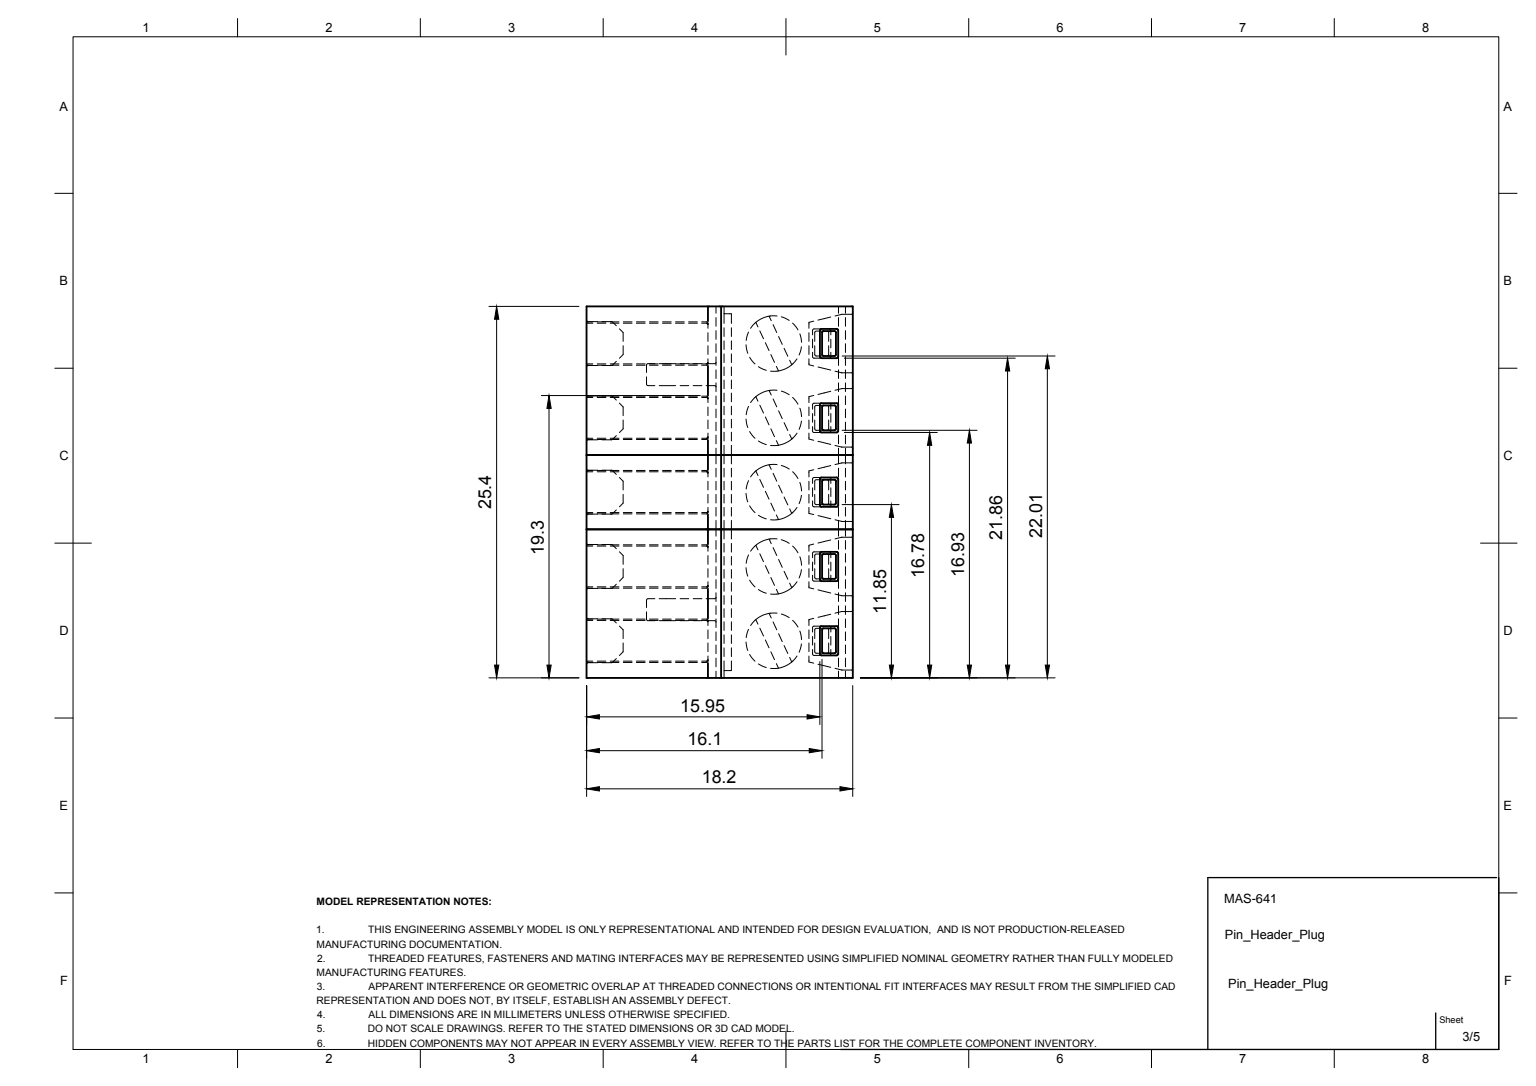
ISO-10303-21;
HEADER;
FILE_DESCRIPTION((''),'2;1');
FILE_NAME('Pin_Header_Plug.step','2026-10-09T09:55:32-07:00',(''),(''),'','','');
FILE_SCHEMA (('AUTOMOTIVE_DESIGN { 1 0 10303 214 3 1 1 }'));
ENDSEC;
DATA;
#10=MECHANICAL_DESIGN_GEOMETRIC_PRESENTATION_REPRESENTATION('',(#79661,#79662,#79663,#79664,#79665,#79666,#79667,#79668,#79669,#79670,#79671,#79672,#79673,#79674,#79675,#79676,#79677,#79678,#79679,#79680,#79681,#79682,#79683,#79684,#79685,#79686,#79687,#79688,#79689,#79690,#79691,#79692,#79693,#79694,#79695,#79696,#79697,#79698,#79699,#79700,#79701,#79702,#79703,#79704,#79705,#79706,#79707,#79708,#79709,#79710,#79711,#79712,#79713,#79714,#79715,#79716,#79717,#79718,#79719,#79720,#79721,#79722,#79723,#79724,#79725,#79726,#79727,#79728,#79729,#79730,#79731,#79732,#79733,#79734,#79735,#79736,#79737,#79738,#79739,#79740,#79741,#79742,#79743,#79744,#79745,#79746,#79747,#79748,#79749,#79750,#79751,#79752,#79753,#79754,#79755,#79756,#79757,#79758,#79759,#79760,#79761,#79762,#79763,#79764,#79765,#79766,#79767,#79768,#79769,#79770,#79771,#79772,#79773,#79774,#79775,#79776,#79777,#79778,#79779,#79780,#79781,#79782,#79783,#79784,#79785,#79786,#79787,#79788,#79789,#79790,#79791,#79792,#79793,#79794,#79795,#79796,#79797,#79798,#79799,#79800,#79801,#79802,#79803,#79804,#79805,#79806,#79807,#79808,#79809,#79810,#79811,#79812,#79813,#79814,#79815,#79816,#79817,#79818,#79819,#79820,#79821,#79822,#79823,#79824,#79825,#79826,#79827,#79828,#79829,#79830,#79831,#79832,#79833,#79834,#79835,#79836,#79837,#79838,#79839,#79840,#79841,#79842,#79843,#79844,#79845,#79846,#79847,#79848,#79849,#79850,#79851,#79852,#79853,#79854,#79855,#79856,#79857,#79858,#79859,#79860,#79861,#79862,#79863,#79864,#79865,#79866,#79867,#79868,#79869,#79870,#79871,#79872,#79873,#79874,#79875,#79876,#79877,#79878,#79879,#79880,#79881,#79882,#79883,#79884,#79885,#79886,#79887,#79888,#79889,#79890,#79891,#79892,#79893,#79894,#79895,#79896,#79897,#79898,#79899,#79900,#79901,#79902,#79903,#79904,#79905,#79906,#79907,#79908,#79909,#79910,#79911,#79912,#79913,#79914,#79915,#79916,#79917,#79918,#79919,#79920,#79921,#79922,#79923,#79924,#79925,#79926,#79927,#79928,#79929,#79930,#79931,#79932,#79933,#79934,#79935,#79936,#79937,#79938,#79939,#79940,#79941,#79942,#79943,#79944,#79945,#79946,#79947,#79948,#79949,#79950,#79951,#79952,#79953,#79954,#79955,#79956,#79957,#79958,#79959,#79960,#79961,#79962,#79963,#79964,#79965,#79966,#79967,#79968,#79969,#79970,#79971,#79972,#79973,#79974,#79975,#79976,#79977,#79978,#79979,#79980,#79981,#79982,#79983,#79984,#79985,#79986,#79987,#79988,#79989,#79990,#79991,#79992,#79993,#79994,#79995,#79996,#79997,#79998,#79999,#80000,#80001,#80002,#80003,#80004,#80005,#80006,#80007,#80008,#80009,#80010,#80011,#80012,#80013,#80014,#80015,#80016,#80017,#80018,#80019,#80020,#80021,#80022,#80023,#80024,#80025,#80026,#80027,#80028,#80029,#80030,#80031,#80032,#80033,#80034,#80035,#80036,#80037,#80038,#80039,#80040,#80041,#80042,#80043,#80044,#80045,#80046,#80047,#80048,#80049,#80050,#80051,#80052,#80053,#80054,#80055,#80056,#80057,#80058,#80059,#80060,#80061,#80062,#80063,#80064,#80065,#80066,#80067,#80068,#80069,#80070,#80071,#80072,#80073,#80074,#80075,#80076,#80077,#80078,#80079,#80080,#80081,#80082,#80083,#80084,#80085,#80086,#80087,#80088,#80089,#80090,#80091,#80092,#80093,#80094,#80095,#80096,#80097,#80098,#80099,#80100,#80101,#80102,#80103,#80104,#80105,#80106,#80107,#80108,#80109,#80110,#80111,#80112,#80113,#80114,#80115,#80116,#80117,#80118,#80119,#80120,#80121,#80122,#80123,#80124,#80125,#80126,#80127,#80128,#80129,#80130,#80131,#80132,#80133,#80134,#80135,#80136,#80137,#80138,#80139,#80140,#80141,#80142,#80143,#80144,#80145,#80146,#80147,#80148,#80149,#80150,#80151,#80152,#80153,#80154,#80155,#80156,#80157,#80158,#80159,#80160,#80161,#80162,#80163,#80164,#80165,#80166,#80167,#80168,#80169,#80170,#80171,#80172,#80173,#80174,#80175,#80176,#80177,#80178,#80179,#80180,#80181,#80182,#80183,#80184,#80185,#80186,#80187,#80188,#80189,#80190,#80191,#80192,#80193,#80194,#80195,#80196,#80197,#80198,#80199,#80200,#80201,#80202,#80203,#80204,#80205,#80206,#80207,#80208,#80209,#80210,#80211,#80212,#80213,#80214,#80215,#80216,#80217,#80218,#80219,#80220,#80221,#80222,#80223,#80224,#80225,#80226,#80227,#80228,#80229,#80230,#80231,#80232,#80233,#80234,#80235,#80236,#80237,#80238,#80239,#80240,#80241,#80242,#80243,#80244,#80245,#80246,#80247,#80248,#80249,#80250,#80251,#80252,#80253,#80254,#80255,#80256,#80257,#80258,#80259,#80260,#80261,#80262,#80263,#80264,#80265,#80266,#80267,#80268,#80269,#80270,#80271,#80272,#80273,#80274,#80275,#80276,#80277,#80278,#80279,#80280,#80281,#80282,#80283,#80284,#80285,#80286,#80287,#80288,#80289,#80290,#80291,#80292,#80293,#80294,#80295,#80296,#80297,#80298,#80299,#80300,#80301,#80302,#80303,#80304,#80305,#80306,#80307,#80308,#80309,#80310,#80311,#80312,#80313,#80314,#80315,#80316,#80317,#80318,#80319,#80320,#80321,#80322,#80323,#80324,#80325,#80326,#80327,#80328,#80329,#80330,#80331,#80332,#80333,#80334,#80335,#80336,#80337,#80338,#80339,#80340,#80341,#80342,#80343,#80344,#80345,#80346,#80347,#80348,#80349,#80350,#80351,#80352,#80353,#80354,#80355,#80356,#80357,#80358,#80359,#80360,#80361,#80362,#80363,#80364,#80365,#80366,#80367,#80368,#80369,#80370,#80371,#80372,#80373,#80374,#80375,#80376,#80377,#80378,#80379,#80380,#80381,#80382,#80383,#80384,#80385,#80386,#80387,#80388,#80389,#80390,#80391,#80392,#80393,#80394,#80395,#80396,#80397,#80398,#80399,#80400,#80401,#80402,#80403,#80404,#80405,#80406,#80407,#80408,#80409,#80410,#80411,#80412,#80413,#80414,#80415,#80416,#80417,#80418,#80419,#80420,#80421,#80422,#80423,#80424,#80425,#80426,#80427,#80428,#80429,#80430,#80431,#80432,#80433,#80434,#80435,#80436,#80437,#80438,#80439,#80440,#80441,#80442,#80443,#80444,#80445,#80446,#80447,#80448,#80449,#80450,#80451,#80452,#80453,#80454,#80455,#80456,#80457,#80458,#80459,#80460,#80461,#80462,#80463,#80464,#80465,#80466,#80467,#80468,#80469,#80470,#80471,#80472,#80473,#80474,#80475,#80476,#80477,#80478,#80479,#80480,#80481,#80482,#80483,#80484,#80485,#80486,#80487,#80488,#80489,#80490,#80491,#80492,#80493,#80494,#80495,#80496,#80497,#80498,#80499,#80500,#80501,#80502,#80503,#80504,#80505,#80506,#80507,#80508,#80509,#80510,#80511,#80512,#80513,#80514,#80515,#80516,#80517,#80518,#80519,#80520,#80521,#80522,#80523,#80524,#80525,#80526,#80527,#80528,#80529,#80530,#80531,#80532,#80533,#80534,#80535,#80536,#80537,#80538,#80539,#80540,#80541,#80542,#80543,#80544,#80545,#80546,#80547,#80548,#80549,#80550,#80551,#80552,#80553,#80554,#80555,#80556,#80557,#80558,#80559,#80560,#80561,#80562,#80563,#80564,#80565,#80566,#80567,#80568,#80569,#80570,#80571,#80572,#80573,#80574,#80575,#80576,#80577,#80578,#80579,#80580,#80581,#80582,#80583,#80584,#80585,#80586,#80587,#80588,#80589,#80590,#80591,#80592,#80593,#80594,#80595,#80596,#80597,#80598,#80599,#80600,#80601,#80602,#80603,#80604,#80605,#80606,#80607,#80608,#80609,#80610,#80611,#80612,#80613,#80614,#80615,#80616,#80617,#80618,#80619,#80620,#80621,#80622,#80623,#80624,#80625,#80626,#80627,#80628,#80629,#80630,#80631,#80632,#80633,#80634,#80635,#80636,#80637,#80638,#80639,#80640,#80641,#80642,#80643,#80644,#80645,#80646,#80647,#80648,#80649,#80650,#80651,#80652,#80653,#80654,#80655,#80656,#80657,#80658,#80659,#80660,#80661,#80662,#80663,#80664,#80665,#80666,#80667,#80668,#80669,#80670,#80671,#80672,#80673,#80674,#80675,#80676,#80677,#80678,#80679,#80680,#80681,#80682,#80683,#80684,#80685,#80686,#80687,#80688,#80689,#80690,#80691,#80692,#80693,#80694,#80695,#80696,#80697,#80698,#80699,#80700,#80701,#80702,#80703,#80704,#80705,#80706,#80707,#80708,#80709,#80710,#80711,#80712,#80713,#80714,#80715,#80716,#80717,#80718,#80719,#80720,#80721,#80722,#80723,#80724,#80725,#80726,#80727,#80728,#80729,#80730,#80731,#80732,#80733,#80734,#80735,#80736,#80737,#80738,#80739,#80740,#80741,#80742,#80743,#80744,#80745,#80746,#80747,#80748,#80749,#80750,#80751,#80752,#80753,#80754,#80755,#80756,#80757,#80758,#80759,#80760,#80761,#80762,#80763,#80764,#80765,#80766,#80767,#80768,#80769,#80770,#80771,#80772,#80773,#80774,#80775,#80776,#80777,#80778,#80779),#170127);
#23=SHAPE_REPRESENTATION_RELATIONSHIP('SRR','None',#170144,#26) ;
#26=ADVANCED_BREP_SHAPE_REPRESENTATION('',(#29,#30,#31),#170124) ;
#29=MANIFOLD_SOLID_BREP('Body1',#91083) ;
#30=MANIFOLD_SOLID_BREP('Body2',#91084) ;
#31=MANIFOLD_SOLID_BREP('Body3',#91085) ;
#34=(
BOUNDED_SURFACE()
B_SPLINE_SURFACE(3,2,((#133940,#133941,#133942),(#133943,#133944,#133945),
(#133946,#133947,#133948),(#133949,#133950,#133951),(#133952,#133953,#133954),
(#133955,#133956,#133957)),.UNSPECIFIED.,.F.,.F.,.F.)
B_SPLINE_SURFACE_WITH_KNOTS((4,2,4),(3,3),(3.14159265358979,3.92699081698724,
4.71238898038469),(0.,1.),.UNSPECIFIED.)
GEOMETRIC_REPRESENTATION_ITEM()
RATIONAL_B_SPLINE_SURFACE(((1.,0.934721701546417,1.),(1.,0.934869636336921,
1.),(1.,0.913780519322362,1.),(1.,0.83464631504231,1.),(1.,0.776518516961033,
1.),(1.,0.707106781186548,1.)))
REPRESENTATION_ITEM('')
SURFACE()
) ;
#35=(
BOUNDED_SURFACE()
B_SPLINE_SURFACE(3,2,((#133968,#133969,#133970),(#133971,#133972,#133973),
(#133974,#133975,#133976),(#133977,#133978,#133979)),.UNSPECIFIED.,.F.,
 .F.,.F.)
B_SPLINE_SURFACE_WITH_KNOTS((4,4),(3,3),(1.5707963267949,2.41495031290807),
(0.,1.),.UNSPECIFIED.)
GEOMETRIC_REPRESENTATION_ITEM()
RATIONAL_B_SPLINE_SURFACE(((1.,0.707106781186547,1.),(1.,0.730803471035897,
1.),(1.,0.752906082887246,1.),(1.,0.76729220397862,1.)))
REPRESENTATION_ITEM('')
SURFACE()
) ;
#36=(
BOUNDED_SURFACE()
B_SPLINE_SURFACE(3,2,((#133996,#133997,#133998),(#133999,#134000,#134001),
(#134002,#134003,#134004),(#134005,#134006,#134007),(#134008,#134009,#134010),
(#134011,#134012,#134013)),.UNSPECIFIED.,.F.,.F.,.F.)
B_SPLINE_SURFACE_WITH_KNOTS((4,2,4),(3,3),(1.56955149927804,2.35619449019234,
3.14283748110665),(-0.00124482751686043,1.),.UNSPECIFIED.)
GEOMETRIC_REPRESENTATION_ITEM()
RATIONAL_B_SPLINE_SURFACE(((1.00073060381457,0.70654415785643,1.),(1.00062673753069,
0.748263304672891,1.),(1.00053422463656,0.785422225437728,1.),(1.00040682904418,
0.836592203069559,1.),(1.00037181710676,0.850655170404881,1.),(1.00037229282027,
0.850464094333141,1.)))
REPRESENTATION_ITEM('')
SURFACE()
) ;
#37=(
BOUNDED_SURFACE()
B_SPLINE_SURFACE(3,2,((#134016,#134017,#134018),(#134019,#134020,#134021),
(#134022,#134023,#134024),(#134025,#134026,#134027),(#134028,#134029,#134030),
(#134031,#134032,#134033)),.UNSPECIFIED.,.F.,.F.,.F.)
B_SPLINE_SURFACE_WITH_KNOTS((4,2,4),(3,3),(4.71238898038469,5.49778714378214,
6.28318530717959),(0.,1.),.UNSPECIFIED.)
GEOMETRIC_REPRESENTATION_ITEM()
RATIONAL_B_SPLINE_SURFACE(((1.,0.707106781186548,1.),(1.,0.776518516961036,
1.),(1.,0.834646315042305,1.),(1.,0.913780519322366,1.),(1.,0.934869636336917,
1.),(1.,0.934721701546417,1.)))
REPRESENTATION_ITEM('')
SURFACE()
) ;
#38=(
BOUNDED_SURFACE()
B_SPLINE_SURFACE(3,2,((#134041,#134042,#134043),(#134044,#134045,#134046),
(#134047,#134048,#134049),(#134050,#134051,#134052)),.UNSPECIFIED.,.F.,
 .F.,.F.)
B_SPLINE_SURFACE_WITH_KNOTS((4,4),(3,3),(0.726642340681724,1.5707963267949),
(0.,1.),.UNSPECIFIED.)
GEOMETRIC_REPRESENTATION_ITEM()
RATIONAL_B_SPLINE_SURFACE(((1.,0.76729220397862,1.),(1.,0.752906082887247,
1.),(1.,0.730803471035896,1.),(1.,0.707106781186548,1.)))
REPRESENTATION_ITEM('')
SURFACE()
) ;
#39=(
BOUNDED_SURFACE()
B_SPLINE_SURFACE(3,2,((#134068,#134069,#134070),(#134071,#134072,#134073),
(#134074,#134075,#134076),(#134077,#134078,#134079),(#134080,#134081,#134082),
(#134083,#134084,#134085)),.UNSPECIFIED.,.F.,.F.,.F.)
B_SPLINE_SURFACE_WITH_KNOTS((4,2,4),(3,3),(-0.00124482751684684,0.785398163397448,
1.57204115431174),(-0.00124482751684684,1.),.UNSPECIFIED.)
GEOMETRIC_REPRESENTATION_ITEM()
RATIONAL_B_SPLINE_SURFACE(((1.00037229282026,0.850464094333143,1.),(1.00037181710676,
0.850655170404876,1.),(1.00040682904417,0.83659220306957,1.),(1.00053422463656,
0.785422225437723,1.),(1.00062673753069,0.748263304672901,1.),(1.00073060381456,
0.706544157856436,1.)))
REPRESENTATION_ITEM('')
SURFACE()
) ;
#40=(
BOUNDED_SURFACE()
B_SPLINE_SURFACE(3,2,((#134097,#134098,#134099),(#134100,#134101,#134102),
(#134103,#134104,#134105),(#134106,#134107,#134108)),.UNSPECIFIED.,.F.,
 .F.,.F.)
B_SPLINE_SURFACE_WITH_KNOTS((4,4),(3,3),(1.10714871779409,1.5707963267949),
(0.,1.),.UNSPECIFIED.)
GEOMETRIC_REPRESENTATION_ITEM()
RATIONAL_B_SPLINE_SURFACE(((1.,0.743704326447946,1.),(1.,0.73267692820235,
1.),(1.,0.720087778783133,1.),(1.,0.707106781186547,1.)))
REPRESENTATION_ITEM('')
SURFACE()
) ;
#41=(
BOUNDED_SURFACE()
B_SPLINE_SURFACE(3,2,((#134116,#134117,#134118),(#134119,#134120,#134121),
(#134122,#134123,#134124),(#134125,#134126,#134127)),.UNSPECIFIED.,.F.,
 .F.,.F.)
B_SPLINE_SURFACE_WITH_KNOTS((4,4),(3,3),(1.5707963267949,2.0344439357957),
(0.,1.),.UNSPECIFIED.)
GEOMETRIC_REPRESENTATION_ITEM()
RATIONAL_B_SPLINE_SURFACE(((1.,0.707106781186547,1.),(1.,0.720087778783132,
1.),(1.,0.73267692820235,1.),(1.,0.743704326447946,1.)))
REPRESENTATION_ITEM('')
SURFACE()
) ;
#42=(
BOUNDED_SURFACE()
B_SPLINE_SURFACE(3,2,((#134402,#134403,#134404),(#134405,#134406,#134407),
(#134408,#134409,#134410),(#134411,#134412,#134413)),.UNSPECIFIED.,.F.,
 .F.,.F.)
B_SPLINE_SURFACE_WITH_KNOTS((4,4),(3,3),(0.000111059871785624,0.00024129664665087),
(0.,1.00030059112233),.UNSPECIFIED.)
GEOMETRIC_REPRESENTATION_ITEM()
RATIONAL_B_SPLINE_SURFACE(((1.,0.839985548969888,1.00009619784685),(1.,
0.797322032917078,1.00012184639519),(1.,0.734686009440384,1.00015950206038),
(1.,0.707018740085181,1.00017613513148)))
REPRESENTATION_ITEM('')
SURFACE()
) ;
#43=(
BOUNDED_SURFACE()
B_SPLINE_SURFACE(3,2,((#134415,#134416,#134417),(#134418,#134419,#134420),
(#134421,#134422,#134423),(#134424,#134425,#134426)),.UNSPECIFIED.,.F.,
 .F.,.F.)
B_SPLINE_SURFACE_WITH_KNOTS((4,4),(3,3),(3.14159265358979,3.68974201455418),
(0.,1.),.UNSPECIFIED.)
GEOMETRIC_REPRESENTATION_ITEM()
RATIONAL_B_SPLINE_SURFACE(((1.,0.860789971413512,1.),(1.,0.86080954675505,
1.),(1.,0.853709425573778,1.),(1.,0.840033633436872,1.)))
REPRESENTATION_ITEM('')
SURFACE()
) ;
#44=(
BOUNDED_SURFACE()
B_SPLINE_SURFACE(3,2,((#134432,#134433,#134434),(#134435,#134436,#134437),
(#134438,#134439,#134440),(#134441,#134442,#134443)),.UNSPECIFIED.,.F.,
 .F.,.F.)
B_SPLINE_SURFACE_WITH_KNOTS((4,4),(3,3),(2.59344329260966,3.14159265358979),
(0.,1.),.UNSPECIFIED.)
GEOMETRIC_REPRESENTATION_ITEM()
RATIONAL_B_SPLINE_SURFACE(((1.,0.840033633435697,1.),(1.,0.853709425573365,
1.),(1.,0.860809546755054,1.),(1.,0.860789971413512,1.)))
REPRESENTATION_ITEM('')
SURFACE()
) ;
#45=(
BOUNDED_SURFACE()
B_SPLINE_SURFACE(3,2,((#134445,#134446,#134447),(#134448,#134449,#134450),
(#134451,#134452,#134453),(#134454,#134455,#134456)),.UNSPECIFIED.,.F.,
 .F.,.F.)
B_SPLINE_SURFACE_WITH_KNOTS((4,4),(3,3),(0.000111059871788868,0.00024129664665087),
(-0.000300086749770041,1.),.UNSPECIFIED.)
GEOMETRIC_REPRESENTATION_ITEM()
RATIONAL_B_SPLINE_SURFACE(((1.00009603638463,0.839985629649273,1.),(1.00012164188345,
0.797322135108583,1.),(1.0001592343459,0.734686143216499,1.),(1.0001758394994,
0.707018887812483,1.)))
REPRESENTATION_ITEM('')
SURFACE()
) ;
#46=(
BOUNDED_SURFACE()
B_SPLINE_SURFACE(3,2,((#134540,#134541,#134542),(#134543,#134544,#134545),
(#134546,#134547,#134548),(#134549,#134550,#134551),(#134552,#134553,#134554),
(#134555,#134556,#134557),(#134558,#134559,#134560),(#134561,#134562,#134563),
(#134564,#134565,#134566),(#134567,#134568,#134569)),.UNSPECIFIED.,.F.,
 .F.,.F.)
B_SPLINE_SURFACE_WITH_KNOTS((4,2,2,2,4),(3,3),(0.00112100122803332,0.00145633576709043,
0.0015908372445872,0.00165808798333558,0.00178849406635728),(-0.000893324189270442,
1.00101552458207),.UNSPECIFIED.)
GEOMETRIC_REPRESENTATION_ITEM()
RATIONAL_B_SPLINE_SURFACE(((1.00061830890916,0.653576280075622,1.00070297498515),
(1.00045188087569,0.746821933830033,1.00051375768191),(1.00032243686652,
0.819346321742885,1.00036658868746),(1.00017052538066,0.904458700444864,
1.00019387570704),(1.00013074576008,0.926746272131238,1.0001486489963),
(1.00007983643892,0.955269549338581,1.0000907685764),(1.00006394848111,
0.964171192776746,1.00007270505389),(1.00002748579919,0.98460036292333,
1.00003124947579),(1.00001632684003,0.990852461324379,1.00001856250163),
(1.00006581963707,0.963122828765907,1.00007483243037)))
REPRESENTATION_ITEM('')
SURFACE()
) ;
#47=(
BOUNDED_SURFACE()
B_SPLINE_SURFACE(3,2,((#134611,#134612,#134613),(#134614,#134615,#134616),
(#134617,#134618,#134619),(#134620,#134621,#134622),(#134623,#134624,#134625),
(#134626,#134627,#134628),(#134629,#134630,#134631),(#134632,#134633,#134634),
(#134635,#134636,#134637),(#134638,#134639,#134640)),.UNSPECIFIED.,.F.,
 .F.,.F.)
B_SPLINE_SURFACE_WITH_KNOTS((4,2,2,2,4),(3,3),(0.00112100122803331,0.00145633576709043,
0.00159083724458721,0.00165808798333559,0.00178849406635727),(-0.00113559264167203,
1.),.UNSPECIFIED.)
GEOMETRIC_REPRESENTATION_ITEM()
RATIONAL_B_SPLINE_SURFACE(((1.0007861837978,0.65384427084655,1.),(1.00057456947123,
0.747017790468101,1.),(1.00040998057203,0.819486074062728,1.),(1.00021682413014,
0.904532610471948,1.),(1.00016624408395,0.926802940661382,1.),(1.00010151255112,
0.955304152477056,1.),(1.00008131090948,0.964198909671164,1.),(1.00003494837236,
0.984612275966157,1.),(1.00002075968326,0.990859537791147,1.),(1.00008369009644,
0.963151356666802,0.999999999999999)))
REPRESENTATION_ITEM('')
SURFACE()
) ;
#48=(
BOUNDED_SURFACE()
B_SPLINE_SURFACE(3,2,((#134677,#134678,#134679),(#134680,#134681,#134682),
(#134683,#134684,#134685),(#134686,#134687,#134688),(#134689,#134690,#134691),
(#134692,#134693,#134694),(#134695,#134696,#134697),(#134698,#134699,#134700),
(#134701,#134702,#134703),(#134704,#134705,#134706),(#134707,#134708,#134709),
(#134710,#134711,#134712),(#134713,#134714,#134715),(#134716,#134717,#134718),
(#134719,#134720,#134721),(#134722,#134723,#134724)),.UNSPECIFIED.,.F.,
 .F.,.F.)
B_SPLINE_SURFACE_WITH_KNOTS((4,2,2,2,2,2,2,4),(3,3),(5.62831031780675E-15,
3.85995771599554E-5,5.7899365737119E-5,6.75492600257008E-5,7.23742071699917E-5,
7.47866807421371E-5,7.59929175282099E-5,7.71991543142826E-5),(0.,1.00107899067816),
 .UNSPECIFIED.)
GEOMETRIC_REPRESENTATION_ITEM()
RATIONAL_B_SPLINE_SURFACE(((1.,0.976255617118809,1.00005123993557),(1.,
0.981339981891257,1.00004026797119),(1.,0.986086237829177,1.00003002563936),
(1.,0.992269463037034,1.00001668235464),(1.,0.994174411180039,1.00001257151206),
(1.,0.996706913506704,1.00000710641926),(1.,0.997492596832092,1.00000541092929),
(1.,0.998537621803389,1.00000315578488),(1.,0.998865045809511,1.00000244920998),
(1.,0.999323526852931,1.00000145981644),(1.,0.999468419970869,1.00000114713979),
(1.,0.99959844684718,1.00000086654422),(1.,0.999614491362717,1.00000083192045),
(1.,0.999732489024762,1.0000005772837),(1.,0.999724369239699,1.00000059480604),
(1.,1.,1.)))
REPRESENTATION_ITEM('')
SURFACE()
) ;
#49=(
BOUNDED_SURFACE()
B_SPLINE_SURFACE(3,2,((#134726,#134727,#134728),(#134729,#134730,#134731),
(#134732,#134733,#134734),(#134735,#134736,#134737),(#134738,#134739,#134740),
(#134741,#134742,#134743),(#134744,#134745,#134746),(#134747,#134748,#134749),
(#134750,#134751,#134752),(#134753,#134754,#134755)),.UNSPECIFIED.,.F.,
 .F.,.F.)
B_SPLINE_SURFACE_WITH_KNOTS((4,2,2,2,4),(3,3),(-0.000110707928511331,0.000553539642556654,
0.000830309463834981,0.000968694374474144,0.00121778721363011),(0.,1.00563383762696),
 .UNSPECIFIED.)
GEOMETRIC_REPRESENTATION_ITEM()
RATIONAL_B_SPLINE_SURFACE(((1.,0.710139408519195,1.00326605501372),(1.,
0.691948125896918,1.00347102847876),(1.,0.728232377173825,1.00306218931854),
(1.,0.818030374423679,1.00205037464707),(1.,0.849110759469254,1.00170017096161),
(1.,0.897979778369935,1.00114953072666),(1.,0.914666724297516,1.00096150763897),
(1.,0.961090538823392,1.00043841917284),(1.,0.990973799041213,1.00010170430118),
(1.,0.9924634551618,1.00008491933977)))
REPRESENTATION_ITEM('')
SURFACE()
) ;
#50=(
BOUNDED_SURFACE()
B_SPLINE_SURFACE(3,2,((#134757,#134758,#134759),(#134760,#134761,#134762),
(#134763,#134764,#134765),(#134766,#134767,#134768),(#134769,#134770,#134771),
(#134772,#134773,#134774),(#134775,#134776,#134777),(#134778,#134779,#134780),
(#134781,#134782,#134783),(#134784,#134785,#134786)),.UNSPECIFIED.,.F.,
 .F.,.F.)
B_SPLINE_SURFACE_WITH_KNOTS((4,2,2,2,4),(3,3),(-0.000137915648493858,0.000139027965246065,
0.000278055930499747,0.00055611186100711,0.00125013859505181),(-0.000741678185408241,
1.00283457365794),.UNSPECIFIED.)
GEOMETRIC_REPRESENTATION_ITEM()
RATIONAL_B_SPLINE_SURFACE(((1.00001340810331,0.990935328833035,1.00005135076282),
(1.00000300543757,0.997968146378466,1.00001151031642),(1.00005311279897,
0.964092605306839,1.00020341301682),(1.00012590576281,0.914880254704014,
1.00048219772916),(1.00015093966337,0.897955856705928,1.00057807332481),
(1.00022375355351,0.84872935869733,1.00085693818127),(1.00026920263019,
0.818003093714666,1.00103100044084),(1.00040494517418,0.726233102310977,
1.0015508713745),(1.00045889592378,0.689759203409617,1.00175749360019),
(1.00042429005305,0.71315481959354,1.00162495898138)))
REPRESENTATION_ITEM('')
SURFACE()
) ;
#51=(
BOUNDED_SURFACE()
B_SPLINE_SURFACE(3,2,((#134788,#134789,#134790),(#134791,#134792,#134793),
(#134794,#134795,#134796),(#134797,#134798,#134799),(#134800,#134801,#134802),
(#134803,#134804,#134805),(#134806,#134807,#134808),(#134809,#134810,#134811),
(#134812,#134813,#134814),(#134815,#134816,#134817),(#134818,#134819,#134820),
(#134821,#134822,#134823),(#134824,#134825,#134826),(#134827,#134828,#134829),
(#134830,#134831,#134832),(#134833,#134834,#134835)),.UNSPECIFIED.,.F.,
 .F.,.F.)
B_SPLINE_SURFACE_WITH_KNOTS((4,2,2,2,2,2,2,4),(3,3),(7.77892019462184E-15,
3.88447601478312E-5,5.82671402178573E-5,6.79783302528704E-5,7.28339252703769E-5,
7.52617227791302E-5,7.64756215335068E-5,7.76895202878834E-5),(-0.00120945525754678,
1.01080070868962),.UNSPECIFIED.)
GEOMETRIC_REPRESENTATION_ITEM()
RATIONAL_B_SPLINE_SURFACE(((1.00005744302265,0.975995723233526,1.00051789333956),
(1.00004519813151,0.981112615457369,1.0004074961621),(1.00003362760161,
0.985947705765597,1.00030317887351),(1.00001854219783,0.992251590743247,
1.00016717227456),(1.00001393966879,0.994174894491123,1.0001256769106),
(1.00000788875349,0.996703449551652,1.00007112322264),(1.00000601414708,
0.997486809637524,1.00005422219392),(1.00000351698944,0.998530321282699,
1.00003170838373),(1.00000273459082,0.998857269833632,1.0000246544542),
(1.00000163903614,0.999315079966001,1.00001477718022),(1.00000129000885,
0.999460931405222,1.00001163042892),(1.0000009745592,0.999592751431242,
1.000008786406),(1.00000093560708,0.99960902873406,1.00000843522246),(1.00000065019919,
0.999728294915416,1.00000586204929),(1.00000066918571,0.99972036083143,
1.00000603322751),(1.,1.,1.)))
REPRESENTATION_ITEM('')
SURFACE()
) ;
#52=(
BOUNDED_SURFACE()
B_SPLINE_SURFACE(3,2,((#135308,#135309,#135310),(#135311,#135312,#135313),
(#135314,#135315,#135316),(#135317,#135318,#135319),(#135320,#135321,#135322),
(#135323,#135324,#135325)),.UNSPECIFIED.,.F.,.F.,.F.)
B_SPLINE_SURFACE_WITH_KNOTS((4,2,4),(3,3),(3.14159265358979,3.92699081698724,
4.71238898038469),(0.,1.),.UNSPECIFIED.)
GEOMETRIC_REPRESENTATION_ITEM()
RATIONAL_B_SPLINE_SURFACE(((1.,0.934721701546417,1.),(1.,0.934869636336909,
1.),(1.,0.913780519322377,1.),(1.,0.834646315042295,1.),(1.,0.776518516961044,
1.),(1.,0.707106781186548,1.)))
REPRESENTATION_ITEM('')
SURFACE()
) ;
#53=(
BOUNDED_SURFACE()
B_SPLINE_SURFACE(3,2,((#135336,#135337,#135338),(#135339,#135340,#135341),
(#135342,#135343,#135344),(#135345,#135346,#135347)),.UNSPECIFIED.,.F.,
 .F.,.F.)
B_SPLINE_SURFACE_WITH_KNOTS((4,4),(3,3),(1.5707963267949,2.41495031290807),
(0.,1.),.UNSPECIFIED.)
GEOMETRIC_REPRESENTATION_ITEM()
RATIONAL_B_SPLINE_SURFACE(((1.,0.707106781186547,1.),(1.,0.730803471035898,
1.),(1.,0.752906082887245,1.),(1.,0.76729220397862,1.)))
REPRESENTATION_ITEM('')
SURFACE()
) ;
#54=(
BOUNDED_SURFACE()
B_SPLINE_SURFACE(3,2,((#135364,#135365,#135366),(#135367,#135368,#135369),
(#135370,#135371,#135372),(#135373,#135374,#135375),(#135376,#135377,#135378),
(#135379,#135380,#135381)),.UNSPECIFIED.,.F.,.F.,.F.)
B_SPLINE_SURFACE_WITH_KNOTS((4,2,4),(3,3),(1.5695514992781,2.35619449019234,
3.14283748110659),(-0.00124482751679711,1.),.UNSPECIFIED.)
GEOMETRIC_REPRESENTATION_ITEM()
RATIONAL_B_SPLINE_SURFACE(((1.00073060381453,0.706544157856458,1.),(1.00062673753066,
0.748263304672962,1.),(1.00053422463654,0.785422225437678,1.),(1.00040682904416,
0.836592203069638,1.),(1.00037181710674,0.850655170404834,1.),(1.00037229282025,
0.850464094333151,1.)))
REPRESENTATION_ITEM('')
SURFACE()
) ;
#55=(
BOUNDED_SURFACE()
B_SPLINE_SURFACE(3,2,((#135384,#135385,#135386),(#135387,#135388,#135389),
(#135390,#135391,#135392),(#135393,#135394,#135395),(#135396,#135397,#135398),
(#135399,#135400,#135401)),.UNSPECIFIED.,.F.,.F.,.F.)
B_SPLINE_SURFACE_WITH_KNOTS((4,2,4),(3,3),(4.71238898038469,5.49778714378214,
6.28318530717959),(0.,1.),.UNSPECIFIED.)
GEOMETRIC_REPRESENTATION_ITEM()
RATIONAL_B_SPLINE_SURFACE(((1.,0.707106781186548,1.),(1.,0.776518516961043,
1.),(1.,0.834646315042294,1.),(1.,0.913780519322378,1.),(1.,0.934869636336909,
1.),(1.,0.934721701546417,1.)))
REPRESENTATION_ITEM('')
SURFACE()
) ;
#56=(
BOUNDED_SURFACE()
B_SPLINE_SURFACE(3,2,((#135409,#135410,#135411),(#135412,#135413,#135414),
(#135415,#135416,#135417),(#135418,#135419,#135420)),.UNSPECIFIED.,.F.,
 .F.,.F.)
B_SPLINE_SURFACE_WITH_KNOTS((4,4),(3,3),(0.726642340681723,1.5707963267949),
(0.,1.),.UNSPECIFIED.)
GEOMETRIC_REPRESENTATION_ITEM()
RATIONAL_B_SPLINE_SURFACE(((1.,0.767292203978618,1.),(1.,0.752906082887251,
1.),(1.,0.730803471035892,1.),(1.,0.70710678118655,1.)))
REPRESENTATION_ITEM('')
SURFACE()
) ;
#57=(
BOUNDED_SURFACE()
B_SPLINE_SURFACE(3,2,((#135436,#135437,#135438),(#135439,#135440,#135441),
(#135442,#135443,#135444),(#135445,#135446,#135447),(#135448,#135449,#135450),
(#135451,#135452,#135453)),.UNSPECIFIED.,.F.,.F.,.F.)
B_SPLINE_SURFACE_WITH_KNOTS((4,2,4),(3,3),(-0.00124482751677724,0.785398163397448,
1.57204115431167),(-0.00124482751677724,1.),.UNSPECIFIED.)
GEOMETRIC_REPRESENTATION_ITEM()
RATIONAL_B_SPLINE_SURFACE(((1.00037229282024,0.850464094333154,1.),(1.00037181710674,
0.850655170404788,1.),(1.00040682904415,0.836592203069706,1.),(1.00053422463653,
0.785422225437613,1.),(1.00062673753065,0.748263304673021,1.),(1.00073060381452,
0.706544157856467,1.)))
REPRESENTATION_ITEM('')
SURFACE()
) ;
#58=(
BOUNDED_SURFACE()
B_SPLINE_SURFACE(3,2,((#135465,#135466,#135467),(#135468,#135469,#135470),
(#135471,#135472,#135473),(#135474,#135475,#135476)),.UNSPECIFIED.,.F.,
 .F.,.F.)
B_SPLINE_SURFACE_WITH_KNOTS((4,4),(3,3),(1.10714871779409,1.5707963267949),
(0.,1.),.UNSPECIFIED.)
GEOMETRIC_REPRESENTATION_ITEM()
RATIONAL_B_SPLINE_SURFACE(((1.,0.743704326447947,1.),(1.,0.732676928202351,
1.),(1.,0.720087778783133,1.),(1.,0.707106781186548,1.)))
REPRESENTATION_ITEM('')
SURFACE()
) ;
#59=(
BOUNDED_SURFACE()
B_SPLINE_SURFACE(3,2,((#135484,#135485,#135486),(#135487,#135488,#135489),
(#135490,#135491,#135492),(#135493,#135494,#135495)),.UNSPECIFIED.,.F.,
 .F.,.F.)
B_SPLINE_SURFACE_WITH_KNOTS((4,4),(3,3),(1.5707963267949,2.0344439357957),
(0.,1.),.UNSPECIFIED.)
GEOMETRIC_REPRESENTATION_ITEM()
RATIONAL_B_SPLINE_SURFACE(((1.,0.707106781186548,1.),(1.,0.720087778783135,
1.),(1.,0.732676928202346,1.),(1.,0.74370432644795,1.)))
REPRESENTATION_ITEM('')
SURFACE()
) ;
#60=(
BOUNDED_SURFACE()
B_SPLINE_SURFACE(3,2,((#135745,#135746,#135747),(#135748,#135749,#135750),
(#135751,#135752,#135753),(#135754,#135755,#135756)),.UNSPECIFIED.,.F.,
 .F.,.F.)
B_SPLINE_SURFACE_WITH_KNOTS((4,4),(3,3),(0.000111059871785624,0.00024129664665087),
(0.,1.00030059112235),.UNSPECIFIED.)
GEOMETRIC_REPRESENTATION_ITEM()
RATIONAL_B_SPLINE_SURFACE(((1.,0.839985548969885,1.00009619784685),(1.,
0.797322032917072,1.0001218463952),(1.,0.734686009440383,1.00015950206039),
(1.,0.707018740085174,1.00017613513149)))
REPRESENTATION_ITEM('')
SURFACE()
) ;
#61=(
BOUNDED_SURFACE()
B_SPLINE_SURFACE(3,2,((#135758,#135759,#135760),(#135761,#135762,#135763),
(#135764,#135765,#135766),(#135767,#135768,#135769)),.UNSPECIFIED.,.F.,
 .F.,.F.)
B_SPLINE_SURFACE_WITH_KNOTS((4,4),(3,3),(3.14159265358979,3.68974201455419),
(0.,1.),.UNSPECIFIED.)
GEOMETRIC_REPRESENTATION_ITEM()
RATIONAL_B_SPLINE_SURFACE(((1.,0.860789971413512,1.),(1.,0.860809546755051,
1.),(1.,0.853709425573777,1.),(1.,0.840033633436872,1.)))
REPRESENTATION_ITEM('')
SURFACE()
) ;
#62=(
BOUNDED_SURFACE()
B_SPLINE_SURFACE(3,2,((#135772,#135773,#135774),(#135775,#135776,#135777),
(#135778,#135779,#135780),(#135781,#135782,#135783)),.UNSPECIFIED.,.F.,
 .F.,.F.)
B_SPLINE_SURFACE_WITH_KNOTS((4,4),(3,3),(2.59344329260966,3.14159265358979),
(0.,1.),.UNSPECIFIED.)
GEOMETRIC_REPRESENTATION_ITEM()
RATIONAL_B_SPLINE_SURFACE(((1.,0.840033633435696,1.),(1.,0.853709425573366,
1.),(1.,0.860809546755054,1.),(1.,0.860789971413512,1.)))
REPRESENTATION_ITEM('')
SURFACE()
) ;
#63=(
BOUNDED_SURFACE()
B_SPLINE_SURFACE(3,2,((#135785,#135786,#135787),(#135788,#135789,#135790),
(#135791,#135792,#135793),(#135794,#135795,#135796)),.UNSPECIFIED.,.F.,
 .F.,.F.)
B_SPLINE_SURFACE_WITH_KNOTS((4,4),(3,3),(0.000111059871788867,0.00024129664665087),
(-0.000300086749674745,1.),.UNSPECIFIED.)
GEOMETRIC_REPRESENTATION_ITEM()
RATIONAL_B_SPLINE_SURFACE(((1.0000960363846,0.839985629649289,1.),(1.00012164188341,
0.797322135108605,1.),(1.00015923434585,0.734686143216524,1.),(1.00017583949934,
0.707018887812511,1.)))
REPRESENTATION_ITEM('')
SURFACE()
) ;
#64=(
BOUNDED_SURFACE()
B_SPLINE_SURFACE(3,2,((#135878,#135879,#135880),(#135881,#135882,#135883),
(#135884,#135885,#135886),(#135887,#135888,#135889),(#135890,#135891,#135892),
(#135893,#135894,#135895),(#135896,#135897,#135898),(#135899,#135900,#135901),
(#135902,#135903,#135904),(#135905,#135906,#135907)),.UNSPECIFIED.,.F.,
 .F.,.F.)
B_SPLINE_SURFACE_WITH_KNOTS((4,2,2,2,4),(3,3),(0.00112100122803333,0.00145633576709043,
0.0015908372445872,0.00165808798333558,0.00178849406635727),(-0.000893324189226138,
1.00101552458159),.UNSPECIFIED.)
GEOMETRIC_REPRESENTATION_ITEM()
RATIONAL_B_SPLINE_SURFACE(((1.00061830890913,0.653576280075824,1.00070297498481),
(1.00045188087567,0.746821933830164,1.00051375768166),(1.0003224368665,
0.819346321742989,1.00036658868727),(1.00017052538065,0.904458700444912,
1.00019387570695),(1.00013074576007,0.926746272131305,1.00014864899623),
(1.00007983643891,0.955269549338591,1.00009076857636),(1.00006394848111,
0.964171192776766,1.00007270505385),(1.00002748579919,0.984600362923336,
1.00003124947577),(1.00001632684003,0.99085246132439,1.00001856250162),
(1.00006581963707,0.963122828765912,1.00007483243033)))
REPRESENTATION_ITEM('')
SURFACE()
) ;
#65=(
BOUNDED_SURFACE()
B_SPLINE_SURFACE(3,2,((#135948,#135949,#135950),(#135951,#135952,#135953),
(#135954,#135955,#135956),(#135957,#135958,#135959),(#135960,#135961,#135962),
(#135963,#135964,#135965),(#135966,#135967,#135968),(#135969,#135970,#135971),
(#135972,#135973,#135974),(#135975,#135976,#135977)),.UNSPECIFIED.,.F.,
 .F.,.F.)
B_SPLINE_SURFACE_WITH_KNOTS((4,2,2,2,4),(3,3),(0.00112100122803332,0.00145633576709043,
0.00159083724458721,0.00165808798333559,0.00178849406635728),(-0.00113559264173565,
1.),.UNSPECIFIED.)
GEOMETRIC_REPRESENTATION_ITEM()
RATIONAL_B_SPLINE_SURFACE(((1.00078618379784,0.653844270846546,1.),(1.00057456947127,
0.747017790468067,1.),(1.00040998057205,0.819486074062731,1.),(1.00021682413015,
0.904532610471937,1.),(1.00016624408396,0.926802940661352,1.),(1.00010151255113,
0.955304152477066,1.),(1.00008131090949,0.964198909671163,1.),(1.00003494837236,
0.984612275966154,1.),(1.00002075968326,0.990859537791153,1.),(1.00008369009645,
0.963151356666784,1.)))
REPRESENTATION_ITEM('')
SURFACE()
) ;
#66=(
BOUNDED_SURFACE()
B_SPLINE_SURFACE(3,2,((#136014,#136015,#136016),(#136017,#136018,#136019),
(#136020,#136021,#136022),(#136023,#136024,#136025),(#136026,#136027,#136028),
(#136029,#136030,#136031),(#136032,#136033,#136034),(#136035,#136036,#136037),
(#136038,#136039,#136040),(#136041,#136042,#136043),(#136044,#136045,#136046),
(#136047,#136048,#136049),(#136050,#136051,#136052),(#136053,#136054,#136055),
(#136056,#136057,#136058),(#136059,#136060,#136061)),.UNSPECIFIED.,.F.,
 .F.,.F.)
B_SPLINE_SURFACE_WITH_KNOTS((4,2,2,2,2,2,2,4),(3,3),(5.62805281979079E-15,
3.85995771599553E-5,5.7899365737119E-5,6.75492600257008E-5,7.23742071699917E-5,
7.47866807421372E-5,7.59929175282099E-5,7.71991543142826E-5),(0.,1.00107899067844),
 .UNSPECIFIED.)
GEOMETRIC_REPRESENTATION_ITEM()
RATIONAL_B_SPLINE_SURFACE(((1.,0.976255617118803,1.00005123993559),(1.,
0.981339981891199,1.0000402679712),(1.,0.986086237829182,1.00003002563937),
(1.,0.992269463037027,1.00001668235464),(1.,0.994174411180035,1.00001257151207),
(1.,0.996706913506705,1.00000710641926),(1.,0.997492596832093,1.00000541092929),
(1.,0.998537621803387,1.00000315578488),(1.,0.998865045809509,1.00000244920998),
(1.,0.999323526852929,1.00000145981644),(1.,0.999468419970868,1.00000114713979),
(1.,0.999598446847179,1.00000086654422),(1.,0.999614491362717,1.00000083192045),
(1.,0.999732489024762,1.0000005772837),(1.,0.999724369239699,1.00000059480604),
(1.,1.,1.)))
REPRESENTATION_ITEM('')
SURFACE()
) ;
#67=(
BOUNDED_SURFACE()
B_SPLINE_SURFACE(3,2,((#136063,#136064,#136065),(#136066,#136067,#136068),
(#136069,#136070,#136071),(#136072,#136073,#136074),(#136075,#136076,#136077),
(#136078,#136079,#136080),(#136081,#136082,#136083),(#136084,#136085,#136086),
(#136087,#136088,#136089),(#136090,#136091,#136092)),.UNSPECIFIED.,.F.,
 .F.,.F.)
B_SPLINE_SURFACE_WITH_KNOTS((4,2,2,2,4),(3,3),(-0.000110707928511331,0.000553539642556654,
0.000830309463834981,0.000968694374474145,0.00121778721363011),(0.,1.00563383762722),
 .UNSPECIFIED.)
GEOMETRIC_REPRESENTATION_ITEM()
RATIONAL_B_SPLINE_SURFACE(((1.,0.710139408519121,1.00326605501387),(1.,
0.691948125896839,1.00347102847892),(1.,0.728232377173756,1.00306218931868),
(1.,0.818030374423633,1.00205037464717),(1.,0.849110759469252,1.00170017096169),
(1.,0.897979778369892,1.00114953072671),(1.,0.914666724297501,1.00096150763901),
(1.,0.961090538823375,1.00043841917286),(1.,0.990973799041227,1.00010170430118),
(1.,0.992463455161771,1.00008491933978)))
REPRESENTATION_ITEM('')
SURFACE()
) ;
#68=(
BOUNDED_SURFACE()
B_SPLINE_SURFACE(3,2,((#136094,#136095,#136096),(#136097,#136098,#136099),
(#136100,#136101,#136102),(#136103,#136104,#136105),(#136106,#136107,#136108),
(#136109,#136110,#136111),(#136112,#136113,#136114),(#136115,#136116,#136117),
(#136118,#136119,#136120),(#136121,#136122,#136123)),.UNSPECIFIED.,.F.,
 .F.,.F.)
B_SPLINE_SURFACE_WITH_KNOTS((4,2,2,2,4),(3,3),(-0.000137915648493859,0.000139027965246065,
0.000278055930499747,0.000556111861007111,0.00125013859505181),(-0.000741678185857755,
1.00283457365566),.UNSPECIFIED.)
GEOMETRIC_REPRESENTATION_ITEM()
RATIONAL_B_SPLINE_SURFACE(((1.00001340810332,0.990935328833157,1.00005135076278),
(1.00000300543756,0.997968146378419,1.00001151031642),(1.00005311279899,
0.96409260530692,1.00020341301665),(1.00012590576288,0.914880254704161,
1.00048219772877),(1.00015093966347,0.897955856706116,1.00057807332434),
(1.00022375355364,0.8487293586976,1.00085693818058),(1.00026920263035,0.818003093714992,
1.00103100044001),(1.00040494517442,0.726233102311489,1.00155087137326),
(1.00045889592406,0.689759203410164,1.00175749359878),(1.0004242900533,
0.713154819594072,1.00162495898007)))
REPRESENTATION_ITEM('')
SURFACE()
) ;
#69=(
BOUNDED_SURFACE()
B_SPLINE_SURFACE(3,2,((#136125,#136126,#136127),(#136128,#136129,#136130),
(#136131,#136132,#136133),(#136134,#136135,#136136),(#136137,#136138,#136139),
(#136140,#136141,#136142),(#136143,#136144,#136145),(#136146,#136147,#136148),
(#136149,#136150,#136151),(#136152,#136153,#136154),(#136155,#136156,#136157),
(#136158,#136159,#136160),(#136161,#136162,#136163),(#136164,#136165,#136166),
(#136167,#136168,#136169),(#136170,#136171,#136172)),.UNSPECIFIED.,.F.,
 .F.,.F.)
B_SPLINE_SURFACE_WITH_KNOTS((4,2,2,2,2,2,2,4),(3,3),(7.77840519858991E-15,
3.8844760147831E-5,5.82671402178573E-5,6.79783302528705E-5,7.28339252703771E-5,
7.52617227791304E-5,7.6475621533507E-5,7.76895202878836E-5),(-0.00120945525754052,
1.01080070868977),.UNSPECIFIED.)
GEOMETRIC_REPRESENTATION_ITEM()
RATIONAL_B_SPLINE_SURFACE(((1.00005744302265,0.975995723233522,1.00051789333957),
(1.00004519813151,0.981112615457372,1.0004074961621),(1.00003362760161,
0.985947705765589,1.00030317887352),(1.00001854219783,0.992251590743248,
1.00016717227456),(1.00001393966879,0.994174894491119,1.0001256769106),
(1.00000788875349,0.996703449551654,1.00007112322264),(1.00000601414708,
0.997486809637525,1.00005422219392),(1.00000351698944,0.9985303212827,1.00003170838373),
(1.00000273459082,0.998857269833632,1.0000246544542),(1.00000163903614,
0.999315079965995,1.00001477718022),(1.00000129000885,0.999460931405222,
1.00001163042892),(1.0000009745592,0.999592751431241,1.000008786406),(1.00000093560708,
0.999609028734061,1.00000843522246),(1.00000065019919,0.999728294915418,
1.00000586204929),(1.00000066918571,0.999720360831427,1.00000603322751),
(1.,1.,1.)))
REPRESENTATION_ITEM('')
SURFACE()
) ;
#70=(
BOUNDED_SURFACE()
B_SPLINE_SURFACE(3,2,((#136214,#136215,#136216),(#136217,#136218,#136219),
(#136220,#136221,#136222),(#136223,#136224,#136225)),.UNSPECIFIED.,.F.,
 .F.,.F.)
B_SPLINE_SURFACE_WITH_KNOTS((4,4),(3,3),(3.14159265358979,4.71238898038469),
(0.,1.),.UNSPECIFIED.)
GEOMETRIC_REPRESENTATION_ITEM()
RATIONAL_B_SPLINE_SURFACE(((1.,0.75750200074082,1.),(1.,0.758151925542941,
1.),(1.,0.735025202593057,1.),(1.,0.707106781186548,1.)))
REPRESENTATION_ITEM('')
SURFACE()
) ;
#71=(
BOUNDED_SURFACE()
B_SPLINE_SURFACE(3,2,((#136227,#136228,#136229),(#136230,#136231,#136232),
(#136233,#136234,#136235),(#136236,#136237,#136238)),.UNSPECIFIED.,.F.,
 .F.,.F.)
B_SPLINE_SURFACE_WITH_KNOTS((4,4),(3,3),(4.71238898038469,6.28318530717959),
(0.,1.),.UNSPECIFIED.)
GEOMETRIC_REPRESENTATION_ITEM()
RATIONAL_B_SPLINE_SURFACE(((1.,0.707106781186548,1.),(1.,0.735025202593054,
1.),(1.,0.758151925542943,1.),(1.,0.75750200074082,1.)))
REPRESENTATION_ITEM('')
SURFACE()
) ;
#72=(
BOUNDED_SURFACE()
B_SPLINE_SURFACE(3,2,((#137643,#137644,#137645),(#137646,#137647,#137648),
(#137649,#137650,#137651),(#137652,#137653,#137654),(#137655,#137656,#137657),
(#137658,#137659,#137660)),.UNSPECIFIED.,.F.,.F.,.F.)
B_SPLINE_SURFACE_WITH_KNOTS((4,2,4),(3,3),(3.14159265358979,3.92699081698724,
4.71238898038469),(0.,1.),.UNSPECIFIED.)
GEOMETRIC_REPRESENTATION_ITEM()
RATIONAL_B_SPLINE_SURFACE(((1.,0.934721701546417,1.),(1.,0.934869636336908,
1.),(1.,0.913780519322379,1.),(1.,0.834646315042289,1.),(1.,0.776518516961048,
1.),(1.,0.707106781186548,1.)))
REPRESENTATION_ITEM('')
SURFACE()
) ;
#73=(
BOUNDED_SURFACE()
B_SPLINE_SURFACE(3,2,((#137671,#137672,#137673),(#137674,#137675,#137676),
(#137677,#137678,#137679),(#137680,#137681,#137682)),.UNSPECIFIED.,.F.,
 .F.,.F.)
B_SPLINE_SURFACE_WITH_KNOTS((4,4),(3,3),(1.5707963267949,2.41495031290807),
(0.,1.),.UNSPECIFIED.)
GEOMETRIC_REPRESENTATION_ITEM()
RATIONAL_B_SPLINE_SURFACE(((1.,0.707106781186547,1.),(1.,0.730803471035896,
1.),(1.,0.752906082887246,1.),(1.,0.767292203978619,1.)))
REPRESENTATION_ITEM('')
SURFACE()
) ;
#74=(
BOUNDED_SURFACE()
B_SPLINE_SURFACE(3,2,((#137699,#137700,#137701),(#137702,#137703,#137704),
(#137705,#137706,#137707),(#137708,#137709,#137710),(#137711,#137712,#137713),
(#137714,#137715,#137716)),.UNSPECIFIED.,.F.,.F.,.F.)
B_SPLINE_SURFACE_WITH_KNOTS((4,2,4),(3,3),(1.56955149927807,2.35619449019234,
3.14283748110662),(-0.00124482751682279,1.),.UNSPECIFIED.)
GEOMETRIC_REPRESENTATION_ITEM()
RATIONAL_B_SPLINE_SURFACE(((1.00073060381455,0.706544157856447,1.),(1.00062673753067,
0.748263304672953,1.),(1.00053422463655,0.78542222543767,1.),(1.00040682904416,
0.836592203069634,1.),(1.00037181710675,0.850655170404833,1.),(1.00037229282025,
0.850464094333147,1.)))
REPRESENTATION_ITEM('')
SURFACE()
) ;
#75=(
BOUNDED_SURFACE()
B_SPLINE_SURFACE(3,2,((#137719,#137720,#137721),(#137722,#137723,#137724),
(#137725,#137726,#137727),(#137728,#137729,#137730),(#137731,#137732,#137733),
(#137734,#137735,#137736)),.UNSPECIFIED.,.F.,.F.,.F.)
B_SPLINE_SURFACE_WITH_KNOTS((4,2,4),(3,3),(4.71238898038469,5.49778714378214,
6.28318530717959),(0.,1.),.UNSPECIFIED.)
GEOMETRIC_REPRESENTATION_ITEM()
RATIONAL_B_SPLINE_SURFACE(((1.,0.707106781186548,1.),(1.,0.776518516961086,
1.),(1.,0.83464631504224,1.),(1.,0.913780519322428,1.),(1.,0.934869636336872,
1.),(1.,0.934721701546417,1.)))
REPRESENTATION_ITEM('')
SURFACE()
) ;
#76=(
BOUNDED_SURFACE()
B_SPLINE_SURFACE(3,2,((#137744,#137745,#137746),(#137747,#137748,#137749),
(#137750,#137751,#137752),(#137753,#137754,#137755)),.UNSPECIFIED.,.F.,
 .F.,.F.)
B_SPLINE_SURFACE_WITH_KNOTS((4,4),(3,3),(0.726642340681723,1.5707963267949),
(0.,1.),.UNSPECIFIED.)
GEOMETRIC_REPRESENTATION_ITEM()
RATIONAL_B_SPLINE_SURFACE(((1.,0.767292203978619,1.),(1.,0.752906082887264,
1.),(1.,0.730803471035884,1.),(1.,0.707106781186547,1.)))
REPRESENTATION_ITEM('')
SURFACE()
) ;
#77=(
BOUNDED_SURFACE()
B_SPLINE_SURFACE(3,2,((#137771,#137772,#137773),(#137774,#137775,#137776),
(#137777,#137778,#137779),(#137780,#137781,#137782),(#137783,#137784,#137785),
(#137786,#137787,#137788)),.UNSPECIFIED.,.F.,.F.,.F.)
B_SPLINE_SURFACE_WITH_KNOTS((4,2,4),(3,3),(-0.00124482751685595,0.785398163397448,
1.57204115431175),(-0.00124482751685595,1.),.UNSPECIFIED.)
GEOMETRIC_REPRESENTATION_ITEM()
RATIONAL_B_SPLINE_SURFACE(((1.00037229282026,0.850464094333142,1.),(1.00037181710676,
0.850655170404827,1.),(1.00040682904418,0.836592203069629,1.),(1.00053422463656,
0.785422225437663,1.),(1.00062673753069,0.748263304672945,1.),(1.00073060381456,
0.706544157856431,1.)))
REPRESENTATION_ITEM('')
SURFACE()
) ;
#78=(
BOUNDED_SURFACE()
B_SPLINE_SURFACE(3,2,((#137800,#137801,#137802),(#137803,#137804,#137805),
(#137806,#137807,#137808),(#137809,#137810,#137811)),.UNSPECIFIED.,.F.,
 .F.,.F.)
B_SPLINE_SURFACE_WITH_KNOTS((4,4),(3,3),(1.10714871779409,1.5707963267949),
(0.,1.),.UNSPECIFIED.)
GEOMETRIC_REPRESENTATION_ITEM()
RATIONAL_B_SPLINE_SURFACE(((1.,0.743704326447947,1.),(1.,0.732676928202348,
1.),(1.,0.720087778783133,1.),(1.,0.707106781186548,1.)))
REPRESENTATION_ITEM('')
SURFACE()
) ;
#79=(
BOUNDED_SURFACE()
B_SPLINE_SURFACE(3,2,((#137819,#137820,#137821),(#137822,#137823,#137824),
(#137825,#137826,#137827),(#137828,#137829,#137830)),.UNSPECIFIED.,.F.,
 .F.,.F.)
B_SPLINE_SURFACE_WITH_KNOTS((4,4),(3,3),(1.5707963267949,2.0344439357957),
(0.,1.),.UNSPECIFIED.)
GEOMETRIC_REPRESENTATION_ITEM()
RATIONAL_B_SPLINE_SURFACE(((1.,0.707106781186548,1.),(1.,0.720087778783145,
1.),(1.,0.732676928202328,1.),(1.,0.743704326447957,1.)))
REPRESENTATION_ITEM('')
SURFACE()
) ;
#80=(
BOUNDED_SURFACE()
B_SPLINE_SURFACE(3,2,((#138105,#138106,#138107),(#138108,#138109,#138110),
(#138111,#138112,#138113),(#138114,#138115,#138116)),.UNSPECIFIED.,.F.,
 .F.,.F.)
B_SPLINE_SURFACE_WITH_KNOTS((4,4),(3,3),(0.000111059871785624,0.000241296646650869),
(0.,1.00030059112236),.UNSPECIFIED.)
GEOMETRIC_REPRESENTATION_ITEM()
RATIONAL_B_SPLINE_SURFACE(((1.,0.839985548969886,1.00009619784686),(1.,
0.79732203291707,1.0001218463952),(1.,0.73468600944038,1.0001595020604),
(1.,0.707018740085173,1.00017613513149)))
REPRESENTATION_ITEM('')
SURFACE()
) ;
#81=(
BOUNDED_SURFACE()
B_SPLINE_SURFACE(3,2,((#138118,#138119,#138120),(#138121,#138122,#138123),
(#138124,#138125,#138126),(#138127,#138128,#138129)),.UNSPECIFIED.,.F.,
 .F.,.F.)
B_SPLINE_SURFACE_WITH_KNOTS((4,4),(3,3),(3.14159265358979,3.68974201455418),
(0.,1.),.UNSPECIFIED.)
GEOMETRIC_REPRESENTATION_ITEM()
RATIONAL_B_SPLINE_SURFACE(((1.,0.860789971413512,1.),(1.,0.860809546755052,
1.),(1.,0.853709425573776,1.),(1.,0.840033633436873,1.)))
REPRESENTATION_ITEM('')
SURFACE()
) ;
#82=(
BOUNDED_SURFACE()
B_SPLINE_SURFACE(3,2,((#138135,#138136,#138137),(#138138,#138139,#138140),
(#138141,#138142,#138143),(#138144,#138145,#138146)),.UNSPECIFIED.,.F.,
 .F.,.F.)
B_SPLINE_SURFACE_WITH_KNOTS((4,4),(3,3),(2.59344329260967,3.14159265358979),
(0.,1.),.UNSPECIFIED.)
GEOMETRIC_REPRESENTATION_ITEM()
RATIONAL_B_SPLINE_SURFACE(((1.,0.840033633435699,1.),(1.,0.853709425573365,
1.),(1.,0.860809546755054,1.),(1.,0.860789971413512,1.)))
REPRESENTATION_ITEM('')
SURFACE()
) ;
#83=(
BOUNDED_SURFACE()
B_SPLINE_SURFACE(3,2,((#138148,#138149,#138150),(#138151,#138152,#138153),
(#138154,#138155,#138156),(#138157,#138158,#138159)),.UNSPECIFIED.,.F.,
 .F.,.F.)
B_SPLINE_SURFACE_WITH_KNOTS((4,4),(3,3),(0.000111059871788868,0.000241296646650869),
(-0.000300086750004719,1.),.UNSPECIFIED.)
GEOMETRIC_REPRESENTATION_ITEM()
RATIONAL_B_SPLINE_SURFACE(((1.00009603638471,0.839985629649231,1.),(1.00012164188355,
0.797322135108548,1.),(1.00015923434603,0.734686143216427,1.),(1.00017583949954,
0.707018887812415,1.)))
REPRESENTATION_ITEM('')
SURFACE()
) ;
#84=(
BOUNDED_SURFACE()
B_SPLINE_SURFACE(3,2,((#138244,#138245,#138246),(#138247,#138248,#138249),
(#138250,#138251,#138252),(#138253,#138254,#138255),(#138256,#138257,#138258),
(#138259,#138260,#138261),(#138262,#138263,#138264),(#138265,#138266,#138267),
(#138268,#138269,#138270),(#138271,#138272,#138273)),.UNSPECIFIED.,.F.,
 .F.,.F.)
B_SPLINE_SURFACE_WITH_KNOTS((4,2,2,2,4),(3,3),(0.00112100122803336,0.00145633576709043,
0.0015908372445872,0.00165808798333558,0.00178849406635727),(-0.000893324189260702,
1.00101552458171),.UNSPECIFIED.)
GEOMETRIC_REPRESENTATION_ITEM()
RATIONAL_B_SPLINE_SURFACE(((1.00061830890916,0.653576280075716,1.0007029749849),
(1.00045188087569,0.746821933830268,1.00051375768173),(1.00032243686651,
0.819346321742879,1.00036658868733),(1.00017052538065,0.904458700444932,
1.00019387570697),(1.00013074576008,0.926746272131252,1.00014864899624),
(1.00007983643892,0.955269549338603,1.00009076857637),(1.00006394848111,
0.964171192776776,1.00007270505386),(1.00002748579919,0.984600362923306,
1.00003124947578),(1.00001632684003,0.990852461324469,1.00001856250162),
(1.00006581963707,0.963122828765763,1.00007483243035)))
REPRESENTATION_ITEM('')
SURFACE()
) ;
#85=(
BOUNDED_SURFACE()
B_SPLINE_SURFACE(3,2,((#138314,#138315,#138316),(#138317,#138318,#138319),
(#138320,#138321,#138322),(#138323,#138324,#138325),(#138326,#138327,#138328),
(#138329,#138330,#138331),(#138332,#138333,#138334),(#138335,#138336,#138337),
(#138338,#138339,#138340),(#138341,#138342,#138343)),.UNSPECIFIED.,.F.,
 .F.,.F.)
B_SPLINE_SURFACE_WITH_KNOTS((4,2,2,2,4),(3,3),(0.00112100122803338,0.00145633576709043,
0.00159083724458721,0.00165808798333559,0.00178849406635728),(-0.00113559264167306,
1.),.UNSPECIFIED.)
GEOMETRIC_REPRESENTATION_ITEM()
RATIONAL_B_SPLINE_SURFACE(((1.0007861837978,0.653844270846518,1.),(1.00057456947124,
0.747017790468252,1.),(1.00040998057203,0.81948607406265,1.),(1.00021682413014,
0.904532610471983,1.),(1.00016624408395,0.926802940661303,1.),(1.00010151255112,
0.955304152477097,1.),(1.00008131090948,0.964198909671178,1.),(1.00003494837236,
0.984612275966134,1.),(1.00002075968324,0.990859537791216,1.),(1.00008369009644,
0.963151356666673,1.)))
REPRESENTATION_ITEM('')
SURFACE()
) ;
#86=(
BOUNDED_SURFACE()
B_SPLINE_SURFACE(3,2,((#138380,#138381,#138382),(#138383,#138384,#138385),
(#138386,#138387,#138388),(#138389,#138390,#138391),(#138392,#138393,#138394),
(#138395,#138396,#138397),(#138398,#138399,#138400),(#138401,#138402,#138403),
(#138404,#138405,#138406),(#138407,#138408,#138409),(#138410,#138411,#138412),
(#138413,#138414,#138415),(#138416,#138417,#138418),(#138419,#138420,#138421),
(#138422,#138423,#138424),(#138425,#138426,#138427)),.UNSPECIFIED.,.F.,
 .F.,.F.)
B_SPLINE_SURFACE_WITH_KNOTS((4,2,2,2,2,2,2,4),(3,3),(5.6285407107684E-15,
3.85995771599558E-5,5.78993657371195E-5,6.75492600257013E-5,7.23742071699922E-5,
7.47866807421377E-5,7.59929175282104E-5,7.71991543142831E-5),(0.,1.00107899067822),
 .UNSPECIFIED.)
GEOMETRIC_REPRESENTATION_ITEM()
RATIONAL_B_SPLINE_SURFACE(((1.,0.976255617118807,1.00005123993558),(1.,
0.981339981891218,1.00004026797119),(1.,0.986086237829171,1.00003002563936),
(1.,0.992269463037035,1.00001668235464),(1.,0.994174411180035,1.00001257151206),
(1.,0.996706913506707,1.00000710641926),(1.,0.997492596832092,1.00000541092929),
(1.,0.998537621803386,1.00000315578488),(1.,0.998865045809506,1.00000244920998),
(1.,0.999323526852926,1.00000145981644),(1.,0.999468419970867,1.00000114713979),
(1.,0.99959844684718,1.00000086654422),(1.,0.999614491362716,1.00000083192045),
(1.,0.999732489024761,1.0000005772837),(1.,0.999724369239699,1.00000059480604),
(1.,1.,1.)))
REPRESENTATION_ITEM('')
SURFACE()
) ;
#87=(
BOUNDED_SURFACE()
B_SPLINE_SURFACE(3,2,((#138429,#138430,#138431),(#138432,#138433,#138434),
(#138435,#138436,#138437),(#138438,#138439,#138440),(#138441,#138442,#138443),
(#138444,#138445,#138446),(#138447,#138448,#138449),(#138450,#138451,#138452),
(#138453,#138454,#138455),(#138456,#138457,#138458)),.UNSPECIFIED.,.F.,
 .F.,.F.)
B_SPLINE_SURFACE_WITH_KNOTS((4,2,2,2,4),(3,3),(-0.00011070792851133,0.000553539642556655,
0.000830309463834981,0.000968694374474145,0.00121778721363011),(0.,1.00563383762715),
 .UNSPECIFIED.)
GEOMETRIC_REPRESENTATION_ITEM()
RATIONAL_B_SPLINE_SURFACE(((1.,0.710139408519237,1.00326605501383),(1.,
0.691948125896667,1.00347102847888),(1.,0.728232377173921,1.00306218931864),
(1.,0.818030374423583,1.00205037464714),(1.,0.8491107594692,1.00170017096167),
(1.,0.897979778369929,1.0011495307267),(1.,0.914666724297522,1.000961507639),
(1.,0.961090538823349,1.00043841917286),(1.,0.990973799041317,1.00010170430118),
(1.,0.992463455161609,1.00008491933978)))
REPRESENTATION_ITEM('')
SURFACE()
) ;
#88=(
BOUNDED_SURFACE()
B_SPLINE_SURFACE(3,2,((#138460,#138461,#138462),(#138463,#138464,#138465),
(#138466,#138467,#138468),(#138469,#138470,#138471),(#138472,#138473,#138474),
(#138475,#138476,#138477),(#138478,#138479,#138480),(#138481,#138482,#138483),
(#138484,#138485,#138486),(#138487,#138488,#138489)),.UNSPECIFIED.,.F.,
 .F.,.F.)
B_SPLINE_SURFACE_WITH_KNOTS((4,2,2,2,4),(3,3),(-0.000137915648493747,0.000139027965246066,
0.000278055930499748,0.000556111861007113,0.00125013859505175),(-0.000741678186154432,
1.00283457365368),.UNSPECIFIED.)
GEOMETRIC_REPRESENTATION_ITEM()
RATIONAL_B_SPLINE_SURFACE(((1.00001340810332,0.990935328832712,1.00005135076275),
(1.00000300543757,0.997968146378609,1.00001151031641),(1.00005311279901,
0.964092605306906,1.0002034130165),(1.00012590576293,0.914880254704336,
1.00048219772843),(1.00015093966353,0.897955856706345,1.00057807332394),
(1.00022375355373,0.848729358697742,1.00085693817998),(1.00026920263046,
0.818003093715361,1.00103100043929),(1.00040494517458,0.726233102311804,
1.00155087137217),(1.00045889592424,0.689759203410913,1.00175749359754),
(1.00042429005347,0.713154819594415,1.00162495897893)))
REPRESENTATION_ITEM('')
SURFACE()
) ;
#89=(
BOUNDED_SURFACE()
B_SPLINE_SURFACE(3,2,((#138491,#138492,#138493),(#138494,#138495,#138496),
(#138497,#138498,#138499),(#138500,#138501,#138502),(#138503,#138504,#138505),
(#138506,#138507,#138508),(#138509,#138510,#138511),(#138512,#138513,#138514),
(#138515,#138516,#138517),(#138518,#138519,#138520),(#138521,#138522,#138523),
(#138524,#138525,#138526),(#138527,#138528,#138529),(#138530,#138531,#138532),
(#138533,#138534,#138535),(#138536,#138537,#138538)),.UNSPECIFIED.,.F.,
 .F.,.F.)
B_SPLINE_SURFACE_WITH_KNOTS((4,2,2,2,2,2,2,4),(3,3),(7.7799501866857E-15,
3.88447601478329E-5,5.82671402178594E-5,6.79783302528727E-5,7.28339252703793E-5,
7.52617227791326E-5,7.64756215335093E-5,7.76895202878859E-5),(-0.00120945525743048,
1.010800708689),.UNSPECIFIED.)
GEOMETRIC_REPRESENTATION_ITEM()
RATIONAL_B_SPLINE_SURFACE(((1.00005744302265,0.975995723233542,1.00051789333953),
(1.00004519813151,0.98111261545739,1.00040749616208),(1.00003362760161,
0.985947705765599,1.00030317887349),(1.00001854219782,0.992251590743256,
1.00016717227455),(1.00001393966879,0.994174894491125,1.0001256769106),
(1.00000788875349,0.996703449551656,1.00007112322263),(1.00000601414708,
0.997486809637528,1.00005422219392),(1.00000351698944,0.998530321282699,
1.00003170838373),(1.00000273459082,0.998857269833612,1.0000246544542),
(1.00000163903614,0.999315079966002,1.00001477718022),(1.00000129000885,
0.999460931405225,1.00001163042892),(1.0000009745592,0.99959275143124,1.000008786406),
(1.00000093560708,0.99960902873406,1.00000843522246),(1.00000065019919,
0.999728294915416,1.00000586204929),(1.00000066918571,0.99972036083143,
1.00000603322751),(1.,1.,1.)))
REPRESENTATION_ITEM('')
SURFACE()
) ;
#90=(
BOUNDED_SURFACE()
B_SPLINE_SURFACE(3,2,((#139011,#139012,#139013),(#139014,#139015,#139016),
(#139017,#139018,#139019),(#139020,#139021,#139022),(#139023,#139024,#139025),
(#139026,#139027,#139028)),.UNSPECIFIED.,.F.,.F.,.F.)
B_SPLINE_SURFACE_WITH_KNOTS((4,2,4),(3,3),(3.14159265358979,3.92699081698724,
4.71238898038469),(0.,1.),.UNSPECIFIED.)
GEOMETRIC_REPRESENTATION_ITEM()
RATIONAL_B_SPLINE_SURFACE(((1.,0.934721701546417,1.),(1.,0.934869636336949,
1.),(1.,0.913780519322321,1.),(1.,0.834646315042351,1.),(1.,0.776518516961002,
1.),(1.,0.707106781186548,1.)))
REPRESENTATION_ITEM('')
SURFACE()
) ;
#91=(
BOUNDED_SURFACE()
B_SPLINE_SURFACE(3,2,((#139039,#139040,#139041),(#139042,#139043,#139044),
(#139045,#139046,#139047),(#139048,#139049,#139050)),.UNSPECIFIED.,.F.,
 .F.,.F.)
B_SPLINE_SURFACE_WITH_KNOTS((4,4),(3,3),(1.5707963267949,2.41495031290807),
(0.,1.),.UNSPECIFIED.)
GEOMETRIC_REPRESENTATION_ITEM()
RATIONAL_B_SPLINE_SURFACE(((1.,0.707106781186553,1.),(1.,0.730803471035898,
1.),(1.,0.752906082887247,1.),(1.,0.76729220397862,1.)))
REPRESENTATION_ITEM('')
SURFACE()
) ;
#92=(
BOUNDED_SURFACE()
B_SPLINE_SURFACE(3,2,((#139067,#139068,#139069),(#139070,#139071,#139072),
(#139073,#139074,#139075),(#139076,#139077,#139078),(#139079,#139080,#139081),
(#139082,#139083,#139084)),.UNSPECIFIED.,.F.,.F.,.F.)
B_SPLINE_SURFACE_WITH_KNOTS((4,2,4),(3,3),(1.56955149927814,2.35619449019234,
3.14283748110655),(-0.00124482751675719,1.),.UNSPECIFIED.)
GEOMETRIC_REPRESENTATION_ITEM()
RATIONAL_B_SPLINE_SURFACE(((1.00073060381451,0.706544157856477,1.),(1.00062673753064,
0.748263304672955,1.),(1.00053422463652,0.785422225437717,1.),(1.00040682904414,
0.83659220306961,1.),(1.00037181710673,0.850655170404864,1.),(1.00037229282023,
0.850464094333156,1.)))
REPRESENTATION_ITEM('')
SURFACE()
) ;
#93=(
BOUNDED_SURFACE()
B_SPLINE_SURFACE(3,2,((#139087,#139088,#139089),(#139090,#139091,#139092),
(#139093,#139094,#139095),(#139096,#139097,#139098),(#139099,#139100,#139101),
(#139102,#139103,#139104)),.UNSPECIFIED.,.F.,.F.,.F.)
B_SPLINE_SURFACE_WITH_KNOTS((4,2,4),(3,3),(4.71238898038469,5.49778714378214,
6.28318530717959),(0.,1.),.UNSPECIFIED.)
GEOMETRIC_REPRESENTATION_ITEM()
RATIONAL_B_SPLINE_SURFACE(((1.,0.707106781186548,1.),(1.,0.776518516960999,
1.),(1.,0.834646315042352,1.),(1.,0.913780519322316,1.),(1.,0.934869636336956,
1.),(1.,0.934721701546417,1.)))
REPRESENTATION_ITEM('')
SURFACE()
) ;
#94=(
BOUNDED_SURFACE()
B_SPLINE_SURFACE(3,2,((#139112,#139113,#139114),(#139115,#139116,#139117),
(#139118,#139119,#139120),(#139121,#139122,#139123)),.UNSPECIFIED.,.F.,
 .F.,.F.)
B_SPLINE_SURFACE_WITH_KNOTS((4,4),(3,3),(0.726642340681723,1.5707963267949),
(0.,1.),.UNSPECIFIED.)
GEOMETRIC_REPRESENTATION_ITEM()
RATIONAL_B_SPLINE_SURFACE(((1.,0.767292203978619,1.),(1.,0.752906082887246,
1.),(1.,0.730803471035896,1.),(1.,0.707106781186547,1.)))
REPRESENTATION_ITEM('')
SURFACE()
) ;
#95=(
BOUNDED_SURFACE()
B_SPLINE_SURFACE(3,2,((#139139,#139140,#139141),(#139142,#139143,#139144),
(#139145,#139146,#139147),(#139148,#139149,#139150),(#139151,#139152,#139153),
(#139154,#139155,#139156)),.UNSPECIFIED.,.F.,.F.,.F.)
B_SPLINE_SURFACE_WITH_KNOTS((4,2,4),(3,3),(-0.00124482751681696,0.785398163397448,
1.57204115431171),(-0.00124482751681696,1.),.UNSPECIFIED.)
GEOMETRIC_REPRESENTATION_ITEM()
RATIONAL_B_SPLINE_SURFACE(((1.00037229282025,0.850464094333147,1.),(1.00037181710675,
0.850655170404832,1.),(1.00040682904416,0.836592203069633,1.),(1.00053422463654,
0.785422225437673,1.),(1.00062673753067,0.748263304672954,1.),(1.00073060381454,
0.706544157856449,1.)))
REPRESENTATION_ITEM('')
SURFACE()
) ;
#96=(
BOUNDED_SURFACE()
B_SPLINE_SURFACE(3,2,((#139168,#139169,#139170),(#139171,#139172,#139173),
(#139174,#139175,#139176),(#139177,#139178,#139179)),.UNSPECIFIED.,.F.,
 .F.,.F.)
B_SPLINE_SURFACE_WITH_KNOTS((4,4),(3,3),(1.10714871779409,1.5707963267949),
(0.,1.),.UNSPECIFIED.)
GEOMETRIC_REPRESENTATION_ITEM()
RATIONAL_B_SPLINE_SURFACE(((1.,0.743704326447947,1.),(1.,0.732676928202349,
1.),(1.,0.720087778783133,1.),(1.,0.707106781186553,1.)))
REPRESENTATION_ITEM('')
SURFACE()
) ;
#97=(
BOUNDED_SURFACE()
B_SPLINE_SURFACE(3,2,((#139187,#139188,#139189),(#139190,#139191,#139192),
(#139193,#139194,#139195),(#139196,#139197,#139198)),.UNSPECIFIED.,.F.,
 .F.,.F.)
B_SPLINE_SURFACE_WITH_KNOTS((4,4),(3,3),(1.5707963267949,2.0344439357957),
(0.,1.),.UNSPECIFIED.)
GEOMETRIC_REPRESENTATION_ITEM()
RATIONAL_B_SPLINE_SURFACE(((1.,0.707106781186548,1.),(1.,0.720087778783133,
1.),(1.,0.73267692820235,1.),(1.,0.743704326447947,1.)))
REPRESENTATION_ITEM('')
SURFACE()
) ;
#98=(
BOUNDED_SURFACE()
B_SPLINE_SURFACE(3,2,((#139448,#139449,#139450),(#139451,#139452,#139453),
(#139454,#139455,#139456),(#139457,#139458,#139459)),.UNSPECIFIED.,.F.,
 .F.,.F.)
B_SPLINE_SURFACE_WITH_KNOTS((4,4),(3,3),(0.000111059871785622,0.000241296646650869),
(0.,1.00030059112227),.UNSPECIFIED.)
GEOMETRIC_REPRESENTATION_ITEM()
RATIONAL_B_SPLINE_SURFACE(((1.,0.839985548969898,1.00009619784683),(1.,
0.797322032917094,1.00012184639517),(1.,0.734686009440392,1.00015950206035),
(1.,0.707018740085205,1.00017613513144)))
REPRESENTATION_ITEM('')
SURFACE()
) ;
#99=(
BOUNDED_SURFACE()
B_SPLINE_SURFACE(3,2,((#139461,#139462,#139463),(#139464,#139465,#139466),
(#139467,#139468,#139469),(#139470,#139471,#139472)),.UNSPECIFIED.,.F.,
 .F.,.F.)
B_SPLINE_SURFACE_WITH_KNOTS((4,4),(3,3),(3.14159265358979,3.68974201455418),
(0.,1.),.UNSPECIFIED.)
GEOMETRIC_REPRESENTATION_ITEM()
RATIONAL_B_SPLINE_SURFACE(((1.,0.860789971413512,1.),(1.,0.860809546755051,
1.),(1.,0.853709425573778,1.),(1.,0.840033633436873,1.)))
REPRESENTATION_ITEM('')
SURFACE()
) ;
#100=(
BOUNDED_SURFACE()
B_SPLINE_SURFACE(3,2,((#139475,#139476,#139477),(#139478,#139479,#139480),
(#139481,#139482,#139483),(#139484,#139485,#139486)),.UNSPECIFIED.,.F.,
 .F.,.F.)
B_SPLINE_SURFACE_WITH_KNOTS((4,4),(3,3),(2.59344329260967,3.14159265358979),
(0.,1.),.UNSPECIFIED.)
GEOMETRIC_REPRESENTATION_ITEM()
RATIONAL_B_SPLINE_SURFACE(((1.,0.840033633435699,1.),(1.,0.853709425573363,
1.),(1.,0.860809546755055,1.),(1.,0.860789971413512,1.)))
REPRESENTATION_ITEM('')
SURFACE()
) ;
#101=(
BOUNDED_SURFACE()
B_SPLINE_SURFACE(3,2,((#139488,#139489,#139490),(#139491,#139492,#139493),
(#139494,#139495,#139496),(#139497,#139498,#139499)),.UNSPECIFIED.,.F.,
 .F.,.F.)
B_SPLINE_SURFACE_WITH_KNOTS((4,4),(3,3),(0.000111059871788868,0.000241296646650869),
(-0.000300086750003606,1.),.UNSPECIFIED.)
GEOMETRIC_REPRESENTATION_ITEM()
RATIONAL_B_SPLINE_SURFACE(((1.0000960363847,0.839985629649235,1.),(1.00012164188355,
0.797322135108538,1.),(1.00015923434603,0.734686143216438,1.),(1.00017583949954,
0.707018887812415,1.)))
REPRESENTATION_ITEM('')
SURFACE()
) ;
#102=(
BOUNDED_SURFACE()
B_SPLINE_SURFACE(3,2,((#139583,#139584,#139585),(#139586,#139587,#139588),
(#139589,#139590,#139591),(#139592,#139593,#139594),(#139595,#139596,#139597),
(#139598,#139599,#139600),(#139601,#139602,#139603),(#139604,#139605,#139606),
(#139607,#139608,#139609),(#139610,#139611,#139612)),.UNSPECIFIED.,.F.,
 .F.,.F.)
B_SPLINE_SURFACE_WITH_KNOTS((4,2,2,2,4),(3,3),(0.00112100122803331,0.00145633576709043,
0.0015908372445872,0.00165808798333558,0.00178849406635728),(-0.000893324189052896,
1.00101552458165),.UNSPECIFIED.)
GEOMETRIC_REPRESENTATION_ITEM()
RATIONAL_B_SPLINE_SURFACE(((1.00061830890902,0.653576280075841,1.00070297498485),
(1.00045188087558,0.746821933830185,1.0005137576817),(1.00032243686644,
0.819346321743005,1.0003665886873),(1.00017052538062,0.904458700444923,
1.00019387570696),(1.00013074576005,0.926746272131313,1.00014864899624),
(1.0000798364389,0.955269549338596,1.00009076857636),(1.0000639484811,0.964171192776782,
1.00007270505386),(1.00002748579918,0.984600362923314,1.00003124947578),
(1.00001632684004,0.990852461324472,1.00001856250162),(1.00006581963706,
0.963122828765752,1.00007483243035)))
REPRESENTATION_ITEM('')
SURFACE()
) ;
#103=(
BOUNDED_SURFACE()
B_SPLINE_SURFACE(3,2,((#139651,#139652,#139653),(#139654,#139655,#139656),
(#139657,#139658,#139659),(#139660,#139661,#139662),(#139663,#139664,#139665),
(#139666,#139667,#139668),(#139669,#139670,#139671),(#139672,#139673,#139674),
(#139675,#139676,#139677),(#139678,#139679,#139680)),.UNSPECIFIED.,.F.,
 .F.,.F.)
B_SPLINE_SURFACE_WITH_KNOTS((4,2,2,2,4),(3,3),(0.00112100122803326,0.00145633576709043,
0.00159083724458721,0.00165808798333559,0.00178849406635729),(-0.00113559264180098,
1.),.UNSPECIFIED.)
GEOMETRIC_REPRESENTATION_ITEM()
RATIONAL_B_SPLINE_SURFACE(((1.00078618379789,0.653844270846382,1.),(1.0005745694713,
0.747017790468173,1.),(1.00040998057207,0.819486074062609,1.),(1.00021682413016,
0.904532610471971,1.),(1.00016624408397,0.926802940661278,1.),(1.00010151255113,
0.955304152477099,1.),(1.00008131090949,0.964198909671174,1.),(1.00003494837237,
0.984612275966134,1.),(1.00002075968325,0.990859537791216,1.),(1.00008369009645,
0.963151356666666,1.)))
REPRESENTATION_ITEM('')
SURFACE()
) ;
#104=(
BOUNDED_SURFACE()
B_SPLINE_SURFACE(3,2,((#139717,#139718,#139719),(#139720,#139721,#139722),
(#139723,#139724,#139725),(#139726,#139727,#139728),(#139729,#139730,#139731),
(#139732,#139733,#139734),(#139735,#139736,#139737),(#139738,#139739,#139740),
(#139741,#139742,#139743),(#139744,#139745,#139746),(#139747,#139748,#139749),
(#139750,#139751,#139752),(#139753,#139754,#139755),(#139756,#139757,#139758),
(#139759,#139760,#139761),(#139762,#139763,#139764)),.UNSPECIFIED.,.F.,
 .F.,.F.)
B_SPLINE_SURFACE_WITH_KNOTS((4,2,2,2,2,2,2,4),(3,3),(5.6278630844106E-15,
3.85995771599556E-5,5.78993657371195E-5,6.75492600257015E-5,7.23742071699924E-5,
7.47866807421379E-5,7.59929175282107E-5,7.71991543142834E-5),(0.,1.00107899067813),
 .UNSPECIFIED.)
GEOMETRIC_REPRESENTATION_ITEM()
RATIONAL_B_SPLINE_SURFACE(((1.,0.976255617118809,1.00005123993557),(1.,
0.981339981891254,1.00004026797119),(1.,0.986086237829182,1.00003002563936),
(1.,0.992269463037031,1.00001668235464),(1.,0.994174411180037,1.00001257151206),
(1.,0.996706913506705,1.00000710641926),(1.,0.997492596832093,1.00000541092929),
(1.,0.99853762180339,1.00000315578488),(1.,0.998865045809501,1.00000244920998),
(1.,0.999323526852926,1.00000145981644),(1.,0.999468419970872,1.00000114713979),
(1.,0.999598446847179,1.00000086654422),(1.,0.999614491362717,1.00000083192045),
(1.,0.999732489024762,1.0000005772837),(1.,0.999724369239697,1.00000059480604),
(1.,1.,1.)))
REPRESENTATION_ITEM('')
SURFACE()
) ;
#105=(
BOUNDED_SURFACE()
B_SPLINE_SURFACE(3,2,((#139766,#139767,#139768),(#139769,#139770,#139771),
(#139772,#139773,#139774),(#139775,#139776,#139777),(#139778,#139779,#139780),
(#139781,#139782,#139783),(#139784,#139785,#139786),(#139787,#139788,#139789),
(#139790,#139791,#139792),(#139793,#139794,#139795)),.UNSPECIFIED.,.F.,
 .F.,.F.)
B_SPLINE_SURFACE_WITH_KNOTS((4,2,2,2,4),(3,3),(-0.000110707928511331,0.000553539642556653,
0.00083030946383498,0.000968694374474144,0.00121778721363011),(0.,1.00563383762645),
 .UNSPECIFIED.)
GEOMETRIC_REPRESENTATION_ITEM()
RATIONAL_B_SPLINE_SURFACE(((1.,0.710139408519343,1.00326605501342),(1.,
0.691948125897072,1.00347102847844),(1.,0.728232377173963,1.00306218931826),
(1.,0.818030374423771,1.00205037464689),(1.,0.849110759469331,1.00170017096146),
(1.,0.897979778369987,1.00114953072656),(1.,0.914666724297546,1.00096150763888),
(1.,0.961090538823436,1.0004384191728),(1.,0.990973799041145,1.00010170430117),
(1.,0.992463455161931,1.00008491933976)))
REPRESENTATION_ITEM('')
SURFACE()
) ;
#106=(
BOUNDED_SURFACE()
B_SPLINE_SURFACE(3,2,((#139797,#139798,#139799),(#139800,#139801,#139802),
(#139803,#139804,#139805),(#139806,#139807,#139808),(#139809,#139810,#139811),
(#139812,#139813,#139814),(#139815,#139816,#139817),(#139818,#139819,#139820),
(#139821,#139822,#139823),(#139824,#139825,#139826)),.UNSPECIFIED.,.F.,
 .F.,.F.)
B_SPLINE_SURFACE_WITH_KNOTS((4,2,2,2,4),(3,3),(-0.000137915648493774,0.000139027965246066,
0.000278055930499748,0.000556111861007112,0.00125013859505186),(-0.000741678186100512,
1.00283457365347),.UNSPECIFIED.)
GEOMETRIC_REPRESENTATION_ITEM()
RATIONAL_B_SPLINE_SURFACE(((1.00001340810332,0.990935328832901,1.00005135076275),
(1.00000300543757,0.997968146378528,1.0000115103164),(1.00005311279901,
0.964092605306946,1.00020341301648),(1.00012590576293,0.914880254704346,
1.00048219772839),(1.00015093966352,0.897955856706357,1.00057807332389),
(1.00022375355372,0.848729358697813,1.00085693817992),(1.00026920263044,
0.818003093715353,1.00103100043921),(1.00040494517455,0.726233102312007,
1.00155087137205),(1.0004588959242,0.689759203410784,1.00175749359741),
(1.00042429005344,0.713154819594625,1.00162495897881)))
REPRESENTATION_ITEM('')
SURFACE()
) ;
#107=(
BOUNDED_SURFACE()
B_SPLINE_SURFACE(3,2,((#139828,#139829,#139830),(#139831,#139832,#139833),
(#139834,#139835,#139836),(#139837,#139838,#139839),(#139840,#139841,#139842),
(#139843,#139844,#139845),(#139846,#139847,#139848),(#139849,#139850,#139851),
(#139852,#139853,#139854),(#139855,#139856,#139857),(#139858,#139859,#139860),
(#139861,#139862,#139863),(#139864,#139865,#139866),(#139867,#139868,#139869),
(#139870,#139871,#139872),(#139873,#139874,#139875)),.UNSPECIFIED.,.F.,
 .F.,.F.)
B_SPLINE_SURFACE_WITH_KNOTS((4,2,2,2,2,2,2,4),(3,3),(7.7799501866857E-15,
3.88447601478329E-5,5.82671402178594E-5,6.79783302528727E-5,7.28339252703793E-5,
7.52617227791326E-5,7.64756215335093E-5,7.76895202878859E-5),(-0.00120945525752119,
1.01080070868862),.UNSPECIFIED.)
GEOMETRIC_REPRESENTATION_ITEM()
RATIONAL_B_SPLINE_SURFACE(((1.00005744302265,0.975995723233548,1.00051789333951),
(1.00004519813151,0.981112615457395,1.00040749616206),(1.00003362760161,
0.985947705765603,1.00030317887348),(1.00001854219783,0.992251590743258,
1.00016717227455),(1.00001393966879,0.994174894491126,1.00012567691059),
(1.00000788875349,0.996703449551657,1.00007112322263),(1.00000601414708,
0.997486809637528,1.00005422219392),(1.00000351698944,0.9985303212827,1.00003170838373),
(1.00000273459082,0.998857269833613,1.0000246544542),(1.00000163903614,
0.999315079966002,1.00001477718021),(1.00000129000885,0.999460931405225,
1.00001163042892),(1.0000009745592,0.99959275143124,1.00000878640599),(1.00000093560708,
0.99960902873406,1.00000843522246),(1.00000065019919,0.999728294915417,
1.00000586204929),(1.00000066918571,0.99972036083143,1.00000603322751),
(1.,1.,1.)))
REPRESENTATION_ITEM('')
SURFACE()
) ;
#108=(
BOUNDED_SURFACE()
B_SPLINE_SURFACE(3,2,((#139917,#139918,#139919),(#139920,#139921,#139922),
(#139923,#139924,#139925),(#139926,#139927,#139928)),.UNSPECIFIED.,.F.,
 .F.,.F.)
B_SPLINE_SURFACE_WITH_KNOTS((4,4),(3,3),(3.14159265358979,4.71238898038469),
(0.,1.),.UNSPECIFIED.)
GEOMETRIC_REPRESENTATION_ITEM()
RATIONAL_B_SPLINE_SURFACE(((1.,0.75750200074082,1.),(1.,0.758151925542946,
1.),(1.,0.735025202593052,1.),(1.,0.707106781186548,1.)))
REPRESENTATION_ITEM('')
SURFACE()
) ;
#109=(
BOUNDED_SURFACE()
B_SPLINE_SURFACE(3,2,((#139930,#139931,#139932),(#139933,#139934,#139935),
(#139936,#139937,#139938),(#139939,#139940,#139941)),.UNSPECIFIED.,.F.,
 .F.,.F.)
B_SPLINE_SURFACE_WITH_KNOTS((4,4),(3,3),(4.71238898038469,6.28318530717959),
(0.,1.),.UNSPECIFIED.)
GEOMETRIC_REPRESENTATION_ITEM()
RATIONAL_B_SPLINE_SURFACE(((1.,0.707106781186548,1.),(1.,0.735025202593053,
1.),(1.,0.758151925542945,1.),(1.,0.75750200074082,1.)))
REPRESENTATION_ITEM('')
SURFACE()
) ;
#110=(
BOUNDED_SURFACE()
B_SPLINE_SURFACE(3,2,((#140939,#140940,#140941),(#140942,#140943,#140944),
(#140945,#140946,#140947),(#140948,#140949,#140950),(#140951,#140952,#140953),
(#140954,#140955,#140956)),.UNSPECIFIED.,.F.,.F.,.F.)
B_SPLINE_SURFACE_WITH_KNOTS((4,2,4),(3,3),(3.14159265358979,3.92699081698724,
4.71238898038469),(0.,1.),.UNSPECIFIED.)
GEOMETRIC_REPRESENTATION_ITEM()
RATIONAL_B_SPLINE_SURFACE(((1.,0.934721701546417,1.),(1.,0.934869636336908,
1.),(1.,0.913780519322377,1.),(1.,0.834646315042295,1.),(1.,0.776518516961044,
1.),(1.,0.707106781186548,1.)))
REPRESENTATION_ITEM('')
SURFACE()
) ;
#111=(
BOUNDED_SURFACE()
B_SPLINE_SURFACE(3,2,((#140967,#140968,#140969),(#140970,#140971,#140972),
(#140973,#140974,#140975),(#140976,#140977,#140978)),.UNSPECIFIED.,.F.,
 .F.,.F.)
B_SPLINE_SURFACE_WITH_KNOTS((4,4),(3,3),(1.5707963267949,2.41495031290807),
(0.,1.),.UNSPECIFIED.)
GEOMETRIC_REPRESENTATION_ITEM()
RATIONAL_B_SPLINE_SURFACE(((1.,0.707106781186547,1.),(1.,0.730803471035897,
1.),(1.,0.752906082887246,1.),(1.,0.76729220397862,1.)))
REPRESENTATION_ITEM('')
SURFACE()
) ;
#112=(
BOUNDED_SURFACE()
B_SPLINE_SURFACE(3,2,((#140995,#140996,#140997),(#140998,#140999,#141000),
(#141001,#141002,#141003),(#141004,#141005,#141006),(#141007,#141008,#141009),
(#141010,#141011,#141012)),.UNSPECIFIED.,.F.,.F.,.F.)
B_SPLINE_SURFACE_WITH_KNOTS((4,2,4),(3,3),(1.56955149927815,2.35619449019234,
3.14283748110654),(-0.00124482751675201,1.),.UNSPECIFIED.)
GEOMETRIC_REPRESENTATION_ITEM()
RATIONAL_B_SPLINE_SURFACE(((1.0007306038145,0.706544157856479,1.),(1.00062673753064,
0.748263304672957,1.),(1.00053422463652,0.785422225437718,1.),(1.00040682904414,
0.83659220306961,1.),(1.00037181710673,0.850655170404865,1.),(1.00037229282023,
0.850464094333157,1.)))
REPRESENTATION_ITEM('')
SURFACE()
) ;
#113=(
BOUNDED_SURFACE()
B_SPLINE_SURFACE(3,2,((#141015,#141016,#141017),(#141018,#141019,#141020),
(#141021,#141022,#141023),(#141024,#141025,#141026),(#141027,#141028,#141029),
(#141030,#141031,#141032)),.UNSPECIFIED.,.F.,.F.,.F.)
B_SPLINE_SURFACE_WITH_KNOTS((4,2,4),(3,3),(4.71238898038469,5.49778714378214,
6.28318530717959),(0.,1.),.UNSPECIFIED.)
GEOMETRIC_REPRESENTATION_ITEM()
RATIONAL_B_SPLINE_SURFACE(((1.,0.707106781186548,1.),(1.,0.776518516961005,
1.),(1.,0.834646315042348,1.),(1.,0.913780519322327,1.),(1.,0.934869636336944,
1.),(1.,0.934721701546417,1.)))
REPRESENTATION_ITEM('')
SURFACE()
) ;
#114=(
BOUNDED_SURFACE()
B_SPLINE_SURFACE(3,2,((#141040,#141041,#141042),(#141043,#141044,#141045),
(#141046,#141047,#141048),(#141049,#141050,#141051)),.UNSPECIFIED.,.F.,
 .F.,.F.)
B_SPLINE_SURFACE_WITH_KNOTS((4,4),(3,3),(0.726642340681723,1.5707963267949),
(0.,1.),.UNSPECIFIED.)
GEOMETRIC_REPRESENTATION_ITEM()
RATIONAL_B_SPLINE_SURFACE(((1.,0.76729220397862,1.),(1.,0.752906082887249,
1.),(1.,0.730803471035892,1.),(1.,0.707106781186547,1.)))
REPRESENTATION_ITEM('')
SURFACE()
) ;
#115=(
BOUNDED_SURFACE()
B_SPLINE_SURFACE(3,2,((#141067,#141068,#141069),(#141070,#141071,#141072),
(#141073,#141074,#141075),(#141076,#141077,#141078),(#141079,#141080,#141081),
(#141082,#141083,#141084)),.UNSPECIFIED.,.F.,.F.,.F.)
B_SPLINE_SURFACE_WITH_KNOTS((4,2,4),(3,3),(-0.001244827516706,0.785398163397448,
1.5720411543116),(-0.001244827516706,1.),.UNSPECIFIED.)
GEOMETRIC_REPRESENTATION_ITEM()
RATIONAL_B_SPLINE_SURFACE(((1.00037229282022,0.850464094333164,1.),(1.00037181710672,
0.850655170404816,1.),(1.00040682904413,0.836592203069687,1.),(1.0005342246365,
0.785422225437665,1.),(1.00062673753062,0.748263304673023,1.),(1.00073060381448,
0.7065441578565,1.)))
REPRESENTATION_ITEM('')
SURFACE()
) ;
#116=(
BOUNDED_SURFACE()
B_SPLINE_SURFACE(3,2,((#141096,#141097,#141098),(#141099,#141100,#141101),
(#141102,#141103,#141104),(#141105,#141106,#141107)),.UNSPECIFIED.,.F.,
 .F.,.F.)
B_SPLINE_SURFACE_WITH_KNOTS((4,4),(3,3),(1.10714871779409,1.5707963267949),
(0.,1.),.UNSPECIFIED.)
GEOMETRIC_REPRESENTATION_ITEM()
RATIONAL_B_SPLINE_SURFACE(((1.,0.743704326447947,1.),(1.,0.732676928202348,
1.),(1.,0.720087778783135,1.),(1.,0.707106781186548,1.)))
REPRESENTATION_ITEM('')
SURFACE()
) ;
#117=(
BOUNDED_SURFACE()
B_SPLINE_SURFACE(3,2,((#141115,#141116,#141117),(#141118,#141119,#141120),
(#141121,#141122,#141123),(#141124,#141125,#141126)),.UNSPECIFIED.,.F.,
 .F.,.F.)
B_SPLINE_SURFACE_WITH_KNOTS((4,4),(3,3),(1.5707963267949,2.0344439357957),
(0.,1.),.UNSPECIFIED.)
GEOMETRIC_REPRESENTATION_ITEM()
RATIONAL_B_SPLINE_SURFACE(((1.,0.707106781186548,1.),(1.,0.720087778783125,
1.),(1.,0.732676928202353,1.),(1.,0.743704326447947,1.)))
REPRESENTATION_ITEM('')
SURFACE()
) ;
#118=(
BOUNDED_SURFACE()
B_SPLINE_SURFACE(3,2,((#141394,#141395,#141396),(#141397,#141398,#141399),
(#141400,#141401,#141402),(#141403,#141404,#141405)),.UNSPECIFIED.,.F.,
 .F.,.F.)
B_SPLINE_SURFACE_WITH_KNOTS((4,4),(3,3),(0.000111059871785624,0.00024129664665087),
(0.,1.00030059112224),.UNSPECIFIED.)
GEOMETRIC_REPRESENTATION_ITEM()
RATIONAL_B_SPLINE_SURFACE(((1.,0.839985548969901,1.00009619784682),(1.,
0.797322032917093,1.00012184639516),(1.,0.734686009440409,1.00015950206034),
(1.,0.707018740085206,1.00017613513143)))
REPRESENTATION_ITEM('')
SURFACE()
) ;
#119=(
BOUNDED_SURFACE()
B_SPLINE_SURFACE(3,2,((#141407,#141408,#141409),(#141410,#141411,#141412),
(#141413,#141414,#141415),(#141416,#141417,#141418)),.UNSPECIFIED.,.F.,
 .F.,.F.)
B_SPLINE_SURFACE_WITH_KNOTS((4,4),(3,3),(3.14159265358979,3.68974201455418),
(0.,1.),.UNSPECIFIED.)
GEOMETRIC_REPRESENTATION_ITEM()
RATIONAL_B_SPLINE_SURFACE(((1.,0.860789971413512,1.),(1.,0.860809546755051,
1.),(1.,0.853709425573777,1.),(1.,0.840033633436873,1.)))
REPRESENTATION_ITEM('')
SURFACE()
) ;
#120=(
BOUNDED_SURFACE()
B_SPLINE_SURFACE(3,2,((#141423,#141424,#141425),(#141426,#141427,#141428),
(#141429,#141430,#141431),(#141432,#141433,#141434)),.UNSPECIFIED.,.F.,
 .F.,.F.)
B_SPLINE_SURFACE_WITH_KNOTS((4,4),(3,3),(2.59344329260965,3.14159265358979),
(0.,1.),.UNSPECIFIED.)
GEOMETRIC_REPRESENTATION_ITEM()
RATIONAL_B_SPLINE_SURFACE(((1.,0.840033633435695,1.),(1.,0.853709425573363,
1.),(1.,0.860809546755055,1.),(1.,0.860789971413512,1.)))
REPRESENTATION_ITEM('')
SURFACE()
) ;
#121=(
BOUNDED_SURFACE()
B_SPLINE_SURFACE(3,2,((#141436,#141437,#141438),(#141439,#141440,#141441),
(#141442,#141443,#141444),(#141445,#141446,#141447)),.UNSPECIFIED.,.F.,
 .F.,.F.)
B_SPLINE_SURFACE_WITH_KNOTS((4,4),(3,3),(0.000111059871788868,0.00024129664665087),
(-0.000300086749610278,1.),.UNSPECIFIED.)
GEOMETRIC_REPRESENTATION_ITEM()
RATIONAL_B_SPLINE_SURFACE(((1.00009603638458,0.839985629649299,1.),(1.00012164188339,
0.797322135108613,1.),(1.00015923434582,0.734686143216544,1.),(1.00017583949931,
0.70701888781253,1.)))
REPRESENTATION_ITEM('')
SURFACE()
) ;
#122=(
BOUNDED_SURFACE()
B_SPLINE_SURFACE(3,2,((#141531,#141532,#141533),(#141534,#141535,#141536),
(#141537,#141538,#141539),(#141540,#141541,#141542),(#141543,#141544,#141545),
(#141546,#141547,#141548),(#141549,#141550,#141551),(#141552,#141553,#141554),
(#141555,#141556,#141557),(#141558,#141559,#141560)),.UNSPECIFIED.,.F.,
 .F.,.F.)
B_SPLINE_SURFACE_WITH_KNOTS((4,2,2,2,4),(3,3),(0.00112100122803331,0.00145633576709043,
0.0015908372445872,0.00165808798333558,0.00178849406635726),(-0.000893324189041646,
1.00101552458189),.UNSPECIFIED.)
GEOMETRIC_REPRESENTATION_ITEM()
RATIONAL_B_SPLINE_SURFACE(((1.00061830890901,0.653576280075763,1.00070297498501),
(1.00045188087558,0.74682193383013,1.00051375768181),(1.00032243686644,
0.819346321742964,1.00036658868739),(1.00017052538061,0.904458700444901,
1.000193875707),(1.00013074576005,0.926746272131261,1.00014864899627),(1.0000798364389,
0.955269549338603,1.00009076857638),(1.0000639484811,0.964171192776774,
1.00007270505388),(1.00002748579918,0.98460036292331,1.00003124947578),
(1.00001632684003,0.990852461324468,1.00001856250162),(1.00006581963706,
0.96312282876575,1.00007483243036)))
REPRESENTATION_ITEM('')
SURFACE()
) ;
#123=(
BOUNDED_SURFACE()
B_SPLINE_SURFACE(3,2,((#141601,#141602,#141603),(#141604,#141605,#141606),
(#141607,#141608,#141609),(#141610,#141611,#141612),(#141613,#141614,#141615),
(#141616,#141617,#141618),(#141619,#141620,#141621),(#141622,#141623,#141624),
(#141625,#141626,#141627),(#141628,#141629,#141630)),.UNSPECIFIED.,.F.,
 .F.,.F.)
B_SPLINE_SURFACE_WITH_KNOTS((4,2,2,2,4),(3,3),(0.00112100122803333,0.00145633576709044,
0.00159083724458721,0.00165808798333559,0.00178849406635728),(-0.00113559264181192,
1.),.UNSPECIFIED.)
GEOMETRIC_REPRESENTATION_ITEM()
RATIONAL_B_SPLINE_SURFACE(((1.0007861837979,0.653844270846462,0.999999999999999),
(1.00057456947131,0.747017790468138,1.),(1.00040998057208,0.819486074062655,
1.),(1.00021682413016,0.904532610471955,1.),(1.00016624408397,0.926802940661334,
1.),(1.00010151255113,0.955304152477068,1.),(1.00008131090949,0.964198909671162,
1.),(1.00003494837237,0.984612275966151,1.),(1.00002075968325,0.990859537791165,
1.),(1.00008369009645,0.963151356666752,1.)))
REPRESENTATION_ITEM('')
SURFACE()
) ;
#124=(
BOUNDED_SURFACE()
B_SPLINE_SURFACE(3,2,((#141667,#141668,#141669),(#141670,#141671,#141672),
(#141673,#141674,#141675),(#141676,#141677,#141678),(#141679,#141680,#141681),
(#141682,#141683,#141684),(#141685,#141686,#141687),(#141688,#141689,#141690),
(#141691,#141692,#141693),(#141694,#141695,#141696),(#141697,#141698,#141699),
(#141700,#141701,#141702),(#141703,#141704,#141705),(#141706,#141707,#141708),
(#141709,#141710,#141711),(#141712,#141713,#141714)),.UNSPECIFIED.,.F.,
 .F.,.F.)
B_SPLINE_SURFACE_WITH_KNOTS((4,2,2,2,2,2,2,4),(3,3),(5.6278630844106E-15,
3.85995771599548E-5,5.78993657371183E-5,6.75492600257001E-5,7.23742071699909E-5,
7.47866807421364E-5,7.59929175282091E-5,7.71991543142818E-5),(0.,1.00107899067834),
 .UNSPECIFIED.)
GEOMETRIC_REPRESENTATION_ITEM()
RATIONAL_B_SPLINE_SURFACE(((1.,0.976255617118804,1.00005123993558),(1.,
0.981339981891258,1.00004026797119),(1.,0.986086237829169,1.00003002563937),
(1.,0.992269463037034,1.00001668235464),(1.,0.994174411180042,1.00001257151207),
(1.,0.996706913506702,1.00000710641926),(1.,0.997492596832094,1.00000541092929),
(1.,0.998537621803387,1.00000315578488),(1.,0.998865045809503,1.00000244920998),
(1.,0.999323526852936,1.00000145981644),(1.,0.999468419970867,1.00000114713979),
(1.,0.99959844684718,1.00000086654422),(1.,0.999614491362718,1.00000083192045),
(1.,0.999732489024762,1.0000005772837),(1.,0.999724369239699,1.00000059480604),
(1.,1.,1.)))
REPRESENTATION_ITEM('')
SURFACE()
) ;
#125=(
BOUNDED_SURFACE()
B_SPLINE_SURFACE(3,2,((#141716,#141717,#141718),(#141719,#141720,#141721),
(#141722,#141723,#141724),(#141725,#141726,#141727),(#141728,#141729,#141730),
(#141731,#141732,#141733),(#141734,#141735,#141736),(#141737,#141738,#141739),
(#141740,#141741,#141742),(#141743,#141744,#141745)),.UNSPECIFIED.,.F.,
 .F.,.F.)
B_SPLINE_SURFACE_WITH_KNOTS((4,2,2,2,4),(3,3),(-0.000110707928511331,0.000553539642556653,
0.00083030946383498,0.000968694374474144,0.00121778721363011),(0.,1.00563383762648),
 .UNSPECIFIED.)
GEOMETRIC_REPRESENTATION_ITEM()
RATIONAL_B_SPLINE_SURFACE(((1.,0.710139408519336,1.00326605501343),(1.,
0.691948125897064,1.00347102847846),(1.,0.728232377173955,1.00306218931827),
(1.,0.818030374423766,1.0020503746469),(1.,0.849110759469326,1.00170017096147),
(1.,0.897979778369984,1.00114953072656),(1.,0.914666724297552,1.00096150763889),
(1.,0.961090538823421,1.00043841917281),(1.,0.990973799041186,1.00010170430117),
(1.,0.992463455161859,1.00008491933977)))
REPRESENTATION_ITEM('')
SURFACE()
) ;
#126=(
BOUNDED_SURFACE()
B_SPLINE_SURFACE(3,2,((#141747,#141748,#141749),(#141750,#141751,#141752),
(#141753,#141754,#141755),(#141756,#141757,#141758),(#141759,#141760,#141761),
(#141762,#141763,#141764),(#141765,#141766,#141767),(#141768,#141769,#141770),
(#141771,#141772,#141773),(#141774,#141775,#141776)),.UNSPECIFIED.,.F.,
 .F.,.F.)
B_SPLINE_SURFACE_WITH_KNOTS((4,2,2,2,4),(3,3),(-0.000137915648493739,0.000139027965246064,
0.000278055930499746,0.00055611186100711,0.00125013859505175),(-0.000741678185789884,
1.00283457365337),.UNSPECIFIED.)
GEOMETRIC_REPRESENTATION_ITEM()
RATIONAL_B_SPLINE_SURFACE(((1.00001340810331,0.990935328832968,1.00005135076275),
(1.00000300543756,0.997968146378497,1.0000115103164),(1.00005311279899,
0.96409260530696,1.00020341301648),(1.00012590576287,0.914880254704378,
1.00048219772838),(1.00015093966345,0.897955856706366,1.00057807332388),
(1.00022375355362,0.848729358697935,1.00085693817989),(1.00026920263033,
0.818003093715416,1.00103100043918),(1.00040494517438,0.726233102312152,
1.001550871372),(1.00045889592401,0.689759203410882,1.00175749359735),(1.00042429005326,
0.713154819594753,1.00162495897875)))
REPRESENTATION_ITEM('')
SURFACE()
) ;
#127=(
BOUNDED_SURFACE()
B_SPLINE_SURFACE(3,2,((#141778,#141779,#141780),(#141781,#141782,#141783),
(#141784,#141785,#141786),(#141787,#141788,#141789),(#141790,#141791,#141792),
(#141793,#141794,#141795),(#141796,#141797,#141798),(#141799,#141800,#141801),
(#141802,#141803,#141804),(#141805,#141806,#141807),(#141808,#141809,#141810),
(#141811,#141812,#141813),(#141814,#141815,#141816),(#141817,#141818,#141819),
(#141820,#141821,#141822),(#141823,#141824,#141825)),.UNSPECIFIED.,.F.,
 .F.,.F.)
B_SPLINE_SURFACE_WITH_KNOTS((4,2,2,2,2,2,2,4),(3,3),(7.77892019462184E-15,
3.88447601478307E-5,5.82671402178566E-5,6.79783302528695E-5,7.2833925270376E-5,
7.52617227791293E-5,7.64756215335059E-5,7.76895202878825E-5),(-0.0012094552576271,
1.01080070868954),.UNSPECIFIED.)
GEOMETRIC_REPRESENTATION_ITEM()
RATIONAL_B_SPLINE_SURFACE(((1.00005744302266,0.975995723233527,1.00051789333955),
(1.00004519813152,0.981112615457371,1.0004074961621),(1.00003362760161,
0.985947705765597,1.00030317887351),(1.00001854219783,0.992251590743248,
1.00016717227456),(1.00001393966879,0.994174894491124,1.0001256769106),
(1.00000788875349,0.996703449551651,1.00007112322264),(1.00000601414708,
0.997486809637525,1.00005422219392),(1.00000351698944,0.998530321282699,
1.00003170838373),(1.00000273459082,0.998857269833631,1.0000246544542),
(1.00000163903614,0.999315079965992,1.00001477718022),(1.00000129000885,
0.999460931405225,1.00001163042892),(1.0000009745592,0.99959275143124,1.000008786406),
(1.00000093560708,0.99960902873406,1.00000843522246),(1.00000065019919,
0.999728294915417,1.00000586204929),(1.00000066918571,0.99972036083143,
1.00000603322751),(1.,1.,1.)))
REPRESENTATION_ITEM('')
SURFACE()
) ;
#267=ELLIPSE('',#91249,0.191322338734783,0.178429548359619) ;
#268=ELLIPSE('',#91250,0.19132233878183,0.178429548383724) ;
#269=ELLIPSE('',#91251,0.191322338731802,0.178429548357439) ;
#270=ELLIPSE('',#91252,0.191322338779123,0.17842954838245) ;
#271=ELLIPSE('',#91300,0.190951225717336,0.171364150514683) ;
#272=ELLIPSE('',#91301,0.184110979856706,0.15942086075581) ;
#273=ELLIPSE('',#91303,0.102944309528002,0.0999999999999975) ;
#274=ELLIPSE('',#91304,0.102944309527982,0.0999999999999795) ;
#275=ELLIPSE('',#91305,0.102944309527979,0.0999999999999756) ;
#276=ELLIPSE('',#91306,0.102944309527978,0.0999999999999751) ;
#277=ELLIPSE('',#91308,0.184110979853722,0.159420860750542) ;
#278=ELLIPSE('',#91309,0.19095122571746,0.171364150514935) ;
#279=ELLIPSE('',#91378,0.102447207929153,0.0855466862257129) ;
#280=ELLIPSE('',#91388,0.102447207928901,0.0855466862253011) ;
#281=ELLIPSE('',#91393,0.141421356237246,0.099999999999956) ;
#282=ELLIPSE('',#91411,0.141421356237246,0.0999999999999589) ;
#283=ELLIPSE('',#91422,0.111310931434027,0.0999999999994426) ;
#284=ELLIPSE('',#91426,0.111310931436794,0.100000000004093) ;
#285=ELLIPSE('',#91433,0.126113554280143,0.0912763326628817) ;
#286=ELLIPSE('',#91447,0.126113554274935,0.0912763326607385) ;
#287=ELLIPSE('',#91665,0.190951225717095,0.171364150514224) ;
#288=ELLIPSE('',#91666,0.18411097985465,0.159420860752213) ;
#289=ELLIPSE('',#91668,0.102944309528002,0.0999999999999973) ;
#290=ELLIPSE('',#91669,0.102944309528015,0.100000000000011) ;
#291=ELLIPSE('',#91670,0.102944309528021,0.100000000000013) ;
#292=ELLIPSE('',#91671,0.102944309527952,0.0999999999999486) ;
#293=ELLIPSE('',#91673,0.184110979853536,0.159420860750266) ;
#294=ELLIPSE('',#91674,0.19095122571723,0.17136415051449) ;
#295=ELLIPSE('',#91743,0.102447207929021,0.085546686225496) ;
#296=ELLIPSE('',#91753,0.102447207929205,0.0855466862258343) ;
#297=ELLIPSE('',#91758,0.14142135623734,0.100000000000021) ;
#298=ELLIPSE('',#91776,0.141421356237089,0.0999999999998527) ;
#299=ELLIPSE('',#91787,0.11131093143594,0.100000000002612) ;
#300=ELLIPSE('',#91791,0.111310931435708,0.10000000000223) ;
#301=ELLIPSE('',#91798,0.126113554274573,0.0912763326605795) ;
#302=ELLIPSE('',#91811,0.126113554276116,0.0912763326612655) ;
#303=ELLIPSE('',#92137,0.191322338736984,0.178429548360737) ;
#304=ELLIPSE('',#92138,0.191322338786359,0.178429548386577) ;
#305=ELLIPSE('',#92139,0.191322338724264,0.17842954835187) ;
#306=ELLIPSE('',#92140,0.191322338783867,0.178429548384638) ;
#307=ELLIPSE('',#92189,0.190951225717061,0.171364150514171) ;
#308=ELLIPSE('',#92190,0.184110979854607,0.159420860752121) ;
#309=ELLIPSE('',#92192,0.102944309527925,0.0999999999999341) ;
#310=ELLIPSE('',#92193,0.102944309528208,0.100000000000198) ;
#311=ELLIPSE('',#92194,0.102944309528197,0.100000000000187) ;
#312=ELLIPSE('',#92195,0.10294430952777,0.0999999999997609) ;
#313=ELLIPSE('',#92197,0.184110979849685,0.159420860743423) ;
#314=ELLIPSE('',#92198,0.190951225717448,0.171364150514883) ;
#315=ELLIPSE('',#92267,0.102447207929559,0.0855466862264446) ;
#316=ELLIPSE('',#92277,0.102447207929716,0.0855466862267171) ;
#317=ELLIPSE('',#92282,0.141421356237578,0.100000000000185) ;
#318=ELLIPSE('',#92300,0.141421356237136,0.0999999999998538) ;
#319=ELLIPSE('',#92311,0.111310931434914,0.100000000000826) ;
#320=ELLIPSE('',#92315,0.111310931434193,0.099999999999555) ;
#321=ELLIPSE('',#92322,0.12611355428909,0.0912763326666119) ;
#322=ELLIPSE('',#92336,0.126113554268033,0.0912763326579103) ;
#323=ELLIPSE('',#92554,0.190951225717901,0.171364150515768) ;
#324=ELLIPSE('',#92555,0.184110979854194,0.159420860751403) ;
#325=ELLIPSE('',#92557,0.102944309528061,0.100000000000057) ;
#326=ELLIPSE('',#92558,0.102944309528071,0.100000000000074) ;
#327=ELLIPSE('',#92559,0.102944309527994,0.0999999999999879) ;
#328=ELLIPSE('',#92560,0.102944309527827,0.0999999999998399) ;
#329=ELLIPSE('',#92562,0.184110979851928,0.159420860747419) ;
#330=ELLIPSE('',#92563,0.190951225717375,0.17136415051477) ;
#331=ELLIPSE('',#92632,0.102447207928804,0.0855466862251576) ;
#332=ELLIPSE('',#92642,0.102447207929456,0.0855466862262483) ;
#333=ELLIPSE('',#92647,0.141421356237259,0.0999999999999835) ;
#334=ELLIPSE('',#92665,0.141421356237111,0.0999999999998622) ;
#335=ELLIPSE('',#92676,0.111310931436081,0.100000000002901) ;
#336=ELLIPSE('',#92680,0.111310931433336,0.0999999999981691) ;
#337=ELLIPSE('',#92686,0.126113554288552,0.0912763326663696) ;
#338=ELLIPSE('',#92700,0.126113554294105,0.0912763326688326) ;
#339=ELLIPSE('',#92960,0.191322338738038,0.178429548361451) ;
#340=ELLIPSE('',#92961,0.191322338777325,0.178429548380458) ;
#341=ELLIPSE('',#93028,0.190951225717903,0.171364150515775) ;
#342=ELLIPSE('',#93029,0.184110979854543,0.159420860752014) ;
#343=ELLIPSE('',#93031,0.10294430952807,0.100000000000064) ;
#344=ELLIPSE('',#93032,0.102944309528103,0.1000000000001) ;
#345=ELLIPSE('',#93033,0.102944309528091,0.100000000000089) ;
#346=ELLIPSE('',#93034,0.102944309527858,0.0999999999998653) ;
#347=ELLIPSE('',#93036,0.184110979854767,0.159420860752386) ;
#348=ELLIPSE('',#93037,0.190951225717425,0.171364150514857) ;
#349=ELLIPSE('',#93106,0.102447207929024,0.0855466862255089) ;
#350=ELLIPSE('',#93116,0.102447207928841,0.0855466862251956) ;
#351=ELLIPSE('',#93121,0.141421356237363,0.100000000000039) ;
#352=ELLIPSE('',#93139,0.141421356237142,0.0999999999998897) ;
#353=ELLIPSE('',#93150,0.111310931435548,0.10000000000196) ;
#354=ELLIPSE('',#93154,0.111310931436154,0.100000000003053) ;
#355=ELLIPSE('',#93161,0.126113554273832,0.0912763326602602) ;
#356=ELLIPSE('',#93175,0.126113554282611,0.0912763326639418) ;
#647=FACE_BOUND('',#22787,.T.) ;
#648=FACE_BOUND('',#22800,.T.) ;
#649=FACE_BOUND('',#22801,.T.) ;
#650=FACE_BOUND('',#22807,.T.) ;
#651=FACE_BOUND('',#22808,.T.) ;
#652=FACE_BOUND('',#22809,.T.) ;
#653=FACE_BOUND('',#22810,.T.) ;
#654=FACE_BOUND('',#22815,.T.) ;
#655=FACE_BOUND('',#22816,.T.) ;
#656=FACE_BOUND('',#22818,.T.) ;
#657=FACE_BOUND('',#22819,.T.) ;
#658=FACE_BOUND('',#22839,.T.) ;
#659=FACE_BOUND('',#22858,.T.) ;
#660=FACE_BOUND('',#23042,.T.) ;
#661=FACE_BOUND('',#23061,.T.) ;
#662=FACE_BOUND('',#23250,.T.) ;
#663=FACE_BOUND('',#23263,.T.) ;
#664=FACE_BOUND('',#23264,.T.) ;
#665=FACE_BOUND('',#23270,.T.) ;
#666=FACE_BOUND('',#23271,.T.) ;
#667=FACE_BOUND('',#23272,.T.) ;
#668=FACE_BOUND('',#23273,.T.) ;
#669=FACE_BOUND('',#23278,.T.) ;
#670=FACE_BOUND('',#23279,.T.) ;
#671=FACE_BOUND('',#23281,.T.) ;
#672=FACE_BOUND('',#23282,.T.) ;
#673=FACE_BOUND('',#23302,.T.) ;
#674=FACE_BOUND('',#23321,.T.) ;
#675=FACE_BOUND('',#23505,.T.) ;
#676=FACE_BOUND('',#23524,.T.) ;
#677=FACE_BOUND('',#23706,.T.) ;
#678=FACE_BOUND('',#23716,.T.) ;
#679=FACE_BOUND('',#23717,.T.) ;
#680=FACE_BOUND('',#23722,.T.) ;
#681=FACE_BOUND('',#23724,.T.) ;
#682=FACE_BOUND('',#23745,.T.) ;
#683=FACE_BOUND('',#23764,.T.) ;
#794=PLANE('',#91213) ;
#795=PLANE('',#91216) ;
#796=PLANE('',#91217) ;
#797=PLANE('',#91218) ;
#798=PLANE('',#91232) ;
#799=PLANE('',#91235) ;
#800=PLANE('',#91236) ;
#801=PLANE('',#91237) ;
#802=PLANE('',#91238) ;
#803=PLANE('',#91247) ;
#804=PLANE('',#91248) ;
#805=PLANE('',#91253) ;
#806=PLANE('',#91254) ;
#807=PLANE('',#91255) ;
#808=PLANE('',#91264) ;
#809=PLANE('',#91265) ;
#810=PLANE('',#91266) ;
#811=PLANE('',#91267) ;
#812=PLANE('',#91268) ;
#813=PLANE('',#91277) ;
#814=PLANE('',#91278) ;
#815=PLANE('',#91279) ;
#816=PLANE('',#91281) ;
#817=PLANE('',#91282) ;
#818=PLANE('',#91297) ;
#819=PLANE('',#91298) ;
#820=PLANE('',#91299) ;
#821=PLANE('',#91302) ;
#822=PLANE('',#91307) ;
#823=PLANE('',#91310) ;
#824=PLANE('',#91311) ;
#825=PLANE('',#91312) ;
#826=PLANE('',#91313) ;
#827=PLANE('',#91314) ;
#828=PLANE('',#91315) ;
#829=PLANE('',#91316) ;
#830=PLANE('',#91317) ;
#831=PLANE('',#91318) ;
#832=PLANE('',#91325) ;
#833=PLANE('',#91328) ;
#834=PLANE('',#91331) ;
#835=PLANE('',#91334) ;
#836=PLANE('',#91335) ;
#837=PLANE('',#91336) ;
#838=PLANE('',#91337) ;
#839=PLANE('',#91338) ;
#840=PLANE('',#91339) ;
#841=PLANE('',#91340) ;
#842=PLANE('',#91341) ;
#843=PLANE('',#91342) ;
#844=PLANE('',#91343) ;
#845=PLANE('',#91344) ;
#846=PLANE('',#91351) ;
#847=PLANE('',#91354) ;
#848=PLANE('',#91357) ;
#849=PLANE('',#91360) ;
#850=PLANE('',#91361) ;
#851=PLANE('',#91362) ;
#852=PLANE('',#91363) ;
#853=PLANE('',#91364) ;
#854=PLANE('',#91365) ;
#855=PLANE('',#91367) ;
#856=PLANE('',#91629) ;
#857=PLANE('',#91630) ;
#858=PLANE('',#91634) ;
#859=PLANE('',#91638) ;
#860=PLANE('',#91642) ;
#861=PLANE('',#91646) ;
#862=PLANE('',#91647) ;
#863=PLANE('',#91649) ;
#864=PLANE('',#91651) ;
#865=PLANE('',#91653) ;
#866=PLANE('',#91654) ;
#867=PLANE('',#91655) ;
#868=PLANE('',#91656) ;
#869=PLANE('',#91662) ;
#870=PLANE('',#91663) ;
#871=PLANE('',#91664) ;
#872=PLANE('',#91667) ;
#873=PLANE('',#91672) ;
#874=PLANE('',#91675) ;
#875=PLANE('',#91676) ;
#876=PLANE('',#91677) ;
#877=PLANE('',#91678) ;
#878=PLANE('',#91679) ;
#879=PLANE('',#91680) ;
#880=PLANE('',#91681) ;
#881=PLANE('',#91682) ;
#882=PLANE('',#91683) ;
#883=PLANE('',#91690) ;
#884=PLANE('',#91693) ;
#885=PLANE('',#91696) ;
#886=PLANE('',#91699) ;
#887=PLANE('',#91700) ;
#888=PLANE('',#91701) ;
#889=PLANE('',#91702) ;
#890=PLANE('',#91703) ;
#891=PLANE('',#91704) ;
#892=PLANE('',#91705) ;
#893=PLANE('',#91706) ;
#894=PLANE('',#91707) ;
#895=PLANE('',#91708) ;
#896=PLANE('',#91709) ;
#897=PLANE('',#91716) ;
#898=PLANE('',#91719) ;
#899=PLANE('',#91722) ;
#900=PLANE('',#91725) ;
#901=PLANE('',#91726) ;
#902=PLANE('',#91727) ;
#903=PLANE('',#91728) ;
#904=PLANE('',#91729) ;
#905=PLANE('',#91730) ;
#906=PLANE('',#91732) ;
#907=PLANE('',#92102) ;
#908=PLANE('',#92105) ;
#909=PLANE('',#92106) ;
#910=PLANE('',#92107) ;
#911=PLANE('',#92121) ;
#912=PLANE('',#92123) ;
#913=PLANE('',#92124) ;
#914=PLANE('',#92125) ;
#915=PLANE('',#92126) ;
#916=PLANE('',#92135) ;
#917=PLANE('',#92136) ;
#918=PLANE('',#92141) ;
#919=PLANE('',#92142) ;
#920=PLANE('',#92143) ;
#921=PLANE('',#92152) ;
#922=PLANE('',#92153) ;
#923=PLANE('',#92154) ;
#924=PLANE('',#92155) ;
#925=PLANE('',#92156) ;
#926=PLANE('',#92165) ;
#927=PLANE('',#92166) ;
#928=PLANE('',#92167) ;
#929=PLANE('',#92170) ;
#930=PLANE('',#92171) ;
#931=PLANE('',#92186) ;
#932=PLANE('',#92187) ;
#933=PLANE('',#92188) ;
#934=PLANE('',#92191) ;
#935=PLANE('',#92196) ;
#936=PLANE('',#92199) ;
#937=PLANE('',#92200) ;
#938=PLANE('',#92201) ;
#939=PLANE('',#92202) ;
#940=PLANE('',#92203) ;
#941=PLANE('',#92204) ;
#942=PLANE('',#92205) ;
#943=PLANE('',#92206) ;
#944=PLANE('',#92207) ;
#945=PLANE('',#92214) ;
#946=PLANE('',#92217) ;
#947=PLANE('',#92220) ;
#948=PLANE('',#92223) ;
#949=PLANE('',#92224) ;
#950=PLANE('',#92225) ;
#951=PLANE('',#92226) ;
#952=PLANE('',#92227) ;
#953=PLANE('',#92228) ;
#954=PLANE('',#92229) ;
#955=PLANE('',#92230) ;
#956=PLANE('',#92231) ;
#957=PLANE('',#92232) ;
#958=PLANE('',#92233) ;
#959=PLANE('',#92240) ;
#960=PLANE('',#92243) ;
#961=PLANE('',#92246) ;
#962=PLANE('',#92249) ;
#963=PLANE('',#92250) ;
#964=PLANE('',#92251) ;
#965=PLANE('',#92252) ;
#966=PLANE('',#92253) ;
#967=PLANE('',#92254) ;
#968=PLANE('',#92256) ;
#969=PLANE('',#92518) ;
#970=PLANE('',#92519) ;
#971=PLANE('',#92523) ;
#972=PLANE('',#92527) ;
#973=PLANE('',#92531) ;
#974=PLANE('',#92535) ;
#975=PLANE('',#92536) ;
#976=PLANE('',#92538) ;
#977=PLANE('',#92540) ;
#978=PLANE('',#92541) ;
#979=PLANE('',#92542) ;
#980=PLANE('',#92543) ;
#981=PLANE('',#92545) ;
#982=PLANE('',#92551) ;
#983=PLANE('',#92552) ;
#984=PLANE('',#92553) ;
#985=PLANE('',#92556) ;
#986=PLANE('',#92561) ;
#987=PLANE('',#92564) ;
#988=PLANE('',#92565) ;
#989=PLANE('',#92566) ;
#990=PLANE('',#92567) ;
#991=PLANE('',#92568) ;
#992=PLANE('',#92569) ;
#993=PLANE('',#92570) ;
#994=PLANE('',#92571) ;
#995=PLANE('',#92572) ;
#996=PLANE('',#92579) ;
#997=PLANE('',#92582) ;
#998=PLANE('',#92585) ;
#999=PLANE('',#92588) ;
#1000=PLANE('',#92589) ;
#1001=PLANE('',#92590) ;
#1002=PLANE('',#92591) ;
#1003=PLANE('',#92592) ;
#1004=PLANE('',#92593) ;
#1005=PLANE('',#92594) ;
#1006=PLANE('',#92595) ;
#1007=PLANE('',#92596) ;
#1008=PLANE('',#92597) ;
#1009=PLANE('',#92598) ;
#1010=PLANE('',#92605) ;
#1011=PLANE('',#92608) ;
#1012=PLANE('',#92611) ;
#1013=PLANE('',#92614) ;
#1014=PLANE('',#92615) ;
#1015=PLANE('',#92616) ;
#1016=PLANE('',#92617) ;
#1017=PLANE('',#92618) ;
#1018=PLANE('',#92619) ;
#1019=PLANE('',#92621) ;
#1020=PLANE('',#92948) ;
#1021=PLANE('',#92950) ;
#1022=PLANE('',#92951) ;
#1023=PLANE('',#92952) ;
#1024=PLANE('',#92953) ;
#1025=PLANE('',#92958) ;
#1026=PLANE('',#92959) ;
#1027=PLANE('',#92962) ;
#1028=PLANE('',#92963) ;
#1029=PLANE('',#92964) ;
#1030=PLANE('',#92965) ;
#1031=PLANE('',#92966) ;
#1032=PLANE('',#92967) ;
#1033=PLANE('',#92968) ;
#1034=PLANE('',#92973) ;
#1035=PLANE('',#92974) ;
#1036=PLANE('',#92975) ;
#1037=PLANE('',#92976) ;
#1038=PLANE('',#92977) ;
#1039=PLANE('',#92982) ;
#1040=PLANE('',#92983) ;
#1041=PLANE('',#92984) ;
#1042=PLANE('',#92986) ;
#1043=PLANE('',#92987) ;
#1044=PLANE('',#93006) ;
#1045=PLANE('',#93025) ;
#1046=PLANE('',#93026) ;
#1047=PLANE('',#93027) ;
#1048=PLANE('',#93030) ;
#1049=PLANE('',#93035) ;
#1050=PLANE('',#93038) ;
#1051=PLANE('',#93039) ;
#1052=PLANE('',#93040) ;
#1053=PLANE('',#93041) ;
#1054=PLANE('',#93042) ;
#1055=PLANE('',#93043) ;
#1056=PLANE('',#93044) ;
#1057=PLANE('',#93045) ;
#1058=PLANE('',#93046) ;
#1059=PLANE('',#93053) ;
#1060=PLANE('',#93056) ;
#1061=PLANE('',#93059) ;
#1062=PLANE('',#93062) ;
#1063=PLANE('',#93063) ;
#1064=PLANE('',#93064) ;
#1065=PLANE('',#93065) ;
#1066=PLANE('',#93066) ;
#1067=PLANE('',#93067) ;
#1068=PLANE('',#93068) ;
#1069=PLANE('',#93069) ;
#1070=PLANE('',#93070) ;
#1071=PLANE('',#93071) ;
#1072=PLANE('',#93072) ;
#1073=PLANE('',#93079) ;
#1074=PLANE('',#93082) ;
#1075=PLANE('',#93085) ;
#1076=PLANE('',#93088) ;
#1077=PLANE('',#93089) ;
#1078=PLANE('',#93090) ;
#1079=PLANE('',#93091) ;
#1080=PLANE('',#93092) ;
#1081=PLANE('',#93093) ;
#1082=PLANE('',#93095) ;
#1999=B_SPLINE_CURVE_WITH_KNOTS('',3,(#132623,#132624,#132625,#132626,#132627,
#132628,#132629,#132630,#132631,#132632),.UNSPECIFIED.,.F.,.F.,(4,2,2,2,
4),(0.0155454932989835,0.0194994353522834,0.0234533774055832,0.0272081302045205,
0.0309628830034577),.UNSPECIFIED.) ;
#2000=B_SPLINE_CURVE_WITH_KNOTS('',3,(#132636,#132637,#132638,#132639,#132640,
#132641,#132642,#132643,#132644,#132645),.UNSPECIFIED.,.F.,.F.,(4,2,2,2,
4),(-0.0304888223793686,-0.0267236306519753,-0.0229584389245819,-0.0190821381960852,
-0.0152058374675885),.UNSPECIFIED.) ;
#2001=B_SPLINE_CURVE_WITH_KNOTS('',3,(#132649,#132650,#132651,#132652,#132653,
#132654,#132655,#132656,#132657,#132658),.UNSPECIFIED.,.F.,.F.,(4,2,2,2,
4),(-0.0457718072911488,-0.041895506562652,-0.0380192058341553,-0.034254014106762,
-0.0304888223793686),.UNSPECIFIED.) ;
#2002=B_SPLINE_CURVE_WITH_KNOTS('',3,(#132662,#132663,#132664,#132665,#132666,
#132667,#132668,#132669,#132670,#132671,#132672,#132673,#132674,#132675,
#132676,#132677,#132678,#132679,#132680,#132681,#132682,#132683,#132684,
#132685,#132686,#132687,#132688,#132689,#132690,#132691,#132692),
 .UNSPECIFIED.,.F.,.F.,(4,3,3,3,3,3,3,3,3,3,4),(0.,1.73748728562045E-5,
3.26506729531324E-5,5.02804002574634E-5,6.52741227887637E-5,8.3439070256478E-5,
9.83241608049985E-5,0.00011756895656783,0.00013250051079383,0.000151525967767889,
0.000159849152172774),.UNSPECIFIED.) ;
#2003=B_SPLINE_CURVE_WITH_KNOTS('',3,(#132696,#132697,#132698,#132699,#132700,
#132701,#132702,#132703,#132704,#132705),.UNSPECIFIED.,.F.,.F.,(4,2,2,2,
4),(0.0155454932989835,0.0194994353522834,0.0234533774055832,0.0272081302045204,
0.0309628830034577),.UNSPECIFIED.) ;
#2004=B_SPLINE_CURVE_WITH_KNOTS('',3,(#132709,#132710,#132711,#132712,#132713,
#132714,#132715,#132716,#132717,#132718),.UNSPECIFIED.,.F.,.F.,(4,2,2,2,
4),(-0.0304888223793686,-0.0267236306519752,-0.0229584389245819,-0.0190821381960852,
-0.0152058374675885),.UNSPECIFIED.) ;
#2005=B_SPLINE_CURVE_WITH_KNOTS('',3,(#132722,#132723,#132724,#132725,#132726,
#132727,#132728,#132729,#132730,#132731),.UNSPECIFIED.,.F.,.F.,(4,2,2,2,
4),(-0.0457718072911488,-0.0418955065626521,-0.0380192058341553,-0.034254014106762,
-0.0304888223793686),.UNSPECIFIED.) ;
#2006=B_SPLINE_CURVE_WITH_KNOTS('',3,(#132735,#132736,#132737,#132738,#132739,
#132740,#132741,#132742,#132743,#132744,#132745,#132746,#132747,#132748,
#132749,#132750,#132751,#132752,#132753,#132754,#132755,#132756,#132757,
#132758,#132759,#132760,#132761,#132762,#132763,#132764,#132765),
 .UNSPECIFIED.,.F.,.F.,(4,3,3,3,3,3,3,3,3,3,4),(0.,1.73748728562068E-5,
3.26506729531323E-5,5.02804002574648E-5,6.52741227887635E-5,8.34390702564692E-5,
9.83241608049985E-5,0.000117568956567848,0.00013250051079383,0.000151525967767866,
0.000159849152172774),.UNSPECIFIED.) ;
#2007=B_SPLINE_CURVE_WITH_KNOTS('',3,(#132848,#132849,#132850,#132851,#132852,
#132853,#132854,#132855,#132856,#132857),.UNSPECIFIED.,.F.,.F.,(4,2,2,2,
4),(0.0155454932989836,0.0194994353522834,0.0234533774055832,0.0272081302045205,
0.0309628830034577),.UNSPECIFIED.) ;
#2008=B_SPLINE_CURVE_WITH_KNOTS('',3,(#132861,#132862,#132863,#132864,#132865,
#132866,#132867,#132868,#132869,#132870),.UNSPECIFIED.,.F.,.F.,(4,2,2,2,
4),(-0.0304888223793686,-0.0267236306519753,-0.0229584389245819,-0.0190821381960852,
-0.0152058374675885),.UNSPECIFIED.) ;
#2009=B_SPLINE_CURVE_WITH_KNOTS('',3,(#132874,#132875,#132876,#132877,#132878,
#132879,#132880,#132881,#132882,#132883),.UNSPECIFIED.,.F.,.F.,(4,2,2,2,
4),(-0.0457718072911489,-0.0418955065626522,-0.0380192058341554,-0.0342540141067621,
-0.0304888223793687),.UNSPECIFIED.) ;
#2010=B_SPLINE_CURVE_WITH_KNOTS('',3,(#132887,#132888,#132889,#132890,#132891,
#132892,#132893,#132894,#132895,#132896,#132897,#132898,#132899,#132900,
#132901,#132902,#132903,#132904,#132905,#132906,#132907,#132908,#132909,
#132910,#132911,#132912,#132913,#132914,#132915,#132916,#132917),
 .UNSPECIFIED.,.F.,.F.,(4,3,3,3,3,3,3,3,3,3,4),(0.,1.73748728562045E-5,
3.26506729531323E-5,5.02804002574719E-5,6.52741227887636E-5,8.34390702564519E-5,
9.83241608049985E-5,0.000117568956567851,0.00013250051079383,0.00015152596776785,
0.000159849152172774),.UNSPECIFIED.) ;
#2011=B_SPLINE_CURVE_WITH_KNOTS('',3,(#132921,#132922,#132923,#132924,#132925,
#132926,#132927,#132928,#132929,#132930),.UNSPECIFIED.,.F.,.F.,(4,2,2,2,
4),(0.0155454932989836,0.0194994353522834,0.0234533774055832,0.0272081302045205,
0.0309628830034577),.UNSPECIFIED.) ;
#2012=B_SPLINE_CURVE_WITH_KNOTS('',3,(#132934,#132935,#132936,#132937,#132938,
#132939,#132940,#132941,#132942,#132943),.UNSPECIFIED.,.F.,.F.,(4,2,2,2,
4),(-0.0304888223793687,-0.0267236306519753,-0.022958438924582,-0.0190821381960853,
-0.0152058374675885),.UNSPECIFIED.) ;
#2013=B_SPLINE_CURVE_WITH_KNOTS('',3,(#132947,#132948,#132949,#132950,#132951,
#132952,#132953,#132954,#132955,#132956),.UNSPECIFIED.,.F.,.F.,(4,2,2,2,
4),(-0.0457718072911488,-0.0418955065626521,-0.0380192058341554,-0.034254014106762,
-0.0304888223793687),.UNSPECIFIED.) ;
#2014=B_SPLINE_CURVE_WITH_KNOTS('',3,(#132960,#132961,#132962,#132963,#132964,
#132965,#132966,#132967,#132968,#132969,#132970,#132971,#132972,#132973,
#132974,#132975,#132976,#132977,#132978,#132979,#132980,#132981,#132982,
#132983,#132984,#132985,#132986,#132987,#132988,#132989,#132990),
 .UNSPECIFIED.,.F.,.F.,(4,3,3,3,3,3,3,3,3,3,4),(0.,1.73748728562037E-5,
3.26506729531323E-5,5.02804002574677E-5,6.52741227887636E-5,8.34390702564633E-5,
9.83241608049985E-5,0.000117568956567858,0.00013250051079383,0.000151525967767868,
0.000159849152172774),.UNSPECIFIED.) ;
#2015=B_SPLINE_CURVE_WITH_KNOTS('',3,(#133008,#133009,#133010,#133011),
 .UNSPECIFIED.,.F.,.F.,(4,4),(0.,1.5707963267949),.UNSPECIFIED.) ;
#2016=B_SPLINE_CURVE_WITH_KNOTS('',3,(#133015,#133016,#133017,#133018),
 .UNSPECIFIED.,.F.,.F.,(4,4),(1.5707963267949,3.14159265358979),
 .UNSPECIFIED.) ;
#2017=B_SPLINE_CURVE_WITH_KNOTS('',3,(#133260,#133261,#133262,#133263,#133264,
#133265),.UNSPECIFIED.,.F.,.F.,(4,2,4),(3.14159265358979,3.92699081698724,
4.71238898038469),.UNSPECIFIED.) ;
#2018=B_SPLINE_CURVE_WITH_KNOTS('',3,(#133269,#133270,#133271,#133272,#133273,
#133274),.UNSPECIFIED.,.F.,.F.,(4,2,4),(3.14159265358979,3.92699081698724,
4.71238898038469),.UNSPECIFIED.) ;
#2019=B_SPLINE_CURVE_WITH_KNOTS('',3,(#133278,#133279,#133280,#133281,#133282,
#133283),.UNSPECIFIED.,.F.,.F.,(4,2,4),(4.71238898038469,5.49778714378214,
6.28318530717959),.UNSPECIFIED.) ;
#2020=B_SPLINE_CURVE_WITH_KNOTS('',3,(#133286,#133287,#133288,#133289,#133290,
#133291),.UNSPECIFIED.,.F.,.F.,(4,2,4),(4.71238898038469,5.49778714378214,
6.28318530717959),.UNSPECIFIED.) ;
#2021=B_SPLINE_CURVE_WITH_KNOTS('',3,(#133296,#133297,#133298,#133299,#133300,
#133301),.UNSPECIFIED.,.F.,.F.,(4,2,4),(3.14159265358979,3.92699081698724,
4.71238898038469),.UNSPECIFIED.) ;
#2022=B_SPLINE_CURVE_WITH_KNOTS('',3,(#133305,#133306,#133307,#133308,#133309,
#133310),.UNSPECIFIED.,.F.,.F.,(4,2,4),(3.14159265358979,3.92699081698724,
4.71238898038469),.UNSPECIFIED.) ;
#2023=B_SPLINE_CURVE_WITH_KNOTS('',3,(#133314,#133315,#133316,#133317,#133318,
#133319),.UNSPECIFIED.,.F.,.F.,(4,2,4),(4.71238898038469,5.49778714378214,
6.28318530717959),.UNSPECIFIED.) ;
#2024=B_SPLINE_CURVE_WITH_KNOTS('',3,(#133322,#133323,#133324,#133325,#133326,
#133327),.UNSPECIFIED.,.F.,.F.,(4,2,4),(4.71238898038469,5.49778714378214,
6.28318530717959),.UNSPECIFIED.) ;
#2025=B_SPLINE_CURVE_WITH_KNOTS('',3,(#133381,#133382,#133383,#133384,#133385,
#133386,#133387,#133388,#133389,#133390,#133391,#133392,#133393,#133394,
#133395,#133396,#133397,#133398,#133399,#133400,#133401,#133402,#133403,
#133404,#133405,#133406,#133407,#133408),.UNSPECIFIED.,.F.,.F.,(4,3,3,3,
3,3,3,3,3,4),(2.16840434497101E-19,0.00010866297864345,0.0002173259572869,
0.000239795331094194,0.000268321712743107,0.000359692996641291,0.000370380550777844,
0.000402443213187502,0.000469559030214579,0.000479590662188387),
 .UNSPECIFIED.) ;
#2026=B_SPLINE_CURVE_WITH_KNOTS('',3,(#133410,#133411,#133412,#133413,#133414,
#133415,#133416,#133417,#133418,#133419),.UNSPECIFIED.,.F.,.F.,(4,2,2,2,
4),(4.46821448257462E-15,0.000139027965256961,0.000278055930509455,0.000556111861014442,
0.00111222372202442),.UNSPECIFIED.) ;
#2027=B_SPLINE_CURVE_WITH_KNOTS('',3,(#133421,#133422,#133423,#133424,#133425,
#133426,#133427,#133428,#133429,#133430,#133431,#133432,#133433,#133434,
#133435,#133436,#133437,#133438,#133439,#133440,#133441,#133442,#133443,
#133444,#133445),.UNSPECIFIED.,.F.,.F.,(4,3,3,3,3,3,3,3,4),(0.,0.000553539642553921,
0.000830309463830882,0.000968694374469362,0.000985992488299172,0.00104653588670351,
0.00108059154830595,0.00109383541670689,0.00110707928510784),
 .UNSPECIFIED.) ;
#2028=B_SPLINE_CURVE_WITH_KNOTS('',3,(#133447,#133448,#133449,#133450,#133451,
#133452,#133453,#133454,#133455,#133456,#133457,#133458,#133459,#133460,
#133461,#133462),.UNSPECIFIED.,.F.,.F.,(4,2,2,2,2,2,2,4),(2.46381126959653E-5,
3.49307346223092E-5,0.000103812737360936,0.000147753773859884,0.000241616793832017,
0.000270869435023803,0.000448933238085274,0.000517100757351641),
 .UNSPECIFIED.) ;
#2029=B_SPLINE_CURVE_WITH_KNOTS('',3,(#133474,#133475,#133476,#133477,#133478,
#133479,#133480,#133481,#133482,#133483,#133484,#133485,#133486,#133487,
#133488,#133489,#133490,#133491,#133492,#133493,#133494,#133495,#133496,
#133497,#133498,#133499,#133500,#133501),.UNSPECIFIED.,.F.,.F.,(4,3,3,3,
3,3,3,3,3,4),(0.,0.000108662978644149,0.000217325957288299,0.000239795331094193,
0.000268321712743106,0.00035969299664129,0.000370380550777843,0.000402443213187502,
0.000469559030214579,0.000479590662188388),.UNSPECIFIED.) ;
#2030=B_SPLINE_CURVE_WITH_KNOTS('',3,(#133503,#133504,#133505,#133506,#133507,
#133508,#133509,#133510,#133511,#133512),.UNSPECIFIED.,.F.,.F.,(4,2,2,2,
4),(4.4671593419464E-15,0.000139027965256961,0.000278055930509454,0.000556111861014442,
0.00111222372202441),.UNSPECIFIED.) ;
#2031=B_SPLINE_CURVE_WITH_KNOTS('',3,(#133514,#133515,#133516,#133517,#133518,
#133519,#133520,#133521,#133522,#133523,#133524,#133525,#133526,#133527,
#133528,#133529,#133530,#133531,#133532,#133533,#133534,#133535,#133536,
#133537,#133538),.UNSPECIFIED.,.F.,.F.,(4,3,3,3,3,3,3,3,4),(0.,0.000553539642553921,
0.000830309463830883,0.000968694374469362,0.000985992488299172,0.00104653588670351,
0.00108059154830595,0.00109383541670689,0.00110707928510784),
 .UNSPECIFIED.) ;
#2032=B_SPLINE_CURVE_WITH_KNOTS('',3,(#133540,#133541,#133542,#133543,#133544,
#133545,#133546,#133547,#133548,#133549,#133550,#133551,#133552,#133553,
#133554,#133555),.UNSPECIFIED.,.F.,.F.,(4,2,2,2,2,2,2,4),(2.46381126959657E-5,
3.49307346223102E-5,0.000103812737360935,0.000147753773859885,0.000241616793832018,
0.000270869435023804,0.000448933238082175,0.00051710075735164),
 .UNSPECIFIED.) ;
#2033=B_SPLINE_CURVE_WITH_KNOTS('',3,(#133959,#133960,#133961,#133962,#133963,
#133964),.UNSPECIFIED.,.F.,.F.,(4,2,4),(1.5707963267949,2.35619449019234,
3.14159265358979),.UNSPECIFIED.) ;
#2034=B_SPLINE_CURVE_WITH_KNOTS('',3,(#134035,#134036,#134037,#134038,#134039,
#134040),.UNSPECIFIED.,.F.,.F.,(4,2,4),(0.,0.785398163397445,1.57079632679489),
 .UNSPECIFIED.) ;
#2035=B_SPLINE_CURVE_WITH_KNOTS('',3,(#134134,#134135,#134136,#134137,#134138,
#134139,#134140,#134141,#134142,#134143,#134144,#134145,#134146,#134147,
#134148,#134149,#134150,#134151,#134152),.UNSPECIFIED.,.F.,.F.,(4,3,3,3,
3,3,4),(5.8575878041605E-5,6.39772274846954E-5,8.50081925564311E-5,0.000101719137060913,
0.000115369906146044,0.000121992710600423,0.000127737589255657),
 .UNSPECIFIED.) ;
#2036=B_SPLINE_CURVE_WITH_KNOTS('',3,(#134159,#134160,#134161,#134162,#134163,
#134164,#134165,#134166,#134167,#134168,#134169,#134170,#134171,#134172),
 .UNSPECIFIED.,.F.,.F.,(4,2,2,2,2,2,4),(0.000106030898883045,0.000114450588602972,
0.0001358619160635,0.000155180925252374,0.000169070632935497,0.000187290067688934,
0.000202757041675869),.UNSPECIFIED.) ;
#2037=B_SPLINE_CURVE_WITH_KNOTS('',3,(#134173,#134174,#134175,#134176,#134177,
#134178,#134179,#134180,#134181,#134182,#134183,#134184,#134185,#134186),
 .UNSPECIFIED.,.F.,.F.,(4,2,2,2,2,2,4),(0.,1.81852425157699E-5,3.36231897823057E-5,
5.26817905680866E-5,7.3668643005217E-5,8.81407292049458E-5,9.65446177718808E-5),
 .UNSPECIFIED.) ;
#2038=B_SPLINE_CURVE_WITH_KNOTS('',3,(#134196,#134197,#134198,#134199,#134200,
#134201,#134202,#134203,#134204,#134205,#134206,#134207,#134208,#134209,
#134210,#134211,#134212,#134213,#134214),.UNSPECIFIED.,.F.,.F.,(4,3,3,3,
3,3,4),(0.,1.26126247467577E-5,2.08447799633808E-5,2.61321988210988E-5,
4.72564717706651E-5,6.39499555081058E-5,6.93621596435636E-5),
 .UNSPECIFIED.) ;
#2039=B_SPLINE_CURVE_WITH_KNOTS('',3,(#134324,#134325,#134326,#134327,#134328,
#134329,#134330,#134331,#134332,#134333,#134334,#134335),.UNSPECIFIED.,
 .F.,.F.,(4,2,2,2,2,4),(2.16840434497101E-19,0.000230913708713648,0.000346370563070472,
0.000404098990248884,0.00043296320383809,0.000461827417427296),
 .UNSPECIFIED.) ;
#2040=B_SPLINE_CURVE_WITH_KNOTS('',3,(#134362,#134363,#134364,#134365,#134366,
#134367,#134368,#134369,#134370,#134371,#134372,#134373),.UNSPECIFIED.,
 .F.,.F.,(4,2,2,2,2,4),(0.,2.92942635586613E-5,5.85885271173226E-5,0.000117177054234646,
0.000234354108469295,0.000468708216938589),.UNSPECIFIED.) ;
#2041=B_SPLINE_CURVE_WITH_KNOTS('',3,(#134463,#134464,#134465,#134466,#134467,
#134468,#134469,#134470,#134471,#134472,#134473,#134474),.UNSPECIFIED.,
 .F.,.F.,(4,2,2,2,2,4),(7.70621319460113E-10,0.000528455713264078,0.000792683184585458,
0.000924796920246148,0.000990853788076493,0.00105691065590684),
 .UNSPECIFIED.) ;
#2042=B_SPLINE_CURVE_WITH_KNOTS('',3,(#134475,#134476,#134477,#134478,#134479,
#134480,#134481,#134482,#134483,#134484,#134485,#134486,#134487,#134488,
#134489,#134490,#134491,#134492,#134493,#134494,#134495,#134496,#134497,
#134498,#134499,#134500,#134501,#134502),.UNSPECIFIED.,.F.,.F.,(4,2,2,2,
2,2,2,2,2,2,2,2,2,4),(0.,1.88814447164022E-5,2.66390109708352E-5,2.82246506940909E-5,
2.82548001019668E-5,4.36852952398544E-5,4.37205777570019E-5,4.63087975636132E-5,
5.19857273366478E-5,5.63013930903595E-5,5.77982263345347E-5,5.8493669267456E-5,
5.96281966878496E-5,6.07824730943691E-5),.UNSPECIFIED.) ;
#2043=B_SPLINE_CURVE_WITH_KNOTS('',3,(#134504,#134505,#134506,#134507,#134508,
#134509,#134510,#134511,#134512,#134513,#134514,#134515,#134516,#134517,
#134518,#134519,#134520,#134521,#134522,#134523,#134524,#134525),
 .UNSPECIFIED.,.F.,.F.,(4,2,2,2,2,2,2,2,2,2,4),(-2.98424671548918E-6,-1.83179854035004E-6,
-6.78494605943823E-7,0.,1.61207185756534E-6,5.98431127542647E-6,1.25056665528015E-5,
1.40350946485193E-5,2.93914218611999E-5,4.85423642734616E-5,5.82245408950306E-5),
 .UNSPECIFIED.) ;
#2044=B_SPLINE_CURVE_WITH_KNOTS('',3,(#134526,#134527,#134528,#134529,#134530,
#134531,#134532,#134533,#134534,#134535,#134536,#134537),.UNSPECIFIED.,
 .F.,.F.,(4,2,2,2,2,4),(0.,6.61189708719518E-5,0.000132237941743904,0.000264475883487807,
0.000528951766975614,0.00105790353395123),.UNSPECIFIED.) ;
#2045=B_SPLINE_CURVE_WITH_KNOTS('',3,(#134570,#134571,#134572,#134573,#134574,
#134575,#134576,#134577,#134578,#134579,#134580,#134581,#134582,#134583,
#134584,#134585,#134586,#134587,#134588,#134589,#134590,#134591,#134592,
#134593,#134594,#134595,#134596,#134597,#134598,#134599,#134600,#134601,
#134602,#134603,#134604,#134605,#134606,#134607),.UNSPECIFIED.,.F.,.F.,
(4,2,2,2,2,2,2,2,2,2,2,2,2,2,2,2,2,2,4),(4.08242498362039E-13,1.91825894880777E-5,
2.29499826201368E-5,2.74799101222728E-5,3.52358269328764E-5,4.12198651829317E-5,
4.25319315563255E-5,4.54442131893302E-5,4.69409045132628E-5,4.80898427132611E-5,
4.9446473946099E-5,4.96432742482141E-5,5.04298720437356E-5,5.14115331535164E-5,
5.17333590635578E-5,5.22889985287821E-5,5.29242843672018E-5,5.37719008581487E-5,
5.49598202435906E-5),.UNSPECIFIED.) ;
#2046=B_SPLINE_CURVE_WITH_KNOTS('',3,(#134641,#134642,#134643,#134644,#134645,
#134646,#134647,#134648,#134649,#134650,#134651,#134652,#134653,#134654,
#134655,#134656,#134657,#134658,#134659,#134660,#134661,#134662,#134663,
#134664,#134665,#134666,#134667,#134668,#134669,#134670,#134671,#134672,
#134673,#134674,#134675,#134676),.UNSPECIFIED.,.F.,.F.,(4,2,2,2,2,2,2,2,
2,2,2,2,2,2,2,2,2,4),(-2.90335387328764E-6,-1.36780202085548E-6,-6.41515161605833E-7,
-6.4061093095502E-8,3.81173304657634E-7,1.44450314270962E-6,2.24472183150878E-6,
2.5078329807616E-6,3.96662365739235E-6,5.28616271355818E-6,8.35978425194598E-6,
9.71024741494835E-6,1.08366011880723E-5,1.65505252295058E-5,2.45765562494323E-5,
2.90642498315122E-5,4.41638722239744E-5,5.20477084101052E-5),
 .UNSPECIFIED.) ;
#2047=B_SPLINE_CURVE_WITH_KNOTS('',3,(#135327,#135328,#135329,#135330,#135331,
#135332),.UNSPECIFIED.,.F.,.F.,(4,2,4),(1.5707963267949,2.35619449019234,
3.14159265358979),.UNSPECIFIED.) ;
#2048=B_SPLINE_CURVE_WITH_KNOTS('',3,(#135403,#135404,#135405,#135406,#135407,
#135408),.UNSPECIFIED.,.F.,.F.,(4,2,4),(0.,0.785398163397448,1.57079632679489),
 .UNSPECIFIED.) ;
#2049=B_SPLINE_CURVE_WITH_KNOTS('',3,(#135502,#135503,#135504,#135505,#135506,
#135507,#135508,#135509,#135510,#135511,#135512,#135513,#135514,#135515,
#135516,#135517,#135518,#135519,#135520),.UNSPECIFIED.,.F.,.F.,(4,3,3,3,
3,3,4),(5.85758780416049E-5,6.39772274846956E-5,8.50081925566845E-5,0.000101719137060913,
0.000115369906146169,0.000121992710600423,0.000127737589255657),
 .UNSPECIFIED.) ;
#2050=B_SPLINE_CURVE_WITH_KNOTS('',3,(#135527,#135528,#135529,#135530,#135531,
#135532,#135533,#135534,#135535,#135536,#135537,#135538,#135539,#135540),
 .UNSPECIFIED.,.F.,.F.,(4,2,2,2,2,2,4),(0.000106030898883045,0.000114450588602972,
0.000135861916063515,0.000155180925252387,0.000169070632935497,0.000187290067688863,
0.000202757041675869),.UNSPECIFIED.) ;
#2051=B_SPLINE_CURVE_WITH_KNOTS('',3,(#135541,#135542,#135543,#135544,#135545,
#135546,#135547,#135548,#135549,#135550,#135551,#135552,#135553,#135554),
 .UNSPECIFIED.,.F.,.F.,(4,2,2,2,2,2,4),(0.,1.81852425155684E-5,3.36231897823057E-5,
5.26817905680615E-5,7.36686430051892E-5,8.81407292049454E-5,9.65446177718809E-5),
 .UNSPECIFIED.) ;
#2052=B_SPLINE_CURVE_WITH_KNOTS('',3,(#135563,#135564,#135565,#135566,#135567,
#135568,#135569,#135570,#135571,#135572,#135573,#135574,#135575,#135576,
#135577,#135578,#135579,#135580,#135581),.UNSPECIFIED.,.F.,.F.,(4,3,3,3,
3,3,4),(0.,1.26126247467848E-5,2.08447799633808E-5,2.61321988210988E-5,
4.72564717709744E-5,6.39499555081057E-5,6.93621596435632E-5),
 .UNSPECIFIED.) ;
#2053=B_SPLINE_CURVE_WITH_KNOTS('',3,(#135691,#135692,#135693,#135694,#135695,
#135696,#135697,#135698,#135699,#135700,#135701,#135702),.UNSPECIFIED.,
 .F.,.F.,(4,2,2,2,2,4),(4.33680868994202E-19,0.000230913708713649,0.000346370563070474,
0.000404098990248885,0.000432963203838091,0.000461827417427296),
 .UNSPECIFIED.) ;
#2054=B_SPLINE_CURVE_WITH_KNOTS('',3,(#135723,#135724,#135725,#135726,#135727,
#135728,#135729,#135730,#135731,#135732,#135733,#135734),.UNSPECIFIED.,
 .F.,.F.,(4,2,2,2,2,4),(0.,2.92942635586604E-5,5.85885271173207E-5,0.000117177054234645,
0.000234354108469293,0.000468708216938593),.UNSPECIFIED.) ;
#2055=B_SPLINE_CURVE_WITH_KNOTS('',3,(#135803,#135804,#135805,#135806,#135807,
#135808,#135809,#135810,#135811,#135812,#135813,#135814),.UNSPECIFIED.,
 .F.,.F.,(4,2,2,2,2,4),(7.70621318557099E-10,0.000528455713264077,0.000792683184585457,
0.000924796920246147,0.000990853788076492,0.00105691065590684),
 .UNSPECIFIED.) ;
#2056=B_SPLINE_CURVE_WITH_KNOTS('',3,(#135815,#135816,#135817,#135818,#135819,
#135820,#135821,#135822,#135823,#135824,#135825,#135826,#135827,#135828,
#135829,#135830,#135831,#135832,#135833,#135834,#135835,#135836,#135837,
#135838,#135839,#135840,#135841,#135842),.UNSPECIFIED.,.F.,.F.,(4,2,2,2,
2,2,2,2,2,2,2,2,2,4),(0.,1.88814447164821E-5,2.66390109708352E-5,2.82246506940927E-5,
2.82548001019694E-5,4.36852952398541E-5,4.37205777570016E-5,4.63087975636134E-5,
5.19857273366473E-5,5.63013930903587E-5,5.77982263345345E-5,5.84936692674544E-5,
5.96281966878474E-5,6.07824730943697E-5),.UNSPECIFIED.) ;
#2057=B_SPLINE_CURVE_WITH_KNOTS('',3,(#135844,#135845,#135846,#135847,#135848,
#135849,#135850,#135851,#135852,#135853,#135854,#135855,#135856,#135857,
#135858,#135859,#135860,#135861,#135862,#135863,#135864,#135865),
 .UNSPECIFIED.,.F.,.F.,(4,2,2,2,2,2,2,2,2,2,4),(-2.98424671548898E-6,-1.83179854035005E-6,
-6.78494605944079E-7,0.,1.61207185756418E-6,5.9843112754236E-6,1.25056665528019E-5,
1.40350946485009E-5,2.93914218611391E-5,4.85423642729475E-5,5.82245408950306E-5),
 .UNSPECIFIED.) ;
#2058=B_SPLINE_CURVE_WITH_KNOTS('',3,(#135866,#135867,#135868,#135869,#135870,
#135871,#135872,#135873,#135874,#135875,#135876,#135877),.UNSPECIFIED.,
 .F.,.F.,(4,2,2,2,2,4),(0.,6.61189708719504E-5,0.000132237941743901,0.000264475883487804,
0.000528951766975613,0.00105790353395123),.UNSPECIFIED.) ;
#2059=B_SPLINE_CURVE_WITH_KNOTS('',3,(#135908,#135909,#135910,#135911,#135912,
#135913,#135914,#135915,#135916,#135917,#135918,#135919,#135920,#135921,
#135922,#135923,#135924,#135925,#135926,#135927,#135928,#135929,#135930,
#135931,#135932,#135933,#135934,#135935,#135936,#135937,#135938,#135939,
#135940,#135941,#135942,#135943,#135944,#135945),.UNSPECIFIED.,.F.,.F.,
(4,2,2,2,2,2,2,2,2,2,2,2,2,2,2,2,2,2,4),(4.08242998125434E-13,1.91825894890263E-5,
2.29499826201337E-5,2.74799101222727E-5,3.52358269328724E-5,4.12198651829315E-5,
4.25319315563219E-5,4.54442131893529E-5,4.694090451326E-5,4.8089842713261E-5,
4.94464739460923E-5,4.9643274248211E-5,5.04298720437361E-5,5.14115331535221E-5,
5.17333590635549E-5,5.22889985287794E-5,5.29242843671993E-5,5.3771900858147E-5,
5.49598202435904E-5),.UNSPECIFIED.) ;
#2060=B_SPLINE_CURVE_WITH_KNOTS('',3,(#135978,#135979,#135980,#135981,#135982,
#135983,#135984,#135985,#135986,#135987,#135988,#135989,#135990,#135991,
#135992,#135993,#135994,#135995,#135996,#135997,#135998,#135999,#136000,
#136001,#136002,#136003,#136004,#136005,#136006,#136007,#136008,#136009,
#136010,#136011,#136012,#136013),.UNSPECIFIED.,.F.,.F.,(4,2,2,2,2,2,2,2,
2,2,2,2,2,2,2,2,2,4),(-2.90335387328765E-6,-1.36780202088648E-6,-6.41515161635526E-7,
-6.40610931249841E-8,3.81173304645144E-7,1.44450314269772E-6,2.24472183150306E-6,
2.5078329807503E-6,3.96662365739234E-6,5.28616271355017E-6,8.35978425189786E-6,
9.71024741494142E-6,1.08366011880723E-5,1.65505252294989E-5,2.45765562494323E-5,
2.9064249831501E-5,4.41638722239248E-5,5.20477084101053E-5),
 .UNSPECIFIED.) ;
#2061=B_SPLINE_CURVE_WITH_KNOTS('',3,(#136198,#136199,#136200,#136201),
 .UNSPECIFIED.,.F.,.F.,(4,4),(3.14159265358979,4.71238898038469),
 .UNSPECIFIED.) ;
#2062=B_SPLINE_CURVE_WITH_KNOTS('',3,(#136206,#136207,#136208,#136209),
 .UNSPECIFIED.,.F.,.F.,(4,4),(4.71238898038469,6.28318530717959),
 .UNSPECIFIED.) ;
#2063=B_SPLINE_CURVE_WITH_KNOTS('',3,(#136326,#136327,#136328,#136329,#136330,
#136331,#136332,#136333,#136334,#136335),.UNSPECIFIED.,.F.,.F.,(4,2,2,2,
4),(0.0155454932989846,0.0194994353522841,0.0234533774055837,0.0272081302045207,
0.0309628830034577),.UNSPECIFIED.) ;
#2064=B_SPLINE_CURVE_WITH_KNOTS('',3,(#136339,#136340,#136341,#136342,#136343,
#136344,#136345,#136346,#136347,#136348),.UNSPECIFIED.,.F.,.F.,(4,2,2,2,
4),(-0.0304888223793687,-0.0267236306519748,-0.0229584389245809,-0.0190821381960837,
-0.0152058374675865),.UNSPECIFIED.) ;
#2065=B_SPLINE_CURVE_WITH_KNOTS('',3,(#136352,#136353,#136354,#136355,#136356,
#136357,#136358,#136359,#136360,#136361),.UNSPECIFIED.,.F.,.F.,(4,2,2,2,
4),(-0.0457718072911502,-0.0418955065626531,-0.038019205834156,-0.0342540141067624,
-0.0304888223793687),.UNSPECIFIED.) ;
#2066=B_SPLINE_CURVE_WITH_KNOTS('',3,(#136365,#136366,#136367,#136368,#136369,
#136370,#136371,#136372,#136373,#136374,#136375,#136376,#136377,#136378,
#136379,#136380,#136381,#136382,#136383,#136384,#136385,#136386,#136387,
#136388,#136389,#136390,#136391,#136392,#136393,#136394,#136395),
 .UNSPECIFIED.,.F.,.F.,(4,3,3,3,3,3,3,3,3,3,4),(0.,1.73748728561907E-5,
3.26506729531324E-5,5.02804002574635E-5,6.52741227887648E-5,8.34390702564386E-5,
9.83241608050006E-5,0.000117568956567835,0.000132500510793831,0.000151525967767874,
0.000159849152172776),.UNSPECIFIED.) ;
#2067=B_SPLINE_CURVE_WITH_KNOTS('',3,(#136399,#136400,#136401,#136402,#136403,
#136404,#136405,#136406,#136407,#136408),.UNSPECIFIED.,.F.,.F.,(4,2,2,2,
4),(0.015545493298985,0.0194994353522845,0.023453377405584,0.0272081302045209,
0.0309628830034578),.UNSPECIFIED.) ;
#2068=B_SPLINE_CURVE_WITH_KNOTS('',3,(#136412,#136413,#136414,#136415,#136416,
#136417,#136418,#136419,#136420,#136421),.UNSPECIFIED.,.F.,.F.,(4,2,2,2,
4),(-0.0304888223793687,-0.0267236306519748,-0.0229584389245809,-0.0190821381960837,
-0.0152058374675865),.UNSPECIFIED.) ;
#2069=B_SPLINE_CURVE_WITH_KNOTS('',3,(#136425,#136426,#136427,#136428,#136429,
#136430,#136431,#136432,#136433,#136434),.UNSPECIFIED.,.F.,.F.,(4,2,2,2,
4),(-0.0457718072911503,-0.0418955065626532,-0.0380192058341561,-0.0342540141067624,
-0.0304888223793688),.UNSPECIFIED.) ;
#2070=B_SPLINE_CURVE_WITH_KNOTS('',3,(#136438,#136439,#136440,#136441,#136442,
#136443,#136444,#136445,#136446,#136447,#136448,#136449,#136450,#136451,
#136452,#136453,#136454,#136455,#136456,#136457,#136458,#136459,#136460,
#136461,#136462,#136463,#136464,#136465,#136466,#136467,#136468),
 .UNSPECIFIED.,.F.,.F.,(4,3,3,3,3,3,3,3,3,3,4),(0.,1.73748728562053E-5,
3.26506729531322E-5,5.02804002574541E-5,6.52741227887639E-5,8.34390702564725E-5,
9.8324160804999E-5,0.000117568956567813,0.00013250051079383,0.000151525967767858,
0.000159849152172774),.UNSPECIFIED.) ;
#2071=B_SPLINE_CURVE_WITH_KNOTS('',3,(#136551,#136552,#136553,#136554,#136555,
#136556,#136557,#136558,#136559,#136560),.UNSPECIFIED.,.F.,.F.,(4,2,2,2,
4),(0.0155454932989845,0.019499435352284,0.0234533774055836,0.0272081302045206,
0.0309628830034576),.UNSPECIFIED.) ;
#2072=B_SPLINE_CURVE_WITH_KNOTS('',3,(#136564,#136565,#136566,#136567,#136568,
#136569,#136570,#136571,#136572,#136573),.UNSPECIFIED.,.F.,.F.,(4,2,2,2,
4),(-0.0304888223793686,-0.0267236306519753,-0.0229584389245819,-0.0190821381960852,
-0.0152058374675885),.UNSPECIFIED.) ;
#2073=B_SPLINE_CURVE_WITH_KNOTS('',3,(#136577,#136578,#136579,#136580,#136581,
#136582,#136583,#136584,#136585,#136586),.UNSPECIFIED.,.F.,.F.,(4,2,2,2,
4),(-0.04577180729115,-0.041895506562653,-0.0380192058341561,-0.0342540141067623,
-0.0304888223793686),.UNSPECIFIED.) ;
#2074=B_SPLINE_CURVE_WITH_KNOTS('',3,(#136590,#136591,#136592,#136593,#136594,
#136595,#136596,#136597,#136598,#136599,#136600,#136601,#136602,#136603,
#136604,#136605,#136606,#136607,#136608,#136609,#136610,#136611,#136612,
#136613,#136614,#136615,#136616,#136617,#136618,#136619,#136620),
 .UNSPECIFIED.,.F.,.F.,(4,3,3,3,3,3,3,3,3,3,4),(0.,1.73748728562061E-5,
3.26506729531324E-5,5.02804002574579E-5,6.52741227887648E-5,8.34390702564438E-5,
9.83241608050006E-5,0.000117568956567808,0.000132500510793831,0.000151525967767823,
0.000159849152172776),.UNSPECIFIED.) ;
#2075=B_SPLINE_CURVE_WITH_KNOTS('',3,(#136624,#136625,#136626,#136627,#136628,
#136629,#136630,#136631,#136632,#136633),.UNSPECIFIED.,.F.,.F.,(4,2,2,2,
4),(0.0155454932989848,0.0194994353522843,0.0234533774055838,0.0272081302045207,
0.0309628830034576),.UNSPECIFIED.) ;
#2076=B_SPLINE_CURVE_WITH_KNOTS('',3,(#136637,#136638,#136639,#136640,#136641,
#136642,#136643,#136644,#136645,#136646),.UNSPECIFIED.,.F.,.F.,(4,2,2,2,
4),(-0.0304888223793686,-0.0267236306519748,-0.0229584389245809,-0.0190821381960837,
-0.0152058374675865),.UNSPECIFIED.) ;
#2077=B_SPLINE_CURVE_WITH_KNOTS('',3,(#136650,#136651,#136652,#136653,#136654,
#136655,#136656,#136657,#136658,#136659),.UNSPECIFIED.,.F.,.F.,(4,2,2,2,
4),(-0.04577180729115,-0.041895506562653,-0.038019205834156,-0.0342540141067624,
-0.0304888223793687),.UNSPECIFIED.) ;
#2078=B_SPLINE_CURVE_WITH_KNOTS('',3,(#136663,#136664,#136665,#136666,#136667,
#136668,#136669,#136670,#136671,#136672,#136673,#136674,#136675,#136676,
#136677,#136678,#136679,#136680,#136681,#136682,#136683,#136684,#136685,
#136686,#136687,#136688,#136689,#136690,#136691,#136692,#136693),
 .UNSPECIFIED.,.F.,.F.,(4,3,3,3,3,3,3,3,3,3,4),(0.,1.73748728562032E-5,
3.26506729531328E-5,5.02804002574436E-5,6.52741227887643E-5,8.34390702564541E-5,
9.83241608049997E-5,0.000117568956567832,0.00013250051079383,0.000151525967767753,
0.000159849152172774),.UNSPECIFIED.) ;
#2079=B_SPLINE_CURVE_WITH_KNOTS('',3,(#136711,#136712,#136713,#136714),
 .UNSPECIFIED.,.F.,.F.,(4,4),(0.,1.5707963267949),.UNSPECIFIED.) ;
#2080=B_SPLINE_CURVE_WITH_KNOTS('',3,(#136718,#136719,#136720,#136721),
 .UNSPECIFIED.,.F.,.F.,(4,4),(1.5707963267949,3.14159265358979),
 .UNSPECIFIED.) ;
#2081=B_SPLINE_CURVE_WITH_KNOTS('',3,(#136963,#136964,#136965,#136966,#136967,
#136968),.UNSPECIFIED.,.F.,.F.,(4,2,4),(3.14159265358979,3.92699081698724,
4.71238898038469),.UNSPECIFIED.) ;
#2082=B_SPLINE_CURVE_WITH_KNOTS('',3,(#136972,#136973,#136974,#136975,#136976,
#136977),.UNSPECIFIED.,.F.,.F.,(4,2,4),(3.14159265358979,3.92699081698724,
4.71238898038469),.UNSPECIFIED.) ;
#2083=B_SPLINE_CURVE_WITH_KNOTS('',3,(#136981,#136982,#136983,#136984,#136985,
#136986),.UNSPECIFIED.,.F.,.F.,(4,2,4),(4.71238898038469,5.49778714378214,
6.28318530717959),.UNSPECIFIED.) ;
#2084=B_SPLINE_CURVE_WITH_KNOTS('',3,(#136989,#136990,#136991,#136992,#136993,
#136994),.UNSPECIFIED.,.F.,.F.,(4,2,4),(4.71238898038469,5.49778714378214,
6.28318530717959),.UNSPECIFIED.) ;
#2085=B_SPLINE_CURVE_WITH_KNOTS('',3,(#136999,#137000,#137001,#137002,#137003,
#137004),.UNSPECIFIED.,.F.,.F.,(4,2,4),(3.14159265358979,3.92699081698724,
4.71238898038469),.UNSPECIFIED.) ;
#2086=B_SPLINE_CURVE_WITH_KNOTS('',3,(#137008,#137009,#137010,#137011,#137012,
#137013),.UNSPECIFIED.,.F.,.F.,(4,2,4),(3.14159265358979,3.92699081698724,
4.71238898038469),.UNSPECIFIED.) ;
#2087=B_SPLINE_CURVE_WITH_KNOTS('',3,(#137017,#137018,#137019,#137020,#137021,
#137022),.UNSPECIFIED.,.F.,.F.,(4,2,4),(4.71238898038469,5.49778714378214,
6.28318530717959),.UNSPECIFIED.) ;
#2088=B_SPLINE_CURVE_WITH_KNOTS('',3,(#137025,#137026,#137027,#137028,#137029,
#137030),.UNSPECIFIED.,.F.,.F.,(4,2,4),(4.71238898038469,5.49778714378214,
6.28318530717959),.UNSPECIFIED.) ;
#2089=B_SPLINE_CURVE_WITH_KNOTS('',3,(#137084,#137085,#137086,#137087,#137088,
#137089,#137090,#137091,#137092,#137093,#137094,#137095,#137096,#137097,
#137098,#137099,#137100,#137101,#137102,#137103,#137104,#137105,#137106,
#137107,#137108,#137109,#137110,#137111),.UNSPECIFIED.,.F.,.F.,(4,3,3,3,
3,3,3,3,3,4),(0.,0.000108662978650454,0.000217325957300909,0.000239795331094189,
0.00026832171274309,0.000359692996641288,0.000370380550777836,0.000402443213187482,
0.000469559030214573,0.000479590662188388),.UNSPECIFIED.) ;
#2090=B_SPLINE_CURVE_WITH_KNOTS('',3,(#137113,#137114,#137115,#137116,#137117,
#137118,#137119,#137120,#137121,#137122),.UNSPECIFIED.,.F.,.F.,(4,2,2,2,
4),(4.46893664505693E-15,0.00013902796525696,0.000278055930509451,0.000556111861014443,
0.00111222372202442),.UNSPECIFIED.) ;
#2091=B_SPLINE_CURVE_WITH_KNOTS('',3,(#137124,#137125,#137126,#137127,#137128,
#137129,#137130,#137131,#137132,#137133,#137134,#137135,#137136,#137137,
#137138,#137139,#137140,#137141,#137142,#137143,#137144,#137145,#137146,
#137147,#137148),.UNSPECIFIED.,.F.,.F.,(4,3,3,3,3,3,3,3,4),(0.,0.000553539642553915,
0.000830309463830878,0.000968694374469359,0.000985992488299169,0.0010465358867035,
0.00108059154830594,0.00109383541670689,0.00110707928510784),
 .UNSPECIFIED.) ;
#2092=B_SPLINE_CURVE_WITH_KNOTS('',3,(#137150,#137151,#137152,#137153,#137154,
#137155,#137156,#137157,#137158,#137159,#137160,#137161,#137162,#137163,
#137164,#137165),.UNSPECIFIED.,.F.,.F.,(4,2,2,2,2,2,2,4),(2.46381126959637E-5,
3.49307346222979E-5,0.000103812737360902,0.00014775377385988,0.000241616793832009,
0.000270869435023796,0.000448933238137038,0.000517100757351638),
 .UNSPECIFIED.) ;
#2093=B_SPLINE_CURVE_WITH_KNOTS('',3,(#137169,#137170,#137171,#137172,#137173,
#137174,#137175,#137176,#137177,#137178,#137179,#137180,#137181,#137182,
#137183,#137184,#137185,#137186,#137187,#137188,#137189,#137190,#137191,
#137192,#137193,#137194,#137195,#137196),.UNSPECIFIED.,.F.,.F.,(4,3,3,3,
3,3,3,3,3,4),(0.,0.000108662978648,0.000217325957296001,0.000239795331094189,
0.000268321712743099,0.000359692996641288,0.000370380550777836,0.00040244321318748,
0.000469559030214573,0.000479590662188388),.UNSPECIFIED.) ;
#2094=B_SPLINE_CURVE_WITH_KNOTS('',3,(#137198,#137199,#137200,#137201,#137202,
#137203,#137204,#137205,#137206,#137207),.UNSPECIFIED.,.F.,.F.,(4,2,2,2,
4),(4.46893664505693E-15,0.00013902796525696,0.00027805593050945,0.000556111861014442,
0.00111222372202442),.UNSPECIFIED.) ;
#2095=B_SPLINE_CURVE_WITH_KNOTS('',3,(#137209,#137210,#137211,#137212,#137213,
#137214,#137215,#137216,#137217,#137218,#137219,#137220,#137221,#137222,
#137223,#137224,#137225,#137226,#137227,#137228,#137229,#137230,#137231,
#137232,#137233),.UNSPECIFIED.,.F.,.F.,(4,3,3,3,3,3,3,3,4),(0.,0.000553539642553922,
0.00083030946383088,0.000968694374469362,0.000985992488299172,0.00104653588670351,
0.00108059154830595,0.00109383541670689,0.00110707928510784),
 .UNSPECIFIED.) ;
#2096=B_SPLINE_CURVE_WITH_KNOTS('',3,(#137235,#137236,#137237,#137238,#137239,
#137240,#137241,#137242,#137243,#137244,#137245,#137246,#137247,#137248,
#137249,#137250),.UNSPECIFIED.,.F.,.F.,(4,2,2,2,2,2,2,4),(2.46381126959657E-5,
3.49307346222963E-5,0.000103812737360898,0.000147753773859885,0.000241616793832011,
0.000270869435023803,0.000448933238140248,0.00051710075735164),
 .UNSPECIFIED.) ;
#2097=B_SPLINE_CURVE_WITH_KNOTS('',3,(#137662,#137663,#137664,#137665,#137666,
#137667),.UNSPECIFIED.,.F.,.F.,(4,2,4),(1.5707963267949,2.35619449019234,
3.14159265358979),.UNSPECIFIED.) ;
#2098=B_SPLINE_CURVE_WITH_KNOTS('',3,(#137738,#137739,#137740,#137741,#137742,
#137743),.UNSPECIFIED.,.F.,.F.,(4,2,4),(0.,0.785398163397447,1.57079632679489),
 .UNSPECIFIED.) ;
#2099=B_SPLINE_CURVE_WITH_KNOTS('',3,(#137837,#137838,#137839,#137840,#137841,
#137842,#137843,#137844,#137845,#137846,#137847,#137848,#137849,#137850,
#137851,#137852,#137853,#137854,#137855),.UNSPECIFIED.,.F.,.F.,(4,3,3,3,
3,3,4),(5.85758780416038E-5,6.39772274846938E-5,8.50081925559283E-5,0.000101719137060913,
0.000115369906146282,0.000121992710600423,0.000127737589255657),
 .UNSPECIFIED.) ;
#2100=B_SPLINE_CURVE_WITH_KNOTS('',3,(#137862,#137863,#137864,#137865,#137866,
#137867,#137868,#137869,#137870,#137871,#137872,#137873,#137874,#137875),
 .UNSPECIFIED.,.F.,.F.,(4,2,2,2,2,2,4),(0.000106030898883045,0.000114450588602971,
0.000135861916063415,0.000155180925252132,0.000169070632935497,0.000187290067688046,
0.000202757041675868),.UNSPECIFIED.) ;
#2101=B_SPLINE_CURVE_WITH_KNOTS('',3,(#137876,#137877,#137878,#137879,#137880,
#137881,#137882,#137883,#137884,#137885,#137886,#137887,#137888,#137889),
 .UNSPECIFIED.,.F.,.F.,(4,2,2,2,2,2,4),(0.,1.81852425150456E-5,3.36231897823044E-5,
5.26817905679537E-5,7.36686430049931E-5,8.81407292049456E-5,9.65446177718811E-5),
 .UNSPECIFIED.) ;
#2102=B_SPLINE_CURVE_WITH_KNOTS('',3,(#137899,#137900,#137901,#137902,#137903,
#137904,#137905,#137906,#137907,#137908,#137909,#137910,#137911,#137912,
#137913,#137914,#137915,#137916,#137917),.UNSPECIFIED.,.F.,.F.,(4,3,3,3,
3,3,4),(0.,1.26126247466114E-5,2.08447799633796E-5,2.61321988210975E-5,
4.72564717703709E-5,6.3949955508106E-5,6.93621596435493E-5),
 .UNSPECIFIED.) ;
#2103=B_SPLINE_CURVE_WITH_KNOTS('',3,(#138027,#138028,#138029,#138030,#138031,
#138032,#138033,#138034,#138035,#138036,#138037,#138038),.UNSPECIFIED.,
 .F.,.F.,(4,2,2,2,2,4),(0.,0.000230913708713649,0.000346370563070478,0.000404098990248888,
0.000432963203838092,0.000461827417427297),.UNSPECIFIED.) ;
#2104=B_SPLINE_CURVE_WITH_KNOTS('',3,(#138065,#138066,#138067,#138068,#138069,
#138070,#138071,#138072,#138073,#138074,#138075,#138076),.UNSPECIFIED.,
 .F.,.F.,(4,2,2,2,2,4),(0.,2.92942635586651E-5,5.85885271173302E-5,0.00011717705423465,
0.000234354108469299,0.000468708216938598),.UNSPECIFIED.) ;
#2105=B_SPLINE_CURVE_WITH_KNOTS('',3,(#138166,#138167,#138168,#138169,#138170,
#138171,#138172,#138173,#138174,#138175,#138176,#138177),.UNSPECIFIED.,
 .F.,.F.,(4,2,2,2,2,4),(7.70621319424336E-10,0.000528455713264088,0.000792683184585472,
0.00092479692024616,0.000990853788076498,0.00105691065590684),
 .UNSPECIFIED.) ;
#2106=B_SPLINE_CURVE_WITH_KNOTS('',3,(#138178,#138179,#138180,#138181,#138182,
#138183,#138184,#138185,#138186,#138187,#138188,#138189,#138190,#138191,
#138192,#138193,#138194,#138195,#138196,#138197,#138198,#138199,#138200,
#138201,#138202,#138203,#138204,#138205),.UNSPECIFIED.,.F.,.F.,(4,2,2,2,
2,2,2,2,2,2,2,2,2,4),(0.,1.88814447163025E-5,2.66390109708352E-5,2.82246506940943E-5,
2.82548001019656E-5,4.36852952398557E-5,4.3720577757044E-5,4.63087975636134E-5,
5.19857273366473E-5,5.63013930903634E-5,5.77982263345347E-5,5.84936692674664E-5,
5.96281966878638E-5,6.07824730943714E-5),.UNSPECIFIED.) ;
#2107=B_SPLINE_CURVE_WITH_KNOTS('',3,(#138207,#138208,#138209,#138210,#138211,
#138212,#138213,#138214,#138215,#138216,#138217,#138218,#138219,#138220,
#138221,#138222,#138223,#138224,#138225,#138226,#138227,#138228),
 .UNSPECIFIED.,.F.,.F.,(4,2,2,2,2,2,2,2,2,2,4),(-2.98424671549139E-6,-1.83179854035283E-6,
-6.78494605945076E-7,0.,1.61207185756484E-6,5.98431127542434E-6,1.25056665527988E-5,
1.40350946484969E-5,2.93914218611264E-5,4.85423642724965E-5,5.82245408950303E-5),
 .UNSPECIFIED.) ;
#2108=B_SPLINE_CURVE_WITH_KNOTS('',3,(#138229,#138230,#138231,#138232,#138233,
#138234,#138235,#138236,#138237,#138238,#138239,#138240),.UNSPECIFIED.,
 .F.,.F.,(4,2,2,2,2,4),(0.,6.61189708719449E-5,0.00013223794174389,0.00026447588348779,
0.000528951766975601,0.00105790353395122),.UNSPECIFIED.) ;
#2109=B_SPLINE_CURVE_WITH_KNOTS('',3,(#138274,#138275,#138276,#138277,#138278,
#138279,#138280,#138281,#138282,#138283,#138284,#138285,#138286,#138287,
#138288,#138289,#138290,#138291,#138292,#138293,#138294,#138295,#138296,
#138297,#138298,#138299,#138300,#138301,#138302,#138303,#138304,#138305,
#138306,#138307,#138308,#138309,#138310,#138311),.UNSPECIFIED.,.F.,.F.,
(4,2,2,2,2,2,2,2,2,2,2,2,2,2,2,2,2,2,4),(4.08239077498685E-13,1.91825894886969E-5,
2.29499826201334E-5,2.74799101222721E-5,3.52358269328737E-5,4.1219865182931E-5,
4.25319315563233E-5,4.54442131892892E-5,4.69409045132602E-5,4.80898427132604E-5,
4.94464739460608E-5,4.9643274248212E-5,5.04298720437271E-5,5.14115331534997E-5,
5.17333590635563E-5,5.22889985287807E-5,5.29242843672003E-5,5.37719008581471E-5,
5.49598202435899E-5),.UNSPECIFIED.) ;
#2110=B_SPLINE_CURVE_WITH_KNOTS('',3,(#138344,#138345,#138346,#138347,#138348,
#138349,#138350,#138351,#138352,#138353,#138354,#138355,#138356,#138357,
#138358,#138359,#138360,#138361,#138362,#138363,#138364,#138365,#138366,
#138367,#138368,#138369,#138370,#138371,#138372,#138373,#138374,#138375,
#138376,#138377,#138378,#138379),.UNSPECIFIED.,.F.,.F.,(4,2,2,2,2,2,2,2,
2,2,2,2,2,2,2,2,2,4),(-2.90335387328777E-6,-1.36780202097199E-6,-6.41515161704647E-7,
-6.40610931867504E-8,3.8117330464249E-7,1.44450314269995E-6,2.24472183151459E-6,
2.50783298075742E-6,3.9666236573922E-6,5.28616271357864E-6,8.35978425016734E-6,
9.71024741498647E-6,1.08366011880722E-5,1.65505252295115E-5,2.45765562494321E-5,
2.90642498314919E-5,4.41638722245607E-5,5.20477084101079E-5),
 .UNSPECIFIED.) ;
#2111=B_SPLINE_CURVE_WITH_KNOTS('',3,(#139030,#139031,#139032,#139033,#139034,
#139035),.UNSPECIFIED.,.F.,.F.,(4,2,4),(1.5707963267949,2.35619449019234,
3.14159265358979),.UNSPECIFIED.) ;
#2112=B_SPLINE_CURVE_WITH_KNOTS('',3,(#139106,#139107,#139108,#139109,#139110,
#139111),.UNSPECIFIED.,.F.,.F.,(4,2,4),(0.,0.785398163397446,1.57079632679489),
 .UNSPECIFIED.) ;
#2113=B_SPLINE_CURVE_WITH_KNOTS('',3,(#139204,#139205,#139206,#139207,#139208,
#139209,#139210,#139211,#139212,#139213,#139214,#139215,#139216,#139217,
#139218,#139219,#139220,#139221,#139222),.UNSPECIFIED.,.F.,.F.,(4,3,3,3,
3,3,4),(5.85758780416038E-5,6.39772274846938E-5,8.5008192556256E-5,0.000101719137060913,
0.000115369906146167,0.000121992710600423,0.000127737589255657),
 .UNSPECIFIED.) ;
#2114=B_SPLINE_CURVE_WITH_KNOTS('',3,(#139229,#139230,#139231,#139232,#139233,
#139234,#139235,#139236,#139237,#139238,#139239,#139240,#139241,#139242),
 .UNSPECIFIED.,.F.,.F.,(4,2,2,2,2,2,4),(0.000106030898883045,0.000114450588602972,
0.00013586191606343,0.000155180925252192,0.000169070632935497,0.00018729006768833,
0.000202757041675869),.UNSPECIFIED.) ;
#2115=B_SPLINE_CURVE_WITH_KNOTS('',3,(#139243,#139244,#139245,#139246,#139247,
#139248,#139249,#139250,#139251,#139252,#139253,#139254,#139255,#139256),
 .UNSPECIFIED.,.F.,.F.,(4,2,2,2,2,2,4),(0.,1.81852425150232E-5,3.36231897823044E-5,
5.26817905679335E-5,7.36686430049626E-5,8.81407292049456E-5,9.65446177718811E-5),
 .UNSPECIFIED.) ;
#2116=B_SPLINE_CURVE_WITH_KNOTS('',3,(#139266,#139267,#139268,#139269,#139270,
#139271,#139272,#139273,#139274,#139275,#139276,#139277,#139278,#139279,
#139280,#139281,#139282,#139283,#139284),.UNSPECIFIED.,.F.,.F.,(4,3,3,3,
3,3,4),(0.,1.26126247466293E-5,2.08447799633812E-5,2.61321988210992E-5,
4.72564717703644E-5,6.39499555081068E-5,6.93621596435509E-5),
 .UNSPECIFIED.) ;
#2117=B_SPLINE_CURVE_WITH_KNOTS('',3,(#139394,#139395,#139396,#139397,#139398,
#139399,#139400,#139401,#139402,#139403,#139404,#139405),.UNSPECIFIED.,
 .F.,.F.,(4,2,2,2,2,4),(0.,0.000230913708713646,0.000346370563070469,0.00040409899024888,
0.000432963203838088,0.000461827417427296),.UNSPECIFIED.) ;
#2118=B_SPLINE_CURVE_WITH_KNOTS('',3,(#139426,#139427,#139428,#139429,#139430,
#139431,#139432,#139433,#139434,#139435,#139436,#139437),.UNSPECIFIED.,
 .F.,.F.,(4,2,2,2,2,4),(0.,2.92942635586651E-5,5.85885271173302E-5,0.00011717705423465,
0.000234354108469299,0.000468708216938598),.UNSPECIFIED.) ;
#2119=B_SPLINE_CURVE_WITH_KNOTS('',3,(#139506,#139507,#139508,#139509,#139510,
#139511,#139512,#139513,#139514,#139515,#139516,#139517),.UNSPECIFIED.,
 .F.,.F.,(4,2,2,2,2,4),(7.70621319424336E-10,0.000528455713264091,0.000792683184585474,
0.00092479692024616,0.000990853788076498,0.00105691065590684),
 .UNSPECIFIED.) ;
#2120=B_SPLINE_CURVE_WITH_KNOTS('',3,(#139518,#139519,#139520,#139521,#139522,
#139523,#139524,#139525,#139526,#139527,#139528,#139529,#139530,#139531,
#139532,#139533,#139534,#139535,#139536,#139537,#139538,#139539,#139540,
#139541,#139542,#139543,#139544,#139545),.UNSPECIFIED.,.F.,.F.,(4,2,2,2,
2,2,2,2,2,2,2,2,2,4),(0.,1.88814447163332E-5,2.66390109708352E-5,2.82246506940923E-5,
2.82548001019634E-5,4.36852952398549E-5,4.37205777570411E-5,4.63087975636134E-5,
5.1985727336649E-5,5.6301393090365E-5,5.77982263345347E-5,5.84936692674662E-5,
5.96281966878616E-5,6.07824730943714E-5),.UNSPECIFIED.) ;
#2121=B_SPLINE_CURVE_WITH_KNOTS('',3,(#139547,#139548,#139549,#139550,#139551,
#139552,#139553,#139554,#139555,#139556,#139557,#139558,#139559,#139560,
#139561,#139562,#139563,#139564,#139565,#139566,#139567,#139568),
 .UNSPECIFIED.,.F.,.F.,(4,2,2,2,2,2,2,2,2,2,4),(-2.98424671548978E-6,-1.83179854034966E-6,
-6.78494605943072E-7,0.,1.6120718575636E-6,5.9843112754229E-6,1.25056665528019E-5,
1.40350946485183E-5,2.93914218612042E-5,4.85423642734593E-5,5.82245408950314E-5),
 .UNSPECIFIED.) ;
#2122=B_SPLINE_CURVE_WITH_KNOTS('',3,(#139569,#139570,#139571,#139572,#139573,
#139574,#139575,#139576,#139577,#139578,#139579,#139580),.UNSPECIFIED.,
 .F.,.F.,(4,2,2,2,2,4),(0.,6.61189708719511E-5,0.000132237941743902,0.000264475883487804,
0.000528951766975613,0.00105790353395123),.UNSPECIFIED.) ;
#2123=B_SPLINE_CURVE_WITH_KNOTS('',3,(#139613,#139614,#139615,#139616,#139617,
#139618,#139619,#139620,#139621,#139622,#139623,#139624,#139625,#139626,
#139627,#139628,#139629,#139630,#139631,#139632,#139633,#139634,#139635,
#139636,#139637,#139638,#139639,#139640,#139641,#139642,#139643,#139644,
#139645,#139646,#139647,#139648,#139649,#139650),.UNSPECIFIED.,.F.,.F.,
(4,2,2,2,2,2,2,2,2,2,2,2,2,2,2,2,2,2,4),(4.08242776004549E-13,1.91825894880122E-5,
2.29499826201316E-5,2.7479910122273E-5,3.52358269328682E-5,4.1219865182932E-5,
4.25319315563182E-5,4.54442131889642E-5,4.6940904513264E-5,4.80898427132615E-5,
4.94464739459852E-5,4.96432742482264E-5,5.04298720437672E-5,5.14115331535745E-5,
5.17333590635751E-5,5.22889985288004E-5,5.2924284367221E-5,5.37719008581647E-5,
5.4959820243591E-5),.UNSPECIFIED.) ;
#2124=B_SPLINE_CURVE_WITH_KNOTS('',3,(#139681,#139682,#139683,#139684,#139685,
#139686,#139687,#139688,#139689,#139690,#139691,#139692,#139693,#139694,
#139695,#139696,#139697,#139698,#139699,#139700,#139701,#139702,#139703,
#139704,#139705,#139706,#139707,#139708,#139709,#139710,#139711,#139712,
#139713,#139714,#139715,#139716),.UNSPECIFIED.,.F.,.F.,(4,2,2,2,2,2,2,2,
2,2,2,2,2,2,2,2,2,4),(-2.90335387328777E-6,-1.36780202111177E-6,-6.41515161821873E-7,
-6.40610932957299E-8,3.81173304625258E-7,1.44450314268527E-6,2.24472183149534E-6,
2.50783298074528E-6,3.9666236573922E-6,5.28616271357869E-6,8.35978424998975E-6,
9.71024741500059E-6,1.08366011880722E-5,1.65505252295281E-5,2.45765562494321E-5,
2.90642498314901E-5,4.41638722228978E-5,5.20477084101061E-5),
 .UNSPECIFIED.) ;
#2125=B_SPLINE_CURVE_WITH_KNOTS('',3,(#139901,#139902,#139903,#139904),
 .UNSPECIFIED.,.F.,.F.,(4,4),(3.14159265358979,4.71238898038469),
 .UNSPECIFIED.) ;
#2126=B_SPLINE_CURVE_WITH_KNOTS('',3,(#139909,#139910,#139911,#139912),
 .UNSPECIFIED.,.F.,.F.,(4,4),(4.71238898038469,6.28318530717959),
 .UNSPECIFIED.) ;
#2127=B_SPLINE_CURVE_WITH_KNOTS('',3,(#140038,#140039,#140040,#140041,#140042,
#140043,#140044,#140045,#140046,#140047),.UNSPECIFIED.,.F.,.F.,(4,2,2,2,
4),(0.0155454932989836,0.0194994353522834,0.0234533774055832,0.0272081302045205,
0.0309628830034577),.UNSPECIFIED.) ;
#2128=B_SPLINE_CURVE_WITH_KNOTS('',3,(#140051,#140052,#140053,#140054,#140055,
#140056,#140057,#140058,#140059,#140060),.UNSPECIFIED.,.F.,.F.,(4,2,2,2,
4),(-0.0304888223793687,-0.0267236306519753,-0.0229584389245819,-0.0190821381960852,
-0.0152058374675885),.UNSPECIFIED.) ;
#2129=B_SPLINE_CURVE_WITH_KNOTS('',3,(#140064,#140065,#140066,#140067,#140068,
#140069,#140070,#140071,#140072,#140073),.UNSPECIFIED.,.F.,.F.,(4,2,2,2,
4),(-0.0457718072911489,-0.0418955065626522,-0.0380192058341555,-0.0342540141067621,
-0.0304888223793687),.UNSPECIFIED.) ;
#2130=B_SPLINE_CURVE_WITH_KNOTS('',3,(#140077,#140078,#140079,#140080,#140081,
#140082,#140083,#140084,#140085,#140086,#140087,#140088,#140089,#140090,
#140091,#140092,#140093,#140094,#140095,#140096,#140097,#140098,#140099,
#140100,#140101,#140102,#140103,#140104,#140105,#140106,#140107),
 .UNSPECIFIED.,.F.,.F.,(4,3,3,3,3,3,3,3,3,3,4),(0.,1.73748728562024E-5,
3.26506729531322E-5,5.028040025746E-5,6.5274122788763E-5,8.34390702564348E-5,
9.83241608049979E-5,0.000117568956567809,0.000132500510793829,0.000151525967767831,
0.000159849152172774),.UNSPECIFIED.) ;
#2131=B_SPLINE_CURVE_WITH_KNOTS('',3,(#140111,#140112,#140113,#140114,#140115,
#140116,#140117,#140118,#140119,#140120),.UNSPECIFIED.,.F.,.F.,(4,2,2,2,
4),(0.0155454932989836,0.0194994353522835,0.0234533774055833,0.0272081302045205,
0.0309628830034578),.UNSPECIFIED.) ;
#2132=B_SPLINE_CURVE_WITH_KNOTS('',3,(#140124,#140125,#140126,#140127,#140128,
#140129,#140130,#140131,#140132,#140133),.UNSPECIFIED.,.F.,.F.,(4,2,2,2,
4),(-0.0304888223793687,-0.0267236306519753,-0.022958438924582,-0.0190821381960853,
-0.0152058374675886),.UNSPECIFIED.) ;
#2133=B_SPLINE_CURVE_WITH_KNOTS('',3,(#140137,#140138,#140139,#140140,#140141,
#140142,#140143,#140144,#140145,#140146),.UNSPECIFIED.,.F.,.F.,(4,2,2,2,
4),(-0.0457718072911489,-0.0418955065626522,-0.0380192058341554,-0.0342540141067621,
-0.0304888223793687),.UNSPECIFIED.) ;
#2134=B_SPLINE_CURVE_WITH_KNOTS('',3,(#140150,#140151,#140152,#140153,#140154,
#140155,#140156,#140157,#140158,#140159,#140160,#140161,#140162,#140163,
#140164,#140165,#140166,#140167,#140168,#140169,#140170,#140171,#140172,
#140173,#140174,#140175,#140176,#140177,#140178,#140179,#140180),
 .UNSPECIFIED.,.F.,.F.,(4,3,3,3,3,3,3,3,3,3,4),(0.,1.73748728562086E-5,
3.2650672953132E-5,5.02804002574591E-5,6.52741227887635E-5,8.34390702564457E-5,
9.83241608049975E-5,0.000117568956567842,0.000132500510793829,0.000151525967767912,
0.000159849152172773),.UNSPECIFIED.) ;
#2135=B_SPLINE_CURVE_WITH_KNOTS('',3,(#140373,#140374,#140375,#140376,#140377,
#140378),.UNSPECIFIED.,.F.,.F.,(4,2,4),(3.14159265358979,3.92699081698724,
4.71238898038469),.UNSPECIFIED.) ;
#2136=B_SPLINE_CURVE_WITH_KNOTS('',3,(#140382,#140383,#140384,#140385,#140386,
#140387),.UNSPECIFIED.,.F.,.F.,(4,2,4),(3.14159265358979,3.92699081698724,
4.71238898038469),.UNSPECIFIED.) ;
#2137=B_SPLINE_CURVE_WITH_KNOTS('',3,(#140391,#140392,#140393,#140394,#140395,
#140396),.UNSPECIFIED.,.F.,.F.,(4,2,4),(4.71238898038469,5.49778714378214,
6.28318530717959),.UNSPECIFIED.) ;
#2138=B_SPLINE_CURVE_WITH_KNOTS('',3,(#140399,#140400,#140401,#140402,#140403,
#140404),.UNSPECIFIED.,.F.,.F.,(4,2,4),(4.71238898038469,5.49778714378214,
6.28318530717959),.UNSPECIFIED.) ;
#2139=B_SPLINE_CURVE_WITH_KNOTS('',3,(#140442,#140443,#140444,#140445,#140446,
#140447,#140448,#140449,#140450,#140451,#140452,#140453,#140454,#140455,
#140456,#140457,#140458,#140459,#140460,#140461,#140462,#140463,#140464,
#140465,#140466,#140467,#140468,#140469),.UNSPECIFIED.,.F.,.F.,(4,3,3,3,
3,3,3,3,3,4),(0.,0.000108662978633385,0.00021732595726677,0.000239795331094194,
0.000268321712743107,0.000359692996641291,0.000370380550777844,0.000402443213187504,
0.000469559030214583,0.000479590662188388),.UNSPECIFIED.) ;
#2140=B_SPLINE_CURVE_WITH_KNOTS('',3,(#140471,#140472,#140473,#140474,#140475,
#140476,#140477,#140478,#140479,#140480),.UNSPECIFIED.,.F.,.F.,(4,2,2,2,
4),(4.46838099282933E-15,0.000139027965256961,0.000278055930509455,0.000556111861014441,
0.00111222372202441),.UNSPECIFIED.) ;
#2141=B_SPLINE_CURVE_WITH_KNOTS('',3,(#140482,#140483,#140484,#140485,#140486,
#140487,#140488,#140489,#140490,#140491,#140492,#140493,#140494,#140495,
#140496,#140497,#140498,#140499,#140500,#140501,#140502,#140503,#140504,
#140505,#140506),.UNSPECIFIED.,.F.,.F.,(4,3,3,3,3,3,3,3,4),(0.,0.000553539642553922,
0.000830309463830885,0.000968694374469364,0.000985992488299174,0.00104653588670351,
0.00108059154830595,0.0010938354167069,0.00110707928510784),
 .UNSPECIFIED.) ;
#2142=B_SPLINE_CURVE_WITH_KNOTS('',3,(#140508,#140509,#140510,#140511,#140512,
#140513,#140514,#140515,#140516,#140517,#140518,#140519,#140520,#140521,
#140522,#140523),.UNSPECIFIED.,.F.,.F.,(4,2,2,2,2,2,2,4),(2.46381126959657E-5,
3.49307346223165E-5,0.000103812737360941,0.000147753773859885,0.000241616793832021,
0.000270869435023803,0.00044893323810819,0.00051710075735164),
 .UNSPECIFIED.) ;
#2143=B_SPLINE_CURVE_WITH_KNOTS('',3,(#140958,#140959,#140960,#140961,#140962,
#140963),.UNSPECIFIED.,.F.,.F.,(4,2,4),(1.5707963267949,2.35619449019235,
3.14159265358979),.UNSPECIFIED.) ;
#2144=B_SPLINE_CURVE_WITH_KNOTS('',3,(#141034,#141035,#141036,#141037,#141038,
#141039),.UNSPECIFIED.,.F.,.F.,(4,2,4),(0.,0.785398163397447,1.57079632679489),
 .UNSPECIFIED.) ;
#2145=B_SPLINE_CURVE_WITH_KNOTS('',3,(#141133,#141134,#141135,#141136,#141137,
#141138,#141139,#141140,#141141,#141142,#141143,#141144,#141145,#141146,
#141147,#141148,#141149,#141150,#141151),.UNSPECIFIED.,.F.,.F.,(4,3,3,3,
3,3,4),(5.85758780416056E-5,6.39772274846961E-5,8.50081925558201E-5,0.000101719137060913,
0.000115369906146294,0.000121992710600423,0.000127737589255657),
 .UNSPECIFIED.) ;
#2146=B_SPLINE_CURVE_WITH_KNOTS('',3,(#141158,#141159,#141160,#141161,#141162,
#141163,#141164,#141165,#141166,#141167,#141168,#141169,#141170,#141171),
 .UNSPECIFIED.,.F.,.F.,(4,2,2,2,2,2,4),(0.000106030898883045,0.000114450588602972,
0.000135861916063444,0.00015518092525221,0.000169070632935497,0.00018729006768838,
0.000202757041675869),.UNSPECIFIED.) ;
#2147=B_SPLINE_CURVE_WITH_KNOTS('',3,(#141172,#141173,#141174,#141175,#141176,
#141177,#141178,#141179,#141180,#141181,#141182,#141183,#141184,#141185),
 .UNSPECIFIED.,.F.,.F.,(4,2,2,2,2,2,4),(0.,1.81852425165316E-5,3.36231897823057E-5,
5.26817905682147E-5,7.36686430054364E-5,8.81407292049455E-5,9.65446177718808E-5),
 .UNSPECIFIED.) ;
#2148=B_SPLINE_CURVE_WITH_KNOTS('',3,(#141195,#141196,#141197,#141198,#141199,
#141200,#141201,#141202,#141203,#141204,#141205,#141206,#141207,#141208,
#141209,#141210,#141211,#141212,#141213),.UNSPECIFIED.,.F.,.F.,(4,3,3,3,
3,3,4),(0.,1.2612624746691E-5,2.08447799633812E-5,2.61321988210992E-5,4.72564717707153E-5,
6.39499555081056E-5,6.93621596435645E-5),.UNSPECIFIED.) ;
#2149=B_SPLINE_CURVE_WITH_KNOTS('',3,(#141323,#141324,#141325,#141326,#141327,
#141328,#141329,#141330,#141331,#141332,#141333,#141334),.UNSPECIFIED.,
 .F.,.F.,(4,2,2,2,2,4),(0.,0.000230913708713651,0.000346370563070476,0.000404098990248888,
0.000432963203838092,0.000461827417427296),.UNSPECIFIED.) ;
#2150=B_SPLINE_CURVE_WITH_KNOTS('',3,(#141359,#141360,#141361,#141362,#141363,
#141364,#141365,#141366,#141367,#141368,#141369,#141370),.UNSPECIFIED.,
 .F.,.F.,(4,2,2,2,2,4),(0.,2.92942635586625E-5,5.85885271173251E-5,0.000117177054234649,
0.000234354108469297,0.000468708216938592),.UNSPECIFIED.) ;
#2151=B_SPLINE_CURVE_WITH_KNOTS('',3,(#141454,#141455,#141456,#141457,#141458,
#141459,#141460,#141461,#141462,#141463,#141464,#141465),.UNSPECIFIED.,
 .F.,.F.,(4,2,2,2,2,4),(7.70621319424336E-10,0.000528455713264076,0.000792683184585456,
0.000924796920246147,0.000990853788076492,0.00105691065590684),
 .UNSPECIFIED.) ;
#2152=B_SPLINE_CURVE_WITH_KNOTS('',3,(#141466,#141467,#141468,#141469,#141470,
#141471,#141472,#141473,#141474,#141475,#141476,#141477,#141478,#141479,
#141480,#141481,#141482,#141483,#141484,#141485,#141486,#141487,#141488,
#141489,#141490,#141491,#141492,#141493),.UNSPECIFIED.,.F.,.F.,(4,2,2,2,
2,2,2,2,2,2,2,2,2,4),(0.,1.88814447164933E-5,2.66390109708352E-5,2.82246506940905E-5,
2.8254800101963E-5,4.36852952398535E-5,4.37205777570259E-5,4.63087975636133E-5,
5.19857273366466E-5,5.63013930903582E-5,5.77982263345344E-5,5.84936692674549E-5,
5.96281966878481E-5,6.07824730943679E-5),.UNSPECIFIED.) ;
#2153=B_SPLINE_CURVE_WITH_KNOTS('',3,(#141495,#141496,#141497,#141498,#141499,
#141500,#141501,#141502,#141503,#141504,#141505,#141506,#141507,#141508,
#141509,#141510,#141511,#141512,#141513,#141514,#141515,#141516),
 .UNSPECIFIED.,.F.,.F.,(4,2,2,2,2,2,2,2,2,2,4),(-2.98424671548817E-6,-1.8317985403492E-6,
-6.78494605942832E-7,0.,1.61207185756534E-6,5.98431127542578E-6,1.25056665528019E-5,
1.40350946485201E-5,2.93914218612042E-5,4.85423642732289E-5,5.82245408950313E-5),
 .UNSPECIFIED.) ;
#2154=B_SPLINE_CURVE_WITH_KNOTS('',3,(#141517,#141518,#141519,#141520,#141521,
#141522,#141523,#141524,#141525,#141526,#141527,#141528),.UNSPECIFIED.,
 .F.,.F.,(4,2,2,2,2,4),(0.,6.6118970871953E-5,0.000132237941743906,0.000264475883487812,
0.000528951766975618,0.00105790353395123),.UNSPECIFIED.) ;
#2155=B_SPLINE_CURVE_WITH_KNOTS('',3,(#141561,#141562,#141563,#141564,#141565,
#141566,#141567,#141568,#141569,#141570,#141571,#141572,#141573,#141574,
#141575,#141576,#141577,#141578,#141579,#141580,#141581,#141582,#141583,
#141584,#141585,#141586,#141587,#141588,#141589,#141590,#141591,#141592,
#141593,#141594,#141595,#141596,#141597,#141598),.UNSPECIFIED.,.F.,.F.,
(4,2,2,2,2,2,2,2,2,2,2,2,2,2,2,2,2,2,4),(4.08242331775179E-13,1.91825894882532E-5,
2.29499826201334E-5,2.7479910122273E-5,3.52358269328724E-5,4.1219865182932E-5,
4.25319315563226E-5,4.54442131889474E-5,4.69409045132582E-5,4.80898427132615E-5,
4.9446473946197E-5,4.96432742482032E-5,5.04298720437313E-5,5.1411533153523E-5,
5.17333590635443E-5,5.2288998528769E-5,5.29242843671897E-5,5.37719008581445E-5,
5.4959820243591E-5),.UNSPECIFIED.) ;
#2156=B_SPLINE_CURVE_WITH_KNOTS('',3,(#141631,#141632,#141633,#141634,#141635,
#141636,#141637,#141638,#141639,#141640,#141641,#141642,#141643,#141644,
#141645,#141646,#141647,#141648,#141649,#141650,#141651,#141652,#141653,
#141654,#141655,#141656,#141657,#141658,#141659,#141660,#141661,#141662,
#141663,#141664,#141665,#141666),.UNSPECIFIED.,.F.,.F.,(4,2,2,2,2,2,2,2,
2,2,2,2,2,2,2,2,2,4),(-2.90335387328765E-6,-1.36780202118156E-6,-6.41515161884124E-7,
-6.40610933545424E-8,3.81173304600826E-7,1.44450314266245E-6,2.2447218314835E-6,
2.50783298072407E-6,3.96662365739231E-6,5.28616271356407E-6,8.35978425208288E-6,
9.71024741497824E-6,1.08366011880723E-5,1.65505252295101E-5,2.45765562494322E-5,
2.90642498314973E-5,4.41638722243032E-5,5.20477084101071E-5),
 .UNSPECIFIED.) ;
#2415=CONICAL_SURFACE('',#91158,1.5,0.78539816339745) ;
#2416=CONICAL_SURFACE('',#91204,1.5,0.78539816339745) ;
#2417=CONICAL_SURFACE('',#92047,1.5,0.78539816339745) ;
#2418=CONICAL_SURFACE('',#92093,1.5,0.78539816339745) ;
#2419=CONICAL_SURFACE('',#92939,1.5,0.78539816339745) ;
#2430=LINE('',#132601,#7984) ;
#2431=LINE('',#132604,#7985) ;
#2432=LINE('',#132615,#7986) ;
#2433=LINE('',#132617,#7987) ;
#2434=LINE('',#132634,#7988) ;
#2435=LINE('',#132660,#7989) ;
#2436=LINE('',#132707,#7990) ;
#2437=LINE('',#132733,#7991) ;
#2438=LINE('',#132767,#7992) ;
#2439=LINE('',#132782,#7993) ;
#2440=LINE('',#132785,#7994) ;
#2441=LINE('',#132826,#7995) ;
#2442=LINE('',#132829,#7996) ;
#2443=LINE('',#132840,#7997) ;
#2444=LINE('',#132842,#7998) ;
#2445=LINE('',#132859,#7999) ;
#2446=LINE('',#132885,#8000) ;
#2447=LINE('',#132932,#8001) ;
#2448=LINE('',#132958,#8002) ;
#2449=LINE('',#132992,#8003) ;
#2450=LINE('',#132996,#8004) ;
#2451=LINE('',#132998,#8005) ;
#2452=LINE('',#133000,#8006) ;
#2453=LINE('',#133001,#8007) ;
#2454=LINE('',#133006,#8008) ;
#2455=LINE('',#133013,#8009) ;
#2456=LINE('',#133020,#8010) ;
#2457=LINE('',#133023,#8011) ;
#2458=LINE('',#133027,#8012) ;
#2459=LINE('',#133029,#8013) ;
#2460=LINE('',#133031,#8014) ;
#2461=LINE('',#133032,#8015) ;
#2462=LINE('',#133036,#8016) ;
#2463=LINE('',#133038,#8017) ;
#2464=LINE('',#133040,#8018) ;
#2465=LINE('',#133041,#8019) ;
#2466=LINE('',#133045,#8020) ;
#2467=LINE('',#133047,#8021) ;
#2468=LINE('',#133049,#8022) ;
#2469=LINE('',#133050,#8023) ;
#2470=LINE('',#133054,#8024) ;
#2471=LINE('',#133067,#8025) ;
#2472=LINE('',#133071,#8026) ;
#2473=LINE('',#133078,#8027) ;
#2474=LINE('',#133081,#8028) ;
#2475=LINE('',#133085,#8029) ;
#2476=LINE('',#133087,#8030) ;
#2477=LINE('',#133089,#8031) ;
#2478=LINE('',#133090,#8032) ;
#2479=LINE('',#133092,#8033) ;
#2480=LINE('',#133094,#8034) ;
#2481=LINE('',#133096,#8035) ;
#2482=LINE('',#133097,#8036) ;
#2483=LINE('',#133099,#8037) ;
#2484=LINE('',#133101,#8038) ;
#2485=LINE('',#133103,#8039) ;
#2486=LINE('',#133105,#8040) ;
#2487=LINE('',#133107,#8041) ;
#2488=LINE('',#133115,#8042) ;
#2489=LINE('',#133123,#8043) ;
#2490=LINE('',#133125,#8044) ;
#2491=LINE('',#133126,#8045) ;
#2492=LINE('',#133128,#8046) ;
#2493=LINE('',#133131,#8047) ;
#2494=LINE('',#133132,#8048) ;
#2495=LINE('',#133133,#8049) ;
#2496=LINE('',#133135,#8050) ;
#2497=LINE('',#133138,#8051) ;
#2498=LINE('',#133141,#8052) ;
#2499=LINE('',#133143,#8053) ;
#2500=LINE('',#133145,#8054) ;
#2501=LINE('',#133146,#8055) ;
#2502=LINE('',#133150,#8056) ;
#2503=LINE('',#133152,#8057) ;
#2504=LINE('',#133156,#8058) ;
#2505=LINE('',#133160,#8059) ;
#2506=LINE('',#133164,#8060) ;
#2507=LINE('',#133168,#8061) ;
#2508=LINE('',#133170,#8062) ;
#2509=LINE('',#133171,#8063) ;
#2510=LINE('',#133175,#8064) ;
#2511=LINE('',#133176,#8065) ;
#2512=LINE('',#133177,#8066) ;
#2513=LINE('',#133180,#8067) ;
#2514=LINE('',#133182,#8068) ;
#2515=LINE('',#133183,#8069) ;
#2516=LINE('',#133184,#8070) ;
#2517=LINE('',#133188,#8071) ;
#2518=LINE('',#133190,#8072) ;
#2519=LINE('',#133192,#8073) ;
#2520=LINE('',#133193,#8074) ;
#2521=LINE('',#133198,#8075) ;
#2522=LINE('',#133202,#8076) ;
#2523=LINE('',#133206,#8077) ;
#2524=LINE('',#133209,#8078) ;
#2525=LINE('',#133214,#8079) ;
#2526=LINE('',#133218,#8080) ;
#2527=LINE('',#133222,#8081) ;
#2528=LINE('',#133225,#8082) ;
#2529=LINE('',#133229,#8083) ;
#2530=LINE('',#133231,#8084) ;
#2531=LINE('',#133233,#8085) ;
#2532=LINE('',#133234,#8086) ;
#2533=LINE('',#133238,#8087) ;
#2534=LINE('',#133239,#8088) ;
#2535=LINE('',#133240,#8089) ;
#2536=LINE('',#133243,#8090) ;
#2537=LINE('',#133245,#8091) ;
#2538=LINE('',#133246,#8092) ;
#2539=LINE('',#133250,#8093) ;
#2540=LINE('',#133252,#8094) ;
#2541=LINE('',#133254,#8095) ;
#2542=LINE('',#133255,#8096) ;
#2543=LINE('',#133258,#8097) ;
#2544=LINE('',#133267,#8098) ;
#2545=LINE('',#133276,#8099) ;
#2546=LINE('',#133285,#8100) ;
#2547=LINE('',#133294,#8101) ;
#2548=LINE('',#133303,#8102) ;
#2549=LINE('',#133312,#8103) ;
#2550=LINE('',#133321,#8104) ;
#2551=LINE('',#133331,#8105) ;
#2552=LINE('',#133333,#8106) ;
#2553=LINE('',#133335,#8107) ;
#2554=LINE('',#133336,#8108) ;
#2555=LINE('',#133341,#8109) ;
#2556=LINE('',#133345,#8110) ;
#2557=LINE('',#133349,#8111) ;
#2558=LINE('',#133352,#8112) ;
#2559=LINE('',#133357,#8113) ;
#2560=LINE('',#133361,#8114) ;
#2561=LINE('',#133365,#8115) ;
#2562=LINE('',#133368,#8116) ;
#2563=LINE('',#133372,#8117) ;
#2564=LINE('',#133374,#8118) ;
#2565=LINE('',#133376,#8119) ;
#2566=LINE('',#133377,#8120) ;
#2567=LINE('',#133464,#8121) ;
#2568=LINE('',#133466,#8122) ;
#2569=LINE('',#133468,#8123) ;
#2570=LINE('',#133470,#8124) ;
#2571=LINE('',#133472,#8125) ;
#2572=LINE('',#133556,#8126) ;
#2573=LINE('',#133560,#8127) ;
#2574=LINE('',#133562,#8128) ;
#2575=LINE('',#133565,#8129) ;
#2576=LINE('',#133569,#8130) ;
#2577=LINE('',#133571,#8131) ;
#2578=LINE('',#133573,#8132) ;
#2579=LINE('',#133574,#8133) ;
#2580=LINE('',#133593,#8134) ;
#2581=LINE('',#133595,#8135) ;
#2582=LINE('',#133597,#8136) ;
#2583=LINE('',#133598,#8137) ;
#2584=LINE('',#133602,#8138) ;
#2585=LINE('',#133604,#8139) ;
#2586=LINE('',#133606,#8140) ;
#2587=LINE('',#133607,#8141) ;
#2588=LINE('',#133613,#8142) ;
#2589=LINE('',#133615,#8143) ;
#2590=LINE('',#133617,#8144) ;
#2591=LINE('',#133621,#8145) ;
#2592=LINE('',#133623,#8146) ;
#2593=LINE('',#133624,#8147) ;
#2594=LINE('',#133628,#8148) ;
#2595=LINE('',#133632,#8149) ;
#2596=LINE('',#133637,#8150) ;
#2597=LINE('',#133643,#8151) ;
#2598=LINE('',#133645,#8152) ;
#2599=LINE('',#133649,#8153) ;
#2600=LINE('',#133651,#8154) ;
#2601=LINE('',#133652,#8155) ;
#2602=LINE('',#133655,#8156) ;
#2603=LINE('',#133657,#8157) ;
#2604=LINE('',#133658,#8158) ;
#2605=LINE('',#133661,#8159) ;
#2606=LINE('',#133663,#8160) ;
#2607=LINE('',#133664,#8161) ;
#2608=LINE('',#133668,#8162) ;
#2609=LINE('',#133670,#8163) ;
#2610=LINE('',#133672,#8164) ;
#2611=LINE('',#133674,#8165) ;
#2612=LINE('',#133676,#8166) ;
#2613=LINE('',#133677,#8167) ;
#2614=LINE('',#133681,#8168) ;
#2615=LINE('',#133683,#8169) ;
#2616=LINE('',#133685,#8170) ;
#2617=LINE('',#133687,#8171) ;
#2618=LINE('',#133689,#8172) ;
#2619=LINE('',#133690,#8173) ;
#2620=LINE('',#133694,#8174) ;
#2621=LINE('',#133696,#8175) ;
#2622=LINE('',#133698,#8176) ;
#2623=LINE('',#133699,#8177) ;
#2624=LINE('',#133703,#8178) ;
#2625=LINE('',#133705,#8179) ;
#2626=LINE('',#133707,#8180) ;
#2627=LINE('',#133708,#8181) ;
#2628=LINE('',#133712,#8182) ;
#2629=LINE('',#133714,#8183) ;
#2630=LINE('',#133716,#8184) ;
#2631=LINE('',#133717,#8185) ;
#2632=LINE('',#133721,#8186) ;
#2633=LINE('',#133723,#8187) ;
#2634=LINE('',#133725,#8188) ;
#2635=LINE('',#133726,#8189) ;
#2636=LINE('',#133730,#8190) ;
#2637=LINE('',#133732,#8191) ;
#2638=LINE('',#133734,#8192) ;
#2639=LINE('',#133735,#8193) ;
#2640=LINE('',#133738,#8194) ;
#2641=LINE('',#133742,#8195) ;
#2642=LINE('',#133746,#8196) ;
#2643=LINE('',#133750,#8197) ;
#2644=LINE('',#133756,#8198) ;
#2645=LINE('',#133757,#8199) ;
#2646=LINE('',#133760,#8200) ;
#2647=LINE('',#133761,#8201) ;
#2648=LINE('',#133765,#8202) ;
#2649=LINE('',#133768,#8203) ;
#2650=LINE('',#133769,#8204) ;
#2651=LINE('',#133773,#8205) ;
#2652=LINE('',#133776,#8206) ;
#2653=LINE('',#133777,#8207) ;
#2654=LINE('',#133781,#8208) ;
#2655=LINE('',#133783,#8209) ;
#2656=LINE('',#133786,#8210) ;
#2657=LINE('',#133788,#8211) ;
#2658=LINE('',#133789,#8212) ;
#2659=LINE('',#133791,#8213) ;
#2660=LINE('',#133792,#8214) ;
#2661=LINE('',#133794,#8215) ;
#2662=LINE('',#133795,#8216) ;
#2663=LINE('',#133799,#8217) ;
#2664=LINE('',#133801,#8218) ;
#2665=LINE('',#133803,#8219) ;
#2666=LINE('',#133804,#8220) ;
#2667=LINE('',#133808,#8221) ;
#2668=LINE('',#133810,#8222) ;
#2669=LINE('',#133812,#8223) ;
#2670=LINE('',#133813,#8224) ;
#2671=LINE('',#133817,#8225) ;
#2672=LINE('',#133819,#8226) ;
#2673=LINE('',#133821,#8227) ;
#2674=LINE('',#133822,#8228) ;
#2675=LINE('',#133826,#8229) ;
#2676=LINE('',#133828,#8230) ;
#2677=LINE('',#133830,#8231) ;
#2678=LINE('',#133831,#8232) ;
#2679=LINE('',#133835,#8233) ;
#2680=LINE('',#133837,#8234) ;
#2681=LINE('',#133839,#8235) ;
#2682=LINE('',#133840,#8236) ;
#2683=LINE('',#133843,#8237) ;
#2684=LINE('',#133847,#8238) ;
#2685=LINE('',#133851,#8239) ;
#2686=LINE('',#133855,#8240) ;
#2687=LINE('',#133859,#8241) ;
#2688=LINE('',#133862,#8242) ;
#2689=LINE('',#133865,#8243) ;
#2690=LINE('',#133866,#8244) ;
#2691=LINE('',#133870,#8245) ;
#2692=LINE('',#133873,#8246) ;
#2693=LINE('',#133874,#8247) ;
#2694=LINE('',#133878,#8248) ;
#2695=LINE('',#133881,#8249) ;
#2696=LINE('',#133882,#8250) ;
#2697=LINE('',#133886,#8251) ;
#2698=LINE('',#133888,#8252) ;
#2699=LINE('',#133892,#8253) ;
#2700=LINE('',#133894,#8254) ;
#2701=LINE('',#133896,#8255) ;
#2702=LINE('',#133897,#8256) ;
#2703=LINE('',#133899,#8257) ;
#2704=LINE('',#133901,#8258) ;
#2705=LINE('',#133903,#8259) ;
#2706=LINE('',#133904,#8260) ;
#2707=LINE('',#133907,#8261) ;
#2708=LINE('',#133909,#8262) ;
#2709=LINE('',#133910,#8263) ;
#2710=LINE('',#133913,#8264) ;
#2711=LINE('',#133914,#8265) ;
#2712=LINE('',#133915,#8266) ;
#2713=LINE('',#133918,#8267) ;
#2714=LINE('',#133922,#8268) ;
#2715=LINE('',#133924,#8269) ;
#2716=LINE('',#133925,#8270) ;
#2717=LINE('',#133936,#8271) ;
#2718=LINE('',#133939,#8272) ;
#2719=LINE('',#134840,#8273) ;
#2720=LINE('',#134842,#8274) ;
#2721=LINE('',#134844,#8275) ;
#2722=LINE('',#134845,#8276) ;
#2723=LINE('',#134850,#8277) ;
#2724=LINE('',#134854,#8278) ;
#2725=LINE('',#134856,#8279) ;
#2726=LINE('',#134857,#8280) ;
#2727=LINE('',#134862,#8281) ;
#2728=LINE('',#134866,#8282) ;
#2729=LINE('',#134868,#8283) ;
#2730=LINE('',#134869,#8284) ;
#2731=LINE('',#134874,#8285) ;
#2732=LINE('',#134878,#8286) ;
#2733=LINE('',#134880,#8287) ;
#2734=LINE('',#134881,#8288) ;
#2735=LINE('',#134886,#8289) ;
#2736=LINE('',#134890,#8290) ;
#2737=LINE('',#134892,#8291) ;
#2738=LINE('',#134893,#8292) ;
#2739=LINE('',#134899,#8293) ;
#2740=LINE('',#134901,#8294) ;
#2741=LINE('',#134903,#8295) ;
#2742=LINE('',#134905,#8296) ;
#2743=LINE('',#134907,#8297) ;
#2744=LINE('',#134908,#8298) ;
#2745=LINE('',#134912,#8299) ;
#2746=LINE('',#134914,#8300) ;
#2747=LINE('',#134916,#8301) ;
#2748=LINE('',#134918,#8302) ;
#2749=LINE('',#134922,#8303) ;
#2750=LINE('',#134923,#8304) ;
#2751=LINE('',#134929,#8305) ;
#2752=LINE('',#134931,#8306) ;
#2753=LINE('',#134932,#8307) ;
#2754=LINE('',#134936,#8308) ;
#2755=LINE('',#134938,#8309) ;
#2756=LINE('',#134939,#8310) ;
#2757=LINE('',#134940,#8311) ;
#2758=LINE('',#134942,#8312) ;
#2759=LINE('',#134946,#8313) ;
#2760=LINE('',#134948,#8314) ;
#2761=LINE('',#134950,#8315) ;
#2762=LINE('',#134951,#8316) ;
#2763=LINE('',#134961,#8317) ;
#2764=LINE('',#134963,#8318) ;
#2765=LINE('',#134965,#8319) ;
#2766=LINE('',#134966,#8320) ;
#2767=LINE('',#134970,#8321) ;
#2768=LINE('',#134972,#8322) ;
#2769=LINE('',#134974,#8323) ;
#2770=LINE('',#134975,#8324) ;
#2771=LINE('',#134981,#8325) ;
#2772=LINE('',#134983,#8326) ;
#2773=LINE('',#134985,#8327) ;
#2774=LINE('',#134989,#8328) ;
#2775=LINE('',#134991,#8329) ;
#2776=LINE('',#134992,#8330) ;
#2777=LINE('',#134996,#8331) ;
#2778=LINE('',#135000,#8332) ;
#2779=LINE('',#135005,#8333) ;
#2780=LINE('',#135011,#8334) ;
#2781=LINE('',#135013,#8335) ;
#2782=LINE('',#135017,#8336) ;
#2783=LINE('',#135019,#8337) ;
#2784=LINE('',#135020,#8338) ;
#2785=LINE('',#135023,#8339) ;
#2786=LINE('',#135025,#8340) ;
#2787=LINE('',#135026,#8341) ;
#2788=LINE('',#135029,#8342) ;
#2789=LINE('',#135031,#8343) ;
#2790=LINE('',#135032,#8344) ;
#2791=LINE('',#135036,#8345) ;
#2792=LINE('',#135038,#8346) ;
#2793=LINE('',#135040,#8347) ;
#2794=LINE('',#135042,#8348) ;
#2795=LINE('',#135044,#8349) ;
#2796=LINE('',#135045,#8350) ;
#2797=LINE('',#135049,#8351) ;
#2798=LINE('',#135051,#8352) ;
#2799=LINE('',#135053,#8353) ;
#2800=LINE('',#135055,#8354) ;
#2801=LINE('',#135057,#8355) ;
#2802=LINE('',#135058,#8356) ;
#2803=LINE('',#135062,#8357) ;
#2804=LINE('',#135064,#8358) ;
#2805=LINE('',#135066,#8359) ;
#2806=LINE('',#135067,#8360) ;
#2807=LINE('',#135071,#8361) ;
#2808=LINE('',#135073,#8362) ;
#2809=LINE('',#135075,#8363) ;
#2810=LINE('',#135076,#8364) ;
#2811=LINE('',#135080,#8365) ;
#2812=LINE('',#135082,#8366) ;
#2813=LINE('',#135084,#8367) ;
#2814=LINE('',#135085,#8368) ;
#2815=LINE('',#135089,#8369) ;
#2816=LINE('',#135091,#8370) ;
#2817=LINE('',#135093,#8371) ;
#2818=LINE('',#135094,#8372) ;
#2819=LINE('',#135098,#8373) ;
#2820=LINE('',#135100,#8374) ;
#2821=LINE('',#135102,#8375) ;
#2822=LINE('',#135103,#8376) ;
#2823=LINE('',#135106,#8377) ;
#2824=LINE('',#135110,#8378) ;
#2825=LINE('',#135114,#8379) ;
#2826=LINE('',#135118,#8380) ;
#2827=LINE('',#135124,#8381) ;
#2828=LINE('',#135125,#8382) ;
#2829=LINE('',#135128,#8383) ;
#2830=LINE('',#135129,#8384) ;
#2831=LINE('',#135133,#8385) ;
#2832=LINE('',#135136,#8386) ;
#2833=LINE('',#135137,#8387) ;
#2834=LINE('',#135141,#8388) ;
#2835=LINE('',#135144,#8389) ;
#2836=LINE('',#135145,#8390) ;
#2837=LINE('',#135149,#8391) ;
#2838=LINE('',#135151,#8392) ;
#2839=LINE('',#135154,#8393) ;
#2840=LINE('',#135156,#8394) ;
#2841=LINE('',#135157,#8395) ;
#2842=LINE('',#135159,#8396) ;
#2843=LINE('',#135160,#8397) ;
#2844=LINE('',#135162,#8398) ;
#2845=LINE('',#135163,#8399) ;
#2846=LINE('',#135167,#8400) ;
#2847=LINE('',#135169,#8401) ;
#2848=LINE('',#135171,#8402) ;
#2849=LINE('',#135172,#8403) ;
#2850=LINE('',#135176,#8404) ;
#2851=LINE('',#135178,#8405) ;
#2852=LINE('',#135180,#8406) ;
#2853=LINE('',#135181,#8407) ;
#2854=LINE('',#135185,#8408) ;
#2855=LINE('',#135187,#8409) ;
#2856=LINE('',#135189,#8410) ;
#2857=LINE('',#135190,#8411) ;
#2858=LINE('',#135194,#8412) ;
#2859=LINE('',#135196,#8413) ;
#2860=LINE('',#135198,#8414) ;
#2861=LINE('',#135199,#8415) ;
#2862=LINE('',#135203,#8416) ;
#2863=LINE('',#135205,#8417) ;
#2864=LINE('',#135207,#8418) ;
#2865=LINE('',#135208,#8419) ;
#2866=LINE('',#135211,#8420) ;
#2867=LINE('',#135215,#8421) ;
#2868=LINE('',#135219,#8422) ;
#2869=LINE('',#135223,#8423) ;
#2870=LINE('',#135227,#8424) ;
#2871=LINE('',#135230,#8425) ;
#2872=LINE('',#135233,#8426) ;
#2873=LINE('',#135234,#8427) ;
#2874=LINE('',#135238,#8428) ;
#2875=LINE('',#135241,#8429) ;
#2876=LINE('',#135242,#8430) ;
#2877=LINE('',#135246,#8431) ;
#2878=LINE('',#135249,#8432) ;
#2879=LINE('',#135250,#8433) ;
#2880=LINE('',#135254,#8434) ;
#2881=LINE('',#135256,#8435) ;
#2882=LINE('',#135260,#8436) ;
#2883=LINE('',#135262,#8437) ;
#2884=LINE('',#135264,#8438) ;
#2885=LINE('',#135265,#8439) ;
#2886=LINE('',#135267,#8440) ;
#2887=LINE('',#135269,#8441) ;
#2888=LINE('',#135271,#8442) ;
#2889=LINE('',#135272,#8443) ;
#2890=LINE('',#135275,#8444) ;
#2891=LINE('',#135277,#8445) ;
#2892=LINE('',#135278,#8446) ;
#2893=LINE('',#135281,#8447) ;
#2894=LINE('',#135282,#8448) ;
#2895=LINE('',#135283,#8449) ;
#2896=LINE('',#135286,#8450) ;
#2897=LINE('',#135290,#8451) ;
#2898=LINE('',#135292,#8452) ;
#2899=LINE('',#135293,#8453) ;
#2900=LINE('',#135304,#8454) ;
#2901=LINE('',#135307,#8455) ;
#2902=LINE('',#136304,#8456) ;
#2903=LINE('',#136307,#8457) ;
#2904=LINE('',#136318,#8458) ;
#2905=LINE('',#136320,#8459) ;
#2906=LINE('',#136337,#8460) ;
#2907=LINE('',#136363,#8461) ;
#2908=LINE('',#136410,#8462) ;
#2909=LINE('',#136436,#8463) ;
#2910=LINE('',#136470,#8464) ;
#2911=LINE('',#136485,#8465) ;
#2912=LINE('',#136488,#8466) ;
#2913=LINE('',#136529,#8467) ;
#2914=LINE('',#136532,#8468) ;
#2915=LINE('',#136543,#8469) ;
#2916=LINE('',#136545,#8470) ;
#2917=LINE('',#136562,#8471) ;
#2918=LINE('',#136588,#8472) ;
#2919=LINE('',#136635,#8473) ;
#2920=LINE('',#136661,#8474) ;
#2921=LINE('',#136695,#8475) ;
#2922=LINE('',#136699,#8476) ;
#2923=LINE('',#136701,#8477) ;
#2924=LINE('',#136703,#8478) ;
#2925=LINE('',#136704,#8479) ;
#2926=LINE('',#136709,#8480) ;
#2927=LINE('',#136716,#8481) ;
#2928=LINE('',#136723,#8482) ;
#2929=LINE('',#136726,#8483) ;
#2930=LINE('',#136730,#8484) ;
#2931=LINE('',#136732,#8485) ;
#2932=LINE('',#136734,#8486) ;
#2933=LINE('',#136735,#8487) ;
#2934=LINE('',#136739,#8488) ;
#2935=LINE('',#136741,#8489) ;
#2936=LINE('',#136743,#8490) ;
#2937=LINE('',#136744,#8491) ;
#2938=LINE('',#136748,#8492) ;
#2939=LINE('',#136750,#8493) ;
#2940=LINE('',#136752,#8494) ;
#2941=LINE('',#136753,#8495) ;
#2942=LINE('',#136758,#8496) ;
#2943=LINE('',#136771,#8497) ;
#2944=LINE('',#136775,#8498) ;
#2945=LINE('',#136781,#8499) ;
#2946=LINE('',#136783,#8500) ;
#2947=LINE('',#136784,#8501) ;
#2948=LINE('',#136788,#8502) ;
#2949=LINE('',#136790,#8503) ;
#2950=LINE('',#136792,#8504) ;
#2951=LINE('',#136793,#8505) ;
#2952=LINE('',#136797,#8506) ;
#2953=LINE('',#136799,#8507) ;
#2954=LINE('',#136800,#8508) ;
#2955=LINE('',#136801,#8509) ;
#2956=LINE('',#136803,#8510) ;
#2957=LINE('',#136805,#8511) ;
#2958=LINE('',#136806,#8512) ;
#2959=LINE('',#136808,#8513) ;
#2960=LINE('',#136811,#8514) ;
#2961=LINE('',#136812,#8515) ;
#2962=LINE('',#136814,#8516) ;
#2963=LINE('',#136816,#8517) ;
#2964=LINE('',#136818,#8518) ;
#2965=LINE('',#136826,#8519) ;
#2966=LINE('',#136834,#8520) ;
#2967=LINE('',#136836,#8521) ;
#2968=LINE('',#136837,#8522) ;
#2969=LINE('',#136839,#8523) ;
#2970=LINE('',#136842,#8524) ;
#2971=LINE('',#136845,#8525) ;
#2972=LINE('',#136847,#8526) ;
#2973=LINE('',#136848,#8527) ;
#2974=LINE('',#136849,#8528) ;
#2975=LINE('',#136853,#8529) ;
#2976=LINE('',#136855,#8530) ;
#2977=LINE('',#136857,#8531) ;
#2978=LINE('',#136861,#8532) ;
#2979=LINE('',#136865,#8533) ;
#2980=LINE('',#136869,#8534) ;
#2981=LINE('',#136873,#8535) ;
#2982=LINE('',#136874,#8536) ;
#2983=LINE('',#136877,#8537) ;
#2984=LINE('',#136879,#8538) ;
#2985=LINE('',#136880,#8539) ;
#2986=LINE('',#136883,#8540) ;
#2987=LINE('',#136885,#8541) ;
#2988=LINE('',#136886,#8542) ;
#2989=LINE('',#136887,#8543) ;
#2990=LINE('',#136891,#8544) ;
#2991=LINE('',#136893,#8545) ;
#2992=LINE('',#136895,#8546) ;
#2993=LINE('',#136896,#8547) ;
#2994=LINE('',#136901,#8548) ;
#2995=LINE('',#136905,#8549) ;
#2996=LINE('',#136909,#8550) ;
#2997=LINE('',#136912,#8551) ;
#2998=LINE('',#136917,#8552) ;
#2999=LINE('',#136921,#8553) ;
#3000=LINE('',#136925,#8554) ;
#3001=LINE('',#136928,#8555) ;
#3002=LINE('',#136932,#8556) ;
#3003=LINE('',#136934,#8557) ;
#3004=LINE('',#136936,#8558) ;
#3005=LINE('',#136937,#8559) ;
#3006=LINE('',#136940,#8560) ;
#3007=LINE('',#136942,#8561) ;
#3008=LINE('',#136943,#8562) ;
#3009=LINE('',#136946,#8563) ;
#3010=LINE('',#136948,#8564) ;
#3011=LINE('',#136949,#8565) ;
#3012=LINE('',#136953,#8566) ;
#3013=LINE('',#136955,#8567) ;
#3014=LINE('',#136957,#8568) ;
#3015=LINE('',#136958,#8569) ;
#3016=LINE('',#136961,#8570) ;
#3017=LINE('',#136970,#8571) ;
#3018=LINE('',#136979,#8572) ;
#3019=LINE('',#136988,#8573) ;
#3020=LINE('',#136997,#8574) ;
#3021=LINE('',#137006,#8575) ;
#3022=LINE('',#137015,#8576) ;
#3023=LINE('',#137024,#8577) ;
#3024=LINE('',#137034,#8578) ;
#3025=LINE('',#137036,#8579) ;
#3026=LINE('',#137038,#8580) ;
#3027=LINE('',#137039,#8581) ;
#3028=LINE('',#137044,#8582) ;
#3029=LINE('',#137048,#8583) ;
#3030=LINE('',#137052,#8584) ;
#3031=LINE('',#137055,#8585) ;
#3032=LINE('',#137060,#8586) ;
#3033=LINE('',#137064,#8587) ;
#3034=LINE('',#137068,#8588) ;
#3035=LINE('',#137071,#8589) ;
#3036=LINE('',#137075,#8590) ;
#3037=LINE('',#137077,#8591) ;
#3038=LINE('',#137079,#8592) ;
#3039=LINE('',#137080,#8593) ;
#3040=LINE('',#137167,#8594) ;
#3041=LINE('',#137252,#8595) ;
#3042=LINE('',#137254,#8596) ;
#3043=LINE('',#137256,#8597) ;
#3044=LINE('',#137258,#8598) ;
#3045=LINE('',#137259,#8599) ;
#3046=LINE('',#137263,#8600) ;
#3047=LINE('',#137267,#8601) ;
#3048=LINE('',#137272,#8602) ;
#3049=LINE('',#137274,#8603) ;
#3050=LINE('',#137276,#8604) ;
#3051=LINE('',#137277,#8605) ;
#3052=LINE('',#137296,#8606) ;
#3053=LINE('',#137298,#8607) ;
#3054=LINE('',#137300,#8608) ;
#3055=LINE('',#137301,#8609) ;
#3056=LINE('',#137305,#8610) ;
#3057=LINE('',#137307,#8611) ;
#3058=LINE('',#137309,#8612) ;
#3059=LINE('',#137310,#8613) ;
#3060=LINE('',#137316,#8614) ;
#3061=LINE('',#137318,#8615) ;
#3062=LINE('',#137320,#8616) ;
#3063=LINE('',#137324,#8617) ;
#3064=LINE('',#137326,#8618) ;
#3065=LINE('',#137327,#8619) ;
#3066=LINE('',#137331,#8620) ;
#3067=LINE('',#137335,#8621) ;
#3068=LINE('',#137340,#8622) ;
#3069=LINE('',#137346,#8623) ;
#3070=LINE('',#137348,#8624) ;
#3071=LINE('',#137352,#8625) ;
#3072=LINE('',#137354,#8626) ;
#3073=LINE('',#137355,#8627) ;
#3074=LINE('',#137358,#8628) ;
#3075=LINE('',#137360,#8629) ;
#3076=LINE('',#137361,#8630) ;
#3077=LINE('',#137364,#8631) ;
#3078=LINE('',#137366,#8632) ;
#3079=LINE('',#137367,#8633) ;
#3080=LINE('',#137371,#8634) ;
#3081=LINE('',#137373,#8635) ;
#3082=LINE('',#137375,#8636) ;
#3083=LINE('',#137377,#8637) ;
#3084=LINE('',#137379,#8638) ;
#3085=LINE('',#137380,#8639) ;
#3086=LINE('',#137384,#8640) ;
#3087=LINE('',#137386,#8641) ;
#3088=LINE('',#137388,#8642) ;
#3089=LINE('',#137390,#8643) ;
#3090=LINE('',#137392,#8644) ;
#3091=LINE('',#137393,#8645) ;
#3092=LINE('',#137397,#8646) ;
#3093=LINE('',#137399,#8647) ;
#3094=LINE('',#137401,#8648) ;
#3095=LINE('',#137402,#8649) ;
#3096=LINE('',#137406,#8650) ;
#3097=LINE('',#137408,#8651) ;
#3098=LINE('',#137410,#8652) ;
#3099=LINE('',#137411,#8653) ;
#3100=LINE('',#137415,#8654) ;
#3101=LINE('',#137417,#8655) ;
#3102=LINE('',#137419,#8656) ;
#3103=LINE('',#137420,#8657) ;
#3104=LINE('',#137424,#8658) ;
#3105=LINE('',#137426,#8659) ;
#3106=LINE('',#137428,#8660) ;
#3107=LINE('',#137429,#8661) ;
#3108=LINE('',#137433,#8662) ;
#3109=LINE('',#137435,#8663) ;
#3110=LINE('',#137437,#8664) ;
#3111=LINE('',#137438,#8665) ;
#3112=LINE('',#137441,#8666) ;
#3113=LINE('',#137445,#8667) ;
#3114=LINE('',#137449,#8668) ;
#3115=LINE('',#137453,#8669) ;
#3116=LINE('',#137459,#8670) ;
#3117=LINE('',#137460,#8671) ;
#3118=LINE('',#137463,#8672) ;
#3119=LINE('',#137464,#8673) ;
#3120=LINE('',#137468,#8674) ;
#3121=LINE('',#137471,#8675) ;
#3122=LINE('',#137472,#8676) ;
#3123=LINE('',#137476,#8677) ;
#3124=LINE('',#137479,#8678) ;
#3125=LINE('',#137480,#8679) ;
#3126=LINE('',#137484,#8680) ;
#3127=LINE('',#137486,#8681) ;
#3128=LINE('',#137489,#8682) ;
#3129=LINE('',#137491,#8683) ;
#3130=LINE('',#137492,#8684) ;
#3131=LINE('',#137494,#8685) ;
#3132=LINE('',#137495,#8686) ;
#3133=LINE('',#137497,#8687) ;
#3134=LINE('',#137498,#8688) ;
#3135=LINE('',#137502,#8689) ;
#3136=LINE('',#137504,#8690) ;
#3137=LINE('',#137506,#8691) ;
#3138=LINE('',#137507,#8692) ;
#3139=LINE('',#137511,#8693) ;
#3140=LINE('',#137513,#8694) ;
#3141=LINE('',#137515,#8695) ;
#3142=LINE('',#137516,#8696) ;
#3143=LINE('',#137520,#8697) ;
#3144=LINE('',#137522,#8698) ;
#3145=LINE('',#137524,#8699) ;
#3146=LINE('',#137525,#8700) ;
#3147=LINE('',#137529,#8701) ;
#3148=LINE('',#137531,#8702) ;
#3149=LINE('',#137533,#8703) ;
#3150=LINE('',#137534,#8704) ;
#3151=LINE('',#137538,#8705) ;
#3152=LINE('',#137540,#8706) ;
#3153=LINE('',#137542,#8707) ;
#3154=LINE('',#137543,#8708) ;
#3155=LINE('',#137546,#8709) ;
#3156=LINE('',#137550,#8710) ;
#3157=LINE('',#137554,#8711) ;
#3158=LINE('',#137558,#8712) ;
#3159=LINE('',#137562,#8713) ;
#3160=LINE('',#137565,#8714) ;
#3161=LINE('',#137568,#8715) ;
#3162=LINE('',#137569,#8716) ;
#3163=LINE('',#137573,#8717) ;
#3164=LINE('',#137576,#8718) ;
#3165=LINE('',#137577,#8719) ;
#3166=LINE('',#137581,#8720) ;
#3167=LINE('',#137584,#8721) ;
#3168=LINE('',#137585,#8722) ;
#3169=LINE('',#137589,#8723) ;
#3170=LINE('',#137591,#8724) ;
#3171=LINE('',#137595,#8725) ;
#3172=LINE('',#137597,#8726) ;
#3173=LINE('',#137599,#8727) ;
#3174=LINE('',#137600,#8728) ;
#3175=LINE('',#137602,#8729) ;
#3176=LINE('',#137604,#8730) ;
#3177=LINE('',#137606,#8731) ;
#3178=LINE('',#137607,#8732) ;
#3179=LINE('',#137610,#8733) ;
#3180=LINE('',#137612,#8734) ;
#3181=LINE('',#137613,#8735) ;
#3182=LINE('',#137616,#8736) ;
#3183=LINE('',#137617,#8737) ;
#3184=LINE('',#137618,#8738) ;
#3185=LINE('',#137621,#8739) ;
#3186=LINE('',#137625,#8740) ;
#3187=LINE('',#137627,#8741) ;
#3188=LINE('',#137628,#8742) ;
#3189=LINE('',#137639,#8743) ;
#3190=LINE('',#137642,#8744) ;
#3191=LINE('',#138543,#8745) ;
#3192=LINE('',#138545,#8746) ;
#3193=LINE('',#138547,#8747) ;
#3194=LINE('',#138548,#8748) ;
#3195=LINE('',#138553,#8749) ;
#3196=LINE('',#138557,#8750) ;
#3197=LINE('',#138559,#8751) ;
#3198=LINE('',#138560,#8752) ;
#3199=LINE('',#138565,#8753) ;
#3200=LINE('',#138569,#8754) ;
#3201=LINE('',#138571,#8755) ;
#3202=LINE('',#138572,#8756) ;
#3203=LINE('',#138577,#8757) ;
#3204=LINE('',#138581,#8758) ;
#3205=LINE('',#138583,#8759) ;
#3206=LINE('',#138584,#8760) ;
#3207=LINE('',#138589,#8761) ;
#3208=LINE('',#138593,#8762) ;
#3209=LINE('',#138595,#8763) ;
#3210=LINE('',#138596,#8764) ;
#3211=LINE('',#138602,#8765) ;
#3212=LINE('',#138604,#8766) ;
#3213=LINE('',#138606,#8767) ;
#3214=LINE('',#138608,#8768) ;
#3215=LINE('',#138610,#8769) ;
#3216=LINE('',#138611,#8770) ;
#3217=LINE('',#138615,#8771) ;
#3218=LINE('',#138617,#8772) ;
#3219=LINE('',#138619,#8773) ;
#3220=LINE('',#138621,#8774) ;
#3221=LINE('',#138625,#8775) ;
#3222=LINE('',#138626,#8776) ;
#3223=LINE('',#138630,#8777) ;
#3224=LINE('',#138632,#8778) ;
#3225=LINE('',#138634,#8779) ;
#3226=LINE('',#138635,#8780) ;
#3227=LINE('',#138637,#8781) ;
#3228=LINE('',#138640,#8782) ;
#3229=LINE('',#138642,#8783) ;
#3230=LINE('',#138644,#8784) ;
#3231=LINE('',#138645,#8785) ;
#3232=LINE('',#138649,#8786) ;
#3233=LINE('',#138651,#8787) ;
#3234=LINE('',#138654,#8788) ;
#3235=LINE('',#138664,#8789) ;
#3236=LINE('',#138666,#8790) ;
#3237=LINE('',#138668,#8791) ;
#3238=LINE('',#138669,#8792) ;
#3239=LINE('',#138673,#8793) ;
#3240=LINE('',#138675,#8794) ;
#3241=LINE('',#138677,#8795) ;
#3242=LINE('',#138678,#8796) ;
#3243=LINE('',#138684,#8797) ;
#3244=LINE('',#138686,#8798) ;
#3245=LINE('',#138688,#8799) ;
#3246=LINE('',#138692,#8800) ;
#3247=LINE('',#138694,#8801) ;
#3248=LINE('',#138695,#8802) ;
#3249=LINE('',#138699,#8803) ;
#3250=LINE('',#138703,#8804) ;
#3251=LINE('',#138708,#8805) ;
#3252=LINE('',#138714,#8806) ;
#3253=LINE('',#138716,#8807) ;
#3254=LINE('',#138720,#8808) ;
#3255=LINE('',#138722,#8809) ;
#3256=LINE('',#138723,#8810) ;
#3257=LINE('',#138726,#8811) ;
#3258=LINE('',#138728,#8812) ;
#3259=LINE('',#138729,#8813) ;
#3260=LINE('',#138732,#8814) ;
#3261=LINE('',#138734,#8815) ;
#3262=LINE('',#138735,#8816) ;
#3263=LINE('',#138739,#8817) ;
#3264=LINE('',#138741,#8818) ;
#3265=LINE('',#138743,#8819) ;
#3266=LINE('',#138745,#8820) ;
#3267=LINE('',#138747,#8821) ;
#3268=LINE('',#138748,#8822) ;
#3269=LINE('',#138752,#8823) ;
#3270=LINE('',#138754,#8824) ;
#3271=LINE('',#138756,#8825) ;
#3272=LINE('',#138758,#8826) ;
#3273=LINE('',#138760,#8827) ;
#3274=LINE('',#138761,#8828) ;
#3275=LINE('',#138765,#8829) ;
#3276=LINE('',#138767,#8830) ;
#3277=LINE('',#138769,#8831) ;
#3278=LINE('',#138770,#8832) ;
#3279=LINE('',#138774,#8833) ;
#3280=LINE('',#138776,#8834) ;
#3281=LINE('',#138778,#8835) ;
#3282=LINE('',#138779,#8836) ;
#3283=LINE('',#138783,#8837) ;
#3284=LINE('',#138785,#8838) ;
#3285=LINE('',#138787,#8839) ;
#3286=LINE('',#138788,#8840) ;
#3287=LINE('',#138792,#8841) ;
#3288=LINE('',#138794,#8842) ;
#3289=LINE('',#138796,#8843) ;
#3290=LINE('',#138797,#8844) ;
#3291=LINE('',#138801,#8845) ;
#3292=LINE('',#138803,#8846) ;
#3293=LINE('',#138805,#8847) ;
#3294=LINE('',#138806,#8848) ;
#3295=LINE('',#138809,#8849) ;
#3296=LINE('',#138813,#8850) ;
#3297=LINE('',#138817,#8851) ;
#3298=LINE('',#138821,#8852) ;
#3299=LINE('',#138827,#8853) ;
#3300=LINE('',#138828,#8854) ;
#3301=LINE('',#138831,#8855) ;
#3302=LINE('',#138832,#8856) ;
#3303=LINE('',#138836,#8857) ;
#3304=LINE('',#138839,#8858) ;
#3305=LINE('',#138840,#8859) ;
#3306=LINE('',#138844,#8860) ;
#3307=LINE('',#138847,#8861) ;
#3308=LINE('',#138848,#8862) ;
#3309=LINE('',#138852,#8863) ;
#3310=LINE('',#138854,#8864) ;
#3311=LINE('',#138857,#8865) ;
#3312=LINE('',#138859,#8866) ;
#3313=LINE('',#138860,#8867) ;
#3314=LINE('',#138862,#8868) ;
#3315=LINE('',#138863,#8869) ;
#3316=LINE('',#138865,#8870) ;
#3317=LINE('',#138866,#8871) ;
#3318=LINE('',#138870,#8872) ;
#3319=LINE('',#138872,#8873) ;
#3320=LINE('',#138874,#8874) ;
#3321=LINE('',#138875,#8875) ;
#3322=LINE('',#138879,#8876) ;
#3323=LINE('',#138881,#8877) ;
#3324=LINE('',#138883,#8878) ;
#3325=LINE('',#138884,#8879) ;
#3326=LINE('',#138888,#8880) ;
#3327=LINE('',#138890,#8881) ;
#3328=LINE('',#138892,#8882) ;
#3329=LINE('',#138893,#8883) ;
#3330=LINE('',#138897,#8884) ;
#3331=LINE('',#138899,#8885) ;
#3332=LINE('',#138901,#8886) ;
#3333=LINE('',#138902,#8887) ;
#3334=LINE('',#138906,#8888) ;
#3335=LINE('',#138908,#8889) ;
#3336=LINE('',#138910,#8890) ;
#3337=LINE('',#138911,#8891) ;
#3338=LINE('',#138914,#8892) ;
#3339=LINE('',#138918,#8893) ;
#3340=LINE('',#138922,#8894) ;
#3341=LINE('',#138926,#8895) ;
#3342=LINE('',#138930,#8896) ;
#3343=LINE('',#138933,#8897) ;
#3344=LINE('',#138936,#8898) ;
#3345=LINE('',#138937,#8899) ;
#3346=LINE('',#138941,#8900) ;
#3347=LINE('',#138944,#8901) ;
#3348=LINE('',#138945,#8902) ;
#3349=LINE('',#138949,#8903) ;
#3350=LINE('',#138952,#8904) ;
#3351=LINE('',#138953,#8905) ;
#3352=LINE('',#138957,#8906) ;
#3353=LINE('',#138959,#8907) ;
#3354=LINE('',#138963,#8908) ;
#3355=LINE('',#138965,#8909) ;
#3356=LINE('',#138967,#8910) ;
#3357=LINE('',#138968,#8911) ;
#3358=LINE('',#138970,#8912) ;
#3359=LINE('',#138972,#8913) ;
#3360=LINE('',#138974,#8914) ;
#3361=LINE('',#138975,#8915) ;
#3362=LINE('',#138978,#8916) ;
#3363=LINE('',#138980,#8917) ;
#3364=LINE('',#138981,#8918) ;
#3365=LINE('',#138984,#8919) ;
#3366=LINE('',#138985,#8920) ;
#3367=LINE('',#138986,#8921) ;
#3368=LINE('',#138989,#8922) ;
#3369=LINE('',#138993,#8923) ;
#3370=LINE('',#138995,#8924) ;
#3371=LINE('',#138996,#8925) ;
#3372=LINE('',#139007,#8926) ;
#3373=LINE('',#139010,#8927) ;
#3374=LINE('',#139972,#8928) ;
#3375=LINE('',#139975,#8929) ;
#3376=LINE('',#140016,#8930) ;
#3377=LINE('',#140019,#8931) ;
#3378=LINE('',#140030,#8932) ;
#3379=LINE('',#140032,#8933) ;
#3380=LINE('',#140049,#8934) ;
#3381=LINE('',#140075,#8935) ;
#3382=LINE('',#140122,#8936) ;
#3383=LINE('',#140148,#8937) ;
#3384=LINE('',#140182,#8938) ;
#3385=LINE('',#140188,#8939) ;
#3386=LINE('',#140190,#8940) ;
#3387=LINE('',#140191,#8941) ;
#3388=LINE('',#140195,#8942) ;
#3389=LINE('',#140197,#8943) ;
#3390=LINE('',#140199,#8944) ;
#3391=LINE('',#140200,#8945) ;
#3392=LINE('',#140204,#8946) ;
#3393=LINE('',#140206,#8947) ;
#3394=LINE('',#140207,#8948) ;
#3395=LINE('',#140208,#8949) ;
#3396=LINE('',#140210,#8950) ;
#3397=LINE('',#140212,#8951) ;
#3398=LINE('',#140214,#8952) ;
#3399=LINE('',#140216,#8953) ;
#3400=LINE('',#140218,#8954) ;
#3401=LINE('',#140226,#8955) ;
#3402=LINE('',#140228,#8956) ;
#3403=LINE('',#140229,#8957) ;
#3404=LINE('',#140231,#8958) ;
#3405=LINE('',#140234,#8959) ;
#3406=LINE('',#140237,#8960) ;
#3407=LINE('',#140239,#8961) ;
#3408=LINE('',#140241,#8962) ;
#3409=LINE('',#140242,#8963) ;
#3410=LINE('',#140246,#8964) ;
#3411=LINE('',#140248,#8965) ;
#3412=LINE('',#140252,#8966) ;
#3413=LINE('',#140256,#8967) ;
#3414=LINE('',#140258,#8968) ;
#3415=LINE('',#140259,#8969) ;
#3416=LINE('',#140263,#8970) ;
#3417=LINE('',#140265,#8971) ;
#3418=LINE('',#140267,#8972) ;
#3419=LINE('',#140268,#8973) ;
#3420=LINE('',#140272,#8974) ;
#3421=LINE('',#140274,#8975) ;
#3422=LINE('',#140276,#8976) ;
#3423=LINE('',#140277,#8977) ;
#3424=LINE('',#140281,#8978) ;
#3425=LINE('',#140283,#8979) ;
#3426=LINE('',#140285,#8980) ;
#3427=LINE('',#140286,#8981) ;
#3428=LINE('',#140290,#8982) ;
#3429=LINE('',#140292,#8983) ;
#3430=LINE('',#140294,#8984) ;
#3431=LINE('',#140295,#8985) ;
#3432=LINE('',#140299,#8986) ;
#3433=LINE('',#140301,#8987) ;
#3434=LINE('',#140303,#8988) ;
#3435=LINE('',#140304,#8989) ;
#3436=LINE('',#140308,#8990) ;
#3437=LINE('',#140310,#8991) ;
#3438=LINE('',#140312,#8992) ;
#3439=LINE('',#140313,#8993) ;
#3440=LINE('',#140317,#8994) ;
#3441=LINE('',#140319,#8995) ;
#3442=LINE('',#140321,#8996) ;
#3443=LINE('',#140322,#8997) ;
#3444=LINE('',#140327,#8998) ;
#3445=LINE('',#140331,#8999) ;
#3446=LINE('',#140335,#9000) ;
#3447=LINE('',#140338,#9001) ;
#3448=LINE('',#140342,#9002) ;
#3449=LINE('',#140344,#9003) ;
#3450=LINE('',#140346,#9004) ;
#3451=LINE('',#140347,#9005) ;
#3452=LINE('',#140350,#9006) ;
#3453=LINE('',#140352,#9007) ;
#3454=LINE('',#140353,#9008) ;
#3455=LINE('',#140356,#9009) ;
#3456=LINE('',#140358,#9010) ;
#3457=LINE('',#140359,#9011) ;
#3458=LINE('',#140363,#9012) ;
#3459=LINE('',#140365,#9013) ;
#3460=LINE('',#140367,#9014) ;
#3461=LINE('',#140368,#9015) ;
#3462=LINE('',#140371,#9016) ;
#3463=LINE('',#140380,#9017) ;
#3464=LINE('',#140389,#9018) ;
#3465=LINE('',#140398,#9019) ;
#3466=LINE('',#140408,#9020) ;
#3467=LINE('',#140410,#9021) ;
#3468=LINE('',#140412,#9022) ;
#3469=LINE('',#140413,#9023) ;
#3470=LINE('',#140418,#9024) ;
#3471=LINE('',#140422,#9025) ;
#3472=LINE('',#140426,#9026) ;
#3473=LINE('',#140429,#9027) ;
#3474=LINE('',#140433,#9028) ;
#3475=LINE('',#140435,#9029) ;
#3476=LINE('',#140437,#9030) ;
#3477=LINE('',#140438,#9031) ;
#3478=LINE('',#140525,#9032) ;
#3479=LINE('',#140527,#9033) ;
#3480=LINE('',#140529,#9034) ;
#3481=LINE('',#140531,#9035) ;
#3482=LINE('',#140532,#9036) ;
#3483=LINE('',#140536,#9037) ;
#3484=LINE('',#140538,#9038) ;
#3485=LINE('',#140541,#9039) ;
#3486=LINE('',#140545,#9040) ;
#3487=LINE('',#140547,#9041) ;
#3488=LINE('',#140549,#9042) ;
#3489=LINE('',#140550,#9043) ;
#3490=LINE('',#140592,#9044) ;
#3491=LINE('',#140594,#9045) ;
#3492=LINE('',#140596,#9046) ;
#3493=LINE('',#140597,#9047) ;
#3494=LINE('',#140601,#9048) ;
#3495=LINE('',#140603,#9049) ;
#3496=LINE('',#140605,#9050) ;
#3497=LINE('',#140606,#9051) ;
#3498=LINE('',#140612,#9052) ;
#3499=LINE('',#140614,#9053) ;
#3500=LINE('',#140616,#9054) ;
#3501=LINE('',#140620,#9055) ;
#3502=LINE('',#140622,#9056) ;
#3503=LINE('',#140623,#9057) ;
#3504=LINE('',#140627,#9058) ;
#3505=LINE('',#140631,#9059) ;
#3506=LINE('',#140636,#9060) ;
#3507=LINE('',#140642,#9061) ;
#3508=LINE('',#140644,#9062) ;
#3509=LINE('',#140648,#9063) ;
#3510=LINE('',#140650,#9064) ;
#3511=LINE('',#140651,#9065) ;
#3512=LINE('',#140654,#9066) ;
#3513=LINE('',#140656,#9067) ;
#3514=LINE('',#140657,#9068) ;
#3515=LINE('',#140660,#9069) ;
#3516=LINE('',#140662,#9070) ;
#3517=LINE('',#140663,#9071) ;
#3518=LINE('',#140667,#9072) ;
#3519=LINE('',#140669,#9073) ;
#3520=LINE('',#140671,#9074) ;
#3521=LINE('',#140673,#9075) ;
#3522=LINE('',#140675,#9076) ;
#3523=LINE('',#140676,#9077) ;
#3524=LINE('',#140680,#9078) ;
#3525=LINE('',#140682,#9079) ;
#3526=LINE('',#140684,#9080) ;
#3527=LINE('',#140686,#9081) ;
#3528=LINE('',#140688,#9082) ;
#3529=LINE('',#140689,#9083) ;
#3530=LINE('',#140693,#9084) ;
#3531=LINE('',#140695,#9085) ;
#3532=LINE('',#140697,#9086) ;
#3533=LINE('',#140698,#9087) ;
#3534=LINE('',#140702,#9088) ;
#3535=LINE('',#140704,#9089) ;
#3536=LINE('',#140706,#9090) ;
#3537=LINE('',#140707,#9091) ;
#3538=LINE('',#140711,#9092) ;
#3539=LINE('',#140713,#9093) ;
#3540=LINE('',#140715,#9094) ;
#3541=LINE('',#140716,#9095) ;
#3542=LINE('',#140720,#9096) ;
#3543=LINE('',#140722,#9097) ;
#3544=LINE('',#140724,#9098) ;
#3545=LINE('',#140725,#9099) ;
#3546=LINE('',#140729,#9100) ;
#3547=LINE('',#140731,#9101) ;
#3548=LINE('',#140733,#9102) ;
#3549=LINE('',#140734,#9103) ;
#3550=LINE('',#140737,#9104) ;
#3551=LINE('',#140741,#9105) ;
#3552=LINE('',#140745,#9106) ;
#3553=LINE('',#140749,#9107) ;
#3554=LINE('',#140755,#9108) ;
#3555=LINE('',#140756,#9109) ;
#3556=LINE('',#140759,#9110) ;
#3557=LINE('',#140760,#9111) ;
#3558=LINE('',#140764,#9112) ;
#3559=LINE('',#140767,#9113) ;
#3560=LINE('',#140768,#9114) ;
#3561=LINE('',#140772,#9115) ;
#3562=LINE('',#140775,#9116) ;
#3563=LINE('',#140776,#9117) ;
#3564=LINE('',#140780,#9118) ;
#3565=LINE('',#140782,#9119) ;
#3566=LINE('',#140785,#9120) ;
#3567=LINE('',#140787,#9121) ;
#3568=LINE('',#140788,#9122) ;
#3569=LINE('',#140790,#9123) ;
#3570=LINE('',#140791,#9124) ;
#3571=LINE('',#140793,#9125) ;
#3572=LINE('',#140794,#9126) ;
#3573=LINE('',#140798,#9127) ;
#3574=LINE('',#140800,#9128) ;
#3575=LINE('',#140802,#9129) ;
#3576=LINE('',#140803,#9130) ;
#3577=LINE('',#140807,#9131) ;
#3578=LINE('',#140809,#9132) ;
#3579=LINE('',#140811,#9133) ;
#3580=LINE('',#140812,#9134) ;
#3581=LINE('',#140816,#9135) ;
#3582=LINE('',#140818,#9136) ;
#3583=LINE('',#140820,#9137) ;
#3584=LINE('',#140821,#9138) ;
#3585=LINE('',#140825,#9139) ;
#3586=LINE('',#140827,#9140) ;
#3587=LINE('',#140829,#9141) ;
#3588=LINE('',#140830,#9142) ;
#3589=LINE('',#140834,#9143) ;
#3590=LINE('',#140836,#9144) ;
#3591=LINE('',#140838,#9145) ;
#3592=LINE('',#140839,#9146) ;
#3593=LINE('',#140842,#9147) ;
#3594=LINE('',#140846,#9148) ;
#3595=LINE('',#140850,#9149) ;
#3596=LINE('',#140854,#9150) ;
#3597=LINE('',#140858,#9151) ;
#3598=LINE('',#140861,#9152) ;
#3599=LINE('',#140864,#9153) ;
#3600=LINE('',#140865,#9154) ;
#3601=LINE('',#140869,#9155) ;
#3602=LINE('',#140872,#9156) ;
#3603=LINE('',#140873,#9157) ;
#3604=LINE('',#140877,#9158) ;
#3605=LINE('',#140880,#9159) ;
#3606=LINE('',#140881,#9160) ;
#3607=LINE('',#140885,#9161) ;
#3608=LINE('',#140887,#9162) ;
#3609=LINE('',#140891,#9163) ;
#3610=LINE('',#140893,#9164) ;
#3611=LINE('',#140895,#9165) ;
#3612=LINE('',#140896,#9166) ;
#3613=LINE('',#140898,#9167) ;
#3614=LINE('',#140900,#9168) ;
#3615=LINE('',#140902,#9169) ;
#3616=LINE('',#140903,#9170) ;
#3617=LINE('',#140906,#9171) ;
#3618=LINE('',#140908,#9172) ;
#3619=LINE('',#140909,#9173) ;
#3620=LINE('',#140912,#9174) ;
#3621=LINE('',#140913,#9175) ;
#3622=LINE('',#140914,#9176) ;
#3623=LINE('',#140917,#9177) ;
#3624=LINE('',#140921,#9178) ;
#3625=LINE('',#140923,#9179) ;
#3626=LINE('',#140924,#9180) ;
#3627=LINE('',#140935,#9181) ;
#3628=LINE('',#140938,#9182) ;
#7984=VECTOR('',#103142,1000.) ;
#7985=VECTOR('',#103145,1000.) ;
#7986=VECTOR('',#103158,1.5) ;
#7987=VECTOR('',#103161,1.5) ;
#7988=VECTOR('',#103166,1000.) ;
#7989=VECTOR('',#103169,1000.) ;
#7990=VECTOR('',#103172,1000.) ;
#7991=VECTOR('',#103175,1000.) ;
#7992=VECTOR('',#103178,1.9) ;
#7993=VECTOR('',#103193,1000.) ;
#7994=VECTOR('',#103196,1000.) ;
#7995=VECTOR('',#103245,1000.) ;
#7996=VECTOR('',#103248,1000.) ;
#7997=VECTOR('',#103261,1.5) ;
#7998=VECTOR('',#103264,1.5) ;
#7999=VECTOR('',#103269,1000.) ;
#8000=VECTOR('',#103272,1000.) ;
#8001=VECTOR('',#103275,1000.) ;
#8002=VECTOR('',#103278,1000.) ;
#8003=VECTOR('',#103281,1.9) ;
#8004=VECTOR('',#103284,1000.) ;
#8005=VECTOR('',#103285,1000.) ;
#8006=VECTOR('',#103286,1000.) ;
#8007=VECTOR('',#103287,1000.) ;
#8008=VECTOR('',#103290,1000.) ;
#8009=VECTOR('',#103291,1000.) ;
#8010=VECTOR('',#103292,1000.) ;
#8011=VECTOR('',#103295,1000.) ;
#8012=VECTOR('',#103298,1000.) ;
#8013=VECTOR('',#103299,1000.) ;
#8014=VECTOR('',#103300,1000.) ;
#8015=VECTOR('',#103301,1000.) ;
#8016=VECTOR('',#103304,1000.) ;
#8017=VECTOR('',#103305,1000.) ;
#8018=VECTOR('',#103306,1000.) ;
#8019=VECTOR('',#103307,1000.) ;
#8020=VECTOR('',#103310,1000.) ;
#8021=VECTOR('',#103311,1000.) ;
#8022=VECTOR('',#103312,1000.) ;
#8023=VECTOR('',#103313,1000.) ;
#8024=VECTOR('',#103316,1000.) ;
#8025=VECTOR('',#103337,1000.) ;
#8026=VECTOR('',#103340,1000.) ;
#8027=VECTOR('',#103347,1000.) ;
#8028=VECTOR('',#103350,1000.) ;
#8029=VECTOR('',#103353,1000.) ;
#8030=VECTOR('',#103354,1000.) ;
#8031=VECTOR('',#103355,1000.) ;
#8032=VECTOR('',#103356,1000.) ;
#8033=VECTOR('',#103359,1000.) ;
#8034=VECTOR('',#103360,1000.) ;
#8035=VECTOR('',#103361,1000.) ;
#8036=VECTOR('',#103362,1000.) ;
#8037=VECTOR('',#103365,1000.) ;
#8038=VECTOR('',#103368,1000.) ;
#8039=VECTOR('',#103369,1000.) ;
#8040=VECTOR('',#103370,1000.) ;
#8041=VECTOR('',#103371,1000.) ;
#8042=VECTOR('',#103378,1000.) ;
#8043=VECTOR('',#103385,1000.) ;
#8044=VECTOR('',#103386,1000.) ;
#8045=VECTOR('',#103387,1000.) ;
#8046=VECTOR('',#103388,1000.) ;
#8047=VECTOR('',#103391,1000.) ;
#8048=VECTOR('',#103392,1000.) ;
#8049=VECTOR('',#103393,1000.) ;
#8050=VECTOR('',#103394,1000.) ;
#8051=VECTOR('',#103397,1000.) ;
#8052=VECTOR('',#103400,1000.) ;
#8053=VECTOR('',#103401,1000.) ;
#8054=VECTOR('',#103402,1000.) ;
#8055=VECTOR('',#103403,1000.) ;
#8056=VECTOR('',#103406,1000.) ;
#8057=VECTOR('',#103407,1000.) ;
#8058=VECTOR('',#103410,1000.) ;
#8059=VECTOR('',#103413,1000.) ;
#8060=VECTOR('',#103416,1000.) ;
#8061=VECTOR('',#103419,1000.) ;
#8062=VECTOR('',#103420,1000.) ;
#8063=VECTOR('',#103421,1000.) ;
#8064=VECTOR('',#103424,1000.) ;
#8065=VECTOR('',#103425,1000.) ;
#8066=VECTOR('',#103426,1000.) ;
#8067=VECTOR('',#103429,1000.) ;
#8068=VECTOR('',#103430,1000.) ;
#8069=VECTOR('',#103431,1000.) ;
#8070=VECTOR('',#103432,1000.) ;
#8071=VECTOR('',#103435,1000.) ;
#8072=VECTOR('',#103436,1000.) ;
#8073=VECTOR('',#103437,1000.) ;
#8074=VECTOR('',#103438,1000.) ;
#8075=VECTOR('',#103441,1000.) ;
#8076=VECTOR('',#103444,1000.) ;
#8077=VECTOR('',#103447,1000.) ;
#8078=VECTOR('',#103450,1000.) ;
#8079=VECTOR('',#103453,1000.) ;
#8080=VECTOR('',#103456,1000.) ;
#8081=VECTOR('',#103459,1000.) ;
#8082=VECTOR('',#103462,1000.) ;
#8083=VECTOR('',#103465,1000.) ;
#8084=VECTOR('',#103466,1000.) ;
#8085=VECTOR('',#103467,1000.) ;
#8086=VECTOR('',#103468,1000.) ;
#8087=VECTOR('',#103471,1000.) ;
#8088=VECTOR('',#103472,1000.) ;
#8089=VECTOR('',#103473,1000.) ;
#8090=VECTOR('',#103476,1000.) ;
#8091=VECTOR('',#103477,1000.) ;
#8092=VECTOR('',#103478,1000.) ;
#8093=VECTOR('',#103481,1000.) ;
#8094=VECTOR('',#103482,1000.) ;
#8095=VECTOR('',#103483,1000.) ;
#8096=VECTOR('',#103484,1000.) ;
#8097=VECTOR('',#103485,1000.) ;
#8098=VECTOR('',#103486,1000.) ;
#8099=VECTOR('',#103487,1000.) ;
#8100=VECTOR('',#103488,1000.) ;
#8101=VECTOR('',#103489,1000.) ;
#8102=VECTOR('',#103490,1000.) ;
#8103=VECTOR('',#103491,1000.) ;
#8104=VECTOR('',#103492,1000.) ;
#8105=VECTOR('',#103495,1000.) ;
#8106=VECTOR('',#103496,1000.) ;
#8107=VECTOR('',#103497,1000.) ;
#8108=VECTOR('',#103498,1000.) ;
#8109=VECTOR('',#103501,1000.) ;
#8110=VECTOR('',#103504,1000.) ;
#8111=VECTOR('',#103507,1000.) ;
#8112=VECTOR('',#103510,1000.) ;
#8113=VECTOR('',#103513,1000.) ;
#8114=VECTOR('',#103516,1000.) ;
#8115=VECTOR('',#103519,1000.) ;
#8116=VECTOR('',#103522,1000.) ;
#8117=VECTOR('',#103525,1000.) ;
#8118=VECTOR('',#103526,1000.) ;
#8119=VECTOR('',#103527,1000.) ;
#8120=VECTOR('',#103528,1000.) ;
#8121=VECTOR('',#103531,1000.) ;
#8122=VECTOR('',#103532,1000.) ;
#8123=VECTOR('',#103533,1000.) ;
#8124=VECTOR('',#103534,1000.) ;
#8125=VECTOR('',#103535,1000.) ;
#8126=VECTOR('',#103536,1000.) ;
#8127=VECTOR('',#103539,1000.) ;
#8128=VECTOR('',#103540,1000.) ;
#8129=VECTOR('',#103543,1000.) ;
#8130=VECTOR('',#103546,1000.) ;
#8131=VECTOR('',#103547,1000.) ;
#8132=VECTOR('',#103548,1000.) ;
#8133=VECTOR('',#103549,1000.) ;
#8134=VECTOR('',#103582,1000.) ;
#8135=VECTOR('',#103583,1000.) ;
#8136=VECTOR('',#103584,1000.) ;
#8137=VECTOR('',#103585,1000.) ;
#8138=VECTOR('',#103588,1000.) ;
#8139=VECTOR('',#103589,1000.) ;
#8140=VECTOR('',#103590,1000.) ;
#8141=VECTOR('',#103591,1000.) ;
#8142=VECTOR('',#103596,1000.) ;
#8143=VECTOR('',#103597,1000.) ;
#8144=VECTOR('',#103598,1000.) ;
#8145=VECTOR('',#103601,1000.) ;
#8146=VECTOR('',#103602,1000.) ;
#8147=VECTOR('',#103603,1000.) ;
#8148=VECTOR('',#103606,1000.) ;
#8149=VECTOR('',#103609,1000.) ;
#8150=VECTOR('',#103614,1000.) ;
#8151=VECTOR('',#103621,1000.) ;
#8152=VECTOR('',#103622,1000.) ;
#8153=VECTOR('',#103625,1000.) ;
#8154=VECTOR('',#103626,1000.) ;
#8155=VECTOR('',#103627,1000.) ;
#8156=VECTOR('',#103630,1000.) ;
#8157=VECTOR('',#103631,1000.) ;
#8158=VECTOR('',#103632,1000.) ;
#8159=VECTOR('',#103635,1000.) ;
#8160=VECTOR('',#103636,1000.) ;
#8161=VECTOR('',#103637,1000.) ;
#8162=VECTOR('',#103640,1000.) ;
#8163=VECTOR('',#103641,1000.) ;
#8164=VECTOR('',#103642,1000.) ;
#8165=VECTOR('',#103643,1000.) ;
#8166=VECTOR('',#103644,1000.) ;
#8167=VECTOR('',#103645,1000.) ;
#8168=VECTOR('',#103648,1000.) ;
#8169=VECTOR('',#103649,1000.) ;
#8170=VECTOR('',#103650,1000.) ;
#8171=VECTOR('',#103651,1000.) ;
#8172=VECTOR('',#103652,1000.) ;
#8173=VECTOR('',#103653,1000.) ;
#8174=VECTOR('',#103656,1000.) ;
#8175=VECTOR('',#103657,1000.) ;
#8176=VECTOR('',#103658,1000.) ;
#8177=VECTOR('',#103659,1000.) ;
#8178=VECTOR('',#103662,1000.) ;
#8179=VECTOR('',#103663,1000.) ;
#8180=VECTOR('',#103664,1000.) ;
#8181=VECTOR('',#103665,1000.) ;
#8182=VECTOR('',#103668,1000.) ;
#8183=VECTOR('',#103669,1000.) ;
#8184=VECTOR('',#103670,1000.) ;
#8185=VECTOR('',#103671,1000.) ;
#8186=VECTOR('',#103674,1000.) ;
#8187=VECTOR('',#103675,1000.) ;
#8188=VECTOR('',#103676,1000.) ;
#8189=VECTOR('',#103677,1000.) ;
#8190=VECTOR('',#103680,1000.) ;
#8191=VECTOR('',#103681,1000.) ;
#8192=VECTOR('',#103682,1000.) ;
#8193=VECTOR('',#103683,1000.) ;
#8194=VECTOR('',#103684,1000.) ;
#8195=VECTOR('',#103687,1000.) ;
#8196=VECTOR('',#103690,1000.) ;
#8197=VECTOR('',#103693,1000.) ;
#8198=VECTOR('',#103700,1000.) ;
#8199=VECTOR('',#103701,1000.) ;
#8200=VECTOR('',#103704,1000.) ;
#8201=VECTOR('',#103705,1000.) ;
#8202=VECTOR('',#103710,1000.) ;
#8203=VECTOR('',#103713,1000.) ;
#8204=VECTOR('',#103714,1000.) ;
#8205=VECTOR('',#103719,1000.) ;
#8206=VECTOR('',#103722,1000.) ;
#8207=VECTOR('',#103723,1000.) ;
#8208=VECTOR('',#103728,1000.) ;
#8209=VECTOR('',#103731,1000.) ;
#8210=VECTOR('',#103736,1000.) ;
#8211=VECTOR('',#103739,1000.) ;
#8212=VECTOR('',#103740,1000.) ;
#8213=VECTOR('',#103743,1000.) ;
#8214=VECTOR('',#103744,1000.) ;
#8215=VECTOR('',#103747,1000.) ;
#8216=VECTOR('',#103748,1000.) ;
#8217=VECTOR('',#103751,1000.) ;
#8218=VECTOR('',#103752,1000.) ;
#8219=VECTOR('',#103753,1000.) ;
#8220=VECTOR('',#103754,1000.) ;
#8221=VECTOR('',#103757,1000.) ;
#8222=VECTOR('',#103758,1000.) ;
#8223=VECTOR('',#103759,1000.) ;
#8224=VECTOR('',#103760,1000.) ;
#8225=VECTOR('',#103763,1000.) ;
#8226=VECTOR('',#103764,1000.) ;
#8227=VECTOR('',#103765,1000.) ;
#8228=VECTOR('',#103766,1000.) ;
#8229=VECTOR('',#103769,1000.) ;
#8230=VECTOR('',#103770,1000.) ;
#8231=VECTOR('',#103771,1000.) ;
#8232=VECTOR('',#103772,1000.) ;
#8233=VECTOR('',#103775,1000.) ;
#8234=VECTOR('',#103776,1000.) ;
#8235=VECTOR('',#103777,1000.) ;
#8236=VECTOR('',#103778,1000.) ;
#8237=VECTOR('',#103779,1000.) ;
#8238=VECTOR('',#103782,1000.) ;
#8239=VECTOR('',#103785,1000.) ;
#8240=VECTOR('',#103788,1000.) ;
#8241=VECTOR('',#103793,1000.) ;
#8242=VECTOR('',#103796,1000.) ;
#8243=VECTOR('',#103799,1000.) ;
#8244=VECTOR('',#103800,1000.) ;
#8245=VECTOR('',#103805,1000.) ;
#8246=VECTOR('',#103808,1000.) ;
#8247=VECTOR('',#103809,1000.) ;
#8248=VECTOR('',#103814,1000.) ;
#8249=VECTOR('',#103817,1000.) ;
#8250=VECTOR('',#103818,1000.) ;
#8251=VECTOR('',#103823,1000.) ;
#8252=VECTOR('',#103826,1000.) ;
#8253=VECTOR('',#103829,1000.) ;
#8254=VECTOR('',#103830,1000.) ;
#8255=VECTOR('',#103831,1000.) ;
#8256=VECTOR('',#103832,1000.) ;
#8257=VECTOR('',#103835,1000.) ;
#8258=VECTOR('',#103836,1000.) ;
#8259=VECTOR('',#103837,1000.) ;
#8260=VECTOR('',#103838,1000.) ;
#8261=VECTOR('',#103841,1000.) ;
#8262=VECTOR('',#103842,1000.) ;
#8263=VECTOR('',#103843,1000.) ;
#8264=VECTOR('',#103846,1000.) ;
#8265=VECTOR('',#103847,1000.) ;
#8266=VECTOR('',#103848,1000.) ;
#8267=VECTOR('',#103851,1000.) ;
#8268=VECTOR('',#103854,1000.) ;
#8269=VECTOR('',#103855,1000.) ;
#8270=VECTOR('',#103856,1000.) ;
#8271=VECTOR('',#103867,1000.) ;
#8272=VECTOR('',#103870,1000.) ;
#8273=VECTOR('',#104387,1000.) ;
#8274=VECTOR('',#104388,1000.) ;
#8275=VECTOR('',#104389,1000.) ;
#8276=VECTOR('',#104390,1000.) ;
#8277=VECTOR('',#104395,1000.) ;
#8278=VECTOR('',#104400,1000.) ;
#8279=VECTOR('',#104401,1000.) ;
#8280=VECTOR('',#104402,1000.) ;
#8281=VECTOR('',#104407,1000.) ;
#8282=VECTOR('',#104412,1000.) ;
#8283=VECTOR('',#104413,1000.) ;
#8284=VECTOR('',#104414,1000.) ;
#8285=VECTOR('',#104419,1000.) ;
#8286=VECTOR('',#104424,1000.) ;
#8287=VECTOR('',#104425,1000.) ;
#8288=VECTOR('',#104426,1000.) ;
#8289=VECTOR('',#104431,1000.) ;
#8290=VECTOR('',#104436,1000.) ;
#8291=VECTOR('',#104437,1000.) ;
#8292=VECTOR('',#104438,1000.) ;
#8293=VECTOR('',#104443,1000.) ;
#8294=VECTOR('',#104444,1000.) ;
#8295=VECTOR('',#104445,1000.) ;
#8296=VECTOR('',#104446,1000.) ;
#8297=VECTOR('',#104447,1000.) ;
#8298=VECTOR('',#104448,1000.) ;
#8299=VECTOR('',#104451,1000.) ;
#8300=VECTOR('',#104452,1000.) ;
#8301=VECTOR('',#104453,1000.) ;
#8302=VECTOR('',#104454,1000.) ;
#8303=VECTOR('',#104457,1000.) ;
#8304=VECTOR('',#104458,1000.) ;
#8305=VECTOR('',#104463,1000.) ;
#8306=VECTOR('',#104464,1000.) ;
#8307=VECTOR('',#104465,1000.) ;
#8308=VECTOR('',#104468,1000.) ;
#8309=VECTOR('',#104469,1000.) ;
#8310=VECTOR('',#104470,1000.) ;
#8311=VECTOR('',#104471,1000.) ;
#8312=VECTOR('',#104474,1000.) ;
#8313=VECTOR('',#104477,1000.) ;
#8314=VECTOR('',#104478,1000.) ;
#8315=VECTOR('',#104479,1000.) ;
#8316=VECTOR('',#104480,1000.) ;
#8317=VECTOR('',#104495,1000.) ;
#8318=VECTOR('',#104496,1000.) ;
#8319=VECTOR('',#104497,1000.) ;
#8320=VECTOR('',#104498,1000.) ;
#8321=VECTOR('',#104501,1000.) ;
#8322=VECTOR('',#104502,1000.) ;
#8323=VECTOR('',#104503,1000.) ;
#8324=VECTOR('',#104504,1000.) ;
#8325=VECTOR('',#104509,1000.) ;
#8326=VECTOR('',#104510,1000.) ;
#8327=VECTOR('',#104511,1000.) ;
#8328=VECTOR('',#104514,1000.) ;
#8329=VECTOR('',#104515,1000.) ;
#8330=VECTOR('',#104516,1000.) ;
#8331=VECTOR('',#104519,1000.) ;
#8332=VECTOR('',#104522,1000.) ;
#8333=VECTOR('',#104527,1000.) ;
#8334=VECTOR('',#104534,1000.) ;
#8335=VECTOR('',#104535,1000.) ;
#8336=VECTOR('',#104538,1000.) ;
#8337=VECTOR('',#104539,1000.) ;
#8338=VECTOR('',#104540,1000.) ;
#8339=VECTOR('',#104543,1000.) ;
#8340=VECTOR('',#104544,1000.) ;
#8341=VECTOR('',#104545,1000.) ;
#8342=VECTOR('',#104548,1000.) ;
#8343=VECTOR('',#104549,1000.) ;
#8344=VECTOR('',#104550,1000.) ;
#8345=VECTOR('',#104553,1000.) ;
#8346=VECTOR('',#104554,1000.) ;
#8347=VECTOR('',#104555,1000.) ;
#8348=VECTOR('',#104556,1000.) ;
#8349=VECTOR('',#104557,1000.) ;
#8350=VECTOR('',#104558,1000.) ;
#8351=VECTOR('',#104561,1000.) ;
#8352=VECTOR('',#104562,1000.) ;
#8353=VECTOR('',#104563,1000.) ;
#8354=VECTOR('',#104564,1000.) ;
#8355=VECTOR('',#104565,1000.) ;
#8356=VECTOR('',#104566,1000.) ;
#8357=VECTOR('',#104569,1000.) ;
#8358=VECTOR('',#104570,1000.) ;
#8359=VECTOR('',#104571,1000.) ;
#8360=VECTOR('',#104572,1000.) ;
#8361=VECTOR('',#104575,1000.) ;
#8362=VECTOR('',#104576,1000.) ;
#8363=VECTOR('',#104577,1000.) ;
#8364=VECTOR('',#104578,1000.) ;
#8365=VECTOR('',#104581,1000.) ;
#8366=VECTOR('',#104582,1000.) ;
#8367=VECTOR('',#104583,1000.) ;
#8368=VECTOR('',#104584,1000.) ;
#8369=VECTOR('',#104587,1000.) ;
#8370=VECTOR('',#104588,1000.) ;
#8371=VECTOR('',#104589,1000.) ;
#8372=VECTOR('',#104590,1000.) ;
#8373=VECTOR('',#104593,1000.) ;
#8374=VECTOR('',#104594,1000.) ;
#8375=VECTOR('',#104595,1000.) ;
#8376=VECTOR('',#104596,1000.) ;
#8377=VECTOR('',#104597,1000.) ;
#8378=VECTOR('',#104600,1000.) ;
#8379=VECTOR('',#104603,1000.) ;
#8380=VECTOR('',#104606,1000.) ;
#8381=VECTOR('',#104613,1000.) ;
#8382=VECTOR('',#104614,1000.) ;
#8383=VECTOR('',#104617,1000.) ;
#8384=VECTOR('',#104618,1000.) ;
#8385=VECTOR('',#104623,1000.) ;
#8386=VECTOR('',#104626,1000.) ;
#8387=VECTOR('',#104627,1000.) ;
#8388=VECTOR('',#104632,1000.) ;
#8389=VECTOR('',#104635,1000.) ;
#8390=VECTOR('',#104636,1000.) ;
#8391=VECTOR('',#104641,1000.) ;
#8392=VECTOR('',#104644,1000.) ;
#8393=VECTOR('',#104649,1000.) ;
#8394=VECTOR('',#104652,1000.) ;
#8395=VECTOR('',#104653,1000.) ;
#8396=VECTOR('',#104656,1000.) ;
#8397=VECTOR('',#104657,1000.) ;
#8398=VECTOR('',#104660,1000.) ;
#8399=VECTOR('',#104661,1000.) ;
#8400=VECTOR('',#104664,1000.) ;
#8401=VECTOR('',#104665,1000.) ;
#8402=VECTOR('',#104666,1000.) ;
#8403=VECTOR('',#104667,1000.) ;
#8404=VECTOR('',#104670,1000.) ;
#8405=VECTOR('',#104671,1000.) ;
#8406=VECTOR('',#104672,1000.) ;
#8407=VECTOR('',#104673,1000.) ;
#8408=VECTOR('',#104676,1000.) ;
#8409=VECTOR('',#104677,1000.) ;
#8410=VECTOR('',#104678,1000.) ;
#8411=VECTOR('',#104679,1000.) ;
#8412=VECTOR('',#104682,1000.) ;
#8413=VECTOR('',#104683,1000.) ;
#8414=VECTOR('',#104684,1000.) ;
#8415=VECTOR('',#104685,1000.) ;
#8416=VECTOR('',#104688,1000.) ;
#8417=VECTOR('',#104689,1000.) ;
#8418=VECTOR('',#104690,1000.) ;
#8419=VECTOR('',#104691,1000.) ;
#8420=VECTOR('',#104692,1000.) ;
#8421=VECTOR('',#104695,1000.) ;
#8422=VECTOR('',#104698,1000.) ;
#8423=VECTOR('',#104701,1000.) ;
#8424=VECTOR('',#104706,1000.) ;
#8425=VECTOR('',#104709,1000.) ;
#8426=VECTOR('',#104712,1000.) ;
#8427=VECTOR('',#104713,1000.) ;
#8428=VECTOR('',#104718,1000.) ;
#8429=VECTOR('',#104721,1000.) ;
#8430=VECTOR('',#104722,1000.) ;
#8431=VECTOR('',#104727,1000.) ;
#8432=VECTOR('',#104730,1000.) ;
#8433=VECTOR('',#104731,1000.) ;
#8434=VECTOR('',#104736,1000.) ;
#8435=VECTOR('',#104739,1000.) ;
#8436=VECTOR('',#104742,1000.) ;
#8437=VECTOR('',#104743,1000.) ;
#8438=VECTOR('',#104744,1000.) ;
#8439=VECTOR('',#104745,1000.) ;
#8440=VECTOR('',#104748,1000.) ;
#8441=VECTOR('',#104749,1000.) ;
#8442=VECTOR('',#104750,1000.) ;
#8443=VECTOR('',#104751,1000.) ;
#8444=VECTOR('',#104754,1000.) ;
#8445=VECTOR('',#104755,1000.) ;
#8446=VECTOR('',#104756,1000.) ;
#8447=VECTOR('',#104759,1000.) ;
#8448=VECTOR('',#104760,1000.) ;
#8449=VECTOR('',#104761,1000.) ;
#8450=VECTOR('',#104764,1000.) ;
#8451=VECTOR('',#104767,1000.) ;
#8452=VECTOR('',#104768,1000.) ;
#8453=VECTOR('',#104769,1000.) ;
#8454=VECTOR('',#104780,1000.) ;
#8455=VECTOR('',#104783,1000.) ;
#8456=VECTOR('',#105392,1000.) ;
#8457=VECTOR('',#105395,1000.) ;
#8458=VECTOR('',#105408,1.5) ;
#8459=VECTOR('',#105411,1.5) ;
#8460=VECTOR('',#105416,1000.) ;
#8461=VECTOR('',#105419,1000.) ;
#8462=VECTOR('',#105422,1000.) ;
#8463=VECTOR('',#105425,1000.) ;
#8464=VECTOR('',#105428,1.9) ;
#8465=VECTOR('',#105443,1000.) ;
#8466=VECTOR('',#105446,1000.) ;
#8467=VECTOR('',#105495,1000.) ;
#8468=VECTOR('',#105498,1000.) ;
#8469=VECTOR('',#105511,1.5) ;
#8470=VECTOR('',#105514,1.5) ;
#8471=VECTOR('',#105519,1000.) ;
#8472=VECTOR('',#105522,1000.) ;
#8473=VECTOR('',#105525,1000.) ;
#8474=VECTOR('',#105528,1000.) ;
#8475=VECTOR('',#105531,1.9) ;
#8476=VECTOR('',#105534,1000.) ;
#8477=VECTOR('',#105535,1000.) ;
#8478=VECTOR('',#105536,1000.) ;
#8479=VECTOR('',#105537,1000.) ;
#8480=VECTOR('',#105540,1000.) ;
#8481=VECTOR('',#105541,1000.) ;
#8482=VECTOR('',#105542,1000.) ;
#8483=VECTOR('',#105545,1000.) ;
#8484=VECTOR('',#105548,1000.) ;
#8485=VECTOR('',#105549,1000.) ;
#8486=VECTOR('',#105550,1000.) ;
#8487=VECTOR('',#105551,1000.) ;
#8488=VECTOR('',#105554,1000.) ;
#8489=VECTOR('',#105555,1000.) ;
#8490=VECTOR('',#105556,1000.) ;
#8491=VECTOR('',#105557,1000.) ;
#8492=VECTOR('',#105560,1000.) ;
#8493=VECTOR('',#105561,1000.) ;
#8494=VECTOR('',#105562,1000.) ;
#8495=VECTOR('',#105563,1000.) ;
#8496=VECTOR('',#105568,1000.) ;
#8497=VECTOR('',#105587,1000.) ;
#8498=VECTOR('',#105592,1000.) ;
#8499=VECTOR('',#105597,1000.) ;
#8500=VECTOR('',#105598,1000.) ;
#8501=VECTOR('',#105599,1000.) ;
#8502=VECTOR('',#105602,1000.) ;
#8503=VECTOR('',#105603,1000.) ;
#8504=VECTOR('',#105604,1000.) ;
#8505=VECTOR('',#105605,1000.) ;
#8506=VECTOR('',#105608,1000.) ;
#8507=VECTOR('',#105609,1000.) ;
#8508=VECTOR('',#105610,1000.) ;
#8509=VECTOR('',#105611,1000.) ;
#8510=VECTOR('',#105614,1000.) ;
#8511=VECTOR('',#105617,1000.) ;
#8512=VECTOR('',#105618,1000.) ;
#8513=VECTOR('',#105619,1000.) ;
#8514=VECTOR('',#105622,1000.) ;
#8515=VECTOR('',#105623,1000.) ;
#8516=VECTOR('',#105624,1000.) ;
#8517=VECTOR('',#105625,1000.) ;
#8518=VECTOR('',#105626,1000.) ;
#8519=VECTOR('',#105633,1000.) ;
#8520=VECTOR('',#105640,1000.) ;
#8521=VECTOR('',#105641,1000.) ;
#8522=VECTOR('',#105642,1000.) ;
#8523=VECTOR('',#105643,1000.) ;
#8524=VECTOR('',#105646,1000.) ;
#8525=VECTOR('',#105649,1000.) ;
#8526=VECTOR('',#105650,1000.) ;
#8527=VECTOR('',#105651,1000.) ;
#8528=VECTOR('',#105652,1000.) ;
#8529=VECTOR('',#105655,1000.) ;
#8530=VECTOR('',#105656,1000.) ;
#8531=VECTOR('',#105657,1000.) ;
#8532=VECTOR('',#105660,1000.) ;
#8533=VECTOR('',#105663,1000.) ;
#8534=VECTOR('',#105666,1000.) ;
#8535=VECTOR('',#105669,1000.) ;
#8536=VECTOR('',#105670,1000.) ;
#8537=VECTOR('',#105673,1000.) ;
#8538=VECTOR('',#105674,1000.) ;
#8539=VECTOR('',#105675,1000.) ;
#8540=VECTOR('',#105678,1000.) ;
#8541=VECTOR('',#105679,1000.) ;
#8542=VECTOR('',#105680,1000.) ;
#8543=VECTOR('',#105681,1000.) ;
#8544=VECTOR('',#105684,1000.) ;
#8545=VECTOR('',#105685,1000.) ;
#8546=VECTOR('',#105686,1000.) ;
#8547=VECTOR('',#105687,1000.) ;
#8548=VECTOR('',#105690,1000.) ;
#8549=VECTOR('',#105693,1000.) ;
#8550=VECTOR('',#105696,1000.) ;
#8551=VECTOR('',#105699,1000.) ;
#8552=VECTOR('',#105702,1000.) ;
#8553=VECTOR('',#105705,1000.) ;
#8554=VECTOR('',#105708,1000.) ;
#8555=VECTOR('',#105711,1000.) ;
#8556=VECTOR('',#105714,1000.) ;
#8557=VECTOR('',#105715,1000.) ;
#8558=VECTOR('',#105716,1000.) ;
#8559=VECTOR('',#105717,1000.) ;
#8560=VECTOR('',#105720,1000.) ;
#8561=VECTOR('',#105721,1000.) ;
#8562=VECTOR('',#105722,1000.) ;
#8563=VECTOR('',#105725,1000.) ;
#8564=VECTOR('',#105726,1000.) ;
#8565=VECTOR('',#105727,1000.) ;
#8566=VECTOR('',#105730,1000.) ;
#8567=VECTOR('',#105731,1000.) ;
#8568=VECTOR('',#105732,1000.) ;
#8569=VECTOR('',#105733,1000.) ;
#8570=VECTOR('',#105734,1000.) ;
#8571=VECTOR('',#105735,1000.) ;
#8572=VECTOR('',#105736,1000.) ;
#8573=VECTOR('',#105737,1000.) ;
#8574=VECTOR('',#105738,1000.) ;
#8575=VECTOR('',#105739,1000.) ;
#8576=VECTOR('',#105740,1000.) ;
#8577=VECTOR('',#105741,1000.) ;
#8578=VECTOR('',#105744,1000.) ;
#8579=VECTOR('',#105745,1000.) ;
#8580=VECTOR('',#105746,1000.) ;
#8581=VECTOR('',#105747,1000.) ;
#8582=VECTOR('',#105750,1000.) ;
#8583=VECTOR('',#105753,1000.) ;
#8584=VECTOR('',#105756,1000.) ;
#8585=VECTOR('',#105759,1000.) ;
#8586=VECTOR('',#105762,1000.) ;
#8587=VECTOR('',#105765,1000.) ;
#8588=VECTOR('',#105768,1000.) ;
#8589=VECTOR('',#105771,1000.) ;
#8590=VECTOR('',#105774,1000.) ;
#8591=VECTOR('',#105775,1000.) ;
#8592=VECTOR('',#105776,1000.) ;
#8593=VECTOR('',#105777,1000.) ;
#8594=VECTOR('',#105780,1000.) ;
#8595=VECTOR('',#105781,1000.) ;
#8596=VECTOR('',#105782,1000.) ;
#8597=VECTOR('',#105783,1000.) ;
#8598=VECTOR('',#105784,1000.) ;
#8599=VECTOR('',#105785,1000.) ;
#8600=VECTOR('',#105788,1000.) ;
#8601=VECTOR('',#105791,1000.) ;
#8602=VECTOR('',#105796,1000.) ;
#8603=VECTOR('',#105797,1000.) ;
#8604=VECTOR('',#105798,1000.) ;
#8605=VECTOR('',#105799,1000.) ;
#8606=VECTOR('',#105832,1000.) ;
#8607=VECTOR('',#105833,1000.) ;
#8608=VECTOR('',#105834,1000.) ;
#8609=VECTOR('',#105835,1000.) ;
#8610=VECTOR('',#105838,1000.) ;
#8611=VECTOR('',#105839,1000.) ;
#8612=VECTOR('',#105840,1000.) ;
#8613=VECTOR('',#105841,1000.) ;
#8614=VECTOR('',#105846,1000.) ;
#8615=VECTOR('',#105847,1000.) ;
#8616=VECTOR('',#105848,1000.) ;
#8617=VECTOR('',#105851,1000.) ;
#8618=VECTOR('',#105852,1000.) ;
#8619=VECTOR('',#105853,1000.) ;
#8620=VECTOR('',#105856,1000.) ;
#8621=VECTOR('',#105859,1000.) ;
#8622=VECTOR('',#105864,1000.) ;
#8623=VECTOR('',#105871,1000.) ;
#8624=VECTOR('',#105872,1000.) ;
#8625=VECTOR('',#105875,1000.) ;
#8626=VECTOR('',#105876,1000.) ;
#8627=VECTOR('',#105877,1000.) ;
#8628=VECTOR('',#105880,1000.) ;
#8629=VECTOR('',#105881,1000.) ;
#8630=VECTOR('',#105882,1000.) ;
#8631=VECTOR('',#105885,1000.) ;
#8632=VECTOR('',#105886,1000.) ;
#8633=VECTOR('',#105887,1000.) ;
#8634=VECTOR('',#105890,1000.) ;
#8635=VECTOR('',#105891,1000.) ;
#8636=VECTOR('',#105892,1000.) ;
#8637=VECTOR('',#105893,1000.) ;
#8638=VECTOR('',#105894,1000.) ;
#8639=VECTOR('',#105895,1000.) ;
#8640=VECTOR('',#105898,1000.) ;
#8641=VECTOR('',#105899,1000.) ;
#8642=VECTOR('',#105900,1000.) ;
#8643=VECTOR('',#105901,1000.) ;
#8644=VECTOR('',#105902,1000.) ;
#8645=VECTOR('',#105903,1000.) ;
#8646=VECTOR('',#105906,1000.) ;
#8647=VECTOR('',#105907,1000.) ;
#8648=VECTOR('',#105908,1000.) ;
#8649=VECTOR('',#105909,1000.) ;
#8650=VECTOR('',#105912,1000.) ;
#8651=VECTOR('',#105913,1000.) ;
#8652=VECTOR('',#105914,1000.) ;
#8653=VECTOR('',#105915,1000.) ;
#8654=VECTOR('',#105918,1000.) ;
#8655=VECTOR('',#105919,1000.) ;
#8656=VECTOR('',#105920,1000.) ;
#8657=VECTOR('',#105921,1000.) ;
#8658=VECTOR('',#105924,1000.) ;
#8659=VECTOR('',#105925,1000.) ;
#8660=VECTOR('',#105926,1000.) ;
#8661=VECTOR('',#105927,1000.) ;
#8662=VECTOR('',#105930,1000.) ;
#8663=VECTOR('',#105931,1000.) ;
#8664=VECTOR('',#105932,1000.) ;
#8665=VECTOR('',#105933,1000.) ;
#8666=VECTOR('',#105934,1000.) ;
#8667=VECTOR('',#105937,1000.) ;
#8668=VECTOR('',#105940,1000.) ;
#8669=VECTOR('',#105943,1000.) ;
#8670=VECTOR('',#105950,1000.) ;
#8671=VECTOR('',#105951,1000.) ;
#8672=VECTOR('',#105954,1000.) ;
#8673=VECTOR('',#105955,1000.) ;
#8674=VECTOR('',#105960,1000.) ;
#8675=VECTOR('',#105963,1000.) ;
#8676=VECTOR('',#105964,1000.) ;
#8677=VECTOR('',#105969,1000.) ;
#8678=VECTOR('',#105972,1000.) ;
#8679=VECTOR('',#105973,1000.) ;
#8680=VECTOR('',#105978,1000.) ;
#8681=VECTOR('',#105981,1000.) ;
#8682=VECTOR('',#105986,1000.) ;
#8683=VECTOR('',#105989,1000.) ;
#8684=VECTOR('',#105990,1000.) ;
#8685=VECTOR('',#105993,1000.) ;
#8686=VECTOR('',#105994,1000.) ;
#8687=VECTOR('',#105997,1000.) ;
#8688=VECTOR('',#105998,1000.) ;
#8689=VECTOR('',#106001,1000.) ;
#8690=VECTOR('',#106002,1000.) ;
#8691=VECTOR('',#106003,1000.) ;
#8692=VECTOR('',#106004,1000.) ;
#8693=VECTOR('',#106007,1000.) ;
#8694=VECTOR('',#106008,1000.) ;
#8695=VECTOR('',#106009,1000.) ;
#8696=VECTOR('',#106010,1000.) ;
#8697=VECTOR('',#106013,1000.) ;
#8698=VECTOR('',#106014,1000.) ;
#8699=VECTOR('',#106015,1000.) ;
#8700=VECTOR('',#106016,1000.) ;
#8701=VECTOR('',#106019,1000.) ;
#8702=VECTOR('',#106020,1000.) ;
#8703=VECTOR('',#106021,1000.) ;
#8704=VECTOR('',#106022,1000.) ;
#8705=VECTOR('',#106025,1000.) ;
#8706=VECTOR('',#106026,1000.) ;
#8707=VECTOR('',#106027,1000.) ;
#8708=VECTOR('',#106028,1000.) ;
#8709=VECTOR('',#106029,1000.) ;
#8710=VECTOR('',#106032,1000.) ;
#8711=VECTOR('',#106035,1000.) ;
#8712=VECTOR('',#106038,1000.) ;
#8713=VECTOR('',#106043,1000.) ;
#8714=VECTOR('',#106046,1000.) ;
#8715=VECTOR('',#106049,1000.) ;
#8716=VECTOR('',#106050,1000.) ;
#8717=VECTOR('',#106055,1000.) ;
#8718=VECTOR('',#106058,1000.) ;
#8719=VECTOR('',#106059,1000.) ;
#8720=VECTOR('',#106064,1000.) ;
#8721=VECTOR('',#106067,1000.) ;
#8722=VECTOR('',#106068,1000.) ;
#8723=VECTOR('',#106073,1000.) ;
#8724=VECTOR('',#106076,1000.) ;
#8725=VECTOR('',#106079,1000.) ;
#8726=VECTOR('',#106080,1000.) ;
#8727=VECTOR('',#106081,1000.) ;
#8728=VECTOR('',#106082,1000.) ;
#8729=VECTOR('',#106085,1000.) ;
#8730=VECTOR('',#106086,1000.) ;
#8731=VECTOR('',#106087,1000.) ;
#8732=VECTOR('',#106088,1000.) ;
#8733=VECTOR('',#106091,1000.) ;
#8734=VECTOR('',#106092,1000.) ;
#8735=VECTOR('',#106093,1000.) ;
#8736=VECTOR('',#106096,1000.) ;
#8737=VECTOR('',#106097,1000.) ;
#8738=VECTOR('',#106098,1000.) ;
#8739=VECTOR('',#106101,1000.) ;
#8740=VECTOR('',#106104,1000.) ;
#8741=VECTOR('',#106105,1000.) ;
#8742=VECTOR('',#106106,1000.) ;
#8743=VECTOR('',#106117,1000.) ;
#8744=VECTOR('',#106120,1000.) ;
#8745=VECTOR('',#106637,1000.) ;
#8746=VECTOR('',#106638,1000.) ;
#8747=VECTOR('',#106639,1000.) ;
#8748=VECTOR('',#106640,1000.) ;
#8749=VECTOR('',#106645,1000.) ;
#8750=VECTOR('',#106650,1000.) ;
#8751=VECTOR('',#106651,1000.) ;
#8752=VECTOR('',#106652,1000.) ;
#8753=VECTOR('',#106657,1000.) ;
#8754=VECTOR('',#106662,1000.) ;
#8755=VECTOR('',#106663,1000.) ;
#8756=VECTOR('',#106664,1000.) ;
#8757=VECTOR('',#106669,1000.) ;
#8758=VECTOR('',#106674,1000.) ;
#8759=VECTOR('',#106675,1000.) ;
#8760=VECTOR('',#106676,1000.) ;
#8761=VECTOR('',#106681,1000.) ;
#8762=VECTOR('',#106686,1000.) ;
#8763=VECTOR('',#106687,1000.) ;
#8764=VECTOR('',#106688,1000.) ;
#8765=VECTOR('',#106693,1000.) ;
#8766=VECTOR('',#106694,1000.) ;
#8767=VECTOR('',#106695,1000.) ;
#8768=VECTOR('',#106696,1000.) ;
#8769=VECTOR('',#106697,1000.) ;
#8770=VECTOR('',#106698,1000.) ;
#8771=VECTOR('',#106701,1000.) ;
#8772=VECTOR('',#106702,1000.) ;
#8773=VECTOR('',#106703,1000.) ;
#8774=VECTOR('',#106704,1000.) ;
#8775=VECTOR('',#106707,1000.) ;
#8776=VECTOR('',#106708,1000.) ;
#8777=VECTOR('',#106711,1000.) ;
#8778=VECTOR('',#106712,1000.) ;
#8779=VECTOR('',#106713,1000.) ;
#8780=VECTOR('',#106714,1000.) ;
#8781=VECTOR('',#106717,1000.) ;
#8782=VECTOR('',#106720,1000.) ;
#8783=VECTOR('',#106721,1000.) ;
#8784=VECTOR('',#106722,1000.) ;
#8785=VECTOR('',#106723,1000.) ;
#8786=VECTOR('',#106726,1000.) ;
#8787=VECTOR('',#106727,1000.) ;
#8788=VECTOR('',#106730,1000.) ;
#8789=VECTOR('',#106745,1000.) ;
#8790=VECTOR('',#106746,1000.) ;
#8791=VECTOR('',#106747,1000.) ;
#8792=VECTOR('',#106748,1000.) ;
#8793=VECTOR('',#106751,1000.) ;
#8794=VECTOR('',#106752,1000.) ;
#8795=VECTOR('',#106753,1000.) ;
#8796=VECTOR('',#106754,1000.) ;
#8797=VECTOR('',#106759,1000.) ;
#8798=VECTOR('',#106760,1000.) ;
#8799=VECTOR('',#106761,1000.) ;
#8800=VECTOR('',#106764,1000.) ;
#8801=VECTOR('',#106765,1000.) ;
#8802=VECTOR('',#106766,1000.) ;
#8803=VECTOR('',#106769,1000.) ;
#8804=VECTOR('',#106772,1000.) ;
#8805=VECTOR('',#106777,1000.) ;
#8806=VECTOR('',#106784,1000.) ;
#8807=VECTOR('',#106785,1000.) ;
#8808=VECTOR('',#106788,1000.) ;
#8809=VECTOR('',#106789,1000.) ;
#8810=VECTOR('',#106790,1000.) ;
#8811=VECTOR('',#106793,1000.) ;
#8812=VECTOR('',#106794,1000.) ;
#8813=VECTOR('',#106795,1000.) ;
#8814=VECTOR('',#106798,1000.) ;
#8815=VECTOR('',#106799,1000.) ;
#8816=VECTOR('',#106800,1000.) ;
#8817=VECTOR('',#106803,1000.) ;
#8818=VECTOR('',#106804,1000.) ;
#8819=VECTOR('',#106805,1000.) ;
#8820=VECTOR('',#106806,1000.) ;
#8821=VECTOR('',#106807,1000.) ;
#8822=VECTOR('',#106808,1000.) ;
#8823=VECTOR('',#106811,1000.) ;
#8824=VECTOR('',#106812,1000.) ;
#8825=VECTOR('',#106813,1000.) ;
#8826=VECTOR('',#106814,1000.) ;
#8827=VECTOR('',#106815,1000.) ;
#8828=VECTOR('',#106816,1000.) ;
#8829=VECTOR('',#106819,1000.) ;
#8830=VECTOR('',#106820,1000.) ;
#8831=VECTOR('',#106821,1000.) ;
#8832=VECTOR('',#106822,1000.) ;
#8833=VECTOR('',#106825,1000.) ;
#8834=VECTOR('',#106826,1000.) ;
#8835=VECTOR('',#106827,1000.) ;
#8836=VECTOR('',#106828,1000.) ;
#8837=VECTOR('',#106831,1000.) ;
#8838=VECTOR('',#106832,1000.) ;
#8839=VECTOR('',#106833,1000.) ;
#8840=VECTOR('',#106834,1000.) ;
#8841=VECTOR('',#106837,1000.) ;
#8842=VECTOR('',#106838,1000.) ;
#8843=VECTOR('',#106839,1000.) ;
#8844=VECTOR('',#106840,1000.) ;
#8845=VECTOR('',#106843,1000.) ;
#8846=VECTOR('',#106844,1000.) ;
#8847=VECTOR('',#106845,1000.) ;
#8848=VECTOR('',#106846,1000.) ;
#8849=VECTOR('',#106847,1000.) ;
#8850=VECTOR('',#106850,1000.) ;
#8851=VECTOR('',#106853,1000.) ;
#8852=VECTOR('',#106856,1000.) ;
#8853=VECTOR('',#106863,1000.) ;
#8854=VECTOR('',#106864,1000.) ;
#8855=VECTOR('',#106867,1000.) ;
#8856=VECTOR('',#106868,1000.) ;
#8857=VECTOR('',#106873,1000.) ;
#8858=VECTOR('',#106876,1000.) ;
#8859=VECTOR('',#106877,1000.) ;
#8860=VECTOR('',#106882,1000.) ;
#8861=VECTOR('',#106885,1000.) ;
#8862=VECTOR('',#106886,1000.) ;
#8863=VECTOR('',#106891,1000.) ;
#8864=VECTOR('',#106894,1000.) ;
#8865=VECTOR('',#106899,1000.) ;
#8866=VECTOR('',#106902,1000.) ;
#8867=VECTOR('',#106903,1000.) ;
#8868=VECTOR('',#106906,1000.) ;
#8869=VECTOR('',#106907,1000.) ;
#8870=VECTOR('',#106910,1000.) ;
#8871=VECTOR('',#106911,1000.) ;
#8872=VECTOR('',#106914,1000.) ;
#8873=VECTOR('',#106915,1000.) ;
#8874=VECTOR('',#106916,1000.) ;
#8875=VECTOR('',#106917,1000.) ;
#8876=VECTOR('',#106920,1000.) ;
#8877=VECTOR('',#106921,1000.) ;
#8878=VECTOR('',#106922,1000.) ;
#8879=VECTOR('',#106923,1000.) ;
#8880=VECTOR('',#106926,1000.) ;
#8881=VECTOR('',#106927,1000.) ;
#8882=VECTOR('',#106928,1000.) ;
#8883=VECTOR('',#106929,1000.) ;
#8884=VECTOR('',#106932,1000.) ;
#8885=VECTOR('',#106933,1000.) ;
#8886=VECTOR('',#106934,1000.) ;
#8887=VECTOR('',#106935,1000.) ;
#8888=VECTOR('',#106938,1000.) ;
#8889=VECTOR('',#106939,1000.) ;
#8890=VECTOR('',#106940,1000.) ;
#8891=VECTOR('',#106941,1000.) ;
#8892=VECTOR('',#106942,1000.) ;
#8893=VECTOR('',#106945,1000.) ;
#8894=VECTOR('',#106948,1000.) ;
#8895=VECTOR('',#106951,1000.) ;
#8896=VECTOR('',#106956,1000.) ;
#8897=VECTOR('',#106959,1000.) ;
#8898=VECTOR('',#106962,1000.) ;
#8899=VECTOR('',#106963,1000.) ;
#8900=VECTOR('',#106968,1000.) ;
#8901=VECTOR('',#106971,1000.) ;
#8902=VECTOR('',#106972,1000.) ;
#8903=VECTOR('',#106977,1000.) ;
#8904=VECTOR('',#106980,1000.) ;
#8905=VECTOR('',#106981,1000.) ;
#8906=VECTOR('',#106986,1000.) ;
#8907=VECTOR('',#106989,1000.) ;
#8908=VECTOR('',#106992,1000.) ;
#8909=VECTOR('',#106993,1000.) ;
#8910=VECTOR('',#106994,1000.) ;
#8911=VECTOR('',#106995,1000.) ;
#8912=VECTOR('',#106998,1000.) ;
#8913=VECTOR('',#106999,1000.) ;
#8914=VECTOR('',#107000,1000.) ;
#8915=VECTOR('',#107001,1000.) ;
#8916=VECTOR('',#107004,1000.) ;
#8917=VECTOR('',#107005,1000.) ;
#8918=VECTOR('',#107006,1000.) ;
#8919=VECTOR('',#107009,1000.) ;
#8920=VECTOR('',#107010,1000.) ;
#8921=VECTOR('',#107011,1000.) ;
#8922=VECTOR('',#107014,1000.) ;
#8923=VECTOR('',#107017,1000.) ;
#8924=VECTOR('',#107018,1000.) ;
#8925=VECTOR('',#107019,1000.) ;
#8926=VECTOR('',#107030,1000.) ;
#8927=VECTOR('',#107033,1000.) ;
#8928=VECTOR('',#107598,1000.) ;
#8929=VECTOR('',#107601,1000.) ;
#8930=VECTOR('',#107650,1000.) ;
#8931=VECTOR('',#107653,1000.) ;
#8932=VECTOR('',#107666,1.5) ;
#8933=VECTOR('',#107669,1.5) ;
#8934=VECTOR('',#107674,1000.) ;
#8935=VECTOR('',#107677,1000.) ;
#8936=VECTOR('',#107680,1000.) ;
#8937=VECTOR('',#107683,1000.) ;
#8938=VECTOR('',#107686,1.9) ;
#8939=VECTOR('',#107691,1000.) ;
#8940=VECTOR('',#107692,1000.) ;
#8941=VECTOR('',#107693,1000.) ;
#8942=VECTOR('',#107696,1000.) ;
#8943=VECTOR('',#107697,1000.) ;
#8944=VECTOR('',#107698,1000.) ;
#8945=VECTOR('',#107699,1000.) ;
#8946=VECTOR('',#107702,1000.) ;
#8947=VECTOR('',#107703,1000.) ;
#8948=VECTOR('',#107704,1000.) ;
#8949=VECTOR('',#107705,1000.) ;
#8950=VECTOR('',#107708,1000.) ;
#8951=VECTOR('',#107711,1000.) ;
#8952=VECTOR('',#107712,1000.) ;
#8953=VECTOR('',#107713,1000.) ;
#8954=VECTOR('',#107714,1000.) ;
#8955=VECTOR('',#107721,1000.) ;
#8956=VECTOR('',#107722,1000.) ;
#8957=VECTOR('',#107723,1000.) ;
#8958=VECTOR('',#107724,1000.) ;
#8959=VECTOR('',#107727,1000.) ;
#8960=VECTOR('',#107730,1000.) ;
#8961=VECTOR('',#107731,1000.) ;
#8962=VECTOR('',#107732,1000.) ;
#8963=VECTOR('',#107733,1000.) ;
#8964=VECTOR('',#107736,1000.) ;
#8965=VECTOR('',#107737,1000.) ;
#8966=VECTOR('',#107740,1000.) ;
#8967=VECTOR('',#107743,1000.) ;
#8968=VECTOR('',#107744,1000.) ;
#8969=VECTOR('',#107745,1000.) ;
#8970=VECTOR('',#107748,1000.) ;
#8971=VECTOR('',#107749,1000.) ;
#8972=VECTOR('',#107750,1000.) ;
#8973=VECTOR('',#107751,1000.) ;
#8974=VECTOR('',#107754,1000.) ;
#8975=VECTOR('',#107755,1000.) ;
#8976=VECTOR('',#107756,1000.) ;
#8977=VECTOR('',#107757,1000.) ;
#8978=VECTOR('',#107760,1000.) ;
#8979=VECTOR('',#107761,1000.) ;
#8980=VECTOR('',#107762,1000.) ;
#8981=VECTOR('',#107763,1000.) ;
#8982=VECTOR('',#107766,1000.) ;
#8983=VECTOR('',#107767,1000.) ;
#8984=VECTOR('',#107768,1000.) ;
#8985=VECTOR('',#107769,1000.) ;
#8986=VECTOR('',#107772,1000.) ;
#8987=VECTOR('',#107773,1000.) ;
#8988=VECTOR('',#107774,1000.) ;
#8989=VECTOR('',#107775,1000.) ;
#8990=VECTOR('',#107778,1000.) ;
#8991=VECTOR('',#107779,1000.) ;
#8992=VECTOR('',#107780,1000.) ;
#8993=VECTOR('',#107781,1000.) ;
#8994=VECTOR('',#107784,1000.) ;
#8995=VECTOR('',#107785,1000.) ;
#8996=VECTOR('',#107786,1000.) ;
#8997=VECTOR('',#107787,1000.) ;
#8998=VECTOR('',#107790,1000.) ;
#8999=VECTOR('',#107793,1000.) ;
#9000=VECTOR('',#107796,1000.) ;
#9001=VECTOR('',#107799,1000.) ;
#9002=VECTOR('',#107802,1000.) ;
#9003=VECTOR('',#107803,1000.) ;
#9004=VECTOR('',#107804,1000.) ;
#9005=VECTOR('',#107805,1000.) ;
#9006=VECTOR('',#107808,1000.) ;
#9007=VECTOR('',#107809,1000.) ;
#9008=VECTOR('',#107810,1000.) ;
#9009=VECTOR('',#107813,1000.) ;
#9010=VECTOR('',#107814,1000.) ;
#9011=VECTOR('',#107815,1000.) ;
#9012=VECTOR('',#107818,1000.) ;
#9013=VECTOR('',#107819,1000.) ;
#9014=VECTOR('',#107820,1000.) ;
#9015=VECTOR('',#107821,1000.) ;
#9016=VECTOR('',#107822,1000.) ;
#9017=VECTOR('',#107823,1000.) ;
#9018=VECTOR('',#107824,1000.) ;
#9019=VECTOR('',#107825,1000.) ;
#9020=VECTOR('',#107828,1000.) ;
#9021=VECTOR('',#107829,1000.) ;
#9022=VECTOR('',#107830,1000.) ;
#9023=VECTOR('',#107831,1000.) ;
#9024=VECTOR('',#107834,1000.) ;
#9025=VECTOR('',#107837,1000.) ;
#9026=VECTOR('',#107840,1000.) ;
#9027=VECTOR('',#107843,1000.) ;
#9028=VECTOR('',#107846,1000.) ;
#9029=VECTOR('',#107847,1000.) ;
#9030=VECTOR('',#107848,1000.) ;
#9031=VECTOR('',#107849,1000.) ;
#9032=VECTOR('',#107852,1000.) ;
#9033=VECTOR('',#107853,1000.) ;
#9034=VECTOR('',#107854,1000.) ;
#9035=VECTOR('',#107855,1000.) ;
#9036=VECTOR('',#107856,1000.) ;
#9037=VECTOR('',#107859,1000.) ;
#9038=VECTOR('',#107860,1000.) ;
#9039=VECTOR('',#107863,1000.) ;
#9040=VECTOR('',#107866,1000.) ;
#9041=VECTOR('',#107867,1000.) ;
#9042=VECTOR('',#107868,1000.) ;
#9043=VECTOR('',#107869,1000.) ;
#9044=VECTOR('',#107948,1000.) ;
#9045=VECTOR('',#107949,1000.) ;
#9046=VECTOR('',#107950,1000.) ;
#9047=VECTOR('',#107951,1000.) ;
#9048=VECTOR('',#107954,1000.) ;
#9049=VECTOR('',#107955,1000.) ;
#9050=VECTOR('',#107956,1000.) ;
#9051=VECTOR('',#107957,1000.) ;
#9052=VECTOR('',#107962,1000.) ;
#9053=VECTOR('',#107963,1000.) ;
#9054=VECTOR('',#107964,1000.) ;
#9055=VECTOR('',#107967,1000.) ;
#9056=VECTOR('',#107968,1000.) ;
#9057=VECTOR('',#107969,1000.) ;
#9058=VECTOR('',#107972,1000.) ;
#9059=VECTOR('',#107975,1000.) ;
#9060=VECTOR('',#107980,1000.) ;
#9061=VECTOR('',#107987,1000.) ;
#9062=VECTOR('',#107988,1000.) ;
#9063=VECTOR('',#107991,1000.) ;
#9064=VECTOR('',#107992,1000.) ;
#9065=VECTOR('',#107993,1000.) ;
#9066=VECTOR('',#107996,1000.) ;
#9067=VECTOR('',#107997,1000.) ;
#9068=VECTOR('',#107998,1000.) ;
#9069=VECTOR('',#108001,1000.) ;
#9070=VECTOR('',#108002,1000.) ;
#9071=VECTOR('',#108003,1000.) ;
#9072=VECTOR('',#108006,1000.) ;
#9073=VECTOR('',#108007,1000.) ;
#9074=VECTOR('',#108008,1000.) ;
#9075=VECTOR('',#108009,1000.) ;
#9076=VECTOR('',#108010,1000.) ;
#9077=VECTOR('',#108011,1000.) ;
#9078=VECTOR('',#108014,1000.) ;
#9079=VECTOR('',#108015,1000.) ;
#9080=VECTOR('',#108016,1000.) ;
#9081=VECTOR('',#108017,1000.) ;
#9082=VECTOR('',#108018,1000.) ;
#9083=VECTOR('',#108019,1000.) ;
#9084=VECTOR('',#108022,1000.) ;
#9085=VECTOR('',#108023,1000.) ;
#9086=VECTOR('',#108024,1000.) ;
#9087=VECTOR('',#108025,1000.) ;
#9088=VECTOR('',#108028,1000.) ;
#9089=VECTOR('',#108029,1000.) ;
#9090=VECTOR('',#108030,1000.) ;
#9091=VECTOR('',#108031,1000.) ;
#9092=VECTOR('',#108034,1000.) ;
#9093=VECTOR('',#108035,1000.) ;
#9094=VECTOR('',#108036,1000.) ;
#9095=VECTOR('',#108037,1000.) ;
#9096=VECTOR('',#108040,1000.) ;
#9097=VECTOR('',#108041,1000.) ;
#9098=VECTOR('',#108042,1000.) ;
#9099=VECTOR('',#108043,1000.) ;
#9100=VECTOR('',#108046,1000.) ;
#9101=VECTOR('',#108047,1000.) ;
#9102=VECTOR('',#108048,1000.) ;
#9103=VECTOR('',#108049,1000.) ;
#9104=VECTOR('',#108050,1000.) ;
#9105=VECTOR('',#108053,1000.) ;
#9106=VECTOR('',#108056,1000.) ;
#9107=VECTOR('',#108059,1000.) ;
#9108=VECTOR('',#108066,1000.) ;
#9109=VECTOR('',#108067,1000.) ;
#9110=VECTOR('',#108070,1000.) ;
#9111=VECTOR('',#108071,1000.) ;
#9112=VECTOR('',#108076,1000.) ;
#9113=VECTOR('',#108079,1000.) ;
#9114=VECTOR('',#108080,1000.) ;
#9115=VECTOR('',#108085,1000.) ;
#9116=VECTOR('',#108088,1000.) ;
#9117=VECTOR('',#108089,1000.) ;
#9118=VECTOR('',#108094,1000.) ;
#9119=VECTOR('',#108097,1000.) ;
#9120=VECTOR('',#108102,1000.) ;
#9121=VECTOR('',#108105,1000.) ;
#9122=VECTOR('',#108106,1000.) ;
#9123=VECTOR('',#108109,1000.) ;
#9124=VECTOR('',#108110,1000.) ;
#9125=VECTOR('',#108113,1000.) ;
#9126=VECTOR('',#108114,1000.) ;
#9127=VECTOR('',#108117,1000.) ;
#9128=VECTOR('',#108118,1000.) ;
#9129=VECTOR('',#108119,1000.) ;
#9130=VECTOR('',#108120,1000.) ;
#9131=VECTOR('',#108123,1000.) ;
#9132=VECTOR('',#108124,1000.) ;
#9133=VECTOR('',#108125,1000.) ;
#9134=VECTOR('',#108126,1000.) ;
#9135=VECTOR('',#108129,1000.) ;
#9136=VECTOR('',#108130,1000.) ;
#9137=VECTOR('',#108131,1000.) ;
#9138=VECTOR('',#108132,1000.) ;
#9139=VECTOR('',#108135,1000.) ;
#9140=VECTOR('',#108136,1000.) ;
#9141=VECTOR('',#108137,1000.) ;
#9142=VECTOR('',#108138,1000.) ;
#9143=VECTOR('',#108141,1000.) ;
#9144=VECTOR('',#108142,1000.) ;
#9145=VECTOR('',#108143,1000.) ;
#9146=VECTOR('',#108144,1000.) ;
#9147=VECTOR('',#108145,1000.) ;
#9148=VECTOR('',#108148,1000.) ;
#9149=VECTOR('',#108151,1000.) ;
#9150=VECTOR('',#108154,1000.) ;
#9151=VECTOR('',#108159,1000.) ;
#9152=VECTOR('',#108162,1000.) ;
#9153=VECTOR('',#108165,1000.) ;
#9154=VECTOR('',#108166,1000.) ;
#9155=VECTOR('',#108171,1000.) ;
#9156=VECTOR('',#108174,1000.) ;
#9157=VECTOR('',#108175,1000.) ;
#9158=VECTOR('',#108180,1000.) ;
#9159=VECTOR('',#108183,1000.) ;
#9160=VECTOR('',#108184,1000.) ;
#9161=VECTOR('',#108189,1000.) ;
#9162=VECTOR('',#108192,1000.) ;
#9163=VECTOR('',#108195,1000.) ;
#9164=VECTOR('',#108196,1000.) ;
#9165=VECTOR('',#108197,1000.) ;
#9166=VECTOR('',#108198,1000.) ;
#9167=VECTOR('',#108201,1000.) ;
#9168=VECTOR('',#108202,1000.) ;
#9169=VECTOR('',#108203,1000.) ;
#9170=VECTOR('',#108204,1000.) ;
#9171=VECTOR('',#108207,1000.) ;
#9172=VECTOR('',#108208,1000.) ;
#9173=VECTOR('',#108209,1000.) ;
#9174=VECTOR('',#108212,1000.) ;
#9175=VECTOR('',#108213,1000.) ;
#9176=VECTOR('',#108214,1000.) ;
#9177=VECTOR('',#108217,1000.) ;
#9178=VECTOR('',#108220,1000.) ;
#9179=VECTOR('',#108221,1000.) ;
#9180=VECTOR('',#108222,1000.) ;
#9181=VECTOR('',#108233,1000.) ;
#9182=VECTOR('',#108236,1000.) ;
#13538=CYLINDRICAL_SURFACE('',#91152,0.0999999999999998) ;
#13539=CYLINDRICAL_SURFACE('',#91160,1.5) ;
#13540=CYLINDRICAL_SURFACE('',#91161,1.9) ;
#13541=CYLINDRICAL_SURFACE('',#91172,0.1) ;
#13542=CYLINDRICAL_SURFACE('',#91198,0.1) ;
#13543=CYLINDRICAL_SURFACE('',#91206,1.5) ;
#13544=CYLINDRICAL_SURFACE('',#91207,1.9) ;
#13545=CYLINDRICAL_SURFACE('',#91219,0.0999999999999998) ;
#13546=CYLINDRICAL_SURFACE('',#91222,0.0999999999999998) ;
#13547=CYLINDRICAL_SURFACE('',#91225,0.0999999999999998) ;
#13548=CYLINDRICAL_SURFACE('',#91228,0.0999999999999998) ;
#13549=CYLINDRICAL_SURFACE('',#91323,0.1) ;
#13550=CYLINDRICAL_SURFACE('',#91326,0.1) ;
#13551=CYLINDRICAL_SURFACE('',#91329,0.1) ;
#13552=CYLINDRICAL_SURFACE('',#91332,0.1) ;
#13553=CYLINDRICAL_SURFACE('',#91349,0.1) ;
#13554=CYLINDRICAL_SURFACE('',#91352,0.1) ;
#13555=CYLINDRICAL_SURFACE('',#91355,0.1) ;
#13556=CYLINDRICAL_SURFACE('',#91358,0.1) ;
#13557=CYLINDRICAL_SURFACE('',#91368,3.) ;
#13558=CYLINDRICAL_SURFACE('',#91375,0.1) ;
#13559=CYLINDRICAL_SURFACE('',#91379,0.0999999999999997) ;
#13560=CYLINDRICAL_SURFACE('',#91381,0.0999999999999997) ;
#13561=CYLINDRICAL_SURFACE('',#91383,0.0999999999999998) ;
#13562=CYLINDRICAL_SURFACE('',#91385,0.1) ;
#13563=CYLINDRICAL_SURFACE('',#91387,0.0999999999999998) ;
#13564=CYLINDRICAL_SURFACE('',#91389,0.0999999999999999) ;
#13565=CYLINDRICAL_SURFACE('',#91397,0.1) ;
#13566=CYLINDRICAL_SURFACE('',#91399,0.0999999999999999) ;
#13567=CYLINDRICAL_SURFACE('',#91401,0.1) ;
#13568=CYLINDRICAL_SURFACE('',#91403,0.0999999999999998) ;
#13569=CYLINDRICAL_SURFACE('',#91405,0.0999999999999997) ;
#13570=CYLINDRICAL_SURFACE('',#91407,0.1) ;
#13571=CYLINDRICAL_SURFACE('',#91414,0.1) ;
#13572=CYLINDRICAL_SURFACE('',#91416,0.0999999999999999) ;
#13573=CYLINDRICAL_SURFACE('',#91418,0.0999999999999999) ;
#13574=CYLINDRICAL_SURFACE('',#91420,0.1) ;
#13575=CYLINDRICAL_SURFACE('',#91425,0.0999999999999998) ;
#13576=CYLINDRICAL_SURFACE('',#91427,0.1) ;
#13577=CYLINDRICAL_SURFACE('',#91430,0.1) ;
#13578=CYLINDRICAL_SURFACE('',#91431,0.0999999999999994) ;
#13579=CYLINDRICAL_SURFACE('',#91432,0.0999999999999998) ;
#13580=CYLINDRICAL_SURFACE('',#91434,0.1) ;
#13581=CYLINDRICAL_SURFACE('',#91437,0.1) ;
#13582=CYLINDRICAL_SURFACE('',#91439,0.1) ;
#13583=CYLINDRICAL_SURFACE('',#91440,0.1) ;
#13584=CYLINDRICAL_SURFACE('',#91445,0.0999999999999994) ;
#13585=CYLINDRICAL_SURFACE('',#91446,0.0999999999999998) ;
#13586=CYLINDRICAL_SURFACE('',#91449,0.0999999999999994) ;
#13587=CYLINDRICAL_SURFACE('',#91450,0.1) ;
#13588=CYLINDRICAL_SURFACE('',#91454,0.1) ;
#13589=CYLINDRICAL_SURFACE('',#91456,0.0999999999999998) ;
#13590=CYLINDRICAL_SURFACE('',#91462,0.0999999999999998) ;
#13591=CYLINDRICAL_SURFACE('',#91464,0.1) ;
#13592=CYLINDRICAL_SURFACE('',#91467,0.0999999999999998) ;
#13593=CYLINDRICAL_SURFACE('',#91476,0.1) ;
#13594=CYLINDRICAL_SURFACE('',#91478,0.1) ;
#13595=CYLINDRICAL_SURFACE('',#91480,0.0999999999999998) ;
#13596=CYLINDRICAL_SURFACE('',#91483,0.1) ;
#13597=CYLINDRICAL_SURFACE('',#91485,0.1) ;
#13598=CYLINDRICAL_SURFACE('',#91487,0.1) ;
#13599=CYLINDRICAL_SURFACE('',#91498,0.1) ;
#13600=CYLINDRICAL_SURFACE('',#91500,0.1) ;
#13601=CYLINDRICAL_SURFACE('',#91502,0.1) ;
#13602=CYLINDRICAL_SURFACE('',#91504,0.1) ;
#13603=CYLINDRICAL_SURFACE('',#91510,0.1) ;
#13604=CYLINDRICAL_SURFACE('',#91511,0.0999999999999998) ;
#13605=CYLINDRICAL_SURFACE('',#91520,0.1) ;
#13606=CYLINDRICAL_SURFACE('',#91522,0.1) ;
#13607=CYLINDRICAL_SURFACE('',#91524,0.0999999999999998) ;
#13608=CYLINDRICAL_SURFACE('',#91527,0.1) ;
#13609=CYLINDRICAL_SURFACE('',#91529,0.1) ;
#13610=CYLINDRICAL_SURFACE('',#91531,0.0999999999999998) ;
#13611=CYLINDRICAL_SURFACE('',#91542,0.1) ;
#13612=CYLINDRICAL_SURFACE('',#91544,0.1) ;
#13613=CYLINDRICAL_SURFACE('',#91546,0.1) ;
#13614=CYLINDRICAL_SURFACE('',#91548,0.1) ;
#13615=CYLINDRICAL_SURFACE('',#91554,0.0999999999999998) ;
#13616=CYLINDRICAL_SURFACE('',#91557,0.1) ;
#13617=CYLINDRICAL_SURFACE('',#91561,0.1) ;
#13618=CYLINDRICAL_SURFACE('',#91563,0.0999999999999994) ;
#13619=CYLINDRICAL_SURFACE('',#91569,0.0999999999999994) ;
#13620=CYLINDRICAL_SURFACE('',#91574,0.0999999999999998) ;
#13621=CYLINDRICAL_SURFACE('',#91576,0.1) ;
#13622=CYLINDRICAL_SURFACE('',#91582,0.0999999999999998) ;
#13623=CYLINDRICAL_SURFACE('',#91584,0.0999999999999998) ;
#13624=CYLINDRICAL_SURFACE('',#91586,0.1) ;
#13625=CYLINDRICAL_SURFACE('',#91588,0.1) ;
#13626=CYLINDRICAL_SURFACE('',#91590,0.1) ;
#13627=CYLINDRICAL_SURFACE('',#91592,0.1) ;
#13628=CYLINDRICAL_SURFACE('',#91594,0.1) ;
#13629=CYLINDRICAL_SURFACE('',#91595,0.1) ;
#13630=CYLINDRICAL_SURFACE('',#91596,0.1) ;
#13631=CYLINDRICAL_SURFACE('',#91597,0.0999999999999999) ;
#13632=CYLINDRICAL_SURFACE('',#91598,0.0999999999999998) ;
#13633=CYLINDRICAL_SURFACE('',#91600,0.0999999999999998) ;
#13634=CYLINDRICAL_SURFACE('',#91602,0.1) ;
#13635=CYLINDRICAL_SURFACE('',#91606,0.1) ;
#13636=CYLINDRICAL_SURFACE('',#91612,0.1) ;
#13637=CYLINDRICAL_SURFACE('',#91613,0.1) ;
#13638=CYLINDRICAL_SURFACE('',#91617,0.1) ;
#13639=CYLINDRICAL_SURFACE('',#91621,0.1) ;
#13640=CYLINDRICAL_SURFACE('',#91623,0.1) ;
#13641=CYLINDRICAL_SURFACE('',#91631,0.100000000000001) ;
#13642=CYLINDRICAL_SURFACE('',#91635,0.0999999999999994) ;
#13643=CYLINDRICAL_SURFACE('',#91639,0.100000000000001) ;
#13644=CYLINDRICAL_SURFACE('',#91643,0.0999999999999994) ;
#13645=CYLINDRICAL_SURFACE('',#91688,0.1) ;
#13646=CYLINDRICAL_SURFACE('',#91691,0.1) ;
#13647=CYLINDRICAL_SURFACE('',#91694,0.1) ;
#13648=CYLINDRICAL_SURFACE('',#91697,0.1) ;
#13649=CYLINDRICAL_SURFACE('',#91714,0.1) ;
#13650=CYLINDRICAL_SURFACE('',#91717,0.1) ;
#13651=CYLINDRICAL_SURFACE('',#91720,0.1) ;
#13652=CYLINDRICAL_SURFACE('',#91723,0.1) ;
#13653=CYLINDRICAL_SURFACE('',#91733,3.) ;
#13654=CYLINDRICAL_SURFACE('',#91740,0.1) ;
#13655=CYLINDRICAL_SURFACE('',#91744,0.0999999999999997) ;
#13656=CYLINDRICAL_SURFACE('',#91746,0.0999999999999997) ;
#13657=CYLINDRICAL_SURFACE('',#91748,0.0999999999999998) ;
#13658=CYLINDRICAL_SURFACE('',#91750,0.1) ;
#13659=CYLINDRICAL_SURFACE('',#91752,0.0999999999999998) ;
#13660=CYLINDRICAL_SURFACE('',#91754,0.0999999999999999) ;
#13661=CYLINDRICAL_SURFACE('',#91762,0.0999999999999998) ;
#13662=CYLINDRICAL_SURFACE('',#91764,0.0999999999999999) ;
#13663=CYLINDRICAL_SURFACE('',#91766,0.1) ;
#13664=CYLINDRICAL_SURFACE('',#91768,0.1) ;
#13665=CYLINDRICAL_SURFACE('',#91770,0.0999999999999997) ;
#13666=CYLINDRICAL_SURFACE('',#91772,0.1) ;
#13667=CYLINDRICAL_SURFACE('',#91779,0.0999999999999999) ;
#13668=CYLINDRICAL_SURFACE('',#91781,0.0999999999999999) ;
#13669=CYLINDRICAL_SURFACE('',#91783,0.0999999999999999) ;
#13670=CYLINDRICAL_SURFACE('',#91785,0.1) ;
#13671=CYLINDRICAL_SURFACE('',#91790,0.0999999999999998) ;
#13672=CYLINDRICAL_SURFACE('',#91792,0.1) ;
#13673=CYLINDRICAL_SURFACE('',#91795,0.0999999999999999) ;
#13674=CYLINDRICAL_SURFACE('',#91796,0.0999999999999994) ;
#13675=CYLINDRICAL_SURFACE('',#91797,0.0999999999999998) ;
#13676=CYLINDRICAL_SURFACE('',#91799,0.1) ;
#13677=CYLINDRICAL_SURFACE('',#91802,0.1) ;
#13678=CYLINDRICAL_SURFACE('',#91804,0.1) ;
#13679=CYLINDRICAL_SURFACE('',#91805,0.1) ;
#13680=CYLINDRICAL_SURFACE('',#91810,0.0999999999999998) ;
#13681=CYLINDRICAL_SURFACE('',#91813,0.0999999999999994) ;
#13682=CYLINDRICAL_SURFACE('',#91814,0.0999999999999999) ;
#13683=CYLINDRICAL_SURFACE('',#91818,0.1) ;
#13684=CYLINDRICAL_SURFACE('',#91820,0.0999999999999998) ;
#13685=CYLINDRICAL_SURFACE('',#91826,0.0999999999999998) ;
#13686=CYLINDRICAL_SURFACE('',#91828,0.1) ;
#13687=CYLINDRICAL_SURFACE('',#91831,0.0999999999999998) ;
#13688=CYLINDRICAL_SURFACE('',#91840,0.0999999999999998) ;
#13689=CYLINDRICAL_SURFACE('',#91842,0.1) ;
#13690=CYLINDRICAL_SURFACE('',#91844,0.0999999999999998) ;
#13691=CYLINDRICAL_SURFACE('',#91847,0.1) ;
#13692=CYLINDRICAL_SURFACE('',#91849,0.1) ;
#13693=CYLINDRICAL_SURFACE('',#91851,0.1) ;
#13694=CYLINDRICAL_SURFACE('',#91862,0.1) ;
#13695=CYLINDRICAL_SURFACE('',#91864,0.1) ;
#13696=CYLINDRICAL_SURFACE('',#91866,0.1) ;
#13697=CYLINDRICAL_SURFACE('',#91868,0.1) ;
#13698=CYLINDRICAL_SURFACE('',#91874,0.1) ;
#13699=CYLINDRICAL_SURFACE('',#91875,0.0999999999999998) ;
#13700=CYLINDRICAL_SURFACE('',#91884,0.1) ;
#13701=CYLINDRICAL_SURFACE('',#91886,0.1) ;
#13702=CYLINDRICAL_SURFACE('',#91888,0.0999999999999998) ;
#13703=CYLINDRICAL_SURFACE('',#91891,0.1) ;
#13704=CYLINDRICAL_SURFACE('',#91893,0.1) ;
#13705=CYLINDRICAL_SURFACE('',#91895,0.0999999999999998) ;
#13706=CYLINDRICAL_SURFACE('',#91906,0.1) ;
#13707=CYLINDRICAL_SURFACE('',#91908,0.1) ;
#13708=CYLINDRICAL_SURFACE('',#91910,0.1) ;
#13709=CYLINDRICAL_SURFACE('',#91912,0.1) ;
#13710=CYLINDRICAL_SURFACE('',#91918,0.0999999999999998) ;
#13711=CYLINDRICAL_SURFACE('',#91923,0.0999999999999998) ;
#13712=CYLINDRICAL_SURFACE('',#91929,0.0999999999999994) ;
#13713=CYLINDRICAL_SURFACE('',#91933,0.1) ;
#13714=CYLINDRICAL_SURFACE('',#91935,0.1) ;
#13715=CYLINDRICAL_SURFACE('',#91940,0.0999999999999998) ;
#13716=CYLINDRICAL_SURFACE('',#91941,0.0999999999999998) ;
#13717=CYLINDRICAL_SURFACE('',#91942,0.1) ;
#13718=CYLINDRICAL_SURFACE('',#91943,0.1) ;
#13719=CYLINDRICAL_SURFACE('',#91946,0.0999999999999999) ;
#13720=CYLINDRICAL_SURFACE('',#91951,0.1) ;
#13721=CYLINDRICAL_SURFACE('',#91954,0.1) ;
#13722=CYLINDRICAL_SURFACE('',#91958,0.1) ;
#13723=CYLINDRICAL_SURFACE('',#91969,0.0999999999999998) ;
#13724=CYLINDRICAL_SURFACE('',#91971,0.1) ;
#13725=CYLINDRICAL_SURFACE('',#91973,0.1) ;
#13726=CYLINDRICAL_SURFACE('',#91975,0.1) ;
#13727=CYLINDRICAL_SURFACE('',#91985,0.1) ;
#13728=CYLINDRICAL_SURFACE('',#91987,0.1) ;
#13729=CYLINDRICAL_SURFACE('',#91988,0.1) ;
#13730=CYLINDRICAL_SURFACE('',#91991,0.1) ;
#13731=CYLINDRICAL_SURFACE('',#91992,0.1) ;
#13732=CYLINDRICAL_SURFACE('',#92000,0.1) ;
#13733=CYLINDRICAL_SURFACE('',#92002,0.0999999999999998) ;
#13734=CYLINDRICAL_SURFACE('',#92004,0.1) ;
#13735=CYLINDRICAL_SURFACE('',#92006,0.1) ;
#13736=CYLINDRICAL_SURFACE('',#92012,0.1) ;
#13737=CYLINDRICAL_SURFACE('',#92041,0.0999999999999994) ;
#13738=CYLINDRICAL_SURFACE('',#92049,1.5) ;
#13739=CYLINDRICAL_SURFACE('',#92050,1.9) ;
#13740=CYLINDRICAL_SURFACE('',#92061,0.1) ;
#13741=CYLINDRICAL_SURFACE('',#92087,0.0999999999999994) ;
#13742=CYLINDRICAL_SURFACE('',#92095,1.5) ;
#13743=CYLINDRICAL_SURFACE('',#92096,1.9) ;
#13744=CYLINDRICAL_SURFACE('',#92108,0.0999999999999998) ;
#13745=CYLINDRICAL_SURFACE('',#92111,0.0999999999999998) ;
#13746=CYLINDRICAL_SURFACE('',#92114,0.0999999999999998) ;
#13747=CYLINDRICAL_SURFACE('',#92117,0.0999999999999998) ;
#13748=CYLINDRICAL_SURFACE('',#92212,0.0999999999999994) ;
#13749=CYLINDRICAL_SURFACE('',#92215,0.0999999999999994) ;
#13750=CYLINDRICAL_SURFACE('',#92218,0.0999999999999994) ;
#13751=CYLINDRICAL_SURFACE('',#92221,0.0999999999999994) ;
#13752=CYLINDRICAL_SURFACE('',#92238,0.0999999999999994) ;
#13753=CYLINDRICAL_SURFACE('',#92241,0.0999999999999994) ;
#13754=CYLINDRICAL_SURFACE('',#92244,0.0999999999999994) ;
#13755=CYLINDRICAL_SURFACE('',#92247,0.0999999999999994) ;
#13756=CYLINDRICAL_SURFACE('',#92257,3.) ;
#13757=CYLINDRICAL_SURFACE('',#92264,0.100000000000002) ;
#13758=CYLINDRICAL_SURFACE('',#92268,0.0999999999999997) ;
#13759=CYLINDRICAL_SURFACE('',#92270,0.0999999999999997) ;
#13760=CYLINDRICAL_SURFACE('',#92272,0.0999999999999994) ;
#13761=CYLINDRICAL_SURFACE('',#92274,0.1) ;
#13762=CYLINDRICAL_SURFACE('',#92276,0.0999999999999998) ;
#13763=CYLINDRICAL_SURFACE('',#92278,0.100000000000002) ;
#13764=CYLINDRICAL_SURFACE('',#92286,0.0999999999999994) ;
#13765=CYLINDRICAL_SURFACE('',#92288,0.0999999999999999) ;
#13766=CYLINDRICAL_SURFACE('',#92290,0.1) ;
#13767=CYLINDRICAL_SURFACE('',#92292,0.0999999999999994) ;
#13768=CYLINDRICAL_SURFACE('',#92294,0.0999999999999997) ;
#13769=CYLINDRICAL_SURFACE('',#92296,0.1) ;
#13770=CYLINDRICAL_SURFACE('',#92303,0.100000000000002) ;
#13771=CYLINDRICAL_SURFACE('',#92305,0.0999999999999999) ;
#13772=CYLINDRICAL_SURFACE('',#92307,0.0999999999999999) ;
#13773=CYLINDRICAL_SURFACE('',#92309,0.0999999999999994) ;
#13774=CYLINDRICAL_SURFACE('',#92314,0.0999999999999998) ;
#13775=CYLINDRICAL_SURFACE('',#92316,0.1) ;
#13776=CYLINDRICAL_SURFACE('',#92319,0.100000000000002) ;
#13777=CYLINDRICAL_SURFACE('',#92320,0.0999999999999994) ;
#13778=CYLINDRICAL_SURFACE('',#92321,0.0999999999999998) ;
#13779=CYLINDRICAL_SURFACE('',#92323,0.0999999999999994) ;
#13780=CYLINDRICAL_SURFACE('',#92326,0.0999999999999994) ;
#13781=CYLINDRICAL_SURFACE('',#92328,0.1) ;
#13782=CYLINDRICAL_SURFACE('',#92329,0.1) ;
#13783=CYLINDRICAL_SURFACE('',#92334,0.0999999999999994) ;
#13784=CYLINDRICAL_SURFACE('',#92335,0.0999999999999998) ;
#13785=CYLINDRICAL_SURFACE('',#92338,0.0999999999999994) ;
#13786=CYLINDRICAL_SURFACE('',#92339,0.0999999999999994) ;
#13787=CYLINDRICAL_SURFACE('',#92343,0.0999999999999994) ;
#13788=CYLINDRICAL_SURFACE('',#92345,0.0999999999999998) ;
#13789=CYLINDRICAL_SURFACE('',#92351,0.0999999999999998) ;
#13790=CYLINDRICAL_SURFACE('',#92353,0.0999999999999994) ;
#13791=CYLINDRICAL_SURFACE('',#92356,0.0999999999999998) ;
#13792=CYLINDRICAL_SURFACE('',#92365,0.0999999999999994) ;
#13793=CYLINDRICAL_SURFACE('',#92367,0.0999999999999994) ;
#13794=CYLINDRICAL_SURFACE('',#92369,0.0999999999999998) ;
#13795=CYLINDRICAL_SURFACE('',#92372,0.0999999999999994) ;
#13796=CYLINDRICAL_SURFACE('',#92374,0.0999999999999994) ;
#13797=CYLINDRICAL_SURFACE('',#92376,0.1) ;
#13798=CYLINDRICAL_SURFACE('',#92387,0.0999999999999994) ;
#13799=CYLINDRICAL_SURFACE('',#92389,0.0999999999999994) ;
#13800=CYLINDRICAL_SURFACE('',#92391,0.0999999999999994) ;
#13801=CYLINDRICAL_SURFACE('',#92393,0.0999999999999994) ;
#13802=CYLINDRICAL_SURFACE('',#92399,0.1) ;
#13803=CYLINDRICAL_SURFACE('',#92400,0.0999999999999998) ;
#13804=CYLINDRICAL_SURFACE('',#92409,0.0999999999999994) ;
#13805=CYLINDRICAL_SURFACE('',#92411,0.0999999999999994) ;
#13806=CYLINDRICAL_SURFACE('',#92413,0.0999999999999998) ;
#13807=CYLINDRICAL_SURFACE('',#92416,0.0999999999999994) ;
#13808=CYLINDRICAL_SURFACE('',#92418,0.0999999999999994) ;
#13809=CYLINDRICAL_SURFACE('',#92420,0.0999999999999998) ;
#13810=CYLINDRICAL_SURFACE('',#92431,0.0999999999999994) ;
#13811=CYLINDRICAL_SURFACE('',#92433,0.0999999999999994) ;
#13812=CYLINDRICAL_SURFACE('',#92435,0.0999999999999994) ;
#13813=CYLINDRICAL_SURFACE('',#92437,0.0999999999999994) ;
#13814=CYLINDRICAL_SURFACE('',#92443,0.0999999999999998) ;
#13815=CYLINDRICAL_SURFACE('',#92446,0.1) ;
#13816=CYLINDRICAL_SURFACE('',#92451,0.0999999999999994) ;
#13817=CYLINDRICAL_SURFACE('',#92453,0.0999999999999994) ;
#13818=CYLINDRICAL_SURFACE('',#92460,0.0999999999999994) ;
#13819=CYLINDRICAL_SURFACE('',#92464,0.0999999999999994) ;
#13820=CYLINDRICAL_SURFACE('',#92466,0.1) ;
#13821=CYLINDRICAL_SURFACE('',#92471,0.0999999999999998) ;
#13822=CYLINDRICAL_SURFACE('',#92473,0.0999999999999998) ;
#13823=CYLINDRICAL_SURFACE('',#92475,0.1) ;
#13824=CYLINDRICAL_SURFACE('',#92477,0.1) ;
#13825=CYLINDRICAL_SURFACE('',#92479,0.1) ;
#13826=CYLINDRICAL_SURFACE('',#92481,0.1) ;
#13827=CYLINDRICAL_SURFACE('',#92483,0.0999999999999995) ;
#13828=CYLINDRICAL_SURFACE('',#92484,0.0999999999999995) ;
#13829=CYLINDRICAL_SURFACE('',#92485,0.0999999999999995) ;
#13830=CYLINDRICAL_SURFACE('',#92486,0.0999999999999995) ;
#13831=CYLINDRICAL_SURFACE('',#92487,0.0999999999999998) ;
#13832=CYLINDRICAL_SURFACE('',#92489,0.0999999999999998) ;
#13833=CYLINDRICAL_SURFACE('',#92491,0.1) ;
#13834=CYLINDRICAL_SURFACE('',#92495,0.0999999999999994) ;
#13835=CYLINDRICAL_SURFACE('',#92501,0.1) ;
#13836=CYLINDRICAL_SURFACE('',#92503,0.1) ;
#13837=CYLINDRICAL_SURFACE('',#92506,0.0999999999999994) ;
#13838=CYLINDRICAL_SURFACE('',#92510,0.1) ;
#13839=CYLINDRICAL_SURFACE('',#92513,0.1) ;
#13840=CYLINDRICAL_SURFACE('',#92520,0.100000000000001) ;
#13841=CYLINDRICAL_SURFACE('',#92524,0.0999999999999994) ;
#13842=CYLINDRICAL_SURFACE('',#92528,0.100000000000001) ;
#13843=CYLINDRICAL_SURFACE('',#92532,0.0999999999999994) ;
#13844=CYLINDRICAL_SURFACE('',#92577,0.0999999999999994) ;
#13845=CYLINDRICAL_SURFACE('',#92580,0.0999999999999994) ;
#13846=CYLINDRICAL_SURFACE('',#92583,0.0999999999999994) ;
#13847=CYLINDRICAL_SURFACE('',#92586,0.0999999999999994) ;
#13848=CYLINDRICAL_SURFACE('',#92603,0.0999999999999994) ;
#13849=CYLINDRICAL_SURFACE('',#92606,0.0999999999999994) ;
#13850=CYLINDRICAL_SURFACE('',#92609,0.0999999999999994) ;
#13851=CYLINDRICAL_SURFACE('',#92612,0.0999999999999994) ;
#13852=CYLINDRICAL_SURFACE('',#92622,3.) ;
#13853=CYLINDRICAL_SURFACE('',#92629,0.1) ;
#13854=CYLINDRICAL_SURFACE('',#92633,0.0999999999999997) ;
#13855=CYLINDRICAL_SURFACE('',#92635,0.0999999999999997) ;
#13856=CYLINDRICAL_SURFACE('',#92637,0.0999999999999994) ;
#13857=CYLINDRICAL_SURFACE('',#92639,0.1) ;
#13858=CYLINDRICAL_SURFACE('',#92641,0.0999999999999998) ;
#13859=CYLINDRICAL_SURFACE('',#92643,0.100000000000002) ;
#13860=CYLINDRICAL_SURFACE('',#92651,0.0999999999999994) ;
#13861=CYLINDRICAL_SURFACE('',#92653,0.0999999999999999) ;
#13862=CYLINDRICAL_SURFACE('',#92655,0.1) ;
#13863=CYLINDRICAL_SURFACE('',#92657,0.0999999999999994) ;
#13864=CYLINDRICAL_SURFACE('',#92659,0.0999999999999997) ;
#13865=CYLINDRICAL_SURFACE('',#92661,0.1) ;
#13866=CYLINDRICAL_SURFACE('',#92668,0.0999999999999999) ;
#13867=CYLINDRICAL_SURFACE('',#92670,0.0999999999999999) ;
#13868=CYLINDRICAL_SURFACE('',#92672,0.0999999999999999) ;
#13869=CYLINDRICAL_SURFACE('',#92674,0.0999999999999994) ;
#13870=CYLINDRICAL_SURFACE('',#92679,0.0999999999999998) ;
#13871=CYLINDRICAL_SURFACE('',#92681,0.1) ;
#13872=CYLINDRICAL_SURFACE('',#92684,0.100000000000002) ;
#13873=CYLINDRICAL_SURFACE('',#92685,0.0999999999999998) ;
#13874=CYLINDRICAL_SURFACE('',#92687,0.0999999999999994) ;
#13875=CYLINDRICAL_SURFACE('',#92690,0.0999999999999994) ;
#13876=CYLINDRICAL_SURFACE('',#92692,0.1) ;
#13877=CYLINDRICAL_SURFACE('',#92693,0.1) ;
#13878=CYLINDRICAL_SURFACE('',#92698,0.0999999999999994) ;
#13879=CYLINDRICAL_SURFACE('',#92699,0.0999999999999998) ;
#13880=CYLINDRICAL_SURFACE('',#92702,0.0999999999999994) ;
#13881=CYLINDRICAL_SURFACE('',#92703,0.0999999999999994) ;
#13882=CYLINDRICAL_SURFACE('',#92707,0.0999999999999994) ;
#13883=CYLINDRICAL_SURFACE('',#92709,0.0999999999999998) ;
#13884=CYLINDRICAL_SURFACE('',#92715,0.0999999999999998) ;
#13885=CYLINDRICAL_SURFACE('',#92717,0.0999999999999994) ;
#13886=CYLINDRICAL_SURFACE('',#92720,0.0999999999999998) ;
#13887=CYLINDRICAL_SURFACE('',#92729,0.0999999999999994) ;
#13888=CYLINDRICAL_SURFACE('',#92731,0.0999999999999994) ;
#13889=CYLINDRICAL_SURFACE('',#92733,0.0999999999999998) ;
#13890=CYLINDRICAL_SURFACE('',#92736,0.0999999999999994) ;
#13891=CYLINDRICAL_SURFACE('',#92738,0.0999999999999994) ;
#13892=CYLINDRICAL_SURFACE('',#92740,0.1) ;
#13893=CYLINDRICAL_SURFACE('',#92751,0.0999999999999994) ;
#13894=CYLINDRICAL_SURFACE('',#92753,0.0999999999999994) ;
#13895=CYLINDRICAL_SURFACE('',#92755,0.0999999999999994) ;
#13896=CYLINDRICAL_SURFACE('',#92757,0.0999999999999994) ;
#13897=CYLINDRICAL_SURFACE('',#92763,0.1) ;
#13898=CYLINDRICAL_SURFACE('',#92764,0.0999999999999998) ;
#13899=CYLINDRICAL_SURFACE('',#92773,0.0999999999999994) ;
#13900=CYLINDRICAL_SURFACE('',#92775,0.0999999999999994) ;
#13901=CYLINDRICAL_SURFACE('',#92777,0.0999999999999998) ;
#13902=CYLINDRICAL_SURFACE('',#92780,0.0999999999999994) ;
#13903=CYLINDRICAL_SURFACE('',#92782,0.0999999999999994) ;
#13904=CYLINDRICAL_SURFACE('',#92784,0.0999999999999998) ;
#13905=CYLINDRICAL_SURFACE('',#92795,0.0999999999999994) ;
#13906=CYLINDRICAL_SURFACE('',#92797,0.0999999999999994) ;
#13907=CYLINDRICAL_SURFACE('',#92799,0.0999999999999994) ;
#13908=CYLINDRICAL_SURFACE('',#92801,0.0999999999999994) ;
#13909=CYLINDRICAL_SURFACE('',#92807,0.0999999999999998) ;
#13910=CYLINDRICAL_SURFACE('',#92810,0.1) ;
#13911=CYLINDRICAL_SURFACE('',#92814,0.0999999999999994) ;
#13912=CYLINDRICAL_SURFACE('',#92816,0.0999999999999994) ;
#13913=CYLINDRICAL_SURFACE('',#92824,0.0999999999999994) ;
#13914=CYLINDRICAL_SURFACE('',#92829,0.1) ;
#13915=CYLINDRICAL_SURFACE('',#92830,0.1) ;
#13916=CYLINDRICAL_SURFACE('',#92831,0.1) ;
#13917=CYLINDRICAL_SURFACE('',#92832,0.1) ;
#13918=CYLINDRICAL_SURFACE('',#92835,0.0999999999999994) ;
#13919=CYLINDRICAL_SURFACE('',#92841,0.1) ;
#13920=CYLINDRICAL_SURFACE('',#92843,0.0999999999999994) ;
#13921=CYLINDRICAL_SURFACE('',#92847,0.1) ;
#13922=CYLINDRICAL_SURFACE('',#92858,0.0999999999999994) ;
#13923=CYLINDRICAL_SURFACE('',#92860,0.1) ;
#13924=CYLINDRICAL_SURFACE('',#92862,0.1) ;
#13925=CYLINDRICAL_SURFACE('',#92864,0.0999999999999994) ;
#13926=CYLINDRICAL_SURFACE('',#92874,0.1) ;
#13927=CYLINDRICAL_SURFACE('',#92876,0.1) ;
#13928=CYLINDRICAL_SURFACE('',#92877,0.1) ;
#13929=CYLINDRICAL_SURFACE('',#92880,0.1) ;
#13930=CYLINDRICAL_SURFACE('',#92881,0.1) ;
#13931=CYLINDRICAL_SURFACE('',#92889,0.1) ;
#13932=CYLINDRICAL_SURFACE('',#92891,0.0999999999999994) ;
#13933=CYLINDRICAL_SURFACE('',#92893,0.0999999999999994) ;
#13934=CYLINDRICAL_SURFACE('',#92895,0.1) ;
#13935=CYLINDRICAL_SURFACE('',#92901,0.1) ;
#13936=CYLINDRICAL_SURFACE('',#92907,0.1) ;
#13937=CYLINDRICAL_SURFACE('',#92933,0.0999999999999994) ;
#13938=CYLINDRICAL_SURFACE('',#92941,1.5) ;
#13939=CYLINDRICAL_SURFACE('',#92942,1.9) ;
#13940=CYLINDRICAL_SURFACE('',#93051,0.0999999999999994) ;
#13941=CYLINDRICAL_SURFACE('',#93054,0.0999999999999994) ;
#13942=CYLINDRICAL_SURFACE('',#93057,0.0999999999999994) ;
#13943=CYLINDRICAL_SURFACE('',#93060,0.0999999999999994) ;
#13944=CYLINDRICAL_SURFACE('',#93077,0.0999999999999994) ;
#13945=CYLINDRICAL_SURFACE('',#93080,0.0999999999999994) ;
#13946=CYLINDRICAL_SURFACE('',#93083,0.0999999999999994) ;
#13947=CYLINDRICAL_SURFACE('',#93086,0.0999999999999994) ;
#13948=CYLINDRICAL_SURFACE('',#93096,3.) ;
#13949=CYLINDRICAL_SURFACE('',#93103,0.1) ;
#13950=CYLINDRICAL_SURFACE('',#93107,0.0999999999999997) ;
#13951=CYLINDRICAL_SURFACE('',#93109,0.0999999999999997) ;
#13952=CYLINDRICAL_SURFACE('',#93111,0.0999999999999994) ;
#13953=CYLINDRICAL_SURFACE('',#93113,0.1) ;
#13954=CYLINDRICAL_SURFACE('',#93115,0.0999999999999998) ;
#13955=CYLINDRICAL_SURFACE('',#93117,0.0999999999999999) ;
#13956=CYLINDRICAL_SURFACE('',#93125,0.0999999999999994) ;
#13957=CYLINDRICAL_SURFACE('',#93127,0.0999999999999999) ;
#13958=CYLINDRICAL_SURFACE('',#93129,0.1) ;
#13959=CYLINDRICAL_SURFACE('',#93131,0.0999999999999994) ;
#13960=CYLINDRICAL_SURFACE('',#93133,0.0999999999999997) ;
#13961=CYLINDRICAL_SURFACE('',#93135,0.1) ;
#13962=CYLINDRICAL_SURFACE('',#93142,0.0999999999999999) ;
#13963=CYLINDRICAL_SURFACE('',#93144,0.0999999999999999) ;
#13964=CYLINDRICAL_SURFACE('',#93146,0.0999999999999999) ;
#13965=CYLINDRICAL_SURFACE('',#93148,0.0999999999999994) ;
#13966=CYLINDRICAL_SURFACE('',#93153,0.0999999999999998) ;
#13967=CYLINDRICAL_SURFACE('',#93155,0.1) ;
#13968=CYLINDRICAL_SURFACE('',#93158,0.0999999999999999) ;
#13969=CYLINDRICAL_SURFACE('',#93159,0.0999999999999994) ;
#13970=CYLINDRICAL_SURFACE('',#93160,0.0999999999999998) ;
#13971=CYLINDRICAL_SURFACE('',#93162,0.0999999999999994) ;
#13972=CYLINDRICAL_SURFACE('',#93165,0.0999999999999994) ;
#13973=CYLINDRICAL_SURFACE('',#93167,0.1) ;
#13974=CYLINDRICAL_SURFACE('',#93168,0.1) ;
#13975=CYLINDRICAL_SURFACE('',#93173,0.0999999999999994) ;
#13976=CYLINDRICAL_SURFACE('',#93174,0.0999999999999998) ;
#13977=CYLINDRICAL_SURFACE('',#93177,0.0999999999999994) ;
#13978=CYLINDRICAL_SURFACE('',#93178,0.0999999999999994) ;
#13979=CYLINDRICAL_SURFACE('',#93182,0.0999999999999994) ;
#13980=CYLINDRICAL_SURFACE('',#93184,0.0999999999999998) ;
#13981=CYLINDRICAL_SURFACE('',#93190,0.0999999999999998) ;
#13982=CYLINDRICAL_SURFACE('',#93192,0.0999999999999994) ;
#13983=CYLINDRICAL_SURFACE('',#93195,0.0999999999999998) ;
#13984=CYLINDRICAL_SURFACE('',#93204,0.0999999999999994) ;
#13985=CYLINDRICAL_SURFACE('',#93206,0.0999999999999994) ;
#13986=CYLINDRICAL_SURFACE('',#93208,0.0999999999999998) ;
#13987=CYLINDRICAL_SURFACE('',#93211,0.0999999999999994) ;
#13988=CYLINDRICAL_SURFACE('',#93213,0.0999999999999994) ;
#13989=CYLINDRICAL_SURFACE('',#93215,0.1) ;
#13990=CYLINDRICAL_SURFACE('',#93226,0.0999999999999994) ;
#13991=CYLINDRICAL_SURFACE('',#93228,0.0999999999999994) ;
#13992=CYLINDRICAL_SURFACE('',#93230,0.0999999999999994) ;
#13993=CYLINDRICAL_SURFACE('',#93232,0.0999999999999994) ;
#13994=CYLINDRICAL_SURFACE('',#93238,0.1) ;
#13995=CYLINDRICAL_SURFACE('',#93239,0.0999999999999998) ;
#13996=CYLINDRICAL_SURFACE('',#93248,0.0999999999999994) ;
#13997=CYLINDRICAL_SURFACE('',#93250,0.0999999999999994) ;
#13998=CYLINDRICAL_SURFACE('',#93252,0.0999999999999998) ;
#13999=CYLINDRICAL_SURFACE('',#93255,0.0999999999999994) ;
#14000=CYLINDRICAL_SURFACE('',#93257,0.0999999999999994) ;
#14001=CYLINDRICAL_SURFACE('',#93259,0.0999999999999998) ;
#14002=CYLINDRICAL_SURFACE('',#93270,0.0999999999999994) ;
#14003=CYLINDRICAL_SURFACE('',#93272,0.0999999999999994) ;
#14004=CYLINDRICAL_SURFACE('',#93274,0.0999999999999994) ;
#14005=CYLINDRICAL_SURFACE('',#93276,0.0999999999999994) ;
#14006=CYLINDRICAL_SURFACE('',#93282,0.0999999999999998) ;
#14007=CYLINDRICAL_SURFACE('',#93285,0.1) ;
#14008=CYLINDRICAL_SURFACE('',#93289,0.0999999999999994) ;
#14009=CYLINDRICAL_SURFACE('',#93291,0.0999999999999994) ;
#14010=CYLINDRICAL_SURFACE('',#93297,0.0999999999999994) ;
#14011=CYLINDRICAL_SURFACE('',#93301,0.0999999999999994) ;
#14012=CYLINDRICAL_SURFACE('',#93303,0.1) ;
#14013=CYLINDRICAL_SURFACE('',#93308,0.0999999999999998) ;
#14014=CYLINDRICAL_SURFACE('',#93309,0.0999999999999998) ;
#14015=CYLINDRICAL_SURFACE('',#93310,0.1) ;
#14016=CYLINDRICAL_SURFACE('',#93311,0.1) ;
#14017=CYLINDRICAL_SURFACE('',#93312,0.1) ;
#14018=CYLINDRICAL_SURFACE('',#93313,0.1) ;
#14019=CYLINDRICAL_SURFACE('',#93314,0.1) ;
#14020=CYLINDRICAL_SURFACE('',#93315,0.1) ;
#14021=CYLINDRICAL_SURFACE('',#93316,0.1) ;
#14022=CYLINDRICAL_SURFACE('',#93317,0.1) ;
#14023=CYLINDRICAL_SURFACE('',#93318,0.0999999999999998) ;
#14024=CYLINDRICAL_SURFACE('',#93319,0.0999999999999998) ;
#14025=CYLINDRICAL_SURFACE('',#93320,0.0999999999999998) ;
#14026=CYLINDRICAL_SURFACE('',#93321,0.0999999999999998) ;
#14027=CYLINDRICAL_SURFACE('',#93322,0.0999999999999998) ;
#14028=CYLINDRICAL_SURFACE('',#93323,0.0999999999999998) ;
#14029=CYLINDRICAL_SURFACE('',#93324,0.1) ;
#14030=CYLINDRICAL_SURFACE('',#93327,0.0999999999999994) ;
#14031=CYLINDRICAL_SURFACE('',#93333,0.1) ;
#14032=CYLINDRICAL_SURFACE('',#93334,0.1) ;
#14033=CYLINDRICAL_SURFACE('',#93337,0.0999999999999994) ;
#14034=CYLINDRICAL_SURFACE('',#93341,0.1) ;
#14035=CYLINDRICAL_SURFACE('',#93343,0.1) ;
#16155=SPHERICAL_SURFACE('',#91148,0.1) ;
#16156=SPHERICAL_SURFACE('',#91154,0.1) ;
#16157=SPHERICAL_SURFACE('',#91194,0.1) ;
#16158=SPHERICAL_SURFACE('',#91200,0.1) ;
#16159=SPHERICAL_SURFACE('',#91391,0.1) ;
#16160=SPHERICAL_SURFACE('',#91409,0.1) ;
#16161=SPHERICAL_SURFACE('',#91412,0.1) ;
#16162=SPHERICAL_SURFACE('',#91423,0.1) ;
#16163=SPHERICAL_SURFACE('',#91451,0.1) ;
#16164=SPHERICAL_SURFACE('',#91458,0.1) ;
#16165=SPHERICAL_SURFACE('',#91460,0.1) ;
#16166=SPHERICAL_SURFACE('',#91466,0.1) ;
#16167=SPHERICAL_SURFACE('',#91492,0.1) ;
#16168=SPHERICAL_SURFACE('',#91494,0.1) ;
#16169=SPHERICAL_SURFACE('',#91506,0.1) ;
#16170=SPHERICAL_SURFACE('',#91508,0.1) ;
#16171=SPHERICAL_SURFACE('',#91536,0.1) ;
#16172=SPHERICAL_SURFACE('',#91538,0.1) ;
#16173=SPHERICAL_SURFACE('',#91550,0.1) ;
#16174=SPHERICAL_SURFACE('',#91552,0.1) ;
#16175=SPHERICAL_SURFACE('',#91559,0.1) ;
#16176=SPHERICAL_SURFACE('',#91579,0.1) ;
#16177=SPHERICAL_SURFACE('',#91604,0.1) ;
#16178=SPHERICAL_SURFACE('',#91619,0.1) ;
#16179=SPHERICAL_SURFACE('',#91756,0.1) ;
#16180=SPHERICAL_SURFACE('',#91774,0.1) ;
#16181=SPHERICAL_SURFACE('',#91777,0.1) ;
#16182=SPHERICAL_SURFACE('',#91788,0.1) ;
#16183=SPHERICAL_SURFACE('',#91815,0.1) ;
#16184=SPHERICAL_SURFACE('',#91822,0.1) ;
#16185=SPHERICAL_SURFACE('',#91824,0.1) ;
#16186=SPHERICAL_SURFACE('',#91830,0.1) ;
#16187=SPHERICAL_SURFACE('',#91856,0.1) ;
#16188=SPHERICAL_SURFACE('',#91858,0.1) ;
#16189=SPHERICAL_SURFACE('',#91870,0.1) ;
#16190=SPHERICAL_SURFACE('',#91872,0.1) ;
#16191=SPHERICAL_SURFACE('',#91900,0.1) ;
#16192=SPHERICAL_SURFACE('',#91902,0.1) ;
#16193=SPHERICAL_SURFACE('',#91914,0.1) ;
#16194=SPHERICAL_SURFACE('',#91916,0.1) ;
#16195=SPHERICAL_SURFACE('',#91921,0.1) ;
#16196=SPHERICAL_SURFACE('',#91937,0.1) ;
#16197=SPHERICAL_SURFACE('',#91944,0.1) ;
#16198=SPHERICAL_SURFACE('',#91956,0.1) ;
#16199=SPHERICAL_SURFACE('',#91963,0.1) ;
#16200=SPHERICAL_SURFACE('',#91966,0.1) ;
#16201=SPHERICAL_SURFACE('',#91977,0.1) ;
#16202=SPHERICAL_SURFACE('',#91979,0.1) ;
#16203=SPHERICAL_SURFACE('',#91981,0.1) ;
#16204=SPHERICAL_SURFACE('',#91983,0.1) ;
#16205=SPHERICAL_SURFACE('',#92037,0.1) ;
#16206=SPHERICAL_SURFACE('',#92043,0.1) ;
#16207=SPHERICAL_SURFACE('',#92083,0.1) ;
#16208=SPHERICAL_SURFACE('',#92089,0.1) ;
#16209=SPHERICAL_SURFACE('',#92280,0.1) ;
#16210=SPHERICAL_SURFACE('',#92298,0.1) ;
#16211=SPHERICAL_SURFACE('',#92301,0.1) ;
#16212=SPHERICAL_SURFACE('',#92312,0.1) ;
#16213=SPHERICAL_SURFACE('',#92340,0.1) ;
#16214=SPHERICAL_SURFACE('',#92347,0.1) ;
#16215=SPHERICAL_SURFACE('',#92349,0.1) ;
#16216=SPHERICAL_SURFACE('',#92355,0.1) ;
#16217=SPHERICAL_SURFACE('',#92381,0.1) ;
#16218=SPHERICAL_SURFACE('',#92383,0.1) ;
#16219=SPHERICAL_SURFACE('',#92395,0.1) ;
#16220=SPHERICAL_SURFACE('',#92397,0.1) ;
#16221=SPHERICAL_SURFACE('',#92425,0.1) ;
#16222=SPHERICAL_SURFACE('',#92427,0.1) ;
#16223=SPHERICAL_SURFACE('',#92439,0.1) ;
#16224=SPHERICAL_SURFACE('',#92441,0.1) ;
#16225=SPHERICAL_SURFACE('',#92449,0.1) ;
#16226=SPHERICAL_SURFACE('',#92468,0.1) ;
#16227=SPHERICAL_SURFACE('',#92493,0.1) ;
#16228=SPHERICAL_SURFACE('',#92508,0.1) ;
#16229=SPHERICAL_SURFACE('',#92645,0.1) ;
#16230=SPHERICAL_SURFACE('',#92663,0.1) ;
#16231=SPHERICAL_SURFACE('',#92666,0.1) ;
#16232=SPHERICAL_SURFACE('',#92677,0.1) ;
#16233=SPHERICAL_SURFACE('',#92704,0.1) ;
#16234=SPHERICAL_SURFACE('',#92711,0.1) ;
#16235=SPHERICAL_SURFACE('',#92713,0.1) ;
#16236=SPHERICAL_SURFACE('',#92719,0.1) ;
#16237=SPHERICAL_SURFACE('',#92745,0.1) ;
#16238=SPHERICAL_SURFACE('',#92747,0.1) ;
#16239=SPHERICAL_SURFACE('',#92759,0.1) ;
#16240=SPHERICAL_SURFACE('',#92761,0.1) ;
#16241=SPHERICAL_SURFACE('',#92789,0.1) ;
#16242=SPHERICAL_SURFACE('',#92791,0.1) ;
#16243=SPHERICAL_SURFACE('',#92803,0.1) ;
#16244=SPHERICAL_SURFACE('',#92805,0.1) ;
#16245=SPHERICAL_SURFACE('',#92812,0.1) ;
#16246=SPHERICAL_SURFACE('',#92826,0.1) ;
#16247=SPHERICAL_SURFACE('',#92833,0.1) ;
#16248=SPHERICAL_SURFACE('',#92845,0.1) ;
#16249=SPHERICAL_SURFACE('',#92852,0.1) ;
#16250=SPHERICAL_SURFACE('',#92855,0.1) ;
#16251=SPHERICAL_SURFACE('',#92866,0.1) ;
#16252=SPHERICAL_SURFACE('',#92868,0.1) ;
#16253=SPHERICAL_SURFACE('',#92870,0.1) ;
#16254=SPHERICAL_SURFACE('',#92872,0.1) ;
#16255=SPHERICAL_SURFACE('',#92929,0.1) ;
#16256=SPHERICAL_SURFACE('',#92935,0.1) ;
#16257=SPHERICAL_SURFACE('',#93119,0.1) ;
#16258=SPHERICAL_SURFACE('',#93137,0.1) ;
#16259=SPHERICAL_SURFACE('',#93140,0.1) ;
#16260=SPHERICAL_SURFACE('',#93151,0.1) ;
#16261=SPHERICAL_SURFACE('',#93179,0.1) ;
#16262=SPHERICAL_SURFACE('',#93186,0.1) ;
#16263=SPHERICAL_SURFACE('',#93188,0.1) ;
#16264=SPHERICAL_SURFACE('',#93194,0.1) ;
#16265=SPHERICAL_SURFACE('',#93220,0.1) ;
#16266=SPHERICAL_SURFACE('',#93222,0.1) ;
#16267=SPHERICAL_SURFACE('',#93234,0.1) ;
#16268=SPHERICAL_SURFACE('',#93236,0.1) ;
#16269=SPHERICAL_SURFACE('',#93264,0.1) ;
#16270=SPHERICAL_SURFACE('',#93266,0.1) ;
#16271=SPHERICAL_SURFACE('',#93278,0.1) ;
#16272=SPHERICAL_SURFACE('',#93280,0.1) ;
#16273=SPHERICAL_SURFACE('',#93287,0.1) ;
#16274=SPHERICAL_SURFACE('',#93305,0.1) ;
#16275=SPHERICAL_SURFACE('',#93325,0.1) ;
#16276=SPHERICAL_SURFACE('',#93339,0.1) ;
#17047=FACE_OUTER_BOUND('',#22763,.T.) ;
#17048=FACE_OUTER_BOUND('',#22764,.T.) ;
#17049=FACE_OUTER_BOUND('',#22765,.T.) ;
#17050=FACE_OUTER_BOUND('',#22766,.T.) ;
#17051=FACE_OUTER_BOUND('',#22767,.T.) ;
#17052=FACE_OUTER_BOUND('',#22768,.T.) ;
#17053=FACE_OUTER_BOUND('',#22769,.T.) ;
#17054=FACE_OUTER_BOUND('',#22770,.T.) ;
#17055=FACE_OUTER_BOUND('',#22771,.T.) ;
#17056=FACE_OUTER_BOUND('',#22772,.T.) ;
#17057=FACE_OUTER_BOUND('',#22773,.T.) ;
#17058=FACE_OUTER_BOUND('',#22774,.T.) ;
#17059=FACE_OUTER_BOUND('',#22775,.T.) ;
#17060=FACE_OUTER_BOUND('',#22776,.T.) ;
#17061=FACE_OUTER_BOUND('',#22777,.T.) ;
#17062=FACE_OUTER_BOUND('',#22778,.T.) ;
#17063=FACE_OUTER_BOUND('',#22779,.T.) ;
#17064=FACE_OUTER_BOUND('',#22780,.T.) ;
#17065=FACE_OUTER_BOUND('',#22781,.T.) ;
#17066=FACE_OUTER_BOUND('',#22782,.T.) ;
#17067=FACE_OUTER_BOUND('',#22783,.T.) ;
#17068=FACE_OUTER_BOUND('',#22784,.T.) ;
#17069=FACE_OUTER_BOUND('',#22785,.T.) ;
#17070=FACE_OUTER_BOUND('',#22786,.T.) ;
#17071=FACE_OUTER_BOUND('',#22788,.T.) ;
#17072=FACE_OUTER_BOUND('',#22789,.T.) ;
#17073=FACE_OUTER_BOUND('',#22790,.T.) ;
#17074=FACE_OUTER_BOUND('',#22791,.T.) ;
#17075=FACE_OUTER_BOUND('',#22792,.T.) ;
#17076=FACE_OUTER_BOUND('',#22793,.T.) ;
#17077=FACE_OUTER_BOUND('',#22794,.T.) ;
#17078=FACE_OUTER_BOUND('',#22795,.T.) ;
#17079=FACE_OUTER_BOUND('',#22796,.T.) ;
#17080=FACE_OUTER_BOUND('',#22797,.T.) ;
#17081=FACE_OUTER_BOUND('',#22798,.T.) ;
#17082=FACE_OUTER_BOUND('',#22799,.T.) ;
#17083=FACE_OUTER_BOUND('',#22802,.T.) ;
#17084=FACE_OUTER_BOUND('',#22803,.T.) ;
#17085=FACE_OUTER_BOUND('',#22804,.T.) ;
#17086=FACE_OUTER_BOUND('',#22805,.T.) ;
#17087=FACE_OUTER_BOUND('',#22806,.T.) ;
#17088=FACE_OUTER_BOUND('',#22811,.T.) ;
#17089=FACE_OUTER_BOUND('',#22812,.T.) ;
#17090=FACE_OUTER_BOUND('',#22813,.T.) ;
#17091=FACE_OUTER_BOUND('',#22814,.T.) ;
#17092=FACE_OUTER_BOUND('',#22817,.T.) ;
#17093=FACE_OUTER_BOUND('',#22820,.T.) ;
#17094=FACE_OUTER_BOUND('',#22821,.T.) ;
#17095=FACE_OUTER_BOUND('',#22822,.T.) ;
#17096=FACE_OUTER_BOUND('',#22823,.T.) ;
#17097=FACE_OUTER_BOUND('',#22824,.T.) ;
#17098=FACE_OUTER_BOUND('',#22825,.T.) ;
#17099=FACE_OUTER_BOUND('',#22826,.T.) ;
#17100=FACE_OUTER_BOUND('',#22827,.T.) ;
#17101=FACE_OUTER_BOUND('',#22828,.T.) ;
#17102=FACE_OUTER_BOUND('',#22829,.T.) ;
#17103=FACE_OUTER_BOUND('',#22830,.T.) ;
#17104=FACE_OUTER_BOUND('',#22831,.T.) ;
#17105=FACE_OUTER_BOUND('',#22832,.T.) ;
#17106=FACE_OUTER_BOUND('',#22833,.T.) ;
#17107=FACE_OUTER_BOUND('',#22834,.T.) ;
#17108=FACE_OUTER_BOUND('',#22835,.T.) ;
#17109=FACE_OUTER_BOUND('',#22836,.T.) ;
#17110=FACE_OUTER_BOUND('',#22837,.T.) ;
#17111=FACE_OUTER_BOUND('',#22838,.T.) ;
#17112=FACE_OUTER_BOUND('',#22840,.T.) ;
#17113=FACE_OUTER_BOUND('',#22841,.T.) ;
#17114=FACE_OUTER_BOUND('',#22842,.T.) ;
#17115=FACE_OUTER_BOUND('',#22843,.T.) ;
#17116=FACE_OUTER_BOUND('',#22844,.T.) ;
#17117=FACE_OUTER_BOUND('',#22845,.T.) ;
#17118=FACE_OUTER_BOUND('',#22846,.T.) ;
#17119=FACE_OUTER_BOUND('',#22847,.T.) ;
#17120=FACE_OUTER_BOUND('',#22848,.T.) ;
#17121=FACE_OUTER_BOUND('',#22849,.T.) ;
#17122=FACE_OUTER_BOUND('',#22850,.T.) ;
#17123=FACE_OUTER_BOUND('',#22851,.T.) ;
#17124=FACE_OUTER_BOUND('',#22852,.T.) ;
#17125=FACE_OUTER_BOUND('',#22853,.T.) ;
#17126=FACE_OUTER_BOUND('',#22854,.T.) ;
#17127=FACE_OUTER_BOUND('',#22855,.T.) ;
#17128=FACE_OUTER_BOUND('',#22856,.T.) ;
#17129=FACE_OUTER_BOUND('',#22857,.T.) ;
#17130=FACE_OUTER_BOUND('',#22859,.T.) ;
#17131=FACE_OUTER_BOUND('',#22860,.T.) ;
#17132=FACE_OUTER_BOUND('',#22861,.T.) ;
#17133=FACE_OUTER_BOUND('',#22862,.T.) ;
#17134=FACE_OUTER_BOUND('',#22863,.T.) ;
#17135=FACE_OUTER_BOUND('',#22864,.T.) ;
#17136=FACE_OUTER_BOUND('',#22865,.T.) ;
#17137=FACE_OUTER_BOUND('',#22866,.T.) ;
#17138=FACE_OUTER_BOUND('',#22867,.T.) ;
#17139=FACE_OUTER_BOUND('',#22868,.T.) ;
#17140=FACE_OUTER_BOUND('',#22869,.T.) ;
#17141=FACE_OUTER_BOUND('',#22870,.T.) ;
#17142=FACE_OUTER_BOUND('',#22871,.T.) ;
#17143=FACE_OUTER_BOUND('',#22872,.T.) ;
#17144=FACE_OUTER_BOUND('',#22873,.T.) ;
#17145=FACE_OUTER_BOUND('',#22874,.T.) ;
#17146=FACE_OUTER_BOUND('',#22875,.T.) ;
#17147=FACE_OUTER_BOUND('',#22876,.T.) ;
#17148=FACE_OUTER_BOUND('',#22877,.T.) ;
#17149=FACE_OUTER_BOUND('',#22878,.T.) ;
#17150=FACE_OUTER_BOUND('',#22879,.T.) ;
#17151=FACE_OUTER_BOUND('',#22880,.T.) ;
#17152=FACE_OUTER_BOUND('',#22881,.T.) ;
#17153=FACE_OUTER_BOUND('',#22882,.T.) ;
#17154=FACE_OUTER_BOUND('',#22883,.T.) ;
#17155=FACE_OUTER_BOUND('',#22884,.T.) ;
#17156=FACE_OUTER_BOUND('',#22885,.T.) ;
#17157=FACE_OUTER_BOUND('',#22886,.T.) ;
#17158=FACE_OUTER_BOUND('',#22887,.T.) ;
#17159=FACE_OUTER_BOUND('',#22888,.T.) ;
#17160=FACE_OUTER_BOUND('',#22889,.T.) ;
#17161=FACE_OUTER_BOUND('',#22890,.T.) ;
#17162=FACE_OUTER_BOUND('',#22891,.T.) ;
#17163=FACE_OUTER_BOUND('',#22892,.T.) ;
#17164=FACE_OUTER_BOUND('',#22893,.T.) ;
#17165=FACE_OUTER_BOUND('',#22894,.T.) ;
#17166=FACE_OUTER_BOUND('',#22895,.T.) ;
#17167=FACE_OUTER_BOUND('',#22896,.T.) ;
#17168=FACE_OUTER_BOUND('',#22897,.T.) ;
#17169=FACE_OUTER_BOUND('',#22898,.T.) ;
#17170=FACE_OUTER_BOUND('',#22899,.T.) ;
#17171=FACE_OUTER_BOUND('',#22900,.T.) ;
#17172=FACE_OUTER_BOUND('',#22901,.T.) ;
#17173=FACE_OUTER_BOUND('',#22902,.T.) ;
#17174=FACE_OUTER_BOUND('',#22903,.T.) ;
#17175=FACE_OUTER_BOUND('',#22904,.T.) ;
#17176=FACE_OUTER_BOUND('',#22905,.T.) ;
#17177=FACE_OUTER_BOUND('',#22906,.T.) ;
#17178=FACE_OUTER_BOUND('',#22907,.T.) ;
#17179=FACE_OUTER_BOUND('',#22908,.T.) ;
#17180=FACE_OUTER_BOUND('',#22909,.T.) ;
#17181=FACE_OUTER_BOUND('',#22910,.T.) ;
#17182=FACE_OUTER_BOUND('',#22911,.T.) ;
#17183=FACE_OUTER_BOUND('',#22912,.T.) ;
#17184=FACE_OUTER_BOUND('',#22913,.T.) ;
#17185=FACE_OUTER_BOUND('',#22914,.T.) ;
#17186=FACE_OUTER_BOUND('',#22915,.T.) ;
#17187=FACE_OUTER_BOUND('',#22916,.T.) ;
#17188=FACE_OUTER_BOUND('',#22917,.T.) ;
#17189=FACE_OUTER_BOUND('',#22918,.T.) ;
#17190=FACE_OUTER_BOUND('',#22919,.T.) ;
#17191=FACE_OUTER_BOUND('',#22920,.T.) ;
#17192=FACE_OUTER_BOUND('',#22921,.T.) ;
#17193=FACE_OUTER_BOUND('',#22922,.T.) ;
#17194=FACE_OUTER_BOUND('',#22923,.T.) ;
#17195=FACE_OUTER_BOUND('',#22924,.T.) ;
#17196=FACE_OUTER_BOUND('',#22925,.T.) ;
#17197=FACE_OUTER_BOUND('',#22926,.T.) ;
#17198=FACE_OUTER_BOUND('',#22927,.T.) ;
#17199=FACE_OUTER_BOUND('',#22928,.T.) ;
#17200=FACE_OUTER_BOUND('',#22929,.T.) ;
#17201=FACE_OUTER_BOUND('',#22930,.T.) ;
#17202=FACE_OUTER_BOUND('',#22931,.T.) ;
#17203=FACE_OUTER_BOUND('',#22932,.T.) ;
#17204=FACE_OUTER_BOUND('',#22933,.T.) ;
#17205=FACE_OUTER_BOUND('',#22934,.T.) ;
#17206=FACE_OUTER_BOUND('',#22935,.T.) ;
#17207=FACE_OUTER_BOUND('',#22936,.T.) ;
#17208=FACE_OUTER_BOUND('',#22937,.T.) ;
#17209=FACE_OUTER_BOUND('',#22938,.T.) ;
#17210=FACE_OUTER_BOUND('',#22939,.T.) ;
#17211=FACE_OUTER_BOUND('',#22940,.T.) ;
#17212=FACE_OUTER_BOUND('',#22941,.T.) ;
#17213=FACE_OUTER_BOUND('',#22942,.T.) ;
#17214=FACE_OUTER_BOUND('',#22943,.T.) ;
#17215=FACE_OUTER_BOUND('',#22944,.T.) ;
#17216=FACE_OUTER_BOUND('',#22945,.T.) ;
#17217=FACE_OUTER_BOUND('',#22946,.T.) ;
#17218=FACE_OUTER_BOUND('',#22947,.T.) ;
#17219=FACE_OUTER_BOUND('',#22948,.T.) ;
#17220=FACE_OUTER_BOUND('',#22949,.T.) ;
#17221=FACE_OUTER_BOUND('',#22950,.T.) ;
#17222=FACE_OUTER_BOUND('',#22951,.T.) ;
#17223=FACE_OUTER_BOUND('',#22952,.T.) ;
#17224=FACE_OUTER_BOUND('',#22953,.T.) ;
#17225=FACE_OUTER_BOUND('',#22954,.T.) ;
#17226=FACE_OUTER_BOUND('',#22955,.T.) ;
#17227=FACE_OUTER_BOUND('',#22956,.T.) ;
#17228=FACE_OUTER_BOUND('',#22957,.T.) ;
#17229=FACE_OUTER_BOUND('',#22958,.T.) ;
#17230=FACE_OUTER_BOUND('',#22959,.T.) ;
#17231=FACE_OUTER_BOUND('',#22960,.T.) ;
#17232=FACE_OUTER_BOUND('',#22961,.T.) ;
#17233=FACE_OUTER_BOUND('',#22962,.T.) ;
#17234=FACE_OUTER_BOUND('',#22963,.T.) ;
#17235=FACE_OUTER_BOUND('',#22964,.T.) ;
#17236=FACE_OUTER_BOUND('',#22965,.T.) ;
#17237=FACE_OUTER_BOUND('',#22966,.T.) ;
#17238=FACE_OUTER_BOUND('',#22967,.T.) ;
#17239=FACE_OUTER_BOUND('',#22968,.T.) ;
#17240=FACE_OUTER_BOUND('',#22969,.T.) ;
#17241=FACE_OUTER_BOUND('',#22970,.T.) ;
#17242=FACE_OUTER_BOUND('',#22971,.T.) ;
#17243=FACE_OUTER_BOUND('',#22972,.T.) ;
#17244=FACE_OUTER_BOUND('',#22973,.T.) ;
#17245=FACE_OUTER_BOUND('',#22974,.T.) ;
#17246=FACE_OUTER_BOUND('',#22975,.T.) ;
#17247=FACE_OUTER_BOUND('',#22976,.T.) ;
#17248=FACE_OUTER_BOUND('',#22977,.T.) ;
#17249=FACE_OUTER_BOUND('',#22978,.T.) ;
#17250=FACE_OUTER_BOUND('',#22979,.T.) ;
#17251=FACE_OUTER_BOUND('',#22980,.T.) ;
#17252=FACE_OUTER_BOUND('',#22981,.T.) ;
#17253=FACE_OUTER_BOUND('',#22982,.T.) ;
#17254=FACE_OUTER_BOUND('',#22983,.T.) ;
#17255=FACE_OUTER_BOUND('',#22984,.T.) ;
#17256=FACE_OUTER_BOUND('',#22985,.T.) ;
#17257=FACE_OUTER_BOUND('',#22986,.T.) ;
#17258=FACE_OUTER_BOUND('',#22987,.T.) ;
#17259=FACE_OUTER_BOUND('',#22988,.T.) ;
#17260=FACE_OUTER_BOUND('',#22989,.T.) ;
#17261=FACE_OUTER_BOUND('',#22990,.T.) ;
#17262=FACE_OUTER_BOUND('',#22991,.T.) ;
#17263=FACE_OUTER_BOUND('',#22992,.T.) ;
#17264=FACE_OUTER_BOUND('',#22993,.T.) ;
#17265=FACE_OUTER_BOUND('',#22994,.T.) ;
#17266=FACE_OUTER_BOUND('',#22995,.T.) ;
#17267=FACE_OUTER_BOUND('',#22996,.T.) ;
#17268=FACE_OUTER_BOUND('',#22997,.T.) ;
#17269=FACE_OUTER_BOUND('',#22998,.T.) ;
#17270=FACE_OUTER_BOUND('',#22999,.T.) ;
#17271=FACE_OUTER_BOUND('',#23000,.T.) ;
#17272=FACE_OUTER_BOUND('',#23001,.T.) ;
#17273=FACE_OUTER_BOUND('',#23002,.T.) ;
#17274=FACE_OUTER_BOUND('',#23003,.T.) ;
#17275=FACE_OUTER_BOUND('',#23004,.T.) ;
#17276=FACE_OUTER_BOUND('',#23005,.T.) ;
#17277=FACE_OUTER_BOUND('',#23006,.T.) ;
#17278=FACE_OUTER_BOUND('',#23007,.T.) ;
#17279=FACE_OUTER_BOUND('',#23008,.T.) ;
#17280=FACE_OUTER_BOUND('',#23009,.T.) ;
#17281=FACE_OUTER_BOUND('',#23010,.T.) ;
#17282=FACE_OUTER_BOUND('',#23011,.T.) ;
#17283=FACE_OUTER_BOUND('',#23012,.T.) ;
#17284=FACE_OUTER_BOUND('',#23013,.T.) ;
#17285=FACE_OUTER_BOUND('',#23014,.T.) ;
#17286=FACE_OUTER_BOUND('',#23015,.T.) ;
#17287=FACE_OUTER_BOUND('',#23016,.T.) ;
#17288=FACE_OUTER_BOUND('',#23017,.T.) ;
#17289=FACE_OUTER_BOUND('',#23018,.T.) ;
#17290=FACE_OUTER_BOUND('',#23019,.T.) ;
#17291=FACE_OUTER_BOUND('',#23020,.T.) ;
#17292=FACE_OUTER_BOUND('',#23021,.T.) ;
#17293=FACE_OUTER_BOUND('',#23022,.T.) ;
#17294=FACE_OUTER_BOUND('',#23023,.T.) ;
#17295=FACE_OUTER_BOUND('',#23024,.T.) ;
#17296=FACE_OUTER_BOUND('',#23025,.T.) ;
#17297=FACE_OUTER_BOUND('',#23026,.T.) ;
#17298=FACE_OUTER_BOUND('',#23027,.T.) ;
#17299=FACE_OUTER_BOUND('',#23028,.T.) ;
#17300=FACE_OUTER_BOUND('',#23029,.T.) ;
#17301=FACE_OUTER_BOUND('',#23030,.T.) ;
#17302=FACE_OUTER_BOUND('',#23031,.T.) ;
#17303=FACE_OUTER_BOUND('',#23032,.T.) ;
#17304=FACE_OUTER_BOUND('',#23033,.T.) ;
#17305=FACE_OUTER_BOUND('',#23034,.T.) ;
#17306=FACE_OUTER_BOUND('',#23035,.T.) ;
#17307=FACE_OUTER_BOUND('',#23036,.T.) ;
#17308=FACE_OUTER_BOUND('',#23037,.T.) ;
#17309=FACE_OUTER_BOUND('',#23038,.T.) ;
#17310=FACE_OUTER_BOUND('',#23039,.T.) ;
#17311=FACE_OUTER_BOUND('',#23040,.T.) ;
#17312=FACE_OUTER_BOUND('',#23041,.T.) ;
#17313=FACE_OUTER_BOUND('',#23043,.T.) ;
#17314=FACE_OUTER_BOUND('',#23044,.T.) ;
#17315=FACE_OUTER_BOUND('',#23045,.T.) ;
#17316=FACE_OUTER_BOUND('',#23046,.T.) ;
#17317=FACE_OUTER_BOUND('',#23047,.T.) ;
#17318=FACE_OUTER_BOUND('',#23048,.T.) ;
#17319=FACE_OUTER_BOUND('',#23049,.T.) ;
#17320=FACE_OUTER_BOUND('',#23050,.T.) ;
#17321=FACE_OUTER_BOUND('',#23051,.T.) ;
#17322=FACE_OUTER_BOUND('',#23052,.T.) ;
#17323=FACE_OUTER_BOUND('',#23053,.T.) ;
#17324=FACE_OUTER_BOUND('',#23054,.T.) ;
#17325=FACE_OUTER_BOUND('',#23055,.T.) ;
#17326=FACE_OUTER_BOUND('',#23056,.T.) ;
#17327=FACE_OUTER_BOUND('',#23057,.T.) ;
#17328=FACE_OUTER_BOUND('',#23058,.T.) ;
#17329=FACE_OUTER_BOUND('',#23059,.T.) ;
#17330=FACE_OUTER_BOUND('',#23060,.T.) ;
#17331=FACE_OUTER_BOUND('',#23062,.T.) ;
#17332=FACE_OUTER_BOUND('',#23063,.T.) ;
#17333=FACE_OUTER_BOUND('',#23064,.T.) ;
#17334=FACE_OUTER_BOUND('',#23065,.T.) ;
#17335=FACE_OUTER_BOUND('',#23066,.T.) ;
#17336=FACE_OUTER_BOUND('',#23067,.T.) ;
#17337=FACE_OUTER_BOUND('',#23068,.T.) ;
#17338=FACE_OUTER_BOUND('',#23069,.T.) ;
#17339=FACE_OUTER_BOUND('',#23070,.T.) ;
#17340=FACE_OUTER_BOUND('',#23071,.T.) ;
#17341=FACE_OUTER_BOUND('',#23072,.T.) ;
#17342=FACE_OUTER_BOUND('',#23073,.T.) ;
#17343=FACE_OUTER_BOUND('',#23074,.T.) ;
#17344=FACE_OUTER_BOUND('',#23075,.T.) ;
#17345=FACE_OUTER_BOUND('',#23076,.T.) ;
#17346=FACE_OUTER_BOUND('',#23077,.T.) ;
#17347=FACE_OUTER_BOUND('',#23078,.T.) ;
#17348=FACE_OUTER_BOUND('',#23079,.T.) ;
#17349=FACE_OUTER_BOUND('',#23080,.T.) ;
#17350=FACE_OUTER_BOUND('',#23081,.T.) ;
#17351=FACE_OUTER_BOUND('',#23082,.T.) ;
#17352=FACE_OUTER_BOUND('',#23083,.T.) ;
#17353=FACE_OUTER_BOUND('',#23084,.T.) ;
#17354=FACE_OUTER_BOUND('',#23085,.T.) ;
#17355=FACE_OUTER_BOUND('',#23086,.T.) ;
#17356=FACE_OUTER_BOUND('',#23087,.T.) ;
#17357=FACE_OUTER_BOUND('',#23088,.T.) ;
#17358=FACE_OUTER_BOUND('',#23089,.T.) ;
#17359=FACE_OUTER_BOUND('',#23090,.T.) ;
#17360=FACE_OUTER_BOUND('',#23091,.T.) ;
#17361=FACE_OUTER_BOUND('',#23092,.T.) ;
#17362=FACE_OUTER_BOUND('',#23093,.T.) ;
#17363=FACE_OUTER_BOUND('',#23094,.T.) ;
#17364=FACE_OUTER_BOUND('',#23095,.T.) ;
#17365=FACE_OUTER_BOUND('',#23096,.T.) ;
#17366=FACE_OUTER_BOUND('',#23097,.T.) ;
#17367=FACE_OUTER_BOUND('',#23098,.T.) ;
#17368=FACE_OUTER_BOUND('',#23099,.T.) ;
#17369=FACE_OUTER_BOUND('',#23100,.T.) ;
#17370=FACE_OUTER_BOUND('',#23101,.T.) ;
#17371=FACE_OUTER_BOUND('',#23102,.T.) ;
#17372=FACE_OUTER_BOUND('',#23103,.T.) ;
#17373=FACE_OUTER_BOUND('',#23104,.T.) ;
#17374=FACE_OUTER_BOUND('',#23105,.T.) ;
#17375=FACE_OUTER_BOUND('',#23106,.T.) ;
#17376=FACE_OUTER_BOUND('',#23107,.T.) ;
#17377=FACE_OUTER_BOUND('',#23108,.T.) ;
#17378=FACE_OUTER_BOUND('',#23109,.T.) ;
#17379=FACE_OUTER_BOUND('',#23110,.T.) ;
#17380=FACE_OUTER_BOUND('',#23111,.T.) ;
#17381=FACE_OUTER_BOUND('',#23112,.T.) ;
#17382=FACE_OUTER_BOUND('',#23113,.T.) ;
#17383=FACE_OUTER_BOUND('',#23114,.T.) ;
#17384=FACE_OUTER_BOUND('',#23115,.T.) ;
#17385=FACE_OUTER_BOUND('',#23116,.T.) ;
#17386=FACE_OUTER_BOUND('',#23117,.T.) ;
#17387=FACE_OUTER_BOUND('',#23118,.T.) ;
#17388=FACE_OUTER_BOUND('',#23119,.T.) ;
#17389=FACE_OUTER_BOUND('',#23120,.T.) ;
#17390=FACE_OUTER_BOUND('',#23121,.T.) ;
#17391=FACE_OUTER_BOUND('',#23122,.T.) ;
#17392=FACE_OUTER_BOUND('',#23123,.T.) ;
#17393=FACE_OUTER_BOUND('',#23124,.T.) ;
#17394=FACE_OUTER_BOUND('',#23125,.T.) ;
#17395=FACE_OUTER_BOUND('',#23126,.T.) ;
#17396=FACE_OUTER_BOUND('',#23127,.T.) ;
#17397=FACE_OUTER_BOUND('',#23128,.T.) ;
#17398=FACE_OUTER_BOUND('',#23129,.T.) ;
#17399=FACE_OUTER_BOUND('',#23130,.T.) ;
#17400=FACE_OUTER_BOUND('',#23131,.T.) ;
#17401=FACE_OUTER_BOUND('',#23132,.T.) ;
#17402=FACE_OUTER_BOUND('',#23133,.T.) ;
#17403=FACE_OUTER_BOUND('',#23134,.T.) ;
#17404=FACE_OUTER_BOUND('',#23135,.T.) ;
#17405=FACE_OUTER_BOUND('',#23136,.T.) ;
#17406=FACE_OUTER_BOUND('',#23137,.T.) ;
#17407=FACE_OUTER_BOUND('',#23138,.T.) ;
#17408=FACE_OUTER_BOUND('',#23139,.T.) ;
#17409=FACE_OUTER_BOUND('',#23140,.T.) ;
#17410=FACE_OUTER_BOUND('',#23141,.T.) ;
#17411=FACE_OUTER_BOUND('',#23142,.T.) ;
#17412=FACE_OUTER_BOUND('',#23143,.T.) ;
#17413=FACE_OUTER_BOUND('',#23144,.T.) ;
#17414=FACE_OUTER_BOUND('',#23145,.T.) ;
#17415=FACE_OUTER_BOUND('',#23146,.T.) ;
#17416=FACE_OUTER_BOUND('',#23147,.T.) ;
#17417=FACE_OUTER_BOUND('',#23148,.T.) ;
#17418=FACE_OUTER_BOUND('',#23149,.T.) ;
#17419=FACE_OUTER_BOUND('',#23150,.T.) ;
#17420=FACE_OUTER_BOUND('',#23151,.T.) ;
#17421=FACE_OUTER_BOUND('',#23152,.T.) ;
#17422=FACE_OUTER_BOUND('',#23153,.T.) ;
#17423=FACE_OUTER_BOUND('',#23154,.T.) ;
#17424=FACE_OUTER_BOUND('',#23155,.T.) ;
#17425=FACE_OUTER_BOUND('',#23156,.T.) ;
#17426=FACE_OUTER_BOUND('',#23157,.T.) ;
#17427=FACE_OUTER_BOUND('',#23158,.T.) ;
#17428=FACE_OUTER_BOUND('',#23159,.T.) ;
#17429=FACE_OUTER_BOUND('',#23160,.T.) ;
#17430=FACE_OUTER_BOUND('',#23161,.T.) ;
#17431=FACE_OUTER_BOUND('',#23162,.T.) ;
#17432=FACE_OUTER_BOUND('',#23163,.T.) ;
#17433=FACE_OUTER_BOUND('',#23164,.T.) ;
#17434=FACE_OUTER_BOUND('',#23165,.T.) ;
#17435=FACE_OUTER_BOUND('',#23166,.T.) ;
#17436=FACE_OUTER_BOUND('',#23167,.T.) ;
#17437=FACE_OUTER_BOUND('',#23168,.T.) ;
#17438=FACE_OUTER_BOUND('',#23169,.T.) ;
#17439=FACE_OUTER_BOUND('',#23170,.T.) ;
#17440=FACE_OUTER_BOUND('',#23171,.T.) ;
#17441=FACE_OUTER_BOUND('',#23172,.T.) ;
#17442=FACE_OUTER_BOUND('',#23173,.T.) ;
#17443=FACE_OUTER_BOUND('',#23174,.T.) ;
#17444=FACE_OUTER_BOUND('',#23175,.T.) ;
#17445=FACE_OUTER_BOUND('',#23176,.T.) ;
#17446=FACE_OUTER_BOUND('',#23177,.T.) ;
#17447=FACE_OUTER_BOUND('',#23178,.T.) ;
#17448=FACE_OUTER_BOUND('',#23179,.T.) ;
#17449=FACE_OUTER_BOUND('',#23180,.T.) ;
#17450=FACE_OUTER_BOUND('',#23181,.T.) ;
#17451=FACE_OUTER_BOUND('',#23182,.T.) ;
#17452=FACE_OUTER_BOUND('',#23183,.T.) ;
#17453=FACE_OUTER_BOUND('',#23184,.T.) ;
#17454=FACE_OUTER_BOUND('',#23185,.T.) ;
#17455=FACE_OUTER_BOUND('',#23186,.T.) ;
#17456=FACE_OUTER_BOUND('',#23187,.T.) ;
#17457=FACE_OUTER_BOUND('',#23188,.T.) ;
#17458=FACE_OUTER_BOUND('',#23189,.T.) ;
#17459=FACE_OUTER_BOUND('',#23190,.T.) ;
#17460=FACE_OUTER_BOUND('',#23191,.T.) ;
#17461=FACE_OUTER_BOUND('',#23192,.T.) ;
#17462=FACE_OUTER_BOUND('',#23193,.T.) ;
#17463=FACE_OUTER_BOUND('',#23194,.T.) ;
#17464=FACE_OUTER_BOUND('',#23195,.T.) ;
#17465=FACE_OUTER_BOUND('',#23196,.T.) ;
#17466=FACE_OUTER_BOUND('',#23197,.T.) ;
#17467=FACE_OUTER_BOUND('',#23198,.T.) ;
#17468=FACE_OUTER_BOUND('',#23199,.T.) ;
#17469=FACE_OUTER_BOUND('',#23200,.T.) ;
#17470=FACE_OUTER_BOUND('',#23201,.T.) ;
#17471=FACE_OUTER_BOUND('',#23202,.T.) ;
#17472=FACE_OUTER_BOUND('',#23203,.T.) ;
#17473=FACE_OUTER_BOUND('',#23204,.T.) ;
#17474=FACE_OUTER_BOUND('',#23205,.T.) ;
#17475=FACE_OUTER_BOUND('',#23206,.T.) ;
#17476=FACE_OUTER_BOUND('',#23207,.T.) ;
#17477=FACE_OUTER_BOUND('',#23208,.T.) ;
#17478=FACE_OUTER_BOUND('',#23209,.T.) ;
#17479=FACE_OUTER_BOUND('',#23210,.T.) ;
#17480=FACE_OUTER_BOUND('',#23211,.T.) ;
#17481=FACE_OUTER_BOUND('',#23212,.T.) ;
#17482=FACE_OUTER_BOUND('',#23213,.T.) ;
#17483=FACE_OUTER_BOUND('',#23214,.T.) ;
#17484=FACE_OUTER_BOUND('',#23215,.T.) ;
#17485=FACE_OUTER_BOUND('',#23216,.T.) ;
#17486=FACE_OUTER_BOUND('',#23217,.T.) ;
#17487=FACE_OUTER_BOUND('',#23218,.T.) ;
#17488=FACE_OUTER_BOUND('',#23219,.T.) ;
#17489=FACE_OUTER_BOUND('',#23220,.T.) ;
#17490=FACE_OUTER_BOUND('',#23221,.T.) ;
#17491=FACE_OUTER_BOUND('',#23222,.T.) ;
#17492=FACE_OUTER_BOUND('',#23223,.T.) ;
#17493=FACE_OUTER_BOUND('',#23224,.T.) ;
#17494=FACE_OUTER_BOUND('',#23225,.T.) ;
#17495=FACE_OUTER_BOUND('',#23226,.T.) ;
#17496=FACE_OUTER_BOUND('',#23227,.T.) ;
#17497=FACE_OUTER_BOUND('',#23228,.T.) ;
#17498=FACE_OUTER_BOUND('',#23229,.T.) ;
#17499=FACE_OUTER_BOUND('',#23230,.T.) ;
#17500=FACE_OUTER_BOUND('',#23231,.T.) ;
#17501=FACE_OUTER_BOUND('',#23232,.T.) ;
#17502=FACE_OUTER_BOUND('',#23233,.T.) ;
#17503=FACE_OUTER_BOUND('',#23234,.T.) ;
#17504=FACE_OUTER_BOUND('',#23235,.T.) ;
#17505=FACE_OUTER_BOUND('',#23236,.T.) ;
#17506=FACE_OUTER_BOUND('',#23237,.T.) ;
#17507=FACE_OUTER_BOUND('',#23238,.T.) ;
#17508=FACE_OUTER_BOUND('',#23239,.T.) ;
#17509=FACE_OUTER_BOUND('',#23240,.T.) ;
#17510=FACE_OUTER_BOUND('',#23241,.T.) ;
#17511=FACE_OUTER_BOUND('',#23242,.T.) ;
#17512=FACE_OUTER_BOUND('',#23243,.T.) ;
#17513=FACE_OUTER_BOUND('',#23244,.T.) ;
#17514=FACE_OUTER_BOUND('',#23245,.T.) ;
#17515=FACE_OUTER_BOUND('',#23246,.T.) ;
#17516=FACE_OUTER_BOUND('',#23247,.T.) ;
#17517=FACE_OUTER_BOUND('',#23248,.T.) ;
#17518=FACE_OUTER_BOUND('',#23249,.T.) ;
#17519=FACE_OUTER_BOUND('',#23251,.T.) ;
#17520=FACE_OUTER_BOUND('',#23252,.T.) ;
#17521=FACE_OUTER_BOUND('',#23253,.T.) ;
#17522=FACE_OUTER_BOUND('',#23254,.T.) ;
#17523=FACE_OUTER_BOUND('',#23255,.T.) ;
#17524=FACE_OUTER_BOUND('',#23256,.T.) ;
#17525=FACE_OUTER_BOUND('',#23257,.T.) ;
#17526=FACE_OUTER_BOUND('',#23258,.T.) ;
#17527=FACE_OUTER_BOUND('',#23259,.T.) ;
#17528=FACE_OUTER_BOUND('',#23260,.T.) ;
#17529=FACE_OUTER_BOUND('',#23261,.T.) ;
#17530=FACE_OUTER_BOUND('',#23262,.T.) ;
#17531=FACE_OUTER_BOUND('',#23265,.T.) ;
#17532=FACE_OUTER_BOUND('',#23266,.T.) ;
#17533=FACE_OUTER_BOUND('',#23267,.T.) ;
#17534=FACE_OUTER_BOUND('',#23268,.T.) ;
#17535=FACE_OUTER_BOUND('',#23269,.T.) ;
#17536=FACE_OUTER_BOUND('',#23274,.T.) ;
#17537=FACE_OUTER_BOUND('',#23275,.T.) ;
#17538=FACE_OUTER_BOUND('',#23276,.T.) ;
#17539=FACE_OUTER_BOUND('',#23277,.T.) ;
#17540=FACE_OUTER_BOUND('',#23280,.T.) ;
#17541=FACE_OUTER_BOUND('',#23283,.T.) ;
#17542=FACE_OUTER_BOUND('',#23284,.T.) ;
#17543=FACE_OUTER_BOUND('',#23285,.T.) ;
#17544=FACE_OUTER_BOUND('',#23286,.T.) ;
#17545=FACE_OUTER_BOUND('',#23287,.T.) ;
#17546=FACE_OUTER_BOUND('',#23288,.T.) ;
#17547=FACE_OUTER_BOUND('',#23289,.T.) ;
#17548=FACE_OUTER_BOUND('',#23290,.T.) ;
#17549=FACE_OUTER_BOUND('',#23291,.T.) ;
#17550=FACE_OUTER_BOUND('',#23292,.T.) ;
#17551=FACE_OUTER_BOUND('',#23293,.T.) ;
#17552=FACE_OUTER_BOUND('',#23294,.T.) ;
#17553=FACE_OUTER_BOUND('',#23295,.T.) ;
#17554=FACE_OUTER_BOUND('',#23296,.T.) ;
#17555=FACE_OUTER_BOUND('',#23297,.T.) ;
#17556=FACE_OUTER_BOUND('',#23298,.T.) ;
#17557=FACE_OUTER_BOUND('',#23299,.T.) ;
#17558=FACE_OUTER_BOUND('',#23300,.T.) ;
#17559=FACE_OUTER_BOUND('',#23301,.T.) ;
#17560=FACE_OUTER_BOUND('',#23303,.T.) ;
#17561=FACE_OUTER_BOUND('',#23304,.T.) ;
#17562=FACE_OUTER_BOUND('',#23305,.T.) ;
#17563=FACE_OUTER_BOUND('',#23306,.T.) ;
#17564=FACE_OUTER_BOUND('',#23307,.T.) ;
#17565=FACE_OUTER_BOUND('',#23308,.T.) ;
#17566=FACE_OUTER_BOUND('',#23309,.T.) ;
#17567=FACE_OUTER_BOUND('',#23310,.T.) ;
#17568=FACE_OUTER_BOUND('',#23311,.T.) ;
#17569=FACE_OUTER_BOUND('',#23312,.T.) ;
#17570=FACE_OUTER_BOUND('',#23313,.T.) ;
#17571=FACE_OUTER_BOUND('',#23314,.T.) ;
#17572=FACE_OUTER_BOUND('',#23315,.T.) ;
#17573=FACE_OUTER_BOUND('',#23316,.T.) ;
#17574=FACE_OUTER_BOUND('',#23317,.T.) ;
#17575=FACE_OUTER_BOUND('',#23318,.T.) ;
#17576=FACE_OUTER_BOUND('',#23319,.T.) ;
#17577=FACE_OUTER_BOUND('',#23320,.T.) ;
#17578=FACE_OUTER_BOUND('',#23322,.T.) ;
#17579=FACE_OUTER_BOUND('',#23323,.T.) ;
#17580=FACE_OUTER_BOUND('',#23324,.T.) ;
#17581=FACE_OUTER_BOUND('',#23325,.T.) ;
#17582=FACE_OUTER_BOUND('',#23326,.T.) ;
#17583=FACE_OUTER_BOUND('',#23327,.T.) ;
#17584=FACE_OUTER_BOUND('',#23328,.T.) ;
#17585=FACE_OUTER_BOUND('',#23329,.T.) ;
#17586=FACE_OUTER_BOUND('',#23330,.T.) ;
#17587=FACE_OUTER_BOUND('',#23331,.T.) ;
#17588=FACE_OUTER_BOUND('',#23332,.T.) ;
#17589=FACE_OUTER_BOUND('',#23333,.T.) ;
#17590=FACE_OUTER_BOUND('',#23334,.T.) ;
#17591=FACE_OUTER_BOUND('',#23335,.T.) ;
#17592=FACE_OUTER_BOUND('',#23336,.T.) ;
#17593=FACE_OUTER_BOUND('',#23337,.T.) ;
#17594=FACE_OUTER_BOUND('',#23338,.T.) ;
#17595=FACE_OUTER_BOUND('',#23339,.T.) ;
#17596=FACE_OUTER_BOUND('',#23340,.T.) ;
#17597=FACE_OUTER_BOUND('',#23341,.T.) ;
#17598=FACE_OUTER_BOUND('',#23342,.T.) ;
#17599=FACE_OUTER_BOUND('',#23343,.T.) ;
#17600=FACE_OUTER_BOUND('',#23344,.T.) ;
#17601=FACE_OUTER_BOUND('',#23345,.T.) ;
#17602=FACE_OUTER_BOUND('',#23346,.T.) ;
#17603=FACE_OUTER_BOUND('',#23347,.T.) ;
#17604=FACE_OUTER_BOUND('',#23348,.T.) ;
#17605=FACE_OUTER_BOUND('',#23349,.T.) ;
#17606=FACE_OUTER_BOUND('',#23350,.T.) ;
#17607=FACE_OUTER_BOUND('',#23351,.T.) ;
#17608=FACE_OUTER_BOUND('',#23352,.T.) ;
#17609=FACE_OUTER_BOUND('',#23353,.T.) ;
#17610=FACE_OUTER_BOUND('',#23354,.T.) ;
#17611=FACE_OUTER_BOUND('',#23355,.T.) ;
#17612=FACE_OUTER_BOUND('',#23356,.T.) ;
#17613=FACE_OUTER_BOUND('',#23357,.T.) ;
#17614=FACE_OUTER_BOUND('',#23358,.T.) ;
#17615=FACE_OUTER_BOUND('',#23359,.T.) ;
#17616=FACE_OUTER_BOUND('',#23360,.T.) ;
#17617=FACE_OUTER_BOUND('',#23361,.T.) ;
#17618=FACE_OUTER_BOUND('',#23362,.T.) ;
#17619=FACE_OUTER_BOUND('',#23363,.T.) ;
#17620=FACE_OUTER_BOUND('',#23364,.T.) ;
#17621=FACE_OUTER_BOUND('',#23365,.T.) ;
#17622=FACE_OUTER_BOUND('',#23366,.T.) ;
#17623=FACE_OUTER_BOUND('',#23367,.T.) ;
#17624=FACE_OUTER_BOUND('',#23368,.T.) ;
#17625=FACE_OUTER_BOUND('',#23369,.T.) ;
#17626=FACE_OUTER_BOUND('',#23370,.T.) ;
#17627=FACE_OUTER_BOUND('',#23371,.T.) ;
#17628=FACE_OUTER_BOUND('',#23372,.T.) ;
#17629=FACE_OUTER_BOUND('',#23373,.T.) ;
#17630=FACE_OUTER_BOUND('',#23374,.T.) ;
#17631=FACE_OUTER_BOUND('',#23375,.T.) ;
#17632=FACE_OUTER_BOUND('',#23376,.T.) ;
#17633=FACE_OUTER_BOUND('',#23377,.T.) ;
#17634=FACE_OUTER_BOUND('',#23378,.T.) ;
#17635=FACE_OUTER_BOUND('',#23379,.T.) ;
#17636=FACE_OUTER_BOUND('',#23380,.T.) ;
#17637=FACE_OUTER_BOUND('',#23381,.T.) ;
#17638=FACE_OUTER_BOUND('',#23382,.T.) ;
#17639=FACE_OUTER_BOUND('',#23383,.T.) ;
#17640=FACE_OUTER_BOUND('',#23384,.T.) ;
#17641=FACE_OUTER_BOUND('',#23385,.T.) ;
#17642=FACE_OUTER_BOUND('',#23386,.T.) ;
#17643=FACE_OUTER_BOUND('',#23387,.T.) ;
#17644=FACE_OUTER_BOUND('',#23388,.T.) ;
#17645=FACE_OUTER_BOUND('',#23389,.T.) ;
#17646=FACE_OUTER_BOUND('',#23390,.T.) ;
#17647=FACE_OUTER_BOUND('',#23391,.T.) ;
#17648=FACE_OUTER_BOUND('',#23392,.T.) ;
#17649=FACE_OUTER_BOUND('',#23393,.T.) ;
#17650=FACE_OUTER_BOUND('',#23394,.T.) ;
#17651=FACE_OUTER_BOUND('',#23395,.T.) ;
#17652=FACE_OUTER_BOUND('',#23396,.T.) ;
#17653=FACE_OUTER_BOUND('',#23397,.T.) ;
#17654=FACE_OUTER_BOUND('',#23398,.T.) ;
#17655=FACE_OUTER_BOUND('',#23399,.T.) ;
#17656=FACE_OUTER_BOUND('',#23400,.T.) ;
#17657=FACE_OUTER_BOUND('',#23401,.T.) ;
#17658=FACE_OUTER_BOUND('',#23402,.T.) ;
#17659=FACE_OUTER_BOUND('',#23403,.T.) ;
#17660=FACE_OUTER_BOUND('',#23404,.T.) ;
#17661=FACE_OUTER_BOUND('',#23405,.T.) ;
#17662=FACE_OUTER_BOUND('',#23406,.T.) ;
#17663=FACE_OUTER_BOUND('',#23407,.T.) ;
#17664=FACE_OUTER_BOUND('',#23408,.T.) ;
#17665=FACE_OUTER_BOUND('',#23409,.T.) ;
#17666=FACE_OUTER_BOUND('',#23410,.T.) ;
#17667=FACE_OUTER_BOUND('',#23411,.T.) ;
#17668=FACE_OUTER_BOUND('',#23412,.T.) ;
#17669=FACE_OUTER_BOUND('',#23413,.T.) ;
#17670=FACE_OUTER_BOUND('',#23414,.T.) ;
#17671=FACE_OUTER_BOUND('',#23415,.T.) ;
#17672=FACE_OUTER_BOUND('',#23416,.T.) ;
#17673=FACE_OUTER_BOUND('',#23417,.T.) ;
#17674=FACE_OUTER_BOUND('',#23418,.T.) ;
#17675=FACE_OUTER_BOUND('',#23419,.T.) ;
#17676=FACE_OUTER_BOUND('',#23420,.T.) ;
#17677=FACE_OUTER_BOUND('',#23421,.T.) ;
#17678=FACE_OUTER_BOUND('',#23422,.T.) ;
#17679=FACE_OUTER_BOUND('',#23423,.T.) ;
#17680=FACE_OUTER_BOUND('',#23424,.T.) ;
#17681=FACE_OUTER_BOUND('',#23425,.T.) ;
#17682=FACE_OUTER_BOUND('',#23426,.T.) ;
#17683=FACE_OUTER_BOUND('',#23427,.T.) ;
#17684=FACE_OUTER_BOUND('',#23428,.T.) ;
#17685=FACE_OUTER_BOUND('',#23429,.T.) ;
#17686=FACE_OUTER_BOUND('',#23430,.T.) ;
#17687=FACE_OUTER_BOUND('',#23431,.T.) ;
#17688=FACE_OUTER_BOUND('',#23432,.T.) ;
#17689=FACE_OUTER_BOUND('',#23433,.T.) ;
#17690=FACE_OUTER_BOUND('',#23434,.T.) ;
#17691=FACE_OUTER_BOUND('',#23435,.T.) ;
#17692=FACE_OUTER_BOUND('',#23436,.T.) ;
#17693=FACE_OUTER_BOUND('',#23437,.T.) ;
#17694=FACE_OUTER_BOUND('',#23438,.T.) ;
#17695=FACE_OUTER_BOUND('',#23439,.T.) ;
#17696=FACE_OUTER_BOUND('',#23440,.T.) ;
#17697=FACE_OUTER_BOUND('',#23441,.T.) ;
#17698=FACE_OUTER_BOUND('',#23442,.T.) ;
#17699=FACE_OUTER_BOUND('',#23443,.T.) ;
#17700=FACE_OUTER_BOUND('',#23444,.T.) ;
#17701=FACE_OUTER_BOUND('',#23445,.T.) ;
#17702=FACE_OUTER_BOUND('',#23446,.T.) ;
#17703=FACE_OUTER_BOUND('',#23447,.T.) ;
#17704=FACE_OUTER_BOUND('',#23448,.T.) ;
#17705=FACE_OUTER_BOUND('',#23449,.T.) ;
#17706=FACE_OUTER_BOUND('',#23450,.T.) ;
#17707=FACE_OUTER_BOUND('',#23451,.T.) ;
#17708=FACE_OUTER_BOUND('',#23452,.T.) ;
#17709=FACE_OUTER_BOUND('',#23453,.T.) ;
#17710=FACE_OUTER_BOUND('',#23454,.T.) ;
#17711=FACE_OUTER_BOUND('',#23455,.T.) ;
#17712=FACE_OUTER_BOUND('',#23456,.T.) ;
#17713=FACE_OUTER_BOUND('',#23457,.T.) ;
#17714=FACE_OUTER_BOUND('',#23458,.T.) ;
#17715=FACE_OUTER_BOUND('',#23459,.T.) ;
#17716=FACE_OUTER_BOUND('',#23460,.T.) ;
#17717=FACE_OUTER_BOUND('',#23461,.T.) ;
#17718=FACE_OUTER_BOUND('',#23462,.T.) ;
#17719=FACE_OUTER_BOUND('',#23463,.T.) ;
#17720=FACE_OUTER_BOUND('',#23464,.T.) ;
#17721=FACE_OUTER_BOUND('',#23465,.T.) ;
#17722=FACE_OUTER_BOUND('',#23466,.T.) ;
#17723=FACE_OUTER_BOUND('',#23467,.T.) ;
#17724=FACE_OUTER_BOUND('',#23468,.T.) ;
#17725=FACE_OUTER_BOUND('',#23469,.T.) ;
#17726=FACE_OUTER_BOUND('',#23470,.T.) ;
#17727=FACE_OUTER_BOUND('',#23471,.T.) ;
#17728=FACE_OUTER_BOUND('',#23472,.T.) ;
#17729=FACE_OUTER_BOUND('',#23473,.T.) ;
#17730=FACE_OUTER_BOUND('',#23474,.T.) ;
#17731=FACE_OUTER_BOUND('',#23475,.T.) ;
#17732=FACE_OUTER_BOUND('',#23476,.T.) ;
#17733=FACE_OUTER_BOUND('',#23477,.T.) ;
#17734=FACE_OUTER_BOUND('',#23478,.T.) ;
#17735=FACE_OUTER_BOUND('',#23479,.T.) ;
#17736=FACE_OUTER_BOUND('',#23480,.T.) ;
#17737=FACE_OUTER_BOUND('',#23481,.T.) ;
#17738=FACE_OUTER_BOUND('',#23482,.T.) ;
#17739=FACE_OUTER_BOUND('',#23483,.T.) ;
#17740=FACE_OUTER_BOUND('',#23484,.T.) ;
#17741=FACE_OUTER_BOUND('',#23485,.T.) ;
#17742=FACE_OUTER_BOUND('',#23486,.T.) ;
#17743=FACE_OUTER_BOUND('',#23487,.T.) ;
#17744=FACE_OUTER_BOUND('',#23488,.T.) ;
#17745=FACE_OUTER_BOUND('',#23489,.T.) ;
#17746=FACE_OUTER_BOUND('',#23490,.T.) ;
#17747=FACE_OUTER_BOUND('',#23491,.T.) ;
#17748=FACE_OUTER_BOUND('',#23492,.T.) ;
#17749=FACE_OUTER_BOUND('',#23493,.T.) ;
#17750=FACE_OUTER_BOUND('',#23494,.T.) ;
#17751=FACE_OUTER_BOUND('',#23495,.T.) ;
#17752=FACE_OUTER_BOUND('',#23496,.T.) ;
#17753=FACE_OUTER_BOUND('',#23497,.T.) ;
#17754=FACE_OUTER_BOUND('',#23498,.T.) ;
#17755=FACE_OUTER_BOUND('',#23499,.T.) ;
#17756=FACE_OUTER_BOUND('',#23500,.T.) ;
#17757=FACE_OUTER_BOUND('',#23501,.T.) ;
#17758=FACE_OUTER_BOUND('',#23502,.T.) ;
#17759=FACE_OUTER_BOUND('',#23503,.T.) ;
#17760=FACE_OUTER_BOUND('',#23504,.T.) ;
#17761=FACE_OUTER_BOUND('',#23506,.T.) ;
#17762=FACE_OUTER_BOUND('',#23507,.T.) ;
#17763=FACE_OUTER_BOUND('',#23508,.T.) ;
#17764=FACE_OUTER_BOUND('',#23509,.T.) ;
#17765=FACE_OUTER_BOUND('',#23510,.T.) ;
#17766=FACE_OUTER_BOUND('',#23511,.T.) ;
#17767=FACE_OUTER_BOUND('',#23512,.T.) ;
#17768=FACE_OUTER_BOUND('',#23513,.T.) ;
#17769=FACE_OUTER_BOUND('',#23514,.T.) ;
#17770=FACE_OUTER_BOUND('',#23515,.T.) ;
#17771=FACE_OUTER_BOUND('',#23516,.T.) ;
#17772=FACE_OUTER_BOUND('',#23517,.T.) ;
#17773=FACE_OUTER_BOUND('',#23518,.T.) ;
#17774=FACE_OUTER_BOUND('',#23519,.T.) ;
#17775=FACE_OUTER_BOUND('',#23520,.T.) ;
#17776=FACE_OUTER_BOUND('',#23521,.T.) ;
#17777=FACE_OUTER_BOUND('',#23522,.T.) ;
#17778=FACE_OUTER_BOUND('',#23523,.T.) ;
#17779=FACE_OUTER_BOUND('',#23525,.T.) ;
#17780=FACE_OUTER_BOUND('',#23526,.T.) ;
#17781=FACE_OUTER_BOUND('',#23527,.T.) ;
#17782=FACE_OUTER_BOUND('',#23528,.T.) ;
#17783=FACE_OUTER_BOUND('',#23529,.T.) ;
#17784=FACE_OUTER_BOUND('',#23530,.T.) ;
#17785=FACE_OUTER_BOUND('',#23531,.T.) ;
#17786=FACE_OUTER_BOUND('',#23532,.T.) ;
#17787=FACE_OUTER_BOUND('',#23533,.T.) ;
#17788=FACE_OUTER_BOUND('',#23534,.T.) ;
#17789=FACE_OUTER_BOUND('',#23535,.T.) ;
#17790=FACE_OUTER_BOUND('',#23536,.T.) ;
#17791=FACE_OUTER_BOUND('',#23537,.T.) ;
#17792=FACE_OUTER_BOUND('',#23538,.T.) ;
#17793=FACE_OUTER_BOUND('',#23539,.T.) ;
#17794=FACE_OUTER_BOUND('',#23540,.T.) ;
#17795=FACE_OUTER_BOUND('',#23541,.T.) ;
#17796=FACE_OUTER_BOUND('',#23542,.T.) ;
#17797=FACE_OUTER_BOUND('',#23543,.T.) ;
#17798=FACE_OUTER_BOUND('',#23544,.T.) ;
#17799=FACE_OUTER_BOUND('',#23545,.T.) ;
#17800=FACE_OUTER_BOUND('',#23546,.T.) ;
#17801=FACE_OUTER_BOUND('',#23547,.T.) ;
#17802=FACE_OUTER_BOUND('',#23548,.T.) ;
#17803=FACE_OUTER_BOUND('',#23549,.T.) ;
#17804=FACE_OUTER_BOUND('',#23550,.T.) ;
#17805=FACE_OUTER_BOUND('',#23551,.T.) ;
#17806=FACE_OUTER_BOUND('',#23552,.T.) ;
#17807=FACE_OUTER_BOUND('',#23553,.T.) ;
#17808=FACE_OUTER_BOUND('',#23554,.T.) ;
#17809=FACE_OUTER_BOUND('',#23555,.T.) ;
#17810=FACE_OUTER_BOUND('',#23556,.T.) ;
#17811=FACE_OUTER_BOUND('',#23557,.T.) ;
#17812=FACE_OUTER_BOUND('',#23558,.T.) ;
#17813=FACE_OUTER_BOUND('',#23559,.T.) ;
#17814=FACE_OUTER_BOUND('',#23560,.T.) ;
#17815=FACE_OUTER_BOUND('',#23561,.T.) ;
#17816=FACE_OUTER_BOUND('',#23562,.T.) ;
#17817=FACE_OUTER_BOUND('',#23563,.T.) ;
#17818=FACE_OUTER_BOUND('',#23564,.T.) ;
#17819=FACE_OUTER_BOUND('',#23565,.T.) ;
#17820=FACE_OUTER_BOUND('',#23566,.T.) ;
#17821=FACE_OUTER_BOUND('',#23567,.T.) ;
#17822=FACE_OUTER_BOUND('',#23568,.T.) ;
#17823=FACE_OUTER_BOUND('',#23569,.T.) ;
#17824=FACE_OUTER_BOUND('',#23570,.T.) ;
#17825=FACE_OUTER_BOUND('',#23571,.T.) ;
#17826=FACE_OUTER_BOUND('',#23572,.T.) ;
#17827=FACE_OUTER_BOUND('',#23573,.T.) ;
#17828=FACE_OUTER_BOUND('',#23574,.T.) ;
#17829=FACE_OUTER_BOUND('',#23575,.T.) ;
#17830=FACE_OUTER_BOUND('',#23576,.T.) ;
#17831=FACE_OUTER_BOUND('',#23577,.T.) ;
#17832=FACE_OUTER_BOUND('',#23578,.T.) ;
#17833=FACE_OUTER_BOUND('',#23579,.T.) ;
#17834=FACE_OUTER_BOUND('',#23580,.T.) ;
#17835=FACE_OUTER_BOUND('',#23581,.T.) ;
#17836=FACE_OUTER_BOUND('',#23582,.T.) ;
#17837=FACE_OUTER_BOUND('',#23583,.T.) ;
#17838=FACE_OUTER_BOUND('',#23584,.T.) ;
#17839=FACE_OUTER_BOUND('',#23585,.T.) ;
#17840=FACE_OUTER_BOUND('',#23586,.T.) ;
#17841=FACE_OUTER_BOUND('',#23587,.T.) ;
#17842=FACE_OUTER_BOUND('',#23588,.T.) ;
#17843=FACE_OUTER_BOUND('',#23589,.T.) ;
#17844=FACE_OUTER_BOUND('',#23590,.T.) ;
#17845=FACE_OUTER_BOUND('',#23591,.T.) ;
#17846=FACE_OUTER_BOUND('',#23592,.T.) ;
#17847=FACE_OUTER_BOUND('',#23593,.T.) ;
#17848=FACE_OUTER_BOUND('',#23594,.T.) ;
#17849=FACE_OUTER_BOUND('',#23595,.T.) ;
#17850=FACE_OUTER_BOUND('',#23596,.T.) ;
#17851=FACE_OUTER_BOUND('',#23597,.T.) ;
#17852=FACE_OUTER_BOUND('',#23598,.T.) ;
#17853=FACE_OUTER_BOUND('',#23599,.T.) ;
#17854=FACE_OUTER_BOUND('',#23600,.T.) ;
#17855=FACE_OUTER_BOUND('',#23601,.T.) ;
#17856=FACE_OUTER_BOUND('',#23602,.T.) ;
#17857=FACE_OUTER_BOUND('',#23603,.T.) ;
#17858=FACE_OUTER_BOUND('',#23604,.T.) ;
#17859=FACE_OUTER_BOUND('',#23605,.T.) ;
#17860=FACE_OUTER_BOUND('',#23606,.T.) ;
#17861=FACE_OUTER_BOUND('',#23607,.T.) ;
#17862=FACE_OUTER_BOUND('',#23608,.T.) ;
#17863=FACE_OUTER_BOUND('',#23609,.T.) ;
#17864=FACE_OUTER_BOUND('',#23610,.T.) ;
#17865=FACE_OUTER_BOUND('',#23611,.T.) ;
#17866=FACE_OUTER_BOUND('',#23612,.T.) ;
#17867=FACE_OUTER_BOUND('',#23613,.T.) ;
#17868=FACE_OUTER_BOUND('',#23614,.T.) ;
#17869=FACE_OUTER_BOUND('',#23615,.T.) ;
#17870=FACE_OUTER_BOUND('',#23616,.T.) ;
#17871=FACE_OUTER_BOUND('',#23617,.T.) ;
#17872=FACE_OUTER_BOUND('',#23618,.T.) ;
#17873=FACE_OUTER_BOUND('',#23619,.T.) ;
#17874=FACE_OUTER_BOUND('',#23620,.T.) ;
#17875=FACE_OUTER_BOUND('',#23621,.T.) ;
#17876=FACE_OUTER_BOUND('',#23622,.T.) ;
#17877=FACE_OUTER_BOUND('',#23623,.T.) ;
#17878=FACE_OUTER_BOUND('',#23624,.T.) ;
#17879=FACE_OUTER_BOUND('',#23625,.T.) ;
#17880=FACE_OUTER_BOUND('',#23626,.T.) ;
#17881=FACE_OUTER_BOUND('',#23627,.T.) ;
#17882=FACE_OUTER_BOUND('',#23628,.T.) ;
#17883=FACE_OUTER_BOUND('',#23629,.T.) ;
#17884=FACE_OUTER_BOUND('',#23630,.T.) ;
#17885=FACE_OUTER_BOUND('',#23631,.T.) ;
#17886=FACE_OUTER_BOUND('',#23632,.T.) ;
#17887=FACE_OUTER_BOUND('',#23633,.T.) ;
#17888=FACE_OUTER_BOUND('',#23634,.T.) ;
#17889=FACE_OUTER_BOUND('',#23635,.T.) ;
#17890=FACE_OUTER_BOUND('',#23636,.T.) ;
#17891=FACE_OUTER_BOUND('',#23637,.T.) ;
#17892=FACE_OUTER_BOUND('',#23638,.T.) ;
#17893=FACE_OUTER_BOUND('',#23639,.T.) ;
#17894=FACE_OUTER_BOUND('',#23640,.T.) ;
#17895=FACE_OUTER_BOUND('',#23641,.T.) ;
#17896=FACE_OUTER_BOUND('',#23642,.T.) ;
#17897=FACE_OUTER_BOUND('',#23643,.T.) ;
#17898=FACE_OUTER_BOUND('',#23644,.T.) ;
#17899=FACE_OUTER_BOUND('',#23645,.T.) ;
#17900=FACE_OUTER_BOUND('',#23646,.T.) ;
#17901=FACE_OUTER_BOUND('',#23647,.T.) ;
#17902=FACE_OUTER_BOUND('',#23648,.T.) ;
#17903=FACE_OUTER_BOUND('',#23649,.T.) ;
#17904=FACE_OUTER_BOUND('',#23650,.T.) ;
#17905=FACE_OUTER_BOUND('',#23651,.T.) ;
#17906=FACE_OUTER_BOUND('',#23652,.T.) ;
#17907=FACE_OUTER_BOUND('',#23653,.T.) ;
#17908=FACE_OUTER_BOUND('',#23654,.T.) ;
#17909=FACE_OUTER_BOUND('',#23655,.T.) ;
#17910=FACE_OUTER_BOUND('',#23656,.T.) ;
#17911=FACE_OUTER_BOUND('',#23657,.T.) ;
#17912=FACE_OUTER_BOUND('',#23658,.T.) ;
#17913=FACE_OUTER_BOUND('',#23659,.T.) ;
#17914=FACE_OUTER_BOUND('',#23660,.T.) ;
#17915=FACE_OUTER_BOUND('',#23661,.T.) ;
#17916=FACE_OUTER_BOUND('',#23662,.T.) ;
#17917=FACE_OUTER_BOUND('',#23663,.T.) ;
#17918=FACE_OUTER_BOUND('',#23664,.T.) ;
#17919=FACE_OUTER_BOUND('',#23665,.T.) ;
#17920=FACE_OUTER_BOUND('',#23666,.T.) ;
#17921=FACE_OUTER_BOUND('',#23667,.T.) ;
#17922=FACE_OUTER_BOUND('',#23668,.T.) ;
#17923=FACE_OUTER_BOUND('',#23669,.T.) ;
#17924=FACE_OUTER_BOUND('',#23670,.T.) ;
#17925=FACE_OUTER_BOUND('',#23671,.T.) ;
#17926=FACE_OUTER_BOUND('',#23672,.T.) ;
#17927=FACE_OUTER_BOUND('',#23673,.T.) ;
#17928=FACE_OUTER_BOUND('',#23674,.T.) ;
#17929=FACE_OUTER_BOUND('',#23675,.T.) ;
#17930=FACE_OUTER_BOUND('',#23676,.T.) ;
#17931=FACE_OUTER_BOUND('',#23677,.T.) ;
#17932=FACE_OUTER_BOUND('',#23678,.T.) ;
#17933=FACE_OUTER_BOUND('',#23679,.T.) ;
#17934=FACE_OUTER_BOUND('',#23680,.T.) ;
#17935=FACE_OUTER_BOUND('',#23681,.T.) ;
#17936=FACE_OUTER_BOUND('',#23682,.T.) ;
#17937=FACE_OUTER_BOUND('',#23683,.T.) ;
#17938=FACE_OUTER_BOUND('',#23684,.T.) ;
#17939=FACE_OUTER_BOUND('',#23685,.T.) ;
#17940=FACE_OUTER_BOUND('',#23686,.T.) ;
#17941=FACE_OUTER_BOUND('',#23687,.T.) ;
#17942=FACE_OUTER_BOUND('',#23688,.T.) ;
#17943=FACE_OUTER_BOUND('',#23689,.T.) ;
#17944=FACE_OUTER_BOUND('',#23690,.T.) ;
#17945=FACE_OUTER_BOUND('',#23691,.T.) ;
#17946=FACE_OUTER_BOUND('',#23692,.T.) ;
#17947=FACE_OUTER_BOUND('',#23693,.T.) ;
#17948=FACE_OUTER_BOUND('',#23694,.T.) ;
#17949=FACE_OUTER_BOUND('',#23695,.T.) ;
#17950=FACE_OUTER_BOUND('',#23696,.T.) ;
#17951=FACE_OUTER_BOUND('',#23697,.T.) ;
#17952=FACE_OUTER_BOUND('',#23698,.T.) ;
#17953=FACE_OUTER_BOUND('',#23699,.T.) ;
#17954=FACE_OUTER_BOUND('',#23700,.T.) ;
#17955=FACE_OUTER_BOUND('',#23701,.T.) ;
#17956=FACE_OUTER_BOUND('',#23702,.T.) ;
#17957=FACE_OUTER_BOUND('',#23703,.T.) ;
#17958=FACE_OUTER_BOUND('',#23704,.T.) ;
#17959=FACE_OUTER_BOUND('',#23705,.T.) ;
#17960=FACE_OUTER_BOUND('',#23707,.T.) ;
#17961=FACE_OUTER_BOUND('',#23708,.T.) ;
#17962=FACE_OUTER_BOUND('',#23709,.T.) ;
#17963=FACE_OUTER_BOUND('',#23710,.T.) ;
#17964=FACE_OUTER_BOUND('',#23711,.T.) ;
#17965=FACE_OUTER_BOUND('',#23712,.T.) ;
#17966=FACE_OUTER_BOUND('',#23713,.T.) ;
#17967=FACE_OUTER_BOUND('',#23714,.T.) ;
#17968=FACE_OUTER_BOUND('',#23715,.T.) ;
#17969=FACE_OUTER_BOUND('',#23718,.T.) ;
#17970=FACE_OUTER_BOUND('',#23719,.T.) ;
#17971=FACE_OUTER_BOUND('',#23720,.T.) ;
#17972=FACE_OUTER_BOUND('',#23721,.T.) ;
#17973=FACE_OUTER_BOUND('',#23723,.T.) ;
#17974=FACE_OUTER_BOUND('',#23725,.T.) ;
#17975=FACE_OUTER_BOUND('',#23726,.T.) ;
#17976=FACE_OUTER_BOUND('',#23727,.T.) ;
#17977=FACE_OUTER_BOUND('',#23728,.T.) ;
#17978=FACE_OUTER_BOUND('',#23729,.T.) ;
#17979=FACE_OUTER_BOUND('',#23730,.T.) ;
#17980=FACE_OUTER_BOUND('',#23731,.T.) ;
#17981=FACE_OUTER_BOUND('',#23732,.T.) ;
#17982=FACE_OUTER_BOUND('',#23733,.T.) ;
#17983=FACE_OUTER_BOUND('',#23734,.T.) ;
#17984=FACE_OUTER_BOUND('',#23735,.T.) ;
#17985=FACE_OUTER_BOUND('',#23736,.T.) ;
#17986=FACE_OUTER_BOUND('',#23737,.T.) ;
#17987=FACE_OUTER_BOUND('',#23738,.T.) ;
#17988=FACE_OUTER_BOUND('',#23739,.T.) ;
#17989=FACE_OUTER_BOUND('',#23740,.T.) ;
#17990=FACE_OUTER_BOUND('',#23741,.T.) ;
#17991=FACE_OUTER_BOUND('',#23742,.T.) ;
#17992=FACE_OUTER_BOUND('',#23743,.T.) ;
#17993=FACE_OUTER_BOUND('',#23744,.T.) ;
#17994=FACE_OUTER_BOUND('',#23746,.T.) ;
#17995=FACE_OUTER_BOUND('',#23747,.T.) ;
#17996=FACE_OUTER_BOUND('',#23748,.T.) ;
#17997=FACE_OUTER_BOUND('',#23749,.T.) ;
#17998=FACE_OUTER_BOUND('',#23750,.T.) ;
#17999=FACE_OUTER_BOUND('',#23751,.T.) ;
#18000=FACE_OUTER_BOUND('',#23752,.T.) ;
#18001=FACE_OUTER_BOUND('',#23753,.T.) ;
#18002=FACE_OUTER_BOUND('',#23754,.T.) ;
#18003=FACE_OUTER_BOUND('',#23755,.T.) ;
#18004=FACE_OUTER_BOUND('',#23756,.T.) ;
#18005=FACE_OUTER_BOUND('',#23757,.T.) ;
#18006=FACE_OUTER_BOUND('',#23758,.T.) ;
#18007=FACE_OUTER_BOUND('',#23759,.T.) ;
#18008=FACE_OUTER_BOUND('',#23760,.T.) ;
#18009=FACE_OUTER_BOUND('',#23761,.T.) ;
#18010=FACE_OUTER_BOUND('',#23762,.T.) ;
#18011=FACE_OUTER_BOUND('',#23763,.T.) ;
#18012=FACE_OUTER_BOUND('',#23765,.T.) ;
#18013=FACE_OUTER_BOUND('',#23766,.T.) ;
#18014=FACE_OUTER_BOUND('',#23767,.T.) ;
#18015=FACE_OUTER_BOUND('',#23768,.T.) ;
#18016=FACE_OUTER_BOUND('',#23769,.T.) ;
#18017=FACE_OUTER_BOUND('',#23770,.T.) ;
#18018=FACE_OUTER_BOUND('',#23771,.T.) ;
#18019=FACE_OUTER_BOUND('',#23772,.T.) ;
#18020=FACE_OUTER_BOUND('',#23773,.T.) ;
#18021=FACE_OUTER_BOUND('',#23774,.T.) ;
#18022=FACE_OUTER_BOUND('',#23775,.T.) ;
#18023=FACE_OUTER_BOUND('',#23776,.T.) ;
#18024=FACE_OUTER_BOUND('',#23777,.T.) ;
#18025=FACE_OUTER_BOUND('',#23778,.T.) ;
#18026=FACE_OUTER_BOUND('',#23779,.T.) ;
#18027=FACE_OUTER_BOUND('',#23780,.T.) ;
#18028=FACE_OUTER_BOUND('',#23781,.T.) ;
#18029=FACE_OUTER_BOUND('',#23782,.T.) ;
#18030=FACE_OUTER_BOUND('',#23783,.T.) ;
#18031=FACE_OUTER_BOUND('',#23784,.T.) ;
#18032=FACE_OUTER_BOUND('',#23785,.T.) ;
#18033=FACE_OUTER_BOUND('',#23786,.T.) ;
#18034=FACE_OUTER_BOUND('',#23787,.T.) ;
#18035=FACE_OUTER_BOUND('',#23788,.T.) ;
#18036=FACE_OUTER_BOUND('',#23789,.T.) ;
#18037=FACE_OUTER_BOUND('',#23790,.T.) ;
#18038=FACE_OUTER_BOUND('',#23791,.T.) ;
#18039=FACE_OUTER_BOUND('',#23792,.T.) ;
#18040=FACE_OUTER_BOUND('',#23793,.T.) ;
#18041=FACE_OUTER_BOUND('',#23794,.T.) ;
#18042=FACE_OUTER_BOUND('',#23795,.T.) ;
#18043=FACE_OUTER_BOUND('',#23796,.T.) ;
#18044=FACE_OUTER_BOUND('',#23797,.T.) ;
#18045=FACE_OUTER_BOUND('',#23798,.T.) ;
#18046=FACE_OUTER_BOUND('',#23799,.T.) ;
#18047=FACE_OUTER_BOUND('',#23800,.T.) ;
#18048=FACE_OUTER_BOUND('',#23801,.T.) ;
#18049=FACE_OUTER_BOUND('',#23802,.T.) ;
#18050=FACE_OUTER_BOUND('',#23803,.T.) ;
#18051=FACE_OUTER_BOUND('',#23804,.T.) ;
#18052=FACE_OUTER_BOUND('',#23805,.T.) ;
#18053=FACE_OUTER_BOUND('',#23806,.T.) ;
#18054=FACE_OUTER_BOUND('',#23807,.T.) ;
#18055=FACE_OUTER_BOUND('',#23808,.T.) ;
#18056=FACE_OUTER_BOUND('',#23809,.T.) ;
#18057=FACE_OUTER_BOUND('',#23810,.T.) ;
#18058=FACE_OUTER_BOUND('',#23811,.T.) ;
#18059=FACE_OUTER_BOUND('',#23812,.T.) ;
#18060=FACE_OUTER_BOUND('',#23813,.T.) ;
#18061=FACE_OUTER_BOUND('',#23814,.T.) ;
#18062=FACE_OUTER_BOUND('',#23815,.T.) ;
#18063=FACE_OUTER_BOUND('',#23816,.T.) ;
#18064=FACE_OUTER_BOUND('',#23817,.T.) ;
#18065=FACE_OUTER_BOUND('',#23818,.T.) ;
#18066=FACE_OUTER_BOUND('',#23819,.T.) ;
#18067=FACE_OUTER_BOUND('',#23820,.T.) ;
#18068=FACE_OUTER_BOUND('',#23821,.T.) ;
#18069=FACE_OUTER_BOUND('',#23822,.T.) ;
#18070=FACE_OUTER_BOUND('',#23823,.T.) ;
#18071=FACE_OUTER_BOUND('',#23824,.T.) ;
#18072=FACE_OUTER_BOUND('',#23825,.T.) ;
#18073=FACE_OUTER_BOUND('',#23826,.T.) ;
#18074=FACE_OUTER_BOUND('',#23827,.T.) ;
#18075=FACE_OUTER_BOUND('',#23828,.T.) ;
#18076=FACE_OUTER_BOUND('',#23829,.T.) ;
#18077=FACE_OUTER_BOUND('',#23830,.T.) ;
#18078=FACE_OUTER_BOUND('',#23831,.T.) ;
#18079=FACE_OUTER_BOUND('',#23832,.T.) ;
#18080=FACE_OUTER_BOUND('',#23833,.T.) ;
#18081=FACE_OUTER_BOUND('',#23834,.T.) ;
#18082=FACE_OUTER_BOUND('',#23835,.T.) ;
#18083=FACE_OUTER_BOUND('',#23836,.T.) ;
#18084=FACE_OUTER_BOUND('',#23837,.T.) ;
#18085=FACE_OUTER_BOUND('',#23838,.T.) ;
#18086=FACE_OUTER_BOUND('',#23839,.T.) ;
#18087=FACE_OUTER_BOUND('',#23840,.T.) ;
#18088=FACE_OUTER_BOUND('',#23841,.T.) ;
#18089=FACE_OUTER_BOUND('',#23842,.T.) ;
#18090=FACE_OUTER_BOUND('',#23843,.T.) ;
#18091=FACE_OUTER_BOUND('',#23844,.T.) ;
#18092=FACE_OUTER_BOUND('',#23845,.T.) ;
#18093=FACE_OUTER_BOUND('',#23846,.T.) ;
#18094=FACE_OUTER_BOUND('',#23847,.T.) ;
#18095=FACE_OUTER_BOUND('',#23848,.T.) ;
#18096=FACE_OUTER_BOUND('',#23849,.T.) ;
#18097=FACE_OUTER_BOUND('',#23850,.T.) ;
#18098=FACE_OUTER_BOUND('',#23851,.T.) ;
#18099=FACE_OUTER_BOUND('',#23852,.T.) ;
#18100=FACE_OUTER_BOUND('',#23853,.T.) ;
#18101=FACE_OUTER_BOUND('',#23854,.T.) ;
#18102=FACE_OUTER_BOUND('',#23855,.T.) ;
#18103=FACE_OUTER_BOUND('',#23856,.T.) ;
#18104=FACE_OUTER_BOUND('',#23857,.T.) ;
#18105=FACE_OUTER_BOUND('',#23858,.T.) ;
#18106=FACE_OUTER_BOUND('',#23859,.T.) ;
#18107=FACE_OUTER_BOUND('',#23860,.T.) ;
#18108=FACE_OUTER_BOUND('',#23861,.T.) ;
#18109=FACE_OUTER_BOUND('',#23862,.T.) ;
#18110=FACE_OUTER_BOUND('',#23863,.T.) ;
#18111=FACE_OUTER_BOUND('',#23864,.T.) ;
#18112=FACE_OUTER_BOUND('',#23865,.T.) ;
#18113=FACE_OUTER_BOUND('',#23866,.T.) ;
#18114=FACE_OUTER_BOUND('',#23867,.T.) ;
#18115=FACE_OUTER_BOUND('',#23868,.T.) ;
#18116=FACE_OUTER_BOUND('',#23869,.T.) ;
#18117=FACE_OUTER_BOUND('',#23870,.T.) ;
#18118=FACE_OUTER_BOUND('',#23871,.T.) ;
#18119=FACE_OUTER_BOUND('',#23872,.T.) ;
#18120=FACE_OUTER_BOUND('',#23873,.T.) ;
#18121=FACE_OUTER_BOUND('',#23874,.T.) ;
#18122=FACE_OUTER_BOUND('',#23875,.T.) ;
#18123=FACE_OUTER_BOUND('',#23876,.T.) ;
#18124=FACE_OUTER_BOUND('',#23877,.T.) ;
#18125=FACE_OUTER_BOUND('',#23878,.T.) ;
#18126=FACE_OUTER_BOUND('',#23879,.T.) ;
#18127=FACE_OUTER_BOUND('',#23880,.T.) ;
#18128=FACE_OUTER_BOUND('',#23881,.T.) ;
#18129=FACE_OUTER_BOUND('',#23882,.T.) ;
#18130=FACE_OUTER_BOUND('',#23883,.T.) ;
#18131=FACE_OUTER_BOUND('',#23884,.T.) ;
#18132=FACE_OUTER_BOUND('',#23885,.T.) ;
#18133=FACE_OUTER_BOUND('',#23886,.T.) ;
#18134=FACE_OUTER_BOUND('',#23887,.T.) ;
#18135=FACE_OUTER_BOUND('',#23888,.T.) ;
#18136=FACE_OUTER_BOUND('',#23889,.T.) ;
#18137=FACE_OUTER_BOUND('',#23890,.T.) ;
#18138=FACE_OUTER_BOUND('',#23891,.T.) ;
#18139=FACE_OUTER_BOUND('',#23892,.T.) ;
#18140=FACE_OUTER_BOUND('',#23893,.T.) ;
#18141=FACE_OUTER_BOUND('',#23894,.T.) ;
#18142=FACE_OUTER_BOUND('',#23895,.T.) ;
#18143=FACE_OUTER_BOUND('',#23896,.T.) ;
#18144=FACE_OUTER_BOUND('',#23897,.T.) ;
#18145=FACE_OUTER_BOUND('',#23898,.T.) ;
#18146=FACE_OUTER_BOUND('',#23899,.T.) ;
#18147=FACE_OUTER_BOUND('',#23900,.T.) ;
#18148=FACE_OUTER_BOUND('',#23901,.T.) ;
#18149=FACE_OUTER_BOUND('',#23902,.T.) ;
#18150=FACE_OUTER_BOUND('',#23903,.T.) ;
#18151=FACE_OUTER_BOUND('',#23904,.T.) ;
#18152=FACE_OUTER_BOUND('',#23905,.T.) ;
#18153=FACE_OUTER_BOUND('',#23906,.T.) ;
#18154=FACE_OUTER_BOUND('',#23907,.T.) ;
#18155=FACE_OUTER_BOUND('',#23908,.T.) ;
#18156=FACE_OUTER_BOUND('',#23909,.T.) ;
#18157=FACE_OUTER_BOUND('',#23910,.T.) ;
#18158=FACE_OUTER_BOUND('',#23911,.T.) ;
#18159=FACE_OUTER_BOUND('',#23912,.T.) ;
#18160=FACE_OUTER_BOUND('',#23913,.T.) ;
#18161=FACE_OUTER_BOUND('',#23914,.T.) ;
#18162=FACE_OUTER_BOUND('',#23915,.T.) ;
#18163=FACE_OUTER_BOUND('',#23916,.T.) ;
#18164=FACE_OUTER_BOUND('',#23917,.T.) ;
#18165=FACE_OUTER_BOUND('',#23918,.T.) ;
#18166=FACE_OUTER_BOUND('',#23919,.T.) ;
#18167=FACE_OUTER_BOUND('',#23920,.T.) ;
#22763=EDGE_LOOP('',(#54031,#54032,#54033,#54034)) ;
#22764=EDGE_LOOP('',(#54035,#54036,#54037,#54038,#54039)) ;
#22765=EDGE_LOOP('',(#54040,#54041,#54042,#54043)) ;
#22766=EDGE_LOOP('',(#54044,#54045,#54046,#54047,#54048)) ;
#22767=EDGE_LOOP('',(#54049,#54050,#54051,#54052)) ;
#22768=EDGE_LOOP('',(#54053,#54054,#54055)) ;
#22769=EDGE_LOOP('',(#54056,#54057,#54058,#54059)) ;
#22770=EDGE_LOOP('',(#54060,#54061,#54062)) ;
#22771=EDGE_LOOP('',(#54063,#54064,#54065,#54066)) ;
#22772=EDGE_LOOP('',(#54067,#54068,#54069,#54070,#54071)) ;
#22773=EDGE_LOOP('',(#54072,#54073,#54074,#54075,#54076,#54077,#54078,#54079,
#54080,#54081,#54082,#54083,#54084,#54085,#54086,#54087,#54088,#54089,#54090,
#54091,#54092)) ;
#22774=EDGE_LOOP('',(#54093,#54094,#54095,#54096)) ;
#22775=EDGE_LOOP('',(#54097,#54098,#54099,#54100)) ;
#22776=EDGE_LOOP('',(#54101,#54102,#54103,#54104,#54105)) ;
#22777=EDGE_LOOP('',(#54106,#54107,#54108,#54109)) ;
#22778=EDGE_LOOP('',(#54110,#54111,#54112,#54113,#54114)) ;
#22779=EDGE_LOOP('',(#54115,#54116,#54117,#54118)) ;
#22780=EDGE_LOOP('',(#54119,#54120,#54121)) ;
#22781=EDGE_LOOP('',(#54122,#54123,#54124,#54125)) ;
#22782=EDGE_LOOP('',(#54126,#54127,#54128)) ;
#22783=EDGE_LOOP('',(#54129,#54130,#54131,#54132)) ;
#22784=EDGE_LOOP('',(#54133,#54134,#54135,#54136,#54137)) ;
#22785=EDGE_LOOP('',(#54138,#54139,#54140,#54141,#54142,#54143,#54144,#54145,
#54146,#54147,#54148,#54149,#54150,#54151,#54152,#54153,#54154,#54155,#54156,
#54157,#54158)) ;
#22786=EDGE_LOOP('',(#54159,#54160,#54161,#54162)) ;
#22787=EDGE_LOOP('',(#54163,#54164,#54165,#54166,#54167,#54168,#54169,#54170)) ;
#22788=EDGE_LOOP('',(#54171,#54172,#54173,#54174)) ;
#22789=EDGE_LOOP('',(#54175,#54176,#54177,#54178)) ;
#22790=EDGE_LOOP('',(#54179,#54180,#54181,#54182)) ;
#22791=EDGE_LOOP('',(#54183,#54184,#54185,#54186)) ;
#22792=EDGE_LOOP('',(#54187,#54188,#54189,#54190)) ;
#22793=EDGE_LOOP('',(#54191,#54192,#54193,#54194)) ;
#22794=EDGE_LOOP('',(#54195,#54196,#54197,#54198,#54199,#54200)) ;
#22795=EDGE_LOOP('',(#54201,#54202,#54203,#54204)) ;
#22796=EDGE_LOOP('',(#54205,#54206,#54207,#54208)) ;
#22797=EDGE_LOOP('',(#54209,#54210,#54211,#54212)) ;
#22798=EDGE_LOOP('',(#54213,#54214,#54215)) ;
#22799=EDGE_LOOP('',(#54216,#54217,#54218,#54219,#54220,#54221,#54222,#54223,
#54224,#54225,#54226,#54227,#54228,#54229,#54230,#54231,#54232,#54233,#54234,
#54235,#54236,#54237,#54238,#54239)) ;
#22800=EDGE_LOOP('',(#54240)) ;
#22801=EDGE_LOOP('',(#54241)) ;
#22802=EDGE_LOOP('',(#54242,#54243,#54244,#54245)) ;
#22803=EDGE_LOOP('',(#54246,#54247,#54248,#54249,#54250,#54251,#54252,#54253,
#54254,#54255,#54256,#54257)) ;
#22804=EDGE_LOOP('',(#54258,#54259,#54260,#54261)) ;
#22805=EDGE_LOOP('',(#54262,#54263,#54264,#54265,#54266,#54267)) ;
#22806=EDGE_LOOP('',(#54268,#54269,#54270,#54271)) ;
#22807=EDGE_LOOP('',(#54272,#54273,#54274,#54275,#54276,#54277,#54278,#54279)) ;
#22808=EDGE_LOOP('',(#54280)) ;
#22809=EDGE_LOOP('',(#54281,#54282,#54283,#54284,#54285,#54286,#54287,#54288)) ;
#22810=EDGE_LOOP('',(#54289)) ;
#22811=EDGE_LOOP('',(#54290,#54291,#54292,#54293)) ;
#22812=EDGE_LOOP('',(#54294,#54295,#54296,#54297)) ;
#22813=EDGE_LOOP('',(#54298,#54299,#54300,#54301)) ;
#22814=EDGE_LOOP('',(#54302,#54303,#54304,#54305)) ;
#22815=EDGE_LOOP('',(#54306,#54307,#54308,#54309,#54310,#54311,#54312,#54313)) ;
#22816=EDGE_LOOP('',(#54314,#54315,#54316,#54317,#54318,#54319,#54320,#54321)) ;
#22817=EDGE_LOOP('',(#54322,#54323,#54324,#54325)) ;
#22818=EDGE_LOOP('',(#54326,#54327,#54328,#54329,#54330,#54331,#54332,#54333)) ;
#22819=EDGE_LOOP('',(#54334,#54335,#54336,#54337,#54338,#54339,#54340,#54341)) ;
#22820=EDGE_LOOP('',(#54342,#54343,#54344,#54345)) ;
#22821=EDGE_LOOP('',(#54346,#54347,#54348,#54349,#54350,#54351,#54352,#54353,
#54354,#54355,#54356,#54357,#54358,#54359)) ;
#22822=EDGE_LOOP('',(#54360,#54361,#54362,#54363)) ;
#22823=EDGE_LOOP('',(#54364,#54365,#54366,#54367)) ;
#22824=EDGE_LOOP('',(#54368,#54369,#54370,#54371,#54372,#54373,#54374,#54375,
#54376,#54377,#54378,#54379,#54380,#54381,#54382,#54383,#54384,#54385,#54386,
#54387,#54388,#54389,#54390,#54391,#54392,#54393,#54394,#54395,#54396,#54397,
#54398,#54399)) ;
#22825=EDGE_LOOP('',(#54400,#54401,#54402,#54403)) ;
#22826=EDGE_LOOP('',(#54404,#54405,#54406,#54407)) ;
#22827=EDGE_LOOP('',(#54408,#54409,#54410,#54411,#54412,#54413,#54414,#54415)) ;
#22828=EDGE_LOOP('',(#54416,#54417,#54418,#54419,#54420,#54421,#54422,#54423)) ;
#22829=EDGE_LOOP('',(#54424,#54425,#54426,#54427,#54428,#54429,#54430,#54431)) ;
#22830=EDGE_LOOP('',(#54432,#54433,#54434,#54435)) ;
#22831=EDGE_LOOP('',(#54436,#54437,#54438,#54439)) ;
#22832=EDGE_LOOP('',(#54440,#54441,#54442,#54443,#54444,#54445)) ;
#22833=EDGE_LOOP('',(#54446,#54447,#54448,#54449,#54450,#54451)) ;
#22834=EDGE_LOOP('',(#54452,#54453,#54454,#54455)) ;
#22835=EDGE_LOOP('',(#54456,#54457,#54458,#54459)) ;
#22836=EDGE_LOOP('',(#54460,#54461,#54462,#54463)) ;
#22837=EDGE_LOOP('',(#54464,#54465,#54466,#54467)) ;
#22838=EDGE_LOOP('',(#54468,#54469,#54470,#54471)) ;
#22839=EDGE_LOOP('',(#54472,#54473,#54474,#54475,#54476,#54477,#54478,#54479)) ;
#22840=EDGE_LOOP('',(#54480,#54481,#54482,#54483)) ;
#22841=EDGE_LOOP('',(#54484,#54485,#54486,#54487)) ;
#22842=EDGE_LOOP('',(#54488,#54489,#54490,#54491)) ;
#22843=EDGE_LOOP('',(#54492,#54493,#54494,#54495)) ;
#22844=EDGE_LOOP('',(#54496,#54497,#54498,#54499)) ;
#22845=EDGE_LOOP('',(#54500,#54501,#54502,#54503)) ;
#22846=EDGE_LOOP('',(#54504,#54505,#54506,#54507)) ;
#22847=EDGE_LOOP('',(#54508,#54509,#54510,#54511)) ;
#22848=EDGE_LOOP('',(#54512,#54513,#54514,#54515,#54516,#54517,#54518,#54519)) ;
#22849=EDGE_LOOP('',(#54520,#54521)) ;
#22850=EDGE_LOOP('',(#54522,#54523,#54524,#54525)) ;
#22851=EDGE_LOOP('',(#54526,#54527,#54528,#54529)) ;
#22852=EDGE_LOOP('',(#54530,#54531,#54532,#54533)) ;
#22853=EDGE_LOOP('',(#54534,#54535,#54536,#54537)) ;
#22854=EDGE_LOOP('',(#54538,#54539,#54540,#54541)) ;
#22855=EDGE_LOOP('',(#54542,#54543,#54544,#54545)) ;
#22856=EDGE_LOOP('',(#54546,#54547,#54548,#54549)) ;
#22857=EDGE_LOOP('',(#54550,#54551,#54552,#54553)) ;
#22858=EDGE_LOOP('',(#54554,#54555,#54556,#54557,#54558,#54559,#54560,#54561)) ;
#22859=EDGE_LOOP('',(#54562,#54563,#54564,#54565)) ;
#22860=EDGE_LOOP('',(#54566,#54567,#54568,#54569)) ;
#22861=EDGE_LOOP('',(#54570,#54571,#54572,#54573)) ;
#22862=EDGE_LOOP('',(#54574,#54575,#54576,#54577)) ;
#22863=EDGE_LOOP('',(#54578,#54579,#54580,#54581)) ;
#22864=EDGE_LOOP('',(#54582,#54583,#54584,#54585)) ;
#22865=EDGE_LOOP('',(#54586,#54587,#54588,#54589)) ;
#22866=EDGE_LOOP('',(#54590,#54591,#54592,#54593)) ;
#22867=EDGE_LOOP('',(#54594,#54595,#54596,#54597)) ;
#22868=EDGE_LOOP('',(#54598,#54599,#54600,#54601)) ;
#22869=EDGE_LOOP('',(#54602,#54603,#54604,#54605)) ;
#22870=EDGE_LOOP('',(#54606,#54607,#54608,#54609)) ;
#22871=EDGE_LOOP('',(#54610,#54611,#54612,#54613,#54614,#54615)) ;
#22872=EDGE_LOOP('',(#54616)) ;
#22873=EDGE_LOOP('',(#54617,#54618,#54619,#54620,#54621,#54622)) ;
#22874=EDGE_LOOP('',(#54623,#54624,#54625,#54626)) ;
#22875=EDGE_LOOP('',(#54627,#54628,#54629,#54630)) ;
#22876=EDGE_LOOP('',(#54631,#54632,#54633,#54634)) ;
#22877=EDGE_LOOP('',(#54635,#54636,#54637,#54638)) ;
#22878=EDGE_LOOP('',(#54639,#54640,#54641,#54642)) ;
#22879=EDGE_LOOP('',(#54643,#54644,#54645,#54646)) ;
#22880=EDGE_LOOP('',(#54647,#54648,#54649,#54650)) ;
#22881=EDGE_LOOP('',(#54651,#54652,#54653,#54654)) ;
#22882=EDGE_LOOP('',(#54655,#54656,#54657,#54658)) ;
#22883=EDGE_LOOP('',(#54659,#54660,#54661)) ;
#22884=EDGE_LOOP('',(#54662,#54663,#54664,#54665)) ;
#22885=EDGE_LOOP('',(#54666,#54667,#54668,#54669)) ;
#22886=EDGE_LOOP('',(#54670,#54671,#54672,#54673)) ;
#22887=EDGE_LOOP('',(#54674,#54675,#54676,#54677)) ;
#22888=EDGE_LOOP('',(#54678,#54679,#54680,#54681)) ;
#22889=EDGE_LOOP('',(#54682,#54683,#54684,#54685)) ;
#22890=EDGE_LOOP('',(#54686,#54687,#54688,#54689)) ;
#22891=EDGE_LOOP('',(#54690,#54691,#54692,#54693)) ;
#22892=EDGE_LOOP('',(#54694,#54695,#54696,#54697)) ;
#22893=EDGE_LOOP('',(#54698,#54699,#54700)) ;
#22894=EDGE_LOOP('',(#54701,#54702,#54703,#54704)) ;
#22895=EDGE_LOOP('',(#54705,#54706,#54707)) ;
#22896=EDGE_LOOP('',(#54708,#54709,#54710,#54711)) ;
#22897=EDGE_LOOP('',(#54712,#54713,#54714,#54715)) ;
#22898=EDGE_LOOP('',(#54716,#54717,#54718,#54719)) ;
#22899=EDGE_LOOP('',(#54720,#54721,#54722,#54723)) ;
#22900=EDGE_LOOP('',(#54724,#54725,#54726,#54727)) ;
#22901=EDGE_LOOP('',(#54728,#54729,#54730)) ;
#22902=EDGE_LOOP('',(#54731,#54732,#54733,#54734)) ;
#22903=EDGE_LOOP('',(#54735,#54736,#54737,#54738)) ;
#22904=EDGE_LOOP('',(#54739,#54740,#54741,#54742)) ;
#22905=EDGE_LOOP('',(#54743,#54744,#54745,#54746)) ;
#22906=EDGE_LOOP('',(#54747,#54748,#54749,#54750)) ;
#22907=EDGE_LOOP('',(#54751,#54752,#54753,#54754,#54755,#54756)) ;
#22908=EDGE_LOOP('',(#54757,#54758,#54759,#54760)) ;
#22909=EDGE_LOOP('',(#54761,#54762,#54763,#54764)) ;
#22910=EDGE_LOOP('',(#54765,#54766,#54767,#54768)) ;
#22911=EDGE_LOOP('',(#54769,#54770,#54771,#54772)) ;
#22912=EDGE_LOOP('',(#54773,#54774,#54775,#54776)) ;
#22913=EDGE_LOOP('',(#54777,#54778,#54779,#54780)) ;
#22914=EDGE_LOOP('',(#54781,#54782,#54783,#54784,#54785,#54786)) ;
#22915=EDGE_LOOP('',(#54787,#54788,#54789,#54790)) ;
#22916=EDGE_LOOP('',(#54791,#54792,#54793,#54794)) ;
#22917=EDGE_LOOP('',(#54795,#54796,#54797)) ;
#22918=EDGE_LOOP('',(#54798,#54799,#54800,#54801)) ;
#22919=EDGE_LOOP('',(#54802,#54803,#54804,#54805)) ;
#22920=EDGE_LOOP('',(#54806,#54807,#54808)) ;
#22921=EDGE_LOOP('',(#54809,#54810,#54811)) ;
#22922=EDGE_LOOP('',(#54812,#54813,#54814,#54815)) ;
#22923=EDGE_LOOP('',(#54816,#54817,#54818,#54819)) ;
#22924=EDGE_LOOP('',(#54820,#54821,#54822)) ;
#22925=EDGE_LOOP('',(#54823,#54824,#54825,#54826)) ;
#22926=EDGE_LOOP('',(#54827,#54828,#54829,#54830)) ;
#22927=EDGE_LOOP('',(#54831,#54832,#54833,#54834)) ;
#22928=EDGE_LOOP('',(#54835,#54836,#54837,#54838)) ;
#22929=EDGE_LOOP('',(#54839,#54840,#54841,#54842)) ;
#22930=EDGE_LOOP('',(#54843,#54844,#54845,#54846)) ;
#22931=EDGE_LOOP('',(#54847,#54848,#54849,#54850)) ;
#22932=EDGE_LOOP('',(#54851,#54852,#54853,#54854)) ;
#22933=EDGE_LOOP('',(#54855,#54856,#54857,#54858)) ;
#22934=EDGE_LOOP('',(#54859,#54860,#54861,#54862)) ;
#22935=EDGE_LOOP('',(#54863,#54864,#54865)) ;
#22936=EDGE_LOOP('',(#54866,#54867,#54868)) ;
#22937=EDGE_LOOP('',(#54869,#54870,#54871,#54872)) ;
#22938=EDGE_LOOP('',(#54873,#54874,#54875,#54876)) ;
#22939=EDGE_LOOP('',(#54877,#54878,#54879,#54880)) ;
#22940=EDGE_LOOP('',(#54881,#54882,#54883,#54884)) ;
#22941=EDGE_LOOP('',(#54885,#54886,#54887,#54888)) ;
#22942=EDGE_LOOP('',(#54889,#54890,#54891)) ;
#22943=EDGE_LOOP('',(#54892,#54893,#54894)) ;
#22944=EDGE_LOOP('',(#54895,#54896,#54897,#54898)) ;
#22945=EDGE_LOOP('',(#54899,#54900,#54901,#54902)) ;
#22946=EDGE_LOOP('',(#54903,#54904,#54905,#54906)) ;
#22947=EDGE_LOOP('',(#54907,#54908,#54909,#54910)) ;
#22948=EDGE_LOOP('',(#54911,#54912,#54913,#54914)) ;
#22949=EDGE_LOOP('',(#54915,#54916,#54917,#54918)) ;
#22950=EDGE_LOOP('',(#54919,#54920,#54921,#54922)) ;
#22951=EDGE_LOOP('',(#54923,#54924,#54925,#54926)) ;
#22952=EDGE_LOOP('',(#54927,#54928,#54929,#54930)) ;
#22953=EDGE_LOOP('',(#54931,#54932,#54933,#54934)) ;
#22954=EDGE_LOOP('',(#54935,#54936,#54937,#54938)) ;
#22955=EDGE_LOOP('',(#54939,#54940,#54941)) ;
#22956=EDGE_LOOP('',(#54942,#54943,#54944)) ;
#22957=EDGE_LOOP('',(#54945,#54946,#54947,#54948)) ;
#22958=EDGE_LOOP('',(#54949,#54950,#54951,#54952)) ;
#22959=EDGE_LOOP('',(#54953,#54954,#54955,#54956)) ;
#22960=EDGE_LOOP('',(#54957,#54958,#54959,#54960)) ;
#22961=EDGE_LOOP('',(#54961,#54962,#54963,#54964)) ;
#22962=EDGE_LOOP('',(#54965,#54966,#54967)) ;
#22963=EDGE_LOOP('',(#54968,#54969,#54970)) ;
#22964=EDGE_LOOP('',(#54971,#54972,#54973,#54974)) ;
#22965=EDGE_LOOP('',(#54975,#54976,#54977,#54978)) ;
#22966=EDGE_LOOP('',(#54979,#54980,#54981,#54982)) ;
#22967=EDGE_LOOP('',(#54983,#54984,#54985)) ;
#22968=EDGE_LOOP('',(#54986,#54987,#54988,#54989)) ;
#22969=EDGE_LOOP('',(#54990,#54991,#54992,#54993)) ;
#22970=EDGE_LOOP('',(#54994,#54995,#54996,#54997)) ;
#22971=EDGE_LOOP('',(#54998,#54999,#55000,#55001)) ;
#22972=EDGE_LOOP('',(#55002,#55003,#55004,#55005)) ;
#22973=EDGE_LOOP('',(#55006,#55007,#55008,#55009)) ;
#22974=EDGE_LOOP('',(#55010,#55011,#55012,#55013)) ;
#22975=EDGE_LOOP('',(#55014,#55015,#55016,#55017)) ;
#22976=EDGE_LOOP('',(#55018,#55019,#55020)) ;
#22977=EDGE_LOOP('',(#55021,#55022,#55023,#55024)) ;
#22978=EDGE_LOOP('',(#55025,#55026,#55027,#55028)) ;
#22979=EDGE_LOOP('',(#55029,#55030,#55031,#55032)) ;
#22980=EDGE_LOOP('',(#55033,#55034,#55035,#55036)) ;
#22981=EDGE_LOOP('',(#55037,#55038,#55039,#55040)) ;
#22982=EDGE_LOOP('',(#55041,#55042,#55043,#55044)) ;
#22983=EDGE_LOOP('',(#55045,#55046,#55047,#55048)) ;
#22984=EDGE_LOOP('',(#55049,#55050,#55051,#55052)) ;
#22985=EDGE_LOOP('',(#55053,#55054,#55055,#55056)) ;
#22986=EDGE_LOOP('',(#55057,#55058,#55059,#55060)) ;
#22987=EDGE_LOOP('',(#55061,#55062,#55063,#55064)) ;
#22988=EDGE_LOOP('',(#55065,#55066,#55067,#55068)) ;
#22989=EDGE_LOOP('',(#55069,#55070,#55071,#55072)) ;
#22990=EDGE_LOOP('',(#55073,#55074,#55075,#55076)) ;
#22991=EDGE_LOOP('',(#55077,#55078,#55079)) ;
#22992=EDGE_LOOP('',(#55080,#55081,#55082,#55083)) ;
#22993=EDGE_LOOP('',(#55084,#55085,#55086,#55087)) ;
#22994=EDGE_LOOP('',(#55088,#55089,#55090,#55091)) ;
#22995=EDGE_LOOP('',(#55092,#55093,#55094,#55095)) ;
#22996=EDGE_LOOP('',(#55096,#55097,#55098,#55099)) ;
#22997=EDGE_LOOP('',(#55100,#55101,#55102,#55103)) ;
#22998=EDGE_LOOP('',(#55104,#55105,#55106,#55107)) ;
#22999=EDGE_LOOP('',(#55108,#55109,#55110,#55111)) ;
#23000=EDGE_LOOP('',(#55112,#55113,#55114,#55115)) ;
#23001=EDGE_LOOP('',(#55116,#55117,#55118)) ;
#23002=EDGE_LOOP('',(#55119,#55120,#55121,#55122,#55123)) ;
#23003=EDGE_LOOP('',(#55124,#55125,#55126,#55127)) ;
#23004=EDGE_LOOP('',(#55128,#55129,#55130,#55131)) ;
#23005=EDGE_LOOP('',(#55132,#55133,#55134,#55135)) ;
#23006=EDGE_LOOP('',(#55136,#55137,#55138,#55139)) ;
#23007=EDGE_LOOP('',(#55140,#55141,#55142)) ;
#23008=EDGE_LOOP('',(#55143,#55144,#55145,#55146)) ;
#23009=EDGE_LOOP('',(#55147,#55148,#55149,#55150)) ;
#23010=EDGE_LOOP('',(#55151,#55152,#55153)) ;
#23011=EDGE_LOOP('',(#55154,#55155,#55156,#55157,#55158,#55159,#55160,#55161)) ;
#23012=EDGE_LOOP('',(#55162,#55163,#55164,#55165)) ;
#23013=EDGE_LOOP('',(#55166,#55167,#55168,#55169)) ;
#23014=EDGE_LOOP('',(#55170,#55171,#55172,#55173)) ;
#23015=EDGE_LOOP('',(#55174,#55175,#55176,#55177)) ;
#23016=EDGE_LOOP('',(#55178,#55179,#55180,#55181)) ;
#23017=EDGE_LOOP('',(#55182,#55183,#55184,#55185)) ;
#23018=EDGE_LOOP('',(#55186,#55187,#55188,#55189)) ;
#23019=EDGE_LOOP('',(#55190,#55191,#55192,#55193)) ;
#23020=EDGE_LOOP('',(#55194,#55195,#55196,#55197)) ;
#23021=EDGE_LOOP('',(#55198,#55199,#55200,#55201,#55202,#55203,#55204)) ;
#23022=EDGE_LOOP('',(#55205,#55206,#55207,#55208,#55209,#55210,#55211)) ;
#23023=EDGE_LOOP('',(#55212,#55213,#55214,#55215)) ;
#23024=EDGE_LOOP('',(#55216,#55217,#55218,#55219)) ;
#23025=EDGE_LOOP('',(#55220,#55221,#55222)) ;
#23026=EDGE_LOOP('',(#55223,#55224,#55225,#55226)) ;
#23027=EDGE_LOOP('',(#55227,#55228,#55229,#55230,#55231,#55232,#55233,#55234,
#55235,#55236,#55237,#55238,#55239,#55240,#55241,#55242,#55243,#55244,#55245,
#55246,#55247,#55248,#55249,#55250,#55251,#55252,#55253,#55254,#55255,#55256,
#55257,#55258,#55259,#55260,#55261,#55262,#55263,#55264)) ;
#23028=EDGE_LOOP('',(#55265,#55266,#55267,#55268)) ;
#23029=EDGE_LOOP('',(#55269,#55270,#55271,#55272)) ;
#23030=EDGE_LOOP('',(#55273,#55274,#55275,#55276,#55277,#55278,#55279,#55280)) ;
#23031=EDGE_LOOP('',(#55281,#55282,#55283,#55284,#55285,#55286,#55287,#55288)) ;
#23032=EDGE_LOOP('',(#55289,#55290,#55291,#55292,#55293,#55294,#55295,#55296)) ;
#23033=EDGE_LOOP('',(#55297,#55298,#55299,#55300)) ;
#23034=EDGE_LOOP('',(#55301,#55302,#55303,#55304)) ;
#23035=EDGE_LOOP('',(#55305,#55306,#55307,#55308,#55309,#55310)) ;
#23036=EDGE_LOOP('',(#55311,#55312,#55313,#55314,#55315,#55316)) ;
#23037=EDGE_LOOP('',(#55317,#55318,#55319,#55320)) ;
#23038=EDGE_LOOP('',(#55321,#55322,#55323,#55324)) ;
#23039=EDGE_LOOP('',(#55325,#55326,#55327,#55328)) ;
#23040=EDGE_LOOP('',(#55329,#55330,#55331,#55332)) ;
#23041=EDGE_LOOP('',(#55333,#55334,#55335,#55336)) ;
#23042=EDGE_LOOP('',(#55337,#55338,#55339,#55340,#55341,#55342,#55343,#55344)) ;
#23043=EDGE_LOOP('',(#55345,#55346,#55347,#55348)) ;
#23044=EDGE_LOOP('',(#55349,#55350,#55351,#55352)) ;
#23045=EDGE_LOOP('',(#55353,#55354,#55355,#55356)) ;
#23046=EDGE_LOOP('',(#55357,#55358,#55359,#55360)) ;
#23047=EDGE_LOOP('',(#55361,#55362,#55363,#55364)) ;
#23048=EDGE_LOOP('',(#55365,#55366,#55367,#55368)) ;
#23049=EDGE_LOOP('',(#55369,#55370,#55371,#55372)) ;
#23050=EDGE_LOOP('',(#55373,#55374,#55375,#55376)) ;
#23051=EDGE_LOOP('',(#55377,#55378,#55379,#55380,#55381,#55382,#55383,#55384)) ;
#23052=EDGE_LOOP('',(#55385,#55386)) ;
#23053=EDGE_LOOP('',(#55387,#55388,#55389,#55390)) ;
#23054=EDGE_LOOP('',(#55391,#55392,#55393,#55394)) ;
#23055=EDGE_LOOP('',(#55395,#55396,#55397,#55398)) ;
#23056=EDGE_LOOP('',(#55399,#55400,#55401,#55402)) ;
#23057=EDGE_LOOP('',(#55403,#55404,#55405,#55406)) ;
#23058=EDGE_LOOP('',(#55407,#55408,#55409,#55410)) ;
#23059=EDGE_LOOP('',(#55411,#55412,#55413,#55414)) ;
#23060=EDGE_LOOP('',(#55415,#55416,#55417,#55418)) ;
#23061=EDGE_LOOP('',(#55419,#55420,#55421,#55422,#55423,#55424,#55425,#55426)) ;
#23062=EDGE_LOOP('',(#55427,#55428,#55429,#55430)) ;
#23063=EDGE_LOOP('',(#55431,#55432,#55433,#55434)) ;
#23064=EDGE_LOOP('',(#55435,#55436,#55437,#55438)) ;
#23065=EDGE_LOOP('',(#55439,#55440,#55441,#55442)) ;
#23066=EDGE_LOOP('',(#55443,#55444,#55445,#55446)) ;
#23067=EDGE_LOOP('',(#55447,#55448,#55449,#55450)) ;
#23068=EDGE_LOOP('',(#55451,#55452,#55453,#55454)) ;
#23069=EDGE_LOOP('',(#55455,#55456,#55457,#55458)) ;
#23070=EDGE_LOOP('',(#55459,#55460,#55461,#55462)) ;
#23071=EDGE_LOOP('',(#55463,#55464,#55465,#55466)) ;
#23072=EDGE_LOOP('',(#55467,#55468,#55469,#55470)) ;
#23073=EDGE_LOOP('',(#55471,#55472,#55473,#55474)) ;
#23074=EDGE_LOOP('',(#55475,#55476,#55477,#55478,#55479,#55480)) ;
#23075=EDGE_LOOP('',(#55481)) ;
#23076=EDGE_LOOP('',(#55482,#55483,#55484,#55485,#55486,#55487)) ;
#23077=EDGE_LOOP('',(#55488,#55489,#55490,#55491)) ;
#23078=EDGE_LOOP('',(#55492,#55493,#55494,#55495)) ;
#23079=EDGE_LOOP('',(#55496,#55497,#55498,#55499)) ;
#23080=EDGE_LOOP('',(#55500,#55501,#55502,#55503)) ;
#23081=EDGE_LOOP('',(#55504,#55505,#55506,#55507)) ;
#23082=EDGE_LOOP('',(#55508,#55509,#55510,#55511)) ;
#23083=EDGE_LOOP('',(#55512,#55513,#55514,#55515)) ;
#23084=EDGE_LOOP('',(#55516,#55517,#55518,#55519)) ;
#23085=EDGE_LOOP('',(#55520,#55521,#55522,#55523)) ;
#23086=EDGE_LOOP('',(#55524,#55525,#55526)) ;
#23087=EDGE_LOOP('',(#55527,#55528,#55529,#55530)) ;
#23088=EDGE_LOOP('',(#55531,#55532,#55533,#55534)) ;
#23089=EDGE_LOOP('',(#55535,#55536,#55537,#55538)) ;
#23090=EDGE_LOOP('',(#55539,#55540,#55541,#55542)) ;
#23091=EDGE_LOOP('',(#55543,#55544,#55545,#55546)) ;
#23092=EDGE_LOOP('',(#55547,#55548,#55549,#55550)) ;
#23093=EDGE_LOOP('',(#55551,#55552,#55553,#55554)) ;
#23094=EDGE_LOOP('',(#55555,#55556,#55557,#55558)) ;
#23095=EDGE_LOOP('',(#55559,#55560,#55561,#55562)) ;
#23096=EDGE_LOOP('',(#55563,#55564,#55565)) ;
#23097=EDGE_LOOP('',(#55566,#55567,#55568,#55569)) ;
#23098=EDGE_LOOP('',(#55570,#55571,#55572)) ;
#23099=EDGE_LOOP('',(#55573,#55574,#55575,#55576)) ;
#23100=EDGE_LOOP('',(#55577,#55578,#55579,#55580)) ;
#23101=EDGE_LOOP('',(#55581,#55582,#55583,#55584)) ;
#23102=EDGE_LOOP('',(#55585,#55586,#55587,#55588)) ;
#23103=EDGE_LOOP('',(#55589,#55590,#55591,#55592)) ;
#23104=EDGE_LOOP('',(#55593,#55594,#55595)) ;
#23105=EDGE_LOOP('',(#55596,#55597,#55598,#55599)) ;
#23106=EDGE_LOOP('',(#55600,#55601,#55602,#55603)) ;
#23107=EDGE_LOOP('',(#55604,#55605,#55606,#55607)) ;
#23108=EDGE_LOOP('',(#55608,#55609,#55610,#55611)) ;
#23109=EDGE_LOOP('',(#55612,#55613,#55614,#55615)) ;
#23110=EDGE_LOOP('',(#55616,#55617,#55618,#55619,#55620,#55621)) ;
#23111=EDGE_LOOP('',(#55622,#55623,#55624,#55625)) ;
#23112=EDGE_LOOP('',(#55626,#55627,#55628,#55629)) ;
#23113=EDGE_LOOP('',(#55630,#55631,#55632,#55633)) ;
#23114=EDGE_LOOP('',(#55634,#55635,#55636,#55637)) ;
#23115=EDGE_LOOP('',(#55638,#55639,#55640,#55641)) ;
#23116=EDGE_LOOP('',(#55642,#55643,#55644,#55645,#55646,#55647)) ;
#23117=EDGE_LOOP('',(#55648,#55649,#55650,#55651)) ;
#23118=EDGE_LOOP('',(#55652,#55653,#55654,#55655)) ;
#23119=EDGE_LOOP('',(#55656,#55657,#55658)) ;
#23120=EDGE_LOOP('',(#55659,#55660,#55661,#55662)) ;
#23121=EDGE_LOOP('',(#55663,#55664,#55665,#55666)) ;
#23122=EDGE_LOOP('',(#55667,#55668,#55669)) ;
#23123=EDGE_LOOP('',(#55670,#55671,#55672)) ;
#23124=EDGE_LOOP('',(#55673,#55674,#55675,#55676)) ;
#23125=EDGE_LOOP('',(#55677,#55678,#55679,#55680)) ;
#23126=EDGE_LOOP('',(#55681,#55682,#55683)) ;
#23127=EDGE_LOOP('',(#55684,#55685,#55686,#55687)) ;
#23128=EDGE_LOOP('',(#55688,#55689,#55690,#55691)) ;
#23129=EDGE_LOOP('',(#55692,#55693,#55694,#55695)) ;
#23130=EDGE_LOOP('',(#55696,#55697,#55698,#55699)) ;
#23131=EDGE_LOOP('',(#55700,#55701,#55702,#55703)) ;
#23132=EDGE_LOOP('',(#55704,#55705,#55706,#55707)) ;
#23133=EDGE_LOOP('',(#55708,#55709,#55710,#55711)) ;
#23134=EDGE_LOOP('',(#55712,#55713,#55714,#55715)) ;
#23135=EDGE_LOOP('',(#55716,#55717,#55718,#55719)) ;
#23136=EDGE_LOOP('',(#55720,#55721,#55722,#55723)) ;
#23137=EDGE_LOOP('',(#55724,#55725,#55726)) ;
#23138=EDGE_LOOP('',(#55727,#55728,#55729)) ;
#23139=EDGE_LOOP('',(#55730,#55731,#55732,#55733)) ;
#23140=EDGE_LOOP('',(#55734,#55735,#55736,#55737)) ;
#23141=EDGE_LOOP('',(#55738,#55739,#55740,#55741)) ;
#23142=EDGE_LOOP('',(#55742,#55743,#55744,#55745)) ;
#23143=EDGE_LOOP('',(#55746,#55747,#55748,#55749)) ;
#23144=EDGE_LOOP('',(#55750,#55751,#55752)) ;
#23145=EDGE_LOOP('',(#55753,#55754,#55755)) ;
#23146=EDGE_LOOP('',(#55756,#55757,#55758,#55759)) ;
#23147=EDGE_LOOP('',(#55760,#55761,#55762,#55763)) ;
#23148=EDGE_LOOP('',(#55764,#55765,#55766,#55767)) ;
#23149=EDGE_LOOP('',(#55768,#55769,#55770,#55771)) ;
#23150=EDGE_LOOP('',(#55772,#55773,#55774,#55775)) ;
#23151=EDGE_LOOP('',(#55776,#55777,#55778,#55779)) ;
#23152=EDGE_LOOP('',(#55780,#55781,#55782,#55783)) ;
#23153=EDGE_LOOP('',(#55784,#55785,#55786,#55787)) ;
#23154=EDGE_LOOP('',(#55788,#55789,#55790,#55791)) ;
#23155=EDGE_LOOP('',(#55792,#55793,#55794,#55795)) ;
#23156=EDGE_LOOP('',(#55796,#55797,#55798,#55799)) ;
#23157=EDGE_LOOP('',(#55800,#55801,#55802)) ;
#23158=EDGE_LOOP('',(#55803,#55804,#55805)) ;
#23159=EDGE_LOOP('',(#55806,#55807,#55808,#55809)) ;
#23160=EDGE_LOOP('',(#55810,#55811,#55812,#55813)) ;
#23161=EDGE_LOOP('',(#55814,#55815,#55816,#55817)) ;
#23162=EDGE_LOOP('',(#55818,#55819,#55820,#55821)) ;
#23163=EDGE_LOOP('',(#55822,#55823,#55824,#55825)) ;
#23164=EDGE_LOOP('',(#55826,#55827,#55828)) ;
#23165=EDGE_LOOP('',(#55829,#55830,#55831)) ;
#23166=EDGE_LOOP('',(#55832,#55833,#55834,#55835)) ;
#23167=EDGE_LOOP('',(#55836,#55837,#55838,#55839)) ;
#23168=EDGE_LOOP('',(#55840,#55841,#55842)) ;
#23169=EDGE_LOOP('',(#55843,#55844,#55845,#55846)) ;
#23170=EDGE_LOOP('',(#55847,#55848,#55849,#55850)) ;
#23171=EDGE_LOOP('',(#55851,#55852,#55853,#55854)) ;
#23172=EDGE_LOOP('',(#55855,#55856,#55857,#55858)) ;
#23173=EDGE_LOOP('',(#55859,#55860,#55861,#55862)) ;
#23174=EDGE_LOOP('',(#55863,#55864,#55865,#55866)) ;
#23175=EDGE_LOOP('',(#55867,#55868,#55869,#55870)) ;
#23176=EDGE_LOOP('',(#55871,#55872,#55873)) ;
#23177=EDGE_LOOP('',(#55874,#55875,#55876,#55877)) ;
#23178=EDGE_LOOP('',(#55878,#55879,#55880,#55881)) ;
#23179=EDGE_LOOP('',(#55882,#55883,#55884,#55885)) ;
#23180=EDGE_LOOP('',(#55886,#55887,#55888,#55889)) ;
#23181=EDGE_LOOP('',(#55890,#55891,#55892,#55893)) ;
#23182=EDGE_LOOP('',(#55894,#55895,#55896)) ;
#23183=EDGE_LOOP('',(#55897,#55898,#55899,#55900)) ;
#23184=EDGE_LOOP('',(#55901,#55902,#55903,#55904)) ;
#23185=EDGE_LOOP('',(#55905,#55906,#55907,#55908)) ;
#23186=EDGE_LOOP('',(#55909,#55910,#55911,#55912)) ;
#23187=EDGE_LOOP('',(#55913,#55914,#55915,#55916)) ;
#23188=EDGE_LOOP('',(#55917,#55918,#55919,#55920)) ;
#23189=EDGE_LOOP('',(#55921,#55922,#55923,#55924)) ;
#23190=EDGE_LOOP('',(#55925,#55926,#55927,#55928)) ;
#23191=EDGE_LOOP('',(#55929,#55930,#55931)) ;
#23192=EDGE_LOOP('',(#55932,#55933,#55934,#55935,#55936)) ;
#23193=EDGE_LOOP('',(#55937,#55938,#55939,#55940)) ;
#23194=EDGE_LOOP('',(#55941,#55942,#55943,#55944)) ;
#23195=EDGE_LOOP('',(#55945,#55946,#55947,#55948)) ;
#23196=EDGE_LOOP('',(#55949,#55950,#55951)) ;
#23197=EDGE_LOOP('',(#55952,#55953,#55954,#55955)) ;
#23198=EDGE_LOOP('',(#55956,#55957,#55958,#55959)) ;
#23199=EDGE_LOOP('',(#55960,#55961,#55962)) ;
#23200=EDGE_LOOP('',(#55963,#55964,#55965)) ;
#23201=EDGE_LOOP('',(#55966,#55967,#55968)) ;
#23202=EDGE_LOOP('',(#55969,#55970,#55971,#55972)) ;
#23203=EDGE_LOOP('',(#55973,#55974,#55975,#55976)) ;
#23204=EDGE_LOOP('',(#55977,#55978,#55979,#55980)) ;
#23205=EDGE_LOOP('',(#55981,#55982,#55983,#55984)) ;
#23206=EDGE_LOOP('',(#55985,#55986,#55987)) ;
#23207=EDGE_LOOP('',(#55988,#55989,#55990)) ;
#23208=EDGE_LOOP('',(#55991,#55992,#55993)) ;
#23209=EDGE_LOOP('',(#55994,#55995,#55996)) ;
#23210=EDGE_LOOP('',(#55997,#55998,#55999,#56000)) ;
#23211=EDGE_LOOP('',(#56001,#56002,#56003,#56004)) ;
#23212=EDGE_LOOP('',(#56005,#56006,#56007,#56008)) ;
#23213=EDGE_LOOP('',(#56009,#56010,#56011,#56012)) ;
#23214=EDGE_LOOP('',(#56013,#56014,#56015,#56016)) ;
#23215=EDGE_LOOP('',(#56017,#56018,#56019,#56020)) ;
#23216=EDGE_LOOP('',(#56021,#56022,#56023,#56024)) ;
#23217=EDGE_LOOP('',(#56025,#56026,#56027,#56028)) ;
#23218=EDGE_LOOP('',(#56029,#56030,#56031,#56032)) ;
#23219=EDGE_LOOP('',(#56033,#56034,#56035,#56036)) ;
#23220=EDGE_LOOP('',(#56037,#56038,#56039,#56040)) ;
#23221=EDGE_LOOP('',(#56041,#56042,#56043,#56044)) ;
#23222=EDGE_LOOP('',(#56045,#56046,#56047,#56048)) ;
#23223=EDGE_LOOP('',(#56049,#56050,#56051,#56052)) ;
#23224=EDGE_LOOP('',(#56053,#56054,#56055,#56056)) ;
#23225=EDGE_LOOP('',(#56057,#56058,#56059,#56060)) ;
#23226=EDGE_LOOP('',(#56061,#56062,#56063,#56064)) ;
#23227=EDGE_LOOP('',(#56065,#56066,#56067,#56068,#56069)) ;
#23228=EDGE_LOOP('',(#56070,#56071,#56072,#56073)) ;
#23229=EDGE_LOOP('',(#56074,#56075,#56076,#56077,#56078)) ;
#23230=EDGE_LOOP('',(#56079,#56080,#56081,#56082)) ;
#23231=EDGE_LOOP('',(#56083,#56084,#56085)) ;
#23232=EDGE_LOOP('',(#56086,#56087,#56088,#56089)) ;
#23233=EDGE_LOOP('',(#56090,#56091,#56092)) ;
#23234=EDGE_LOOP('',(#56093,#56094,#56095,#56096)) ;
#23235=EDGE_LOOP('',(#56097,#56098,#56099,#56100,#56101)) ;
#23236=EDGE_LOOP('',(#56102,#56103,#56104,#56105,#56106,#56107,#56108,#56109,
#56110,#56111,#56112,#56113,#56114,#56115,#56116,#56117,#56118,#56119,#56120,
#56121,#56122)) ;
#23237=EDGE_LOOP('',(#56123,#56124,#56125,#56126)) ;
#23238=EDGE_LOOP('',(#56127,#56128,#56129,#56130)) ;
#23239=EDGE_LOOP('',(#56131,#56132,#56133,#56134,#56135)) ;
#23240=EDGE_LOOP('',(#56136,#56137,#56138,#56139)) ;
#23241=EDGE_LOOP('',(#56140,#56141,#56142,#56143,#56144)) ;
#23242=EDGE_LOOP('',(#56145,#56146,#56147,#56148)) ;
#23243=EDGE_LOOP('',(#56149,#56150,#56151)) ;
#23244=EDGE_LOOP('',(#56152,#56153,#56154,#56155)) ;
#23245=EDGE_LOOP('',(#56156,#56157,#56158)) ;
#23246=EDGE_LOOP('',(#56159,#56160,#56161,#56162)) ;
#23247=EDGE_LOOP('',(#56163,#56164,#56165,#56166,#56167)) ;
#23248=EDGE_LOOP('',(#56168,#56169,#56170,#56171,#56172,#56173,#56174,#56175,
#56176,#56177,#56178,#56179,#56180,#56181,#56182,#56183,#56184,#56185,#56186,
#56187,#56188)) ;
#23249=EDGE_LOOP('',(#56189,#56190,#56191,#56192)) ;
#23250=EDGE_LOOP('',(#56193,#56194,#56195,#56196,#56197,#56198,#56199,#56200)) ;
#23251=EDGE_LOOP('',(#56201,#56202,#56203,#56204)) ;
#23252=EDGE_LOOP('',(#56205,#56206,#56207,#56208)) ;
#23253=EDGE_LOOP('',(#56209,#56210,#56211,#56212)) ;
#23254=EDGE_LOOP('',(#56213,#56214,#56215,#56216)) ;
#23255=EDGE_LOOP('',(#56217,#56218,#56219,#56220)) ;
#23256=EDGE_LOOP('',(#56221,#56222,#56223,#56224)) ;
#23257=EDGE_LOOP('',(#56225,#56226,#56227,#56228,#56229,#56230)) ;
#23258=EDGE_LOOP('',(#56231,#56232,#56233,#56234)) ;
#23259=EDGE_LOOP('',(#56235,#56236,#56237,#56238)) ;
#23260=EDGE_LOOP('',(#56239,#56240,#56241,#56242)) ;
#23261=EDGE_LOOP('',(#56243,#56244,#56245)) ;
#23262=EDGE_LOOP('',(#56246,#56247,#56248,#56249,#56250,#56251,#56252,#56253,
#56254,#56255,#56256,#56257,#56258,#56259,#56260,#56261,#56262,#56263,#56264,
#56265,#56266,#56267,#56268,#56269)) ;
#23263=EDGE_LOOP('',(#56270)) ;
#23264=EDGE_LOOP('',(#56271)) ;
#23265=EDGE_LOOP('',(#56272,#56273,#56274,#56275)) ;
#23266=EDGE_LOOP('',(#56276,#56277,#56278,#56279,#56280,#56281,#56282,#56283,
#56284,#56285,#56286,#56287)) ;
#23267=EDGE_LOOP('',(#56288,#56289,#56290,#56291)) ;
#23268=EDGE_LOOP('',(#56292,#56293,#56294,#56295,#56296,#56297)) ;
#23269=EDGE_LOOP('',(#56298,#56299,#56300,#56301)) ;
#23270=EDGE_LOOP('',(#56302,#56303,#56304,#56305,#56306,#56307,#56308,#56309)) ;
#23271=EDGE_LOOP('',(#56310)) ;
#23272=EDGE_LOOP('',(#56311,#56312,#56313,#56314,#56315,#56316,#56317,#56318)) ;
#23273=EDGE_LOOP('',(#56319)) ;
#23274=EDGE_LOOP('',(#56320,#56321,#56322,#56323)) ;
#23275=EDGE_LOOP('',(#56324,#56325,#56326,#56327)) ;
#23276=EDGE_LOOP('',(#56328,#56329,#56330,#56331)) ;
#23277=EDGE_LOOP('',(#56332,#56333,#56334,#56335)) ;
#23278=EDGE_LOOP('',(#56336,#56337,#56338,#56339,#56340,#56341,#56342,#56343)) ;
#23279=EDGE_LOOP('',(#56344,#56345,#56346,#56347,#56348,#56349,#56350,#56351)) ;
#23280=EDGE_LOOP('',(#56352,#56353,#56354,#56355)) ;
#23281=EDGE_LOOP('',(#56356,#56357,#56358,#56359,#56360,#56361,#56362,#56363)) ;
#23282=EDGE_LOOP('',(#56364,#56365,#56366,#56367,#56368,#56369,#56370,#56371)) ;
#23283=EDGE_LOOP('',(#56372,#56373,#56374,#56375)) ;
#23284=EDGE_LOOP('',(#56376,#56377,#56378,#56379,#56380,#56381,#56382,#56383,
#56384,#56385,#56386,#56387,#56388,#56389)) ;
#23285=EDGE_LOOP('',(#56390,#56391,#56392,#56393)) ;
#23286=EDGE_LOOP('',(#56394,#56395,#56396,#56397)) ;
#23287=EDGE_LOOP('',(#56398,#56399,#56400,#56401,#56402,#56403,#56404,#56405,
#56406,#56407,#56408,#56409,#56410,#56411,#56412,#56413,#56414,#56415,#56416,
#56417,#56418,#56419,#56420,#56421,#56422,#56423,#56424,#56425,#56426,#56427,
#56428,#56429)) ;
#23288=EDGE_LOOP('',(#56430,#56431,#56432,#56433)) ;
#23289=EDGE_LOOP('',(#56434,#56435,#56436,#56437)) ;
#23290=EDGE_LOOP('',(#56438,#56439,#56440,#56441,#56442,#56443,#56444,#56445)) ;
#23291=EDGE_LOOP('',(#56446,#56447,#56448,#56449,#56450,#56451,#56452,#56453)) ;
#23292=EDGE_LOOP('',(#56454,#56455,#56456,#56457,#56458,#56459,#56460,#56461)) ;
#23293=EDGE_LOOP('',(#56462,#56463,#56464,#56465)) ;
#23294=EDGE_LOOP('',(#56466,#56467,#56468,#56469)) ;
#23295=EDGE_LOOP('',(#56470,#56471,#56472,#56473,#56474,#56475)) ;
#23296=EDGE_LOOP('',(#56476,#56477,#56478,#56479,#56480,#56481)) ;
#23297=EDGE_LOOP('',(#56482,#56483,#56484,#56485)) ;
#23298=EDGE_LOOP('',(#56486,#56487,#56488,#56489)) ;
#23299=EDGE_LOOP('',(#56490,#56491,#56492,#56493)) ;
#23300=EDGE_LOOP('',(#56494,#56495,#56496,#56497)) ;
#23301=EDGE_LOOP('',(#56498,#56499,#56500,#56501)) ;
#23302=EDGE_LOOP('',(#56502,#56503,#56504,#56505,#56506,#56507,#56508,#56509)) ;
#23303=EDGE_LOOP('',(#56510,#56511,#56512,#56513)) ;
#23304=EDGE_LOOP('',(#56514,#56515,#56516,#56517)) ;
#23305=EDGE_LOOP('',(#56518,#56519,#56520,#56521)) ;
#23306=EDGE_LOOP('',(#56522,#56523,#56524,#56525)) ;
#23307=EDGE_LOOP('',(#56526,#56527,#56528,#56529)) ;
#23308=EDGE_LOOP('',(#56530,#56531,#56532,#56533)) ;
#23309=EDGE_LOOP('',(#56534,#56535,#56536,#56537)) ;
#23310=EDGE_LOOP('',(#56538,#56539,#56540,#56541)) ;
#23311=EDGE_LOOP('',(#56542,#56543,#56544,#56545,#56546,#56547,#56548,#56549)) ;
#23312=EDGE_LOOP('',(#56550,#56551)) ;
#23313=EDGE_LOOP('',(#56552,#56553,#56554,#56555)) ;
#23314=EDGE_LOOP('',(#56556,#56557,#56558,#56559)) ;
#23315=EDGE_LOOP('',(#56560,#56561,#56562,#56563)) ;
#23316=EDGE_LOOP('',(#56564,#56565,#56566,#56567)) ;
#23317=EDGE_LOOP('',(#56568,#56569,#56570,#56571)) ;
#23318=EDGE_LOOP('',(#56572,#56573,#56574,#56575)) ;
#23319=EDGE_LOOP('',(#56576,#56577,#56578,#56579)) ;
#23320=EDGE_LOOP('',(#56580,#56581,#56582,#56583)) ;
#23321=EDGE_LOOP('',(#56584,#56585,#56586,#56587,#56588,#56589,#56590,#56591)) ;
#23322=EDGE_LOOP('',(#56592,#56593,#56594,#56595)) ;
#23323=EDGE_LOOP('',(#56596,#56597,#56598,#56599)) ;
#23324=EDGE_LOOP('',(#56600,#56601,#56602,#56603)) ;
#23325=EDGE_LOOP('',(#56604,#56605,#56606,#56607)) ;
#23326=EDGE_LOOP('',(#56608,#56609,#56610,#56611)) ;
#23327=EDGE_LOOP('',(#56612,#56613,#56614,#56615)) ;
#23328=EDGE_LOOP('',(#56616,#56617,#56618,#56619)) ;
#23329=EDGE_LOOP('',(#56620,#56621,#56622,#56623)) ;
#23330=EDGE_LOOP('',(#56624,#56625,#56626,#56627)) ;
#23331=EDGE_LOOP('',(#56628,#56629,#56630,#56631)) ;
#23332=EDGE_LOOP('',(#56632,#56633,#56634,#56635)) ;
#23333=EDGE_LOOP('',(#56636,#56637,#56638,#56639)) ;
#23334=EDGE_LOOP('',(#56640,#56641,#56642,#56643,#56644,#56645)) ;
#23335=EDGE_LOOP('',(#56646)) ;
#23336=EDGE_LOOP('',(#56647,#56648,#56649,#56650,#56651,#56652)) ;
#23337=EDGE_LOOP('',(#56653,#56654,#56655,#56656)) ;
#23338=EDGE_LOOP('',(#56657,#56658,#56659,#56660)) ;
#23339=EDGE_LOOP('',(#56661,#56662,#56663,#56664)) ;
#23340=EDGE_LOOP('',(#56665,#56666,#56667,#56668)) ;
#23341=EDGE_LOOP('',(#56669,#56670,#56671,#56672)) ;
#23342=EDGE_LOOP('',(#56673,#56674,#56675,#56676)) ;
#23343=EDGE_LOOP('',(#56677,#56678,#56679,#56680)) ;
#23344=EDGE_LOOP('',(#56681,#56682,#56683,#56684)) ;
#23345=EDGE_LOOP('',(#56685,#56686,#56687,#56688)) ;
#23346=EDGE_LOOP('',(#56689,#56690,#56691)) ;
#23347=EDGE_LOOP('',(#56692,#56693,#56694,#56695)) ;
#23348=EDGE_LOOP('',(#56696,#56697,#56698,#56699)) ;
#23349=EDGE_LOOP('',(#56700,#56701,#56702,#56703)) ;
#23350=EDGE_LOOP('',(#56704,#56705,#56706,#56707)) ;
#23351=EDGE_LOOP('',(#56708,#56709,#56710,#56711)) ;
#23352=EDGE_LOOP('',(#56712,#56713,#56714,#56715)) ;
#23353=EDGE_LOOP('',(#56716,#56717,#56718,#56719)) ;
#23354=EDGE_LOOP('',(#56720,#56721,#56722,#56723)) ;
#23355=EDGE_LOOP('',(#56724,#56725,#56726,#56727)) ;
#23356=EDGE_LOOP('',(#56728,#56729,#56730)) ;
#23357=EDGE_LOOP('',(#56731,#56732,#56733,#56734)) ;
#23358=EDGE_LOOP('',(#56735,#56736,#56737)) ;
#23359=EDGE_LOOP('',(#56738,#56739,#56740,#56741)) ;
#23360=EDGE_LOOP('',(#56742,#56743,#56744,#56745)) ;
#23361=EDGE_LOOP('',(#56746,#56747,#56748,#56749)) ;
#23362=EDGE_LOOP('',(#56750,#56751,#56752,#56753)) ;
#23363=EDGE_LOOP('',(#56754,#56755,#56756,#56757)) ;
#23364=EDGE_LOOP('',(#56758,#56759,#56760)) ;
#23365=EDGE_LOOP('',(#56761,#56762,#56763,#56764)) ;
#23366=EDGE_LOOP('',(#56765,#56766,#56767,#56768)) ;
#23367=EDGE_LOOP('',(#56769,#56770,#56771,#56772)) ;
#23368=EDGE_LOOP('',(#56773,#56774,#56775,#56776)) ;
#23369=EDGE_LOOP('',(#56777,#56778,#56779,#56780)) ;
#23370=EDGE_LOOP('',(#56781,#56782,#56783,#56784,#56785,#56786)) ;
#23371=EDGE_LOOP('',(#56787,#56788,#56789,#56790)) ;
#23372=EDGE_LOOP('',(#56791,#56792,#56793,#56794)) ;
#23373=EDGE_LOOP('',(#56795,#56796,#56797,#56798)) ;
#23374=EDGE_LOOP('',(#56799,#56800,#56801,#56802)) ;
#23375=EDGE_LOOP('',(#56803,#56804,#56805,#56806)) ;
#23376=EDGE_LOOP('',(#56807,#56808,#56809,#56810)) ;
#23377=EDGE_LOOP('',(#56811,#56812,#56813,#56814,#56815,#56816)) ;
#23378=EDGE_LOOP('',(#56817,#56818,#56819,#56820)) ;
#23379=EDGE_LOOP('',(#56821,#56822,#56823,#56824)) ;
#23380=EDGE_LOOP('',(#56825,#56826,#56827)) ;
#23381=EDGE_LOOP('',(#56828,#56829,#56830,#56831)) ;
#23382=EDGE_LOOP('',(#56832,#56833,#56834,#56835)) ;
#23383=EDGE_LOOP('',(#56836,#56837,#56838)) ;
#23384=EDGE_LOOP('',(#56839,#56840,#56841)) ;
#23385=EDGE_LOOP('',(#56842,#56843,#56844,#56845)) ;
#23386=EDGE_LOOP('',(#56846,#56847,#56848,#56849)) ;
#23387=EDGE_LOOP('',(#56850,#56851,#56852)) ;
#23388=EDGE_LOOP('',(#56853,#56854,#56855,#56856)) ;
#23389=EDGE_LOOP('',(#56857,#56858,#56859,#56860)) ;
#23390=EDGE_LOOP('',(#56861,#56862,#56863,#56864)) ;
#23391=EDGE_LOOP('',(#56865,#56866,#56867,#56868)) ;
#23392=EDGE_LOOP('',(#56869,#56870,#56871,#56872)) ;
#23393=EDGE_LOOP('',(#56873,#56874,#56875,#56876)) ;
#23394=EDGE_LOOP('',(#56877,#56878,#56879,#56880)) ;
#23395=EDGE_LOOP('',(#56881,#56882,#56883,#56884)) ;
#23396=EDGE_LOOP('',(#56885,#56886,#56887,#56888)) ;
#23397=EDGE_LOOP('',(#56889,#56890,#56891,#56892)) ;
#23398=EDGE_LOOP('',(#56893,#56894,#56895)) ;
#23399=EDGE_LOOP('',(#56896,#56897,#56898)) ;
#23400=EDGE_LOOP('',(#56899,#56900,#56901,#56902)) ;
#23401=EDGE_LOOP('',(#56903,#56904,#56905,#56906)) ;
#23402=EDGE_LOOP('',(#56907,#56908,#56909,#56910)) ;
#23403=EDGE_LOOP('',(#56911,#56912,#56913,#56914)) ;
#23404=EDGE_LOOP('',(#56915,#56916,#56917,#56918)) ;
#23405=EDGE_LOOP('',(#56919,#56920,#56921)) ;
#23406=EDGE_LOOP('',(#56922,#56923,#56924)) ;
#23407=EDGE_LOOP('',(#56925,#56926,#56927,#56928)) ;
#23408=EDGE_LOOP('',(#56929,#56930,#56931,#56932)) ;
#23409=EDGE_LOOP('',(#56933,#56934,#56935,#56936)) ;
#23410=EDGE_LOOP('',(#56937,#56938,#56939,#56940)) ;
#23411=EDGE_LOOP('',(#56941,#56942,#56943,#56944)) ;
#23412=EDGE_LOOP('',(#56945,#56946,#56947,#56948)) ;
#23413=EDGE_LOOP('',(#56949,#56950,#56951,#56952)) ;
#23414=EDGE_LOOP('',(#56953,#56954,#56955,#56956)) ;
#23415=EDGE_LOOP('',(#56957,#56958,#56959,#56960)) ;
#23416=EDGE_LOOP('',(#56961,#56962,#56963,#56964)) ;
#23417=EDGE_LOOP('',(#56965,#56966,#56967,#56968)) ;
#23418=EDGE_LOOP('',(#56969,#56970,#56971)) ;
#23419=EDGE_LOOP('',(#56972,#56973,#56974)) ;
#23420=EDGE_LOOP('',(#56975,#56976,#56977,#56978)) ;
#23421=EDGE_LOOP('',(#56979,#56980,#56981,#56982)) ;
#23422=EDGE_LOOP('',(#56983,#56984,#56985,#56986)) ;
#23423=EDGE_LOOP('',(#56987,#56988,#56989,#56990)) ;
#23424=EDGE_LOOP('',(#56991,#56992,#56993,#56994)) ;
#23425=EDGE_LOOP('',(#56995,#56996,#56997)) ;
#23426=EDGE_LOOP('',(#56998,#56999,#57000)) ;
#23427=EDGE_LOOP('',(#57001,#57002,#57003,#57004)) ;
#23428=EDGE_LOOP('',(#57005,#57006,#57007,#57008)) ;
#23429=EDGE_LOOP('',(#57009,#57010,#57011,#57012)) ;
#23430=EDGE_LOOP('',(#57013,#57014,#57015)) ;
#23431=EDGE_LOOP('',(#57016,#57017,#57018,#57019)) ;
#23432=EDGE_LOOP('',(#57020,#57021,#57022,#57023)) ;
#23433=EDGE_LOOP('',(#57024,#57025,#57026,#57027)) ;
#23434=EDGE_LOOP('',(#57028,#57029,#57030,#57031)) ;
#23435=EDGE_LOOP('',(#57032,#57033,#57034,#57035)) ;
#23436=EDGE_LOOP('',(#57036,#57037,#57038,#57039)) ;
#23437=EDGE_LOOP('',(#57040,#57041,#57042,#57043)) ;
#23438=EDGE_LOOP('',(#57044,#57045,#57046,#57047)) ;
#23439=EDGE_LOOP('',(#57048,#57049,#57050)) ;
#23440=EDGE_LOOP('',(#57051,#57052,#57053,#57054)) ;
#23441=EDGE_LOOP('',(#57055,#57056,#57057,#57058)) ;
#23442=EDGE_LOOP('',(#57059,#57060,#57061,#57062)) ;
#23443=EDGE_LOOP('',(#57063,#57064,#57065,#57066)) ;
#23444=EDGE_LOOP('',(#57067,#57068,#57069,#57070)) ;
#23445=EDGE_LOOP('',(#57071,#57072,#57073,#57074)) ;
#23446=EDGE_LOOP('',(#57075,#57076,#57077,#57078)) ;
#23447=EDGE_LOOP('',(#57079,#57080,#57081,#57082)) ;
#23448=EDGE_LOOP('',(#57083,#57084,#57085,#57086)) ;
#23449=EDGE_LOOP('',(#57087,#57088,#57089,#57090)) ;
#23450=EDGE_LOOP('',(#57091,#57092,#57093,#57094)) ;
#23451=EDGE_LOOP('',(#57095,#57096,#57097,#57098)) ;
#23452=EDGE_LOOP('',(#57099,#57100,#57101,#57102)) ;
#23453=EDGE_LOOP('',(#57103,#57104,#57105,#57106)) ;
#23454=EDGE_LOOP('',(#57107,#57108,#57109)) ;
#23455=EDGE_LOOP('',(#57110,#57111,#57112,#57113)) ;
#23456=EDGE_LOOP('',(#57114,#57115,#57116,#57117)) ;
#23457=EDGE_LOOP('',(#57118,#57119,#57120,#57121)) ;
#23458=EDGE_LOOP('',(#57122,#57123,#57124,#57125)) ;
#23459=EDGE_LOOP('',(#57126,#57127,#57128,#57129)) ;
#23460=EDGE_LOOP('',(#57130,#57131,#57132,#57133)) ;
#23461=EDGE_LOOP('',(#57134,#57135,#57136,#57137)) ;
#23462=EDGE_LOOP('',(#57138,#57139,#57140,#57141)) ;
#23463=EDGE_LOOP('',(#57142,#57143,#57144,#57145)) ;
#23464=EDGE_LOOP('',(#57146,#57147,#57148)) ;
#23465=EDGE_LOOP('',(#57149,#57150,#57151,#57152,#57153)) ;
#23466=EDGE_LOOP('',(#57154,#57155,#57156,#57157)) ;
#23467=EDGE_LOOP('',(#57158,#57159,#57160,#57161)) ;
#23468=EDGE_LOOP('',(#57162,#57163,#57164,#57165)) ;
#23469=EDGE_LOOP('',(#57166,#57167,#57168,#57169)) ;
#23470=EDGE_LOOP('',(#57170,#57171,#57172)) ;
#23471=EDGE_LOOP('',(#57173,#57174,#57175,#57176)) ;
#23472=EDGE_LOOP('',(#57177,#57178,#57179,#57180)) ;
#23473=EDGE_LOOP('',(#57181,#57182,#57183)) ;
#23474=EDGE_LOOP('',(#57184,#57185,#57186,#57187,#57188,#57189,#57190,#57191)) ;
#23475=EDGE_LOOP('',(#57192,#57193,#57194,#57195)) ;
#23476=EDGE_LOOP('',(#57196,#57197,#57198,#57199)) ;
#23477=EDGE_LOOP('',(#57200,#57201,#57202,#57203)) ;
#23478=EDGE_LOOP('',(#57204,#57205,#57206,#57207)) ;
#23479=EDGE_LOOP('',(#57208,#57209,#57210,#57211)) ;
#23480=EDGE_LOOP('',(#57212,#57213,#57214,#57215)) ;
#23481=EDGE_LOOP('',(#57216,#57217,#57218,#57219)) ;
#23482=EDGE_LOOP('',(#57220,#57221,#57222,#57223)) ;
#23483=EDGE_LOOP('',(#57224,#57225,#57226,#57227)) ;
#23484=EDGE_LOOP('',(#57228,#57229,#57230,#57231,#57232,#57233,#57234)) ;
#23485=EDGE_LOOP('',(#57235,#57236,#57237,#57238,#57239,#57240,#57241)) ;
#23486=EDGE_LOOP('',(#57242,#57243,#57244,#57245)) ;
#23487=EDGE_LOOP('',(#57246,#57247,#57248)) ;
#23488=EDGE_LOOP('',(#57249,#57250,#57251,#57252)) ;
#23489=EDGE_LOOP('',(#57253,#57254,#57255,#57256)) ;
#23490=EDGE_LOOP('',(#57257,#57258,#57259,#57260,#57261,#57262,#57263,#57264,
#57265,#57266,#57267,#57268,#57269,#57270,#57271,#57272,#57273,#57274,#57275,
#57276,#57277,#57278,#57279,#57280,#57281,#57282,#57283,#57284,#57285,#57286,
#57287,#57288,#57289,#57290,#57291,#57292,#57293,#57294)) ;
#23491=EDGE_LOOP('',(#57295,#57296,#57297,#57298)) ;
#23492=EDGE_LOOP('',(#57299,#57300,#57301,#57302)) ;
#23493=EDGE_LOOP('',(#57303,#57304,#57305,#57306,#57307,#57308,#57309,#57310)) ;
#23494=EDGE_LOOP('',(#57311,#57312,#57313,#57314,#57315,#57316,#57317,#57318)) ;
#23495=EDGE_LOOP('',(#57319,#57320,#57321,#57322,#57323,#57324,#57325,#57326)) ;
#23496=EDGE_LOOP('',(#57327,#57328,#57329,#57330)) ;
#23497=EDGE_LOOP('',(#57331,#57332,#57333,#57334)) ;
#23498=EDGE_LOOP('',(#57335,#57336,#57337,#57338,#57339,#57340)) ;
#23499=EDGE_LOOP('',(#57341,#57342,#57343,#57344,#57345,#57346)) ;
#23500=EDGE_LOOP('',(#57347,#57348,#57349,#57350)) ;
#23501=EDGE_LOOP('',(#57351,#57352,#57353,#57354)) ;
#23502=EDGE_LOOP('',(#57355,#57356,#57357,#57358)) ;
#23503=EDGE_LOOP('',(#57359,#57360,#57361,#57362)) ;
#23504=EDGE_LOOP('',(#57363,#57364,#57365,#57366)) ;
#23505=EDGE_LOOP('',(#57367,#57368,#57369,#57370,#57371,#57372,#57373,#57374)) ;
#23506=EDGE_LOOP('',(#57375,#57376,#57377,#57378)) ;
#23507=EDGE_LOOP('',(#57379,#57380,#57381,#57382)) ;
#23508=EDGE_LOOP('',(#57383,#57384,#57385,#57386)) ;
#23509=EDGE_LOOP('',(#57387,#57388,#57389,#57390)) ;
#23510=EDGE_LOOP('',(#57391,#57392,#57393,#57394)) ;
#23511=EDGE_LOOP('',(#57395,#57396,#57397,#57398)) ;
#23512=EDGE_LOOP('',(#57399,#57400,#57401,#57402)) ;
#23513=EDGE_LOOP('',(#57403,#57404,#57405,#57406)) ;
#23514=EDGE_LOOP('',(#57407,#57408,#57409,#57410,#57411,#57412,#57413,#57414)) ;
#23515=EDGE_LOOP('',(#57415,#57416)) ;
#23516=EDGE_LOOP('',(#57417,#57418,#57419,#57420)) ;
#23517=EDGE_LOOP('',(#57421,#57422,#57423,#57424)) ;
#23518=EDGE_LOOP('',(#57425,#57426,#57427,#57428)) ;
#23519=EDGE_LOOP('',(#57429,#57430,#57431,#57432)) ;
#23520=EDGE_LOOP('',(#57433,#57434,#57435,#57436)) ;
#23521=EDGE_LOOP('',(#57437,#57438,#57439,#57440)) ;
#23522=EDGE_LOOP('',(#57441,#57442,#57443,#57444)) ;
#23523=EDGE_LOOP('',(#57445,#57446,#57447,#57448)) ;
#23524=EDGE_LOOP('',(#57449,#57450,#57451,#57452,#57453,#57454,#57455,#57456)) ;
#23525=EDGE_LOOP('',(#57457,#57458,#57459,#57460)) ;
#23526=EDGE_LOOP('',(#57461,#57462,#57463,#57464)) ;
#23527=EDGE_LOOP('',(#57465,#57466,#57467,#57468)) ;
#23528=EDGE_LOOP('',(#57469,#57470,#57471,#57472)) ;
#23529=EDGE_LOOP('',(#57473,#57474,#57475,#57476)) ;
#23530=EDGE_LOOP('',(#57477,#57478,#57479,#57480)) ;
#23531=EDGE_LOOP('',(#57481,#57482,#57483,#57484)) ;
#23532=EDGE_LOOP('',(#57485,#57486,#57487,#57488)) ;
#23533=EDGE_LOOP('',(#57489,#57490,#57491,#57492)) ;
#23534=EDGE_LOOP('',(#57493,#57494,#57495,#57496)) ;
#23535=EDGE_LOOP('',(#57497,#57498,#57499,#57500)) ;
#23536=EDGE_LOOP('',(#57501,#57502,#57503,#57504)) ;
#23537=EDGE_LOOP('',(#57505,#57506,#57507,#57508,#57509,#57510)) ;
#23538=EDGE_LOOP('',(#57511)) ;
#23539=EDGE_LOOP('',(#57512,#57513,#57514,#57515,#57516,#57517)) ;
#23540=EDGE_LOOP('',(#57518,#57519,#57520,#57521)) ;
#23541=EDGE_LOOP('',(#57522,#57523,#57524,#57525)) ;
#23542=EDGE_LOOP('',(#57526,#57527,#57528,#57529)) ;
#23543=EDGE_LOOP('',(#57530,#57531,#57532,#57533)) ;
#23544=EDGE_LOOP('',(#57534,#57535,#57536,#57537)) ;
#23545=EDGE_LOOP('',(#57538,#57539,#57540,#57541)) ;
#23546=EDGE_LOOP('',(#57542,#57543,#57544,#57545)) ;
#23547=EDGE_LOOP('',(#57546,#57547,#57548,#57549)) ;
#23548=EDGE_LOOP('',(#57550,#57551,#57552,#57553)) ;
#23549=EDGE_LOOP('',(#57554,#57555,#57556)) ;
#23550=EDGE_LOOP('',(#57557,#57558,#57559,#57560)) ;
#23551=EDGE_LOOP('',(#57561,#57562,#57563,#57564)) ;
#23552=EDGE_LOOP('',(#57565,#57566,#57567,#57568)) ;
#23553=EDGE_LOOP('',(#57569,#57570,#57571,#57572)) ;
#23554=EDGE_LOOP('',(#57573,#57574,#57575,#57576)) ;
#23555=EDGE_LOOP('',(#57577,#57578,#57579,#57580)) ;
#23556=EDGE_LOOP('',(#57581,#57582,#57583,#57584)) ;
#23557=EDGE_LOOP('',(#57585,#57586,#57587,#57588)) ;
#23558=EDGE_LOOP('',(#57589,#57590,#57591,#57592)) ;
#23559=EDGE_LOOP('',(#57593,#57594,#57595)) ;
#23560=EDGE_LOOP('',(#57596,#57597,#57598,#57599)) ;
#23561=EDGE_LOOP('',(#57600,#57601,#57602)) ;
#23562=EDGE_LOOP('',(#57603,#57604,#57605,#57606)) ;
#23563=EDGE_LOOP('',(#57607,#57608,#57609,#57610)) ;
#23564=EDGE_LOOP('',(#57611,#57612,#57613,#57614)) ;
#23565=EDGE_LOOP('',(#57615,#57616,#57617,#57618)) ;
#23566=EDGE_LOOP('',(#57619,#57620,#57621,#57622)) ;
#23567=EDGE_LOOP('',(#57623,#57624,#57625)) ;
#23568=EDGE_LOOP('',(#57626,#57627,#57628,#57629)) ;
#23569=EDGE_LOOP('',(#57630,#57631,#57632,#57633)) ;
#23570=EDGE_LOOP('',(#57634,#57635,#57636,#57637)) ;
#23571=EDGE_LOOP('',(#57638,#57639,#57640,#57641)) ;
#23572=EDGE_LOOP('',(#57642,#57643,#57644,#57645,#57646,#57647)) ;
#23573=EDGE_LOOP('',(#57648,#57649,#57650,#57651)) ;
#23574=EDGE_LOOP('',(#57652,#57653,#57654,#57655)) ;
#23575=EDGE_LOOP('',(#57656,#57657,#57658,#57659)) ;
#23576=EDGE_LOOP('',(#57660,#57661,#57662,#57663)) ;
#23577=EDGE_LOOP('',(#57664,#57665,#57666,#57667)) ;
#23578=EDGE_LOOP('',(#57668,#57669,#57670,#57671)) ;
#23579=EDGE_LOOP('',(#57672,#57673,#57674,#57675,#57676,#57677)) ;
#23580=EDGE_LOOP('',(#57678,#57679,#57680,#57681)) ;
#23581=EDGE_LOOP('',(#57682,#57683,#57684,#57685)) ;
#23582=EDGE_LOOP('',(#57686,#57687,#57688)) ;
#23583=EDGE_LOOP('',(#57689,#57690,#57691,#57692)) ;
#23584=EDGE_LOOP('',(#57693,#57694,#57695,#57696)) ;
#23585=EDGE_LOOP('',(#57697,#57698,#57699)) ;
#23586=EDGE_LOOP('',(#57700,#57701,#57702)) ;
#23587=EDGE_LOOP('',(#57703,#57704,#57705,#57706)) ;
#23588=EDGE_LOOP('',(#57707,#57708,#57709,#57710)) ;
#23589=EDGE_LOOP('',(#57711,#57712,#57713)) ;
#23590=EDGE_LOOP('',(#57714,#57715,#57716,#57717)) ;
#23591=EDGE_LOOP('',(#57718,#57719,#57720,#57721)) ;
#23592=EDGE_LOOP('',(#57722,#57723,#57724,#57725)) ;
#23593=EDGE_LOOP('',(#57726,#57727,#57728,#57729)) ;
#23594=EDGE_LOOP('',(#57730,#57731,#57732,#57733)) ;
#23595=EDGE_LOOP('',(#57734,#57735,#57736,#57737)) ;
#23596=EDGE_LOOP('',(#57738,#57739,#57740,#57741)) ;
#23597=EDGE_LOOP('',(#57742,#57743,#57744,#57745)) ;
#23598=EDGE_LOOP('',(#57746,#57747,#57748,#57749)) ;
#23599=EDGE_LOOP('',(#57750,#57751,#57752,#57753)) ;
#23600=EDGE_LOOP('',(#57754,#57755,#57756)) ;
#23601=EDGE_LOOP('',(#57757,#57758,#57759)) ;
#23602=EDGE_LOOP('',(#57760,#57761,#57762,#57763)) ;
#23603=EDGE_LOOP('',(#57764,#57765,#57766,#57767)) ;
#23604=EDGE_LOOP('',(#57768,#57769,#57770,#57771)) ;
#23605=EDGE_LOOP('',(#57772,#57773,#57774,#57775)) ;
#23606=EDGE_LOOP('',(#57776,#57777,#57778,#57779)) ;
#23607=EDGE_LOOP('',(#57780,#57781,#57782)) ;
#23608=EDGE_LOOP('',(#57783,#57784,#57785)) ;
#23609=EDGE_LOOP('',(#57786,#57787,#57788,#57789)) ;
#23610=EDGE_LOOP('',(#57790,#57791,#57792,#57793)) ;
#23611=EDGE_LOOP('',(#57794,#57795,#57796,#57797)) ;
#23612=EDGE_LOOP('',(#57798,#57799,#57800,#57801)) ;
#23613=EDGE_LOOP('',(#57802,#57803,#57804,#57805)) ;
#23614=EDGE_LOOP('',(#57806,#57807,#57808,#57809)) ;
#23615=EDGE_LOOP('',(#57810,#57811,#57812,#57813)) ;
#23616=EDGE_LOOP('',(#57814,#57815,#57816,#57817)) ;
#23617=EDGE_LOOP('',(#57818,#57819,#57820,#57821)) ;
#23618=EDGE_LOOP('',(#57822,#57823,#57824,#57825)) ;
#23619=EDGE_LOOP('',(#57826,#57827,#57828,#57829)) ;
#23620=EDGE_LOOP('',(#57830,#57831,#57832)) ;
#23621=EDGE_LOOP('',(#57833,#57834,#57835)) ;
#23622=EDGE_LOOP('',(#57836,#57837,#57838,#57839)) ;
#23623=EDGE_LOOP('',(#57840,#57841,#57842,#57843)) ;
#23624=EDGE_LOOP('',(#57844,#57845,#57846,#57847)) ;
#23625=EDGE_LOOP('',(#57848,#57849,#57850,#57851)) ;
#23626=EDGE_LOOP('',(#57852,#57853,#57854,#57855)) ;
#23627=EDGE_LOOP('',(#57856,#57857,#57858)) ;
#23628=EDGE_LOOP('',(#57859,#57860,#57861)) ;
#23629=EDGE_LOOP('',(#57862,#57863,#57864,#57865)) ;
#23630=EDGE_LOOP('',(#57866,#57867,#57868,#57869)) ;
#23631=EDGE_LOOP('',(#57870,#57871,#57872,#57873)) ;
#23632=EDGE_LOOP('',(#57874,#57875,#57876)) ;
#23633=EDGE_LOOP('',(#57877,#57878,#57879,#57880)) ;
#23634=EDGE_LOOP('',(#57881,#57882,#57883,#57884)) ;
#23635=EDGE_LOOP('',(#57885,#57886,#57887,#57888)) ;
#23636=EDGE_LOOP('',(#57889,#57890,#57891,#57892)) ;
#23637=EDGE_LOOP('',(#57893,#57894,#57895,#57896)) ;
#23638=EDGE_LOOP('',(#57897,#57898,#57899,#57900)) ;
#23639=EDGE_LOOP('',(#57901,#57902,#57903)) ;
#23640=EDGE_LOOP('',(#57904,#57905,#57906,#57907)) ;
#23641=EDGE_LOOP('',(#57908,#57909,#57910,#57911)) ;
#23642=EDGE_LOOP('',(#57912,#57913,#57914,#57915)) ;
#23643=EDGE_LOOP('',(#57916,#57917,#57918,#57919)) ;
#23644=EDGE_LOOP('',(#57920,#57921,#57922,#57923)) ;
#23645=EDGE_LOOP('',(#57924,#57925,#57926)) ;
#23646=EDGE_LOOP('',(#57927,#57928,#57929,#57930)) ;
#23647=EDGE_LOOP('',(#57931,#57932,#57933,#57934)) ;
#23648=EDGE_LOOP('',(#57935,#57936,#57937,#57938)) ;
#23649=EDGE_LOOP('',(#57939,#57940,#57941,#57942)) ;
#23650=EDGE_LOOP('',(#57943,#57944,#57945,#57946)) ;
#23651=EDGE_LOOP('',(#57947,#57948,#57949,#57950)) ;
#23652=EDGE_LOOP('',(#57951,#57952,#57953,#57954)) ;
#23653=EDGE_LOOP('',(#57955,#57956,#57957,#57958)) ;
#23654=EDGE_LOOP('',(#57959,#57960,#57961)) ;
#23655=EDGE_LOOP('',(#57962,#57963,#57964,#57965,#57966)) ;
#23656=EDGE_LOOP('',(#57967,#57968,#57969,#57970)) ;
#23657=EDGE_LOOP('',(#57971,#57972,#57973,#57974)) ;
#23658=EDGE_LOOP('',(#57975,#57976,#57977,#57978)) ;
#23659=EDGE_LOOP('',(#57979,#57980,#57981)) ;
#23660=EDGE_LOOP('',(#57982,#57983,#57984,#57985)) ;
#23661=EDGE_LOOP('',(#57986,#57987,#57988,#57989)) ;
#23662=EDGE_LOOP('',(#57990,#57991,#57992)) ;
#23663=EDGE_LOOP('',(#57993,#57994,#57995)) ;
#23664=EDGE_LOOP('',(#57996,#57997,#57998)) ;
#23665=EDGE_LOOP('',(#57999,#58000,#58001,#58002)) ;
#23666=EDGE_LOOP('',(#58003,#58004,#58005,#58006)) ;
#23667=EDGE_LOOP('',(#58007,#58008,#58009,#58010)) ;
#23668=EDGE_LOOP('',(#58011,#58012,#58013,#58014)) ;
#23669=EDGE_LOOP('',(#58015,#58016,#58017)) ;
#23670=EDGE_LOOP('',(#58018,#58019,#58020)) ;
#23671=EDGE_LOOP('',(#58021,#58022,#58023)) ;
#23672=EDGE_LOOP('',(#58024,#58025,#58026)) ;
#23673=EDGE_LOOP('',(#58027,#58028,#58029,#58030)) ;
#23674=EDGE_LOOP('',(#58031,#58032,#58033,#58034)) ;
#23675=EDGE_LOOP('',(#58035,#58036,#58037,#58038)) ;
#23676=EDGE_LOOP('',(#58039,#58040,#58041,#58042)) ;
#23677=EDGE_LOOP('',(#58043,#58044,#58045,#58046)) ;
#23678=EDGE_LOOP('',(#58047,#58048,#58049,#58050)) ;
#23679=EDGE_LOOP('',(#58051,#58052,#58053,#58054)) ;
#23680=EDGE_LOOP('',(#58055,#58056,#58057,#58058)) ;
#23681=EDGE_LOOP('',(#58059,#58060,#58061,#58062)) ;
#23682=EDGE_LOOP('',(#58063,#58064,#58065,#58066)) ;
#23683=EDGE_LOOP('',(#58067,#58068,#58069,#58070)) ;
#23684=EDGE_LOOP('',(#58071,#58072,#58073,#58074)) ;
#23685=EDGE_LOOP('',(#58075,#58076,#58077,#58078)) ;
#23686=EDGE_LOOP('',(#58079,#58080,#58081,#58082)) ;
#23687=EDGE_LOOP('',(#58083,#58084,#58085,#58086)) ;
#23688=EDGE_LOOP('',(#58087,#58088,#58089,#58090)) ;
#23689=EDGE_LOOP('',(#58091,#58092,#58093,#58094)) ;
#23690=EDGE_LOOP('',(#58095,#58096,#58097,#58098)) ;
#23691=EDGE_LOOP('',(#58099,#58100,#58101,#58102,#58103)) ;
#23692=EDGE_LOOP('',(#58104,#58105,#58106,#58107)) ;
#23693=EDGE_LOOP('',(#58108,#58109,#58110,#58111,#58112)) ;
#23694=EDGE_LOOP('',(#58113,#58114,#58115,#58116)) ;
#23695=EDGE_LOOP('',(#58117,#58118,#58119)) ;
#23696=EDGE_LOOP('',(#58120,#58121,#58122,#58123)) ;
#23697=EDGE_LOOP('',(#58124,#58125,#58126)) ;
#23698=EDGE_LOOP('',(#58127,#58128,#58129,#58130)) ;
#23699=EDGE_LOOP('',(#58131,#58132,#58133,#58134,#58135)) ;
#23700=EDGE_LOOP('',(#58136,#58137,#58138,#58139,#58140,#58141,#58142,#58143,
#58144,#58145,#58146,#58147,#58148,#58149,#58150,#58151,#58152,#58153,#58154,
#58155,#58156)) ;
#23701=EDGE_LOOP('',(#58157,#58158,#58159,#58160)) ;
#23702=EDGE_LOOP('',(#58161,#58162,#58163,#58164)) ;
#23703=EDGE_LOOP('',(#58165,#58166,#58167,#58168)) ;
#23704=EDGE_LOOP('',(#58169,#58170,#58171)) ;
#23705=EDGE_LOOP('',(#58172,#58173,#58174,#58175,#58176,#58177,#58178,#58179,
#58180,#58181,#58182,#58183,#58184,#58185)) ;
#23706=EDGE_LOOP('',(#58186)) ;
#23707=EDGE_LOOP('',(#58187,#58188,#58189,#58190)) ;
#23708=EDGE_LOOP('',(#58191,#58192,#58193,#58194,#58195,#58196,#58197,#58198)) ;
#23709=EDGE_LOOP('',(#58199,#58200,#58201,#58202)) ;
#23710=EDGE_LOOP('',(#58203,#58204,#58205,#58206)) ;
#23711=EDGE_LOOP('',(#58207,#58208,#58209,#58210)) ;
#23712=EDGE_LOOP('',(#58211,#58212,#58213,#58214)) ;
#23713=EDGE_LOOP('',(#58215,#58216,#58217,#58218)) ;
#23714=EDGE_LOOP('',(#58219,#58220,#58221,#58222)) ;
#23715=EDGE_LOOP('',(#58223,#58224,#58225,#58226)) ;
#23716=EDGE_LOOP('',(#58227,#58228,#58229,#58230,#58231,#58232,#58233,#58234)) ;
#23717=EDGE_LOOP('',(#58235)) ;
#23718=EDGE_LOOP('',(#58236,#58237,#58238,#58239)) ;
#23719=EDGE_LOOP('',(#58240,#58241,#58242,#58243)) ;
#23720=EDGE_LOOP('',(#58244,#58245,#58246,#58247)) ;
#23721=EDGE_LOOP('',(#58248,#58249,#58250,#58251)) ;
#23722=EDGE_LOOP('',(#58252,#58253,#58254,#58255,#58256,#58257,#58258,#58259)) ;
#23723=EDGE_LOOP('',(#58260,#58261,#58262,#58263)) ;
#23724=EDGE_LOOP('',(#58264,#58265,#58266,#58267,#58268,#58269,#58270,#58271)) ;
#23725=EDGE_LOOP('',(#58272,#58273,#58274,#58275)) ;
#23726=EDGE_LOOP('',(#58276,#58277,#58278,#58279,#58280,#58281,#58282,#58283,
#58284)) ;
#23727=EDGE_LOOP('',(#58285,#58286,#58287,#58288)) ;
#23728=EDGE_LOOP('',(#58289,#58290,#58291,#58292)) ;
#23729=EDGE_LOOP('',(#58293,#58294,#58295,#58296,#58297,#58298,#58299,#58300,
#58301,#58302,#58303,#58304,#58305,#58306,#58307,#58308,#58309,#58310,#58311,
#58312,#58313,#58314,#58315,#58316,#58317,#58318,#58319,#58320,#58321,#58322,
#58323,#58324,#58325,#58326,#58327,#58328,#58329,#58330)) ;
#23730=EDGE_LOOP('',(#58331,#58332,#58333,#58334,#58335,#58336,#58337,#58338,
#58339,#58340,#58341,#58342,#58343,#58344,#58345,#58346,#58347,#58348,#58349,
#58350,#58351,#58352,#58353,#58354,#58355,#58356,#58357,#58358,#58359,#58360,
#58361,#58362,#58363,#58364,#58365,#58366,#58367,#58368)) ;
#23731=EDGE_LOOP('',(#58369,#58370,#58371,#58372)) ;
#23732=EDGE_LOOP('',(#58373,#58374,#58375,#58376)) ;
#23733=EDGE_LOOP('',(#58377,#58378,#58379,#58380,#58381,#58382,#58383,#58384)) ;
#23734=EDGE_LOOP('',(#58385,#58386,#58387,#58388,#58389,#58390,#58391,#58392)) ;
#23735=EDGE_LOOP('',(#58393,#58394,#58395,#58396,#58397,#58398,#58399,#58400)) ;
#23736=EDGE_LOOP('',(#58401,#58402,#58403,#58404)) ;
#23737=EDGE_LOOP('',(#58405,#58406,#58407,#58408)) ;
#23738=EDGE_LOOP('',(#58409,#58410,#58411,#58412,#58413,#58414)) ;
#23739=EDGE_LOOP('',(#58415,#58416,#58417,#58418,#58419,#58420)) ;
#23740=EDGE_LOOP('',(#58421,#58422,#58423,#58424)) ;
#23741=EDGE_LOOP('',(#58425,#58426,#58427,#58428)) ;
#23742=EDGE_LOOP('',(#58429,#58430,#58431,#58432)) ;
#23743=EDGE_LOOP('',(#58433,#58434,#58435,#58436)) ;
#23744=EDGE_LOOP('',(#58437,#58438,#58439,#58440)) ;
#23745=EDGE_LOOP('',(#58441,#58442,#58443,#58444,#58445,#58446,#58447,#58448)) ;
#23746=EDGE_LOOP('',(#58449,#58450,#58451,#58452)) ;
#23747=EDGE_LOOP('',(#58453,#58454,#58455,#58456)) ;
#23748=EDGE_LOOP('',(#58457,#58458,#58459,#58460)) ;
#23749=EDGE_LOOP('',(#58461,#58462,#58463,#58464)) ;
#23750=EDGE_LOOP('',(#58465,#58466,#58467,#58468)) ;
#23751=EDGE_LOOP('',(#58469,#58470,#58471,#58472)) ;
#23752=EDGE_LOOP('',(#58473,#58474,#58475,#58476)) ;
#23753=EDGE_LOOP('',(#58477,#58478,#58479,#58480)) ;
#23754=EDGE_LOOP('',(#58481,#58482,#58483,#58484,#58485,#58486,#58487,#58488)) ;
#23755=EDGE_LOOP('',(#58489,#58490)) ;
#23756=EDGE_LOOP('',(#58491,#58492,#58493,#58494)) ;
#23757=EDGE_LOOP('',(#58495,#58496,#58497,#58498)) ;
#23758=EDGE_LOOP('',(#58499,#58500,#58501,#58502)) ;
#23759=EDGE_LOOP('',(#58503,#58504,#58505,#58506)) ;
#23760=EDGE_LOOP('',(#58507,#58508,#58509,#58510)) ;
#23761=EDGE_LOOP('',(#58511,#58512,#58513,#58514)) ;
#23762=EDGE_LOOP('',(#58515,#58516,#58517,#58518)) ;
#23763=EDGE_LOOP('',(#58519,#58520,#58521,#58522)) ;
#23764=EDGE_LOOP('',(#58523,#58524,#58525,#58526,#58527,#58528,#58529,#58530)) ;
#23765=EDGE_LOOP('',(#58531,#58532,#58533,#58534)) ;
#23766=EDGE_LOOP('',(#58535,#58536,#58537,#58538)) ;
#23767=EDGE_LOOP('',(#58539,#58540,#58541,#58542)) ;
#23768=EDGE_LOOP('',(#58543,#58544,#58545,#58546)) ;
#23769=EDGE_LOOP('',(#58547,#58548,#58549,#58550)) ;
#23770=EDGE_LOOP('',(#58551,#58552,#58553,#58554)) ;
#23771=EDGE_LOOP('',(#58555,#58556,#58557,#58558)) ;
#23772=EDGE_LOOP('',(#58559,#58560,#58561,#58562)) ;
#23773=EDGE_LOOP('',(#58563,#58564,#58565,#58566)) ;
#23774=EDGE_LOOP('',(#58567,#58568,#58569,#58570)) ;
#23775=EDGE_LOOP('',(#58571,#58572,#58573,#58574)) ;
#23776=EDGE_LOOP('',(#58575,#58576,#58577,#58578)) ;
#23777=EDGE_LOOP('',(#58579,#58580,#58581,#58582,#58583,#58584)) ;
#23778=EDGE_LOOP('',(#58585)) ;
#23779=EDGE_LOOP('',(#58586,#58587,#58588,#58589,#58590,#58591)) ;
#23780=EDGE_LOOP('',(#58592,#58593,#58594,#58595)) ;
#23781=EDGE_LOOP('',(#58596,#58597,#58598,#58599)) ;
#23782=EDGE_LOOP('',(#58600,#58601,#58602,#58603)) ;
#23783=EDGE_LOOP('',(#58604,#58605,#58606,#58607)) ;
#23784=EDGE_LOOP('',(#58608,#58609,#58610,#58611)) ;
#23785=EDGE_LOOP('',(#58612,#58613,#58614,#58615)) ;
#23786=EDGE_LOOP('',(#58616,#58617,#58618,#58619)) ;
#23787=EDGE_LOOP('',(#58620,#58621,#58622,#58623)) ;
#23788=EDGE_LOOP('',(#58624,#58625,#58626,#58627)) ;
#23789=EDGE_LOOP('',(#58628,#58629,#58630)) ;
#23790=EDGE_LOOP('',(#58631,#58632,#58633,#58634)) ;
#23791=EDGE_LOOP('',(#58635,#58636,#58637,#58638)) ;
#23792=EDGE_LOOP('',(#58639,#58640,#58641,#58642)) ;
#23793=EDGE_LOOP('',(#58643,#58644,#58645,#58646)) ;
#23794=EDGE_LOOP('',(#58647,#58648,#58649,#58650)) ;
#23795=EDGE_LOOP('',(#58651,#58652,#58653,#58654)) ;
#23796=EDGE_LOOP('',(#58655,#58656,#58657,#58658)) ;
#23797=EDGE_LOOP('',(#58659,#58660,#58661,#58662)) ;
#23798=EDGE_LOOP('',(#58663,#58664,#58665,#58666)) ;
#23799=EDGE_LOOP('',(#58667,#58668,#58669)) ;
#23800=EDGE_LOOP('',(#58670,#58671,#58672,#58673)) ;
#23801=EDGE_LOOP('',(#58674,#58675,#58676)) ;
#23802=EDGE_LOOP('',(#58677,#58678,#58679,#58680)) ;
#23803=EDGE_LOOP('',(#58681,#58682,#58683,#58684)) ;
#23804=EDGE_LOOP('',(#58685,#58686,#58687,#58688)) ;
#23805=EDGE_LOOP('',(#58689,#58690,#58691,#58692)) ;
#23806=EDGE_LOOP('',(#58693,#58694,#58695,#58696)) ;
#23807=EDGE_LOOP('',(#58697,#58698,#58699)) ;
#23808=EDGE_LOOP('',(#58700,#58701,#58702,#58703)) ;
#23809=EDGE_LOOP('',(#58704,#58705,#58706,#58707)) ;
#23810=EDGE_LOOP('',(#58708,#58709,#58710,#58711)) ;
#23811=EDGE_LOOP('',(#58712,#58713,#58714,#58715)) ;
#23812=EDGE_LOOP('',(#58716,#58717,#58718,#58719)) ;
#23813=EDGE_LOOP('',(#58720,#58721,#58722,#58723,#58724,#58725)) ;
#23814=EDGE_LOOP('',(#58726,#58727,#58728,#58729)) ;
#23815=EDGE_LOOP('',(#58730,#58731,#58732,#58733)) ;
#23816=EDGE_LOOP('',(#58734,#58735,#58736,#58737)) ;
#23817=EDGE_LOOP('',(#58738,#58739,#58740,#58741)) ;
#23818=EDGE_LOOP('',(#58742,#58743,#58744,#58745)) ;
#23819=EDGE_LOOP('',(#58746,#58747,#58748,#58749)) ;
#23820=EDGE_LOOP('',(#58750,#58751,#58752,#58753,#58754,#58755)) ;
#23821=EDGE_LOOP('',(#58756,#58757,#58758,#58759)) ;
#23822=EDGE_LOOP('',(#58760,#58761,#58762,#58763)) ;
#23823=EDGE_LOOP('',(#58764,#58765,#58766)) ;
#23824=EDGE_LOOP('',(#58767,#58768,#58769,#58770)) ;
#23825=EDGE_LOOP('',(#58771,#58772,#58773,#58774)) ;
#23826=EDGE_LOOP('',(#58775,#58776,#58777)) ;
#23827=EDGE_LOOP('',(#58778,#58779,#58780)) ;
#23828=EDGE_LOOP('',(#58781,#58782,#58783,#58784)) ;
#23829=EDGE_LOOP('',(#58785,#58786,#58787,#58788)) ;
#23830=EDGE_LOOP('',(#58789,#58790,#58791)) ;
#23831=EDGE_LOOP('',(#58792,#58793,#58794,#58795)) ;
#23832=EDGE_LOOP('',(#58796,#58797,#58798,#58799)) ;
#23833=EDGE_LOOP('',(#58800,#58801,#58802,#58803)) ;
#23834=EDGE_LOOP('',(#58804,#58805,#58806,#58807)) ;
#23835=EDGE_LOOP('',(#58808,#58809,#58810,#58811)) ;
#23836=EDGE_LOOP('',(#58812,#58813,#58814,#58815)) ;
#23837=EDGE_LOOP('',(#58816,#58817,#58818,#58819)) ;
#23838=EDGE_LOOP('',(#58820,#58821,#58822,#58823)) ;
#23839=EDGE_LOOP('',(#58824,#58825,#58826,#58827)) ;
#23840=EDGE_LOOP('',(#58828,#58829,#58830,#58831)) ;
#23841=EDGE_LOOP('',(#58832,#58833,#58834)) ;
#23842=EDGE_LOOP('',(#58835,#58836,#58837)) ;
#23843=EDGE_LOOP('',(#58838,#58839,#58840,#58841)) ;
#23844=EDGE_LOOP('',(#58842,#58843,#58844,#58845)) ;
#23845=EDGE_LOOP('',(#58846,#58847,#58848,#58849)) ;
#23846=EDGE_LOOP('',(#58850,#58851,#58852,#58853)) ;
#23847=EDGE_LOOP('',(#58854,#58855,#58856,#58857)) ;
#23848=EDGE_LOOP('',(#58858,#58859,#58860)) ;
#23849=EDGE_LOOP('',(#58861,#58862,#58863)) ;
#23850=EDGE_LOOP('',(#58864,#58865,#58866,#58867)) ;
#23851=EDGE_LOOP('',(#58868,#58869,#58870,#58871)) ;
#23852=EDGE_LOOP('',(#58872,#58873,#58874,#58875)) ;
#23853=EDGE_LOOP('',(#58876,#58877,#58878,#58879)) ;
#23854=EDGE_LOOP('',(#58880,#58881,#58882,#58883)) ;
#23855=EDGE_LOOP('',(#58884,#58885,#58886,#58887)) ;
#23856=EDGE_LOOP('',(#58888,#58889,#58890,#58891)) ;
#23857=EDGE_LOOP('',(#58892,#58893,#58894,#58895)) ;
#23858=EDGE_LOOP('',(#58896,#58897,#58898,#58899)) ;
#23859=EDGE_LOOP('',(#58900,#58901,#58902,#58903)) ;
#23860=EDGE_LOOP('',(#58904,#58905,#58906,#58907)) ;
#23861=EDGE_LOOP('',(#58908,#58909,#58910)) ;
#23862=EDGE_LOOP('',(#58911,#58912,#58913)) ;
#23863=EDGE_LOOP('',(#58914,#58915,#58916,#58917)) ;
#23864=EDGE_LOOP('',(#58918,#58919,#58920,#58921)) ;
#23865=EDGE_LOOP('',(#58922,#58923,#58924,#58925)) ;
#23866=EDGE_LOOP('',(#58926,#58927,#58928,#58929)) ;
#23867=EDGE_LOOP('',(#58930,#58931,#58932,#58933)) ;
#23868=EDGE_LOOP('',(#58934,#58935,#58936)) ;
#23869=EDGE_LOOP('',(#58937,#58938,#58939)) ;
#23870=EDGE_LOOP('',(#58940,#58941,#58942,#58943)) ;
#23871=EDGE_LOOP('',(#58944,#58945,#58946,#58947)) ;
#23872=EDGE_LOOP('',(#58948,#58949,#58950,#58951)) ;
#23873=EDGE_LOOP('',(#58952,#58953,#58954)) ;
#23874=EDGE_LOOP('',(#58955,#58956,#58957,#58958)) ;
#23875=EDGE_LOOP('',(#58959,#58960,#58961,#58962)) ;
#23876=EDGE_LOOP('',(#58963,#58964,#58965,#58966)) ;
#23877=EDGE_LOOP('',(#58967,#58968,#58969,#58970)) ;
#23878=EDGE_LOOP('',(#58971,#58972,#58973,#58974)) ;
#23879=EDGE_LOOP('',(#58975,#58976,#58977,#58978)) ;
#23880=EDGE_LOOP('',(#58979,#58980,#58981,#58982)) ;
#23881=EDGE_LOOP('',(#58983,#58984,#58985,#58986)) ;
#23882=EDGE_LOOP('',(#58987,#58988,#58989)) ;
#23883=EDGE_LOOP('',(#58990,#58991,#58992,#58993)) ;
#23884=EDGE_LOOP('',(#58994,#58995,#58996,#58997)) ;
#23885=EDGE_LOOP('',(#58998,#58999,#59000,#59001)) ;
#23886=EDGE_LOOP('',(#59002,#59003,#59004,#59005)) ;
#23887=EDGE_LOOP('',(#59006,#59007,#59008,#59009)) ;
#23888=EDGE_LOOP('',(#59010,#59011,#59012,#59013)) ;
#23889=EDGE_LOOP('',(#59014,#59015,#59016,#59017)) ;
#23890=EDGE_LOOP('',(#59018,#59019,#59020,#59021)) ;
#23891=EDGE_LOOP('',(#59022,#59023,#59024,#59025)) ;
#23892=EDGE_LOOP('',(#59026,#59027,#59028,#59029)) ;
#23893=EDGE_LOOP('',(#59030,#59031,#59032,#59033)) ;
#23894=EDGE_LOOP('',(#59034,#59035,#59036,#59037)) ;
#23895=EDGE_LOOP('',(#59038,#59039,#59040,#59041)) ;
#23896=EDGE_LOOP('',(#59042,#59043,#59044,#59045)) ;
#23897=EDGE_LOOP('',(#59046,#59047,#59048,#59049)) ;
#23898=EDGE_LOOP('',(#59050,#59051,#59052,#59053)) ;
#23899=EDGE_LOOP('',(#59054,#59055,#59056,#59057)) ;
#23900=EDGE_LOOP('',(#59058,#59059,#59060,#59061)) ;
#23901=EDGE_LOOP('',(#59062,#59063,#59064)) ;
#23902=EDGE_LOOP('',(#59065,#59066,#59067,#59068)) ;
#23903=EDGE_LOOP('',(#59069,#59070,#59071,#59072)) ;
#23904=EDGE_LOOP('',(#59073,#59074,#59075,#59076)) ;
#23905=EDGE_LOOP('',(#59077,#59078,#59079,#59080)) ;
#23906=EDGE_LOOP('',(#59081,#59082,#59083,#59084)) ;
#23907=EDGE_LOOP('',(#59085,#59086,#59087,#59088)) ;
#23908=EDGE_LOOP('',(#59089,#59090,#59091,#59092)) ;
#23909=EDGE_LOOP('',(#59093,#59094,#59095,#59096)) ;
#23910=EDGE_LOOP('',(#59097,#59098,#59099,#59100)) ;
#23911=EDGE_LOOP('',(#59101,#59102,#59103)) ;
#23912=EDGE_LOOP('',(#59104,#59105,#59106,#59107,#59108)) ;
#23913=EDGE_LOOP('',(#59109,#59110,#59111,#59112)) ;
#23914=EDGE_LOOP('',(#59113,#59114,#59115,#59116)) ;
#23915=EDGE_LOOP('',(#59117,#59118,#59119,#59120)) ;
#23916=EDGE_LOOP('',(#59121,#59122,#59123,#59124)) ;
#23917=EDGE_LOOP('',(#59125,#59126,#59127)) ;
#23918=EDGE_LOOP('',(#59128,#59129,#59130,#59131)) ;
#23919=EDGE_LOOP('',(#59132,#59133,#59134,#59135)) ;
#23920=EDGE_LOOP('',(#59136,#59137,#59138)) ;
#28626=CIRCLE('',#91125,0.2) ;
#28627=CIRCLE('',#91126,0.1) ;
#28628=CIRCLE('',#91127,0.1) ;
#28629=CIRCLE('',#91128,0.1) ;
#28630=CIRCLE('',#91130,2.) ;
#28631=CIRCLE('',#91131,0.1) ;
#28632=CIRCLE('',#91132,1.9) ;
#28633=CIRCLE('',#91133,1.9) ;
#28634=CIRCLE('',#91135,1.47071067811865) ;
#28635=CIRCLE('',#91136,0.1) ;
#28636=CIRCLE('',#91137,1.5) ;
#28637=CIRCLE('',#91139,1.6) ;
#28638=CIRCLE('',#91140,0.1) ;
#28639=CIRCLE('',#91141,1.5) ;
#28640=CIRCLE('',#91142,1.5) ;
#28641=CIRCLE('',#91144,0.0999999999999998) ;
#28642=CIRCLE('',#91145,0.0999999999999998) ;
#28643=CIRCLE('',#91146,0.2) ;
#28644=CIRCLE('',#91147,0.0999999999999994) ;
#28645=CIRCLE('',#91149,0.0999999999999998) ;
#28646=CIRCLE('',#91150,0.0999999999999994) ;
#28647=CIRCLE('',#91151,0.0999999999999998) ;
#28648=CIRCLE('',#91153,0.0999999999999998) ;
#28649=CIRCLE('',#91155,0.1) ;
#28650=CIRCLE('',#91156,0.0999999999999994) ;
#28651=CIRCLE('',#91157,0.1) ;
#28652=CIRCLE('',#91159,0.749999999999996) ;
#28653=CIRCLE('',#91162,1.9) ;
#28654=CIRCLE('',#91163,1.9) ;
#28655=CIRCLE('',#91164,1.9) ;
#28656=CIRCLE('',#91165,1.9) ;
#28657=CIRCLE('',#91166,1.9) ;
#28658=CIRCLE('',#91168,0.2) ;
#28659=CIRCLE('',#91169,0.1) ;
#28660=CIRCLE('',#91170,0.1) ;
#28661=CIRCLE('',#91171,0.1) ;
#28662=CIRCLE('',#91173,0.1) ;
#28663=CIRCLE('',#91174,0.1) ;
#28664=CIRCLE('',#91176,2.) ;
#28665=CIRCLE('',#91177,0.1) ;
#28666=CIRCLE('',#91178,1.9) ;
#28667=CIRCLE('',#91179,1.9) ;
#28668=CIRCLE('',#91181,1.47071067811866) ;
#28669=CIRCLE('',#91182,0.1) ;
#28670=CIRCLE('',#91183,1.5) ;
#28671=CIRCLE('',#91185,1.6) ;
#28672=CIRCLE('',#91186,0.1) ;
#28673=CIRCLE('',#91187,1.5) ;
#28674=CIRCLE('',#91188,1.5) ;
#28675=CIRCLE('',#91190,0.1) ;
#28676=CIRCLE('',#91191,0.1) ;
#28677=CIRCLE('',#91192,0.2) ;
#28678=CIRCLE('',#91193,0.0999999999999994) ;
#28679=CIRCLE('',#91195,0.1) ;
#28680=CIRCLE('',#91196,0.0999999999999994) ;
#28681=CIRCLE('',#91197,0.1) ;
#28682=CIRCLE('',#91199,0.1) ;
#28683=CIRCLE('',#91201,0.1) ;
#28684=CIRCLE('',#91202,0.0999999999999994) ;
#28685=CIRCLE('',#91203,0.1) ;
#28686=CIRCLE('',#91205,0.749999999999997) ;
#28687=CIRCLE('',#91208,1.9) ;
#28688=CIRCLE('',#91209,1.9) ;
#28689=CIRCLE('',#91210,1.9) ;
#28690=CIRCLE('',#91211,1.9) ;
#28691=CIRCLE('',#91212,1.9) ;
#28692=CIRCLE('',#91214,0.2) ;
#28693=CIRCLE('',#91215,0.2) ;
#28694=CIRCLE('',#91220,0.0999999999999994) ;
#28695=CIRCLE('',#91221,0.0999999999999998) ;
#28696=CIRCLE('',#91223,0.0999999999999994) ;
#28697=CIRCLE('',#91224,0.0999999999999998) ;
#28698=CIRCLE('',#91226,0.0999999999999994) ;
#28699=CIRCLE('',#91227,0.0999999999999998) ;
#28700=CIRCLE('',#91229,0.1) ;
#28701=CIRCLE('',#91230,0.0999999999999998) ;
#28702=CIRCLE('',#91231,0.0999999999999998) ;
#28703=CIRCLE('',#91233,3.1) ;
#28704=CIRCLE('',#91234,3.1) ;
#28705=CIRCLE('',#91239,0.2) ;
#28706=CIRCLE('',#91240,2.9) ;
#28707=CIRCLE('',#91241,0.2) ;
#28708=CIRCLE('',#91242,0.2) ;
#28709=CIRCLE('',#91243,2.9) ;
#28710=CIRCLE('',#91244,0.2) ;
#28711=CIRCLE('',#91245,0.2) ;
#28712=CIRCLE('',#91246,0.2) ;
#28713=CIRCLE('',#91256,0.2) ;
#28714=CIRCLE('',#91257,0.2) ;
#28715=CIRCLE('',#91258,0.2) ;
#28716=CIRCLE('',#91259,0.2) ;
#28717=CIRCLE('',#91260,0.2) ;
#28718=CIRCLE('',#91261,0.2) ;
#28719=CIRCLE('',#91262,0.2) ;
#28720=CIRCLE('',#91263,0.2) ;
#28721=CIRCLE('',#91269,0.2) ;
#28722=CIRCLE('',#91270,0.2) ;
#28723=CIRCLE('',#91271,0.2) ;
#28724=CIRCLE('',#91272,0.2) ;
#28725=CIRCLE('',#91273,0.2) ;
#28726=CIRCLE('',#91274,0.2) ;
#28727=CIRCLE('',#91275,0.2) ;
#28728=CIRCLE('',#91276,0.2) ;
#28729=CIRCLE('',#91280,3.1) ;
#28730=CIRCLE('',#91283,0.0999999999999998) ;
#28731=CIRCLE('',#91284,0.1) ;
#28732=CIRCLE('',#91285,0.1) ;
#28733=CIRCLE('',#91286,0.1) ;
#28734=CIRCLE('',#91287,0.1) ;
#28735=CIRCLE('',#91288,0.0999999999999998) ;
#28736=CIRCLE('',#91289,0.0999999999999998) ;
#28737=CIRCLE('',#91290,0.1) ;
#28738=CIRCLE('',#91291,0.1) ;
#28739=CIRCLE('',#91292,0.0999999999999994) ;
#28740=CIRCLE('',#91293,0.0999999999999994) ;
#28741=CIRCLE('',#91294,0.1) ;
#28742=CIRCLE('',#91295,0.1) ;
#28743=CIRCLE('',#91296,0.0999999999999998) ;
#28744=CIRCLE('',#91319,0.1) ;
#28745=CIRCLE('',#91320,0.1) ;
#28746=CIRCLE('',#91321,0.1) ;
#28747=CIRCLE('',#91322,0.1) ;
#28748=CIRCLE('',#91324,0.1) ;
#28749=CIRCLE('',#91327,0.1) ;
#28750=CIRCLE('',#91330,0.1) ;
#28751=CIRCLE('',#91333,0.1) ;
#28752=CIRCLE('',#91345,0.1) ;
#28753=CIRCLE('',#91346,0.1) ;
#28754=CIRCLE('',#91347,0.1) ;
#28755=CIRCLE('',#91348,0.1) ;
#28756=CIRCLE('',#91350,0.1) ;
#28757=CIRCLE('',#91353,0.1) ;
#28758=CIRCLE('',#91356,0.1) ;
#28759=CIRCLE('',#91359,0.1) ;
#28760=CIRCLE('',#91366,0.2) ;
#28761=CIRCLE('',#91369,3.) ;
#28762=CIRCLE('',#91370,3.) ;
#28763=CIRCLE('',#91371,3.) ;
#28764=CIRCLE('',#91372,3.) ;
#28765=CIRCLE('',#91373,0.1) ;
#28766=CIRCLE('',#91374,0.0999999999999998) ;
#28767=CIRCLE('',#91376,0.1) ;
#28768=CIRCLE('',#91377,0.0999999999999999) ;
#28769=CIRCLE('',#91380,0.1) ;
#28770=CIRCLE('',#91382,0.0999999999999997) ;
#28771=CIRCLE('',#91384,0.0999999999999998) ;
#28772=CIRCLE('',#91386,0.1) ;
#28773=CIRCLE('',#91390,0.1) ;
#28774=CIRCLE('',#91392,0.1) ;
#28775=CIRCLE('',#91394,0.1) ;
#28776=CIRCLE('',#91395,0.0999999999999998) ;
#28777=CIRCLE('',#91396,0.1) ;
#28778=CIRCLE('',#91398,0.1) ;
#28779=CIRCLE('',#91400,0.1) ;
#28780=CIRCLE('',#91402,0.1) ;
#28781=CIRCLE('',#91404,0.0999999999999998) ;
#28782=CIRCLE('',#91406,0.1) ;
#28783=CIRCLE('',#91408,0.0999999999999998) ;
#28784=CIRCLE('',#91410,0.0999999999999999) ;
#28785=CIRCLE('',#91413,0.1) ;
#28786=CIRCLE('',#91415,0.1) ;
#28787=CIRCLE('',#91417,0.0999999999999999) ;
#28788=CIRCLE('',#91419,0.1) ;
#28789=CIRCLE('',#91421,0.1) ;
#28790=CIRCLE('',#91424,0.1) ;
#28791=CIRCLE('',#91428,0.0999999999999999) ;
#28792=CIRCLE('',#91429,0.1) ;
#28793=CIRCLE('',#91435,0.1) ;
#28794=CIRCLE('',#91436,0.1) ;
#28795=CIRCLE('',#91438,0.1) ;
#28796=CIRCLE('',#91441,0.1) ;
#28797=CIRCLE('',#91442,0.1) ;
#28798=CIRCLE('',#91444,0.0999999999999994) ;
#28799=CIRCLE('',#91448,0.1) ;
#28800=CIRCLE('',#91452,0.0999999999999998) ;
#28801=CIRCLE('',#91453,0.1) ;
#28802=CIRCLE('',#91455,0.1) ;
#28803=CIRCLE('',#91457,0.0999999999999998) ;
#28804=CIRCLE('',#91459,0.0999999999999998) ;
#28805=CIRCLE('',#91461,0.1) ;
#28806=CIRCLE('',#91463,0.0999999999999998) ;
#28807=CIRCLE('',#91465,0.0999999999999994) ;
#28808=CIRCLE('',#91468,0.0999999999999998) ;
#28809=CIRCLE('',#91469,0.0999999999999998) ;
#28810=CIRCLE('',#91471,0.1) ;
#28811=CIRCLE('',#91472,0.1) ;
#28812=CIRCLE('',#91474,0.1) ;
#28813=CIRCLE('',#91475,0.1) ;
#28814=CIRCLE('',#91477,0.1) ;
#28815=CIRCLE('',#91479,0.1) ;
#28816=CIRCLE('',#91481,0.0999999999999998) ;
#28817=CIRCLE('',#91482,0.0999999999999998) ;
#28818=CIRCLE('',#91484,0.1) ;
#28819=CIRCLE('',#91486,0.1) ;
#28820=CIRCLE('',#91488,0.1) ;
#28821=CIRCLE('',#91489,0.1) ;
#28822=CIRCLE('',#91491,0.1) ;
#28823=CIRCLE('',#91493,0.1) ;
#28824=CIRCLE('',#91495,0.1) ;
#28825=CIRCLE('',#91497,0.1) ;
#28826=CIRCLE('',#91499,0.1) ;
#28827=CIRCLE('',#91501,0.1) ;
#28828=CIRCLE('',#91503,0.1) ;
#28829=CIRCLE('',#91505,0.1) ;
#28830=CIRCLE('',#91507,0.1) ;
#28831=CIRCLE('',#91509,0.1) ;
#28832=CIRCLE('',#91512,0.1) ;
#28833=CIRCLE('',#91513,0.0999999999999998) ;
#28834=CIRCLE('',#91515,0.1) ;
#28835=CIRCLE('',#91516,0.1) ;
#28836=CIRCLE('',#91518,0.1) ;
#28837=CIRCLE('',#91519,0.1) ;
#28838=CIRCLE('',#91521,0.1) ;
#28839=CIRCLE('',#91523,0.1) ;
#28840=CIRCLE('',#91525,0.0999999999999998) ;
#28841=CIRCLE('',#91526,0.0999999999999998) ;
#28842=CIRCLE('',#91528,0.1) ;
#28843=CIRCLE('',#91530,0.1) ;
#28844=CIRCLE('',#91532,0.0999999999999998) ;
#28845=CIRCLE('',#91533,0.0999999999999998) ;
#28846=CIRCLE('',#91535,0.1) ;
#28847=CIRCLE('',#91537,0.1) ;
#28848=CIRCLE('',#91539,0.1) ;
#28849=CIRCLE('',#91541,0.1) ;
#28850=CIRCLE('',#91543,0.1) ;
#28851=CIRCLE('',#91545,0.1) ;
#28852=CIRCLE('',#91547,0.1) ;
#28853=CIRCLE('',#91549,0.1) ;
#28854=CIRCLE('',#91551,0.0999999999999998) ;
#28855=CIRCLE('',#91553,0.0999999999999998) ;
#28856=CIRCLE('',#91556,0.1) ;
#28857=CIRCLE('',#91558,0.1) ;
#28858=CIRCLE('',#91560,0.1) ;
#28859=CIRCLE('',#91562,0.0999999999999998) ;
#28860=CIRCLE('',#91564,0.0999999999999994) ;
#28861=CIRCLE('',#91566,0.0999999999999999) ;
#28862=CIRCLE('',#91568,0.0999999999999999) ;
#28863=CIRCLE('',#91570,0.0999999999999994) ;
#28864=CIRCLE('',#91571,0.0999999999999994) ;
#28865=CIRCLE('',#91573,0.1) ;
#28866=CIRCLE('',#91575,0.0999999999999998) ;
#28867=CIRCLE('',#91577,0.1) ;
#28868=CIRCLE('',#91578,0.0999999999999998) ;
#28869=CIRCLE('',#91580,0.1) ;
#28870=CIRCLE('',#91583,0.0999999999999998) ;
#28871=CIRCLE('',#91585,0.0999999999999998) ;
#28872=CIRCLE('',#91587,0.1) ;
#28873=CIRCLE('',#91589,0.1) ;
#28874=CIRCLE('',#91591,0.1) ;
#28875=CIRCLE('',#91593,0.1) ;
#28876=CIRCLE('',#91599,0.0999999999999998) ;
#28877=CIRCLE('',#91601,0.0999999999999998) ;
#28878=CIRCLE('',#91603,0.1) ;
#28879=CIRCLE('',#91605,0.1) ;
#28880=CIRCLE('',#91607,0.1) ;
#28881=CIRCLE('',#91609,0.1) ;
#28882=CIRCLE('',#91610,0.1) ;
#28883=CIRCLE('',#91611,0.1) ;
#28884=CIRCLE('',#91614,0.1) ;
#28885=CIRCLE('',#91615,0.1) ;
#28886=CIRCLE('',#91616,0.1) ;
#28887=CIRCLE('',#91618,0.1) ;
#28888=CIRCLE('',#91622,0.1) ;
#28889=CIRCLE('',#91624,0.1) ;
#28890=CIRCLE('',#91625,0.1) ;
#28891=CIRCLE('',#91626,0.1) ;
#28892=CIRCLE('',#91627,0.0999999999999998) ;
#28893=CIRCLE('',#91628,0.1) ;
#28894=CIRCLE('',#91632,0.100000000000001) ;
#28895=CIRCLE('',#91633,0.100000000000001) ;
#28896=CIRCLE('',#91636,0.0999999999999994) ;
#28897=CIRCLE('',#91637,0.0999999999999994) ;
#28898=CIRCLE('',#91640,0.100000000000001) ;
#28899=CIRCLE('',#91641,0.100000000000001) ;
#28900=CIRCLE('',#91644,0.0999999999999994) ;
#28901=CIRCLE('',#91645,0.0999999999999994) ;
#28902=CIRCLE('',#91648,0.199999999999999) ;
#28903=CIRCLE('',#91650,0.199999999999999) ;
#28904=CIRCLE('',#91652,3.1) ;
#28905=CIRCLE('',#91657,0.1) ;
#28906=CIRCLE('',#91658,0.1) ;
#28907=CIRCLE('',#91659,0.0999999999999994) ;
#28908=CIRCLE('',#91660,0.0999999999999994) ;
#28909=CIRCLE('',#91661,0.1) ;
#28910=CIRCLE('',#91684,0.1) ;
#28911=CIRCLE('',#91685,0.1) ;
#28912=CIRCLE('',#91686,0.1) ;
#28913=CIRCLE('',#91687,0.1) ;
#28914=CIRCLE('',#91689,0.1) ;
#28915=CIRCLE('',#91692,0.1) ;
#28916=CIRCLE('',#91695,0.1) ;
#28917=CIRCLE('',#91698,0.1) ;
#28918=CIRCLE('',#91710,0.1) ;
#28919=CIRCLE('',#91711,0.1) ;
#28920=CIRCLE('',#91712,0.1) ;
#28921=CIRCLE('',#91713,0.1) ;
#28922=CIRCLE('',#91715,0.1) ;
#28923=CIRCLE('',#91718,0.1) ;
#28924=CIRCLE('',#91721,0.1) ;
#28925=CIRCLE('',#91724,0.1) ;
#28926=CIRCLE('',#91731,0.2) ;
#28927=CIRCLE('',#91734,3.) ;
#28928=CIRCLE('',#91735,3.) ;
#28929=CIRCLE('',#91736,3.) ;
#28930=CIRCLE('',#91737,3.) ;
#28931=CIRCLE('',#91738,0.1) ;
#28932=CIRCLE('',#91739,0.0999999999999998) ;
#28933=CIRCLE('',#91741,0.0999999999999999) ;
#28934=CIRCLE('',#91742,0.0999999999999999) ;
#28935=CIRCLE('',#91745,0.1) ;
#28936=CIRCLE('',#91747,0.0999999999999997) ;
#28937=CIRCLE('',#91749,0.0999999999999998) ;
#28938=CIRCLE('',#91751,0.1) ;
#28939=CIRCLE('',#91755,0.0999999999999999) ;
#28940=CIRCLE('',#91757,0.1) ;
#28941=CIRCLE('',#91759,0.1) ;
#28942=CIRCLE('',#91760,0.1) ;
#28943=CIRCLE('',#91761,0.1) ;
#28944=CIRCLE('',#91763,0.1) ;
#28945=CIRCLE('',#91765,0.1) ;
#28946=CIRCLE('',#91767,0.1) ;
#28947=CIRCLE('',#91769,0.1) ;
#28948=CIRCLE('',#91771,0.1) ;
#28949=CIRCLE('',#91773,0.0999999999999998) ;
#28950=CIRCLE('',#91775,0.1) ;
#28951=CIRCLE('',#91778,0.1) ;
#28952=CIRCLE('',#91780,0.0999999999999999) ;
#28953=CIRCLE('',#91782,0.0999999999999999) ;
#28954=CIRCLE('',#91784,0.1) ;
#28955=CIRCLE('',#91786,0.1) ;
#28956=CIRCLE('',#91789,0.1) ;
#28957=CIRCLE('',#91793,0.0999999999999999) ;
#28958=CIRCLE('',#91794,0.0999999999999999) ;
#28959=CIRCLE('',#91800,0.1) ;
#28960=CIRCLE('',#91801,0.1) ;
#28961=CIRCLE('',#91803,0.1) ;
#28962=CIRCLE('',#91806,0.1) ;
#28963=CIRCLE('',#91807,0.1) ;
#28964=CIRCLE('',#91809,0.0999999999999994) ;
#28965=CIRCLE('',#91812,0.0999999999999998) ;
#28966=CIRCLE('',#91816,0.0999999999999998) ;
#28967=CIRCLE('',#91817,0.1) ;
#28968=CIRCLE('',#91819,0.1) ;
#28969=CIRCLE('',#91821,0.0999999999999998) ;
#28970=CIRCLE('',#91823,0.0999999999999998) ;
#28971=CIRCLE('',#91825,0.1) ;
#28972=CIRCLE('',#91827,0.0999999999999998) ;
#28973=CIRCLE('',#91829,0.0999999999999994) ;
#28974=CIRCLE('',#91832,0.0999999999999998) ;
#28975=CIRCLE('',#91833,0.0999999999999998) ;
#28976=CIRCLE('',#91835,0.1) ;
#28977=CIRCLE('',#91836,0.1) ;
#28978=CIRCLE('',#91838,0.1) ;
#28979=CIRCLE('',#91839,0.1) ;
#28980=CIRCLE('',#91841,0.0999999999999998) ;
#28981=CIRCLE('',#91843,0.1) ;
#28982=CIRCLE('',#91845,0.0999999999999998) ;
#28983=CIRCLE('',#91846,0.0999999999999998) ;
#28984=CIRCLE('',#91848,0.1) ;
#28985=CIRCLE('',#91850,0.1) ;
#28986=CIRCLE('',#91852,0.1) ;
#28987=CIRCLE('',#91853,0.1) ;
#28988=CIRCLE('',#91855,0.1) ;
#28989=CIRCLE('',#91857,0.1) ;
#28990=CIRCLE('',#91859,0.1) ;
#28991=CIRCLE('',#91861,0.1) ;
#28992=CIRCLE('',#91863,0.1) ;
#28993=CIRCLE('',#91865,0.1) ;
#28994=CIRCLE('',#91867,0.1) ;
#28995=CIRCLE('',#91869,0.1) ;
#28996=CIRCLE('',#91871,0.1) ;
#28997=CIRCLE('',#91873,0.1) ;
#28998=CIRCLE('',#91876,0.1) ;
#28999=CIRCLE('',#91877,0.0999999999999998) ;
#29000=CIRCLE('',#91879,0.0999999999999998) ;
#29001=CIRCLE('',#91880,0.1) ;
#29002=CIRCLE('',#91882,0.1) ;
#29003=CIRCLE('',#91883,0.1) ;
#29004=CIRCLE('',#91885,0.1) ;
#29005=CIRCLE('',#91887,0.1) ;
#29006=CIRCLE('',#91889,0.0999999999999998) ;
#29007=CIRCLE('',#91890,0.0999999999999998) ;
#29008=CIRCLE('',#91892,0.1) ;
#29009=CIRCLE('',#91894,0.1) ;
#29010=CIRCLE('',#91896,0.0999999999999998) ;
#29011=CIRCLE('',#91897,0.0999999999999998) ;
#29012=CIRCLE('',#91899,0.1) ;
#29013=CIRCLE('',#91901,0.1) ;
#29014=CIRCLE('',#91903,0.1) ;
#29015=CIRCLE('',#91905,0.1) ;
#29016=CIRCLE('',#91907,0.1) ;
#29017=CIRCLE('',#91909,0.1) ;
#29018=CIRCLE('',#91911,0.1) ;
#29019=CIRCLE('',#91913,0.1) ;
#29020=CIRCLE('',#91915,0.0999999999999998) ;
#29021=CIRCLE('',#91917,0.0999999999999998) ;
#29022=CIRCLE('',#91920,0.1) ;
#29023=CIRCLE('',#91922,0.0999999999999998) ;
#29024=CIRCLE('',#91924,0.0999999999999998) ;
#29025=CIRCLE('',#91926,0.1) ;
#29026=CIRCLE('',#91928,0.1) ;
#29027=CIRCLE('',#91930,0.0999999999999994) ;
#29028=CIRCLE('',#91932,0.1) ;
#29029=CIRCLE('',#91934,0.1) ;
#29030=CIRCLE('',#91936,0.0999999999999998) ;
#29031=CIRCLE('',#91938,0.1) ;
#29032=CIRCLE('',#91945,0.0999999999999998) ;
#29033=CIRCLE('',#91947,0.0999999999999998) ;
#29034=CIRCLE('',#91949,0.1) ;
#29035=CIRCLE('',#91950,0.1) ;
#29036=CIRCLE('',#91952,0.1) ;
#29037=CIRCLE('',#91953,0.1) ;
#29038=CIRCLE('',#91955,0.1) ;
#29039=CIRCLE('',#91959,0.1) ;
#29040=CIRCLE('',#91960,0.1) ;
#29041=CIRCLE('',#91961,0.0999999999999998) ;
#29042=CIRCLE('',#91962,0.1) ;
#29043=CIRCLE('',#91964,0.0999999999999995) ;
#29044=CIRCLE('',#91965,0.0999999999999998) ;
#29045=CIRCLE('',#91967,0.1) ;
#29046=CIRCLE('',#91968,0.0999999999999995) ;
#29047=CIRCLE('',#91970,0.0999999999999998) ;
#29048=CIRCLE('',#91972,0.1) ;
#29049=CIRCLE('',#91974,0.1) ;
#29050=CIRCLE('',#91976,0.1) ;
#29051=CIRCLE('',#91978,0.1) ;
#29052=CIRCLE('',#91980,0.0999999999999999) ;
#29053=CIRCLE('',#91982,0.0999999999999999) ;
#29054=CIRCLE('',#91984,0.1) ;
#29055=CIRCLE('',#91986,0.1) ;
#29056=CIRCLE('',#91989,0.1) ;
#29057=CIRCLE('',#91990,0.1) ;
#29058=CIRCLE('',#91993,0.0999999999999999) ;
#29059=CIRCLE('',#91995,0.0999999999999998) ;
#29060=CIRCLE('',#91996,0.0999999999999998) ;
#29061=CIRCLE('',#91997,0.1) ;
#29062=CIRCLE('',#91999,0.1) ;
#29063=CIRCLE('',#92001,0.0999999999999998) ;
#29064=CIRCLE('',#92003,0.0999999999999998) ;
#29065=CIRCLE('',#92005,0.1) ;
#29066=CIRCLE('',#92007,0.1) ;
#29067=CIRCLE('',#92009,0.1) ;
#29068=CIRCLE('',#92011,0.1) ;
#29069=CIRCLE('',#92014,0.199999999999999) ;
#29070=CIRCLE('',#92015,0.0999999999999994) ;
#29071=CIRCLE('',#92016,0.0999999999999994) ;
#29072=CIRCLE('',#92017,0.100000000000001) ;
#29073=CIRCLE('',#92019,2.) ;
#29074=CIRCLE('',#92020,0.1) ;
#29075=CIRCLE('',#92021,1.9) ;
#29076=CIRCLE('',#92022,1.9) ;
#29077=CIRCLE('',#92024,1.47071067811865) ;
#29078=CIRCLE('',#92025,0.1) ;
#29079=CIRCLE('',#92026,1.5) ;
#29080=CIRCLE('',#92028,1.6) ;
#29081=CIRCLE('',#92029,0.1) ;
#29082=CIRCLE('',#92030,1.5) ;
#29083=CIRCLE('',#92031,1.5) ;
#29084=CIRCLE('',#92033,0.0999999999999994) ;
#29085=CIRCLE('',#92034,0.0999999999999994) ;
#29086=CIRCLE('',#92035,0.200000000000001) ;
#29087=CIRCLE('',#92036,0.0999999999999994) ;
#29088=CIRCLE('',#92038,0.0999999999999994) ;
#29089=CIRCLE('',#92039,0.0999999999999994) ;
#29090=CIRCLE('',#92040,0.0999999999999994) ;
#29091=CIRCLE('',#92042,0.0999999999999994) ;
#29092=CIRCLE('',#92044,0.0999999999999994) ;
#29093=CIRCLE('',#92045,0.0999999999999994) ;
#29094=CIRCLE('',#92046,0.0999999999999994) ;
#29095=CIRCLE('',#92048,0.749999999999997) ;
#29096=CIRCLE('',#92051,1.9) ;
#29097=CIRCLE('',#92052,1.9) ;
#29098=CIRCLE('',#92053,1.9) ;
#29099=CIRCLE('',#92054,1.9) ;
#29100=CIRCLE('',#92055,1.9) ;
#29101=CIRCLE('',#92057,0.199999999999999) ;
#29102=CIRCLE('',#92058,0.0999999999999994) ;
#29103=CIRCLE('',#92059,0.0999999999999994) ;
#29104=CIRCLE('',#92060,0.100000000000001) ;
#29105=CIRCLE('',#92062,0.1) ;
#29106=CIRCLE('',#92063,0.1) ;
#29107=CIRCLE('',#92065,2.) ;
#29108=CIRCLE('',#92066,0.1) ;
#29109=CIRCLE('',#92067,1.9) ;
#29110=CIRCLE('',#92068,1.9) ;
#29111=CIRCLE('',#92070,1.47071067811865) ;
#29112=CIRCLE('',#92071,0.1) ;
#29113=CIRCLE('',#92072,1.5) ;
#29114=CIRCLE('',#92074,1.6) ;
#29115=CIRCLE('',#92075,0.1) ;
#29116=CIRCLE('',#92076,1.5) ;
#29117=CIRCLE('',#92077,1.5) ;
#29118=CIRCLE('',#92079,0.0999999999999994) ;
#29119=CIRCLE('',#92080,0.0999999999999994) ;
#29120=CIRCLE('',#92081,0.199999999999999) ;
#29121=CIRCLE('',#92082,0.0999999999999994) ;
#29122=CIRCLE('',#92084,0.0999999999999994) ;
#29123=CIRCLE('',#92085,0.0999999999999994) ;
#29124=CIRCLE('',#92086,0.0999999999999994) ;
#29125=CIRCLE('',#92088,0.0999999999999994) ;
#29126=CIRCLE('',#92090,0.0999999999999994) ;
#29127=CIRCLE('',#92091,0.0999999999999994) ;
#29128=CIRCLE('',#92092,0.0999999999999994) ;
#29129=CIRCLE('',#92094,0.749999999999997) ;
#29130=CIRCLE('',#92097,1.9) ;
#29131=CIRCLE('',#92098,1.9) ;
#29132=CIRCLE('',#92099,1.9) ;
#29133=CIRCLE('',#92100,1.9) ;
#29134=CIRCLE('',#92101,1.9) ;
#29135=CIRCLE('',#92103,0.199999999999999) ;
#29136=CIRCLE('',#92104,0.199999999999999) ;
#29137=CIRCLE('',#92109,0.0999999999999998) ;
#29138=CIRCLE('',#92110,0.0999999999999998) ;
#29139=CIRCLE('',#92112,0.0999999999999998) ;
#29140=CIRCLE('',#92113,0.0999999999999998) ;
#29141=CIRCLE('',#92115,0.0999999999999998) ;
#29142=CIRCLE('',#92116,0.0999999999999998) ;
#29143=CIRCLE('',#92118,0.0999999999999998) ;
#29144=CIRCLE('',#92119,0.0999999999999998) ;
#29145=CIRCLE('',#92120,0.0999999999999998) ;
#29146=CIRCLE('',#92122,3.1) ;
#29147=CIRCLE('',#92127,0.199999999999999) ;
#29148=CIRCLE('',#92128,0.200000000000001) ;
#29149=CIRCLE('',#92129,2.9) ;
#29150=CIRCLE('',#92130,0.199999999999999) ;
#29151=CIRCLE('',#92131,0.199999999999999) ;
#29152=CIRCLE('',#92132,2.9) ;
#29153=CIRCLE('',#92133,0.199999999999999) ;
#29154=CIRCLE('',#92134,0.199999999999999) ;
#29155=CIRCLE('',#92144,0.199999999999999) ;
#29156=CIRCLE('',#92145,0.200000000000001) ;
#29157=CIRCLE('',#92146,0.200000000000001) ;
#29158=CIRCLE('',#92147,0.199999999999999) ;
#29159=CIRCLE('',#92148,0.199999999999999) ;
#29160=CIRCLE('',#92149,0.199999999999999) ;
#29161=CIRCLE('',#92150,0.199999999999999) ;
#29162=CIRCLE('',#92151,0.199999999999999) ;
#29163=CIRCLE('',#92157,0.199999999999999) ;
#29164=CIRCLE('',#92158,0.200000000000001) ;
#29165=CIRCLE('',#92159,0.200000000000001) ;
#29166=CIRCLE('',#92160,0.199999999999999) ;
#29167=CIRCLE('',#92161,0.199999999999999) ;
#29168=CIRCLE('',#92162,0.199999999999999) ;
#29169=CIRCLE('',#92163,0.199999999999999) ;
#29170=CIRCLE('',#92164,0.199999999999999) ;
#29171=CIRCLE('',#92168,3.1) ;
#29172=CIRCLE('',#92169,3.1) ;
#29173=CIRCLE('',#92172,0.0999999999999998) ;
#29174=CIRCLE('',#92173,0.0999999999999998) ;
#29175=CIRCLE('',#92174,0.1) ;
#29176=CIRCLE('',#92175,0.1) ;
#29177=CIRCLE('',#92176,0.0999999999999994) ;
#29178=CIRCLE('',#92177,0.0999999999999994) ;
#29179=CIRCLE('',#92178,0.1) ;
#29180=CIRCLE('',#92179,0.1) ;
#29181=CIRCLE('',#92180,0.0999999999999998) ;
#29182=CIRCLE('',#92181,0.0999999999999998) ;
#29183=CIRCLE('',#92182,0.1) ;
#29184=CIRCLE('',#92183,0.1) ;
#29185=CIRCLE('',#92184,0.1) ;
#29186=CIRCLE('',#92185,0.1) ;
#29187=CIRCLE('',#92208,0.0999999999999994) ;
#29188=CIRCLE('',#92209,0.0999999999999994) ;
#29189=CIRCLE('',#92210,0.0999999999999994) ;
#29190=CIRCLE('',#92211,0.0999999999999994) ;
#29191=CIRCLE('',#92213,0.0999999999999994) ;
#29192=CIRCLE('',#92216,0.0999999999999994) ;
#29193=CIRCLE('',#92219,0.0999999999999994) ;
#29194=CIRCLE('',#92222,0.0999999999999994) ;
#29195=CIRCLE('',#92234,0.0999999999999994) ;
#29196=CIRCLE('',#92235,0.0999999999999994) ;
#29197=CIRCLE('',#92236,0.0999999999999994) ;
#29198=CIRCLE('',#92237,0.0999999999999994) ;
#29199=CIRCLE('',#92239,0.0999999999999994) ;
#29200=CIRCLE('',#92242,0.0999999999999994) ;
#29201=CIRCLE('',#92245,0.0999999999999994) ;
#29202=CIRCLE('',#92248,0.0999999999999994) ;
#29203=CIRCLE('',#92255,0.199999999999999) ;
#29204=CIRCLE('',#92258,3.) ;
#29205=CIRCLE('',#92259,3.) ;
#29206=CIRCLE('',#92260,3.) ;
#29207=CIRCLE('',#92261,3.) ;
#29208=CIRCLE('',#92262,0.1) ;
#29209=CIRCLE('',#92263,0.0999999999999994) ;
#29210=CIRCLE('',#92265,0.100000000000002) ;
#29211=CIRCLE('',#92266,0.1) ;
#29212=CIRCLE('',#92269,0.1) ;
#29213=CIRCLE('',#92271,0.0999999999999997) ;
#29214=CIRCLE('',#92273,0.0999999999999994) ;
#29215=CIRCLE('',#92275,0.1) ;
#29216=CIRCLE('',#92279,0.100000000000002) ;
#29217=CIRCLE('',#92281,0.1) ;
#29218=CIRCLE('',#92283,0.1) ;
#29219=CIRCLE('',#92284,0.0999999999999994) ;
#29220=CIRCLE('',#92285,0.0999999999999999) ;
#29221=CIRCLE('',#92287,0.1) ;
#29222=CIRCLE('',#92289,0.1) ;
#29223=CIRCLE('',#92291,0.1) ;
#29224=CIRCLE('',#92293,0.0999999999999994) ;
#29225=CIRCLE('',#92295,0.1) ;
#29226=CIRCLE('',#92297,0.0999999999999998) ;
#29227=CIRCLE('',#92299,0.0999999999999998) ;
#29228=CIRCLE('',#92302,0.1) ;
#29229=CIRCLE('',#92304,0.100000000000002) ;
#29230=CIRCLE('',#92306,0.0999999999999999) ;
#29231=CIRCLE('',#92308,0.1) ;
#29232=CIRCLE('',#92310,0.1) ;
#29233=CIRCLE('',#92313,0.1) ;
#29234=CIRCLE('',#92317,0.0999999999999999) ;
#29235=CIRCLE('',#92318,0.100000000000002) ;
#29236=CIRCLE('',#92324,0.0999999999999994) ;
#29237=CIRCLE('',#92325,0.0999999999999994) ;
#29238=CIRCLE('',#92327,0.0999999999999994) ;
#29239=CIRCLE('',#92330,0.1) ;
#29240=CIRCLE('',#92331,0.1) ;
#29241=CIRCLE('',#92333,0.0999999999999994) ;
#29242=CIRCLE('',#92337,0.0999999999999994) ;
#29243=CIRCLE('',#92341,0.0999999999999998) ;
#29244=CIRCLE('',#92342,0.0999999999999994) ;
#29245=CIRCLE('',#92344,0.0999999999999994) ;
#29246=CIRCLE('',#92346,0.0999999999999998) ;
#29247=CIRCLE('',#92348,0.0999999999999998) ;
#29248=CIRCLE('',#92350,0.0999999999999994) ;
#29249=CIRCLE('',#92352,0.0999999999999998) ;
#29250=CIRCLE('',#92354,0.0999999999999994) ;
#29251=CIRCLE('',#92357,0.0999999999999998) ;
#29252=CIRCLE('',#92358,0.0999999999999998) ;
#29253=CIRCLE('',#92360,0.0999999999999994) ;
#29254=CIRCLE('',#92361,0.0999999999999994) ;
#29255=CIRCLE('',#92363,0.0999999999999994) ;
#29256=CIRCLE('',#92364,0.0999999999999994) ;
#29257=CIRCLE('',#92366,0.0999999999999994) ;
#29258=CIRCLE('',#92368,0.0999999999999994) ;
#29259=CIRCLE('',#92370,0.0999999999999998) ;
#29260=CIRCLE('',#92371,0.0999999999999998) ;
#29261=CIRCLE('',#92373,0.0999999999999994) ;
#29262=CIRCLE('',#92375,0.0999999999999994) ;
#29263=CIRCLE('',#92377,0.1) ;
#29264=CIRCLE('',#92378,0.1) ;
#29265=CIRCLE('',#92380,0.0999999999999994) ;
#29266=CIRCLE('',#92382,0.0999999999999994) ;
#29267=CIRCLE('',#92384,0.0999999999999994) ;
#29268=CIRCLE('',#92386,0.0999999999999994) ;
#29269=CIRCLE('',#92388,0.0999999999999994) ;
#29270=CIRCLE('',#92390,0.0999999999999994) ;
#29271=CIRCLE('',#92392,0.0999999999999994) ;
#29272=CIRCLE('',#92394,0.0999999999999994) ;
#29273=CIRCLE('',#92396,0.1) ;
#29274=CIRCLE('',#92398,0.1) ;
#29275=CIRCLE('',#92401,0.1) ;
#29276=CIRCLE('',#92402,0.0999999999999998) ;
#29277=CIRCLE('',#92404,0.0999999999999994) ;
#29278=CIRCLE('',#92405,0.0999999999999994) ;
#29279=CIRCLE('',#92407,0.0999999999999994) ;
#29280=CIRCLE('',#92408,0.0999999999999994) ;
#29281=CIRCLE('',#92410,0.0999999999999994) ;
#29282=CIRCLE('',#92412,0.0999999999999994) ;
#29283=CIRCLE('',#92414,0.0999999999999998) ;
#29284=CIRCLE('',#92415,0.0999999999999998) ;
#29285=CIRCLE('',#92417,0.0999999999999994) ;
#29286=CIRCLE('',#92419,0.0999999999999994) ;
#29287=CIRCLE('',#92421,0.0999999999999998) ;
#29288=CIRCLE('',#92422,0.0999999999999998) ;
#29289=CIRCLE('',#92424,0.0999999999999994) ;
#29290=CIRCLE('',#92426,0.0999999999999994) ;
#29291=CIRCLE('',#92428,0.0999999999999994) ;
#29292=CIRCLE('',#92430,0.0999999999999994) ;
#29293=CIRCLE('',#92432,0.0999999999999994) ;
#29294=CIRCLE('',#92434,0.0999999999999994) ;
#29295=CIRCLE('',#92436,0.0999999999999994) ;
#29296=CIRCLE('',#92438,0.0999999999999994) ;
#29297=CIRCLE('',#92440,0.0999999999999998) ;
#29298=CIRCLE('',#92442,0.0999999999999998) ;
#29299=CIRCLE('',#92445,0.100000000000001) ;
#29300=CIRCLE('',#92447,0.0999999999999998) ;
#29301=CIRCLE('',#92448,0.1) ;
#29302=CIRCLE('',#92450,0.0999999999999994) ;
#29303=CIRCLE('',#92452,0.0999999999999994) ;
#29304=CIRCLE('',#92454,0.0999999999999994) ;
#29305=CIRCLE('',#92455,0.0999999999999994) ;
#29306=CIRCLE('',#92457,0.099999999999999) ;
#29307=CIRCLE('',#92459,0.099999999999999) ;
#29308=CIRCLE('',#92461,0.0999999999999994) ;
#29309=CIRCLE('',#92463,0.0999999999999994) ;
#29310=CIRCLE('',#92465,0.0999999999999994) ;
#29311=CIRCLE('',#92467,0.0999999999999998) ;
#29312=CIRCLE('',#92469,0.099999999999999) ;
#29313=CIRCLE('',#92472,0.0999999999999998) ;
#29314=CIRCLE('',#92474,0.0999999999999998) ;
#29315=CIRCLE('',#92476,0.1) ;
#29316=CIRCLE('',#92478,0.1) ;
#29317=CIRCLE('',#92480,0.1) ;
#29318=CIRCLE('',#92482,0.1) ;
#29319=CIRCLE('',#92488,0.0999999999999998) ;
#29320=CIRCLE('',#92490,0.0999999999999998) ;
#29321=CIRCLE('',#92492,0.1) ;
#29322=CIRCLE('',#92494,0.0999999999999994) ;
#29323=CIRCLE('',#92496,0.0999999999999994) ;
#29324=CIRCLE('',#92498,0.100000000000001) ;
#29325=CIRCLE('',#92499,0.1) ;
#29326=CIRCLE('',#92500,0.1) ;
#29327=CIRCLE('',#92502,0.1) ;
#29328=CIRCLE('',#92504,0.1) ;
#29329=CIRCLE('',#92505,0.0999999999999998) ;
#29330=CIRCLE('',#92507,0.0999999999999994) ;
#29331=CIRCLE('',#92511,0.1) ;
#29332=CIRCLE('',#92512,0.1) ;
#29333=CIRCLE('',#92514,0.1) ;
#29334=CIRCLE('',#92515,0.100000000000001) ;
#29335=CIRCLE('',#92516,0.0999999999999998) ;
#29336=CIRCLE('',#92517,0.100000000000001) ;
#29337=CIRCLE('',#92521,0.100000000000001) ;
#29338=CIRCLE('',#92522,0.100000000000001) ;
#29339=CIRCLE('',#92525,0.0999999999999994) ;
#29340=CIRCLE('',#92526,0.0999999999999994) ;
#29341=CIRCLE('',#92529,0.100000000000001) ;
#29342=CIRCLE('',#92530,0.100000000000001) ;
#29343=CIRCLE('',#92533,0.0999999999999994) ;
#29344=CIRCLE('',#92534,0.0999999999999994) ;
#29345=CIRCLE('',#92537,0.199999999999999) ;
#29346=CIRCLE('',#92539,0.199999999999999) ;
#29347=CIRCLE('',#92544,3.1) ;
#29348=CIRCLE('',#92546,0.1) ;
#29349=CIRCLE('',#92547,0.1) ;
#29350=CIRCLE('',#92548,0.0999999999999994) ;
#29351=CIRCLE('',#92549,0.0999999999999994) ;
#29352=CIRCLE('',#92550,0.1) ;
#29353=CIRCLE('',#92573,0.0999999999999994) ;
#29354=CIRCLE('',#92574,0.0999999999999994) ;
#29355=CIRCLE('',#92575,0.0999999999999994) ;
#29356=CIRCLE('',#92576,0.0999999999999994) ;
#29357=CIRCLE('',#92578,0.0999999999999994) ;
#29358=CIRCLE('',#92581,0.0999999999999994) ;
#29359=CIRCLE('',#92584,0.0999999999999994) ;
#29360=CIRCLE('',#92587,0.0999999999999994) ;
#29361=CIRCLE('',#92599,0.0999999999999994) ;
#29362=CIRCLE('',#92600,0.0999999999999994) ;
#29363=CIRCLE('',#92601,0.0999999999999994) ;
#29364=CIRCLE('',#92602,0.0999999999999994) ;
#29365=CIRCLE('',#92604,0.0999999999999994) ;
#29366=CIRCLE('',#92607,0.0999999999999994) ;
#29367=CIRCLE('',#92610,0.0999999999999994) ;
#29368=CIRCLE('',#92613,0.0999999999999994) ;
#29369=CIRCLE('',#92620,0.200000000000001) ;
#29370=CIRCLE('',#92623,3.) ;
#29371=CIRCLE('',#92624,3.) ;
#29372=CIRCLE('',#92625,3.) ;
#29373=CIRCLE('',#92626,3.) ;
#29374=CIRCLE('',#92627,0.1) ;
#29375=CIRCLE('',#92628,0.0999999999999994) ;
#29376=CIRCLE('',#92630,0.0999999999999999) ;
#29377=CIRCLE('',#92631,0.0999999999999999) ;
#29378=CIRCLE('',#92634,0.1) ;
#29379=CIRCLE('',#92636,0.0999999999999997) ;
#29380=CIRCLE('',#92638,0.0999999999999994) ;
#29381=CIRCLE('',#92640,0.1) ;
#29382=CIRCLE('',#92644,0.100000000000002) ;
#29383=CIRCLE('',#92646,0.1) ;
#29384=CIRCLE('',#92648,0.1) ;
#29385=CIRCLE('',#92649,0.0999999999999994) ;
#29386=CIRCLE('',#92650,0.0999999999999999) ;
#29387=CIRCLE('',#92652,0.1) ;
#29388=CIRCLE('',#92654,0.1) ;
#29389=CIRCLE('',#92656,0.1) ;
#29390=CIRCLE('',#92658,0.0999999999999994) ;
#29391=CIRCLE('',#92660,0.1) ;
#29392=CIRCLE('',#92662,0.0999999999999998) ;
#29393=CIRCLE('',#92664,0.1) ;
#29394=CIRCLE('',#92667,0.1) ;
#29395=CIRCLE('',#92669,0.0999999999999999) ;
#29396=CIRCLE('',#92671,0.0999999999999999) ;
#29397=CIRCLE('',#92673,0.1) ;
#29398=CIRCLE('',#92675,0.1) ;
#29399=CIRCLE('',#92678,0.1) ;
#29400=CIRCLE('',#92682,0.0999999999999999) ;
#29401=CIRCLE('',#92683,0.100000000000002) ;
#29402=CIRCLE('',#92688,0.0999999999999994) ;
#29403=CIRCLE('',#92689,0.0999999999999994) ;
#29404=CIRCLE('',#92691,0.0999999999999994) ;
#29405=CIRCLE('',#92694,0.1) ;
#29406=CIRCLE('',#92695,0.1) ;
#29407=CIRCLE('',#92697,0.0999999999999994) ;
#29408=CIRCLE('',#92701,0.0999999999999994) ;
#29409=CIRCLE('',#92705,0.0999999999999998) ;
#29410=CIRCLE('',#92706,0.0999999999999994) ;
#29411=CIRCLE('',#92708,0.0999999999999994) ;
#29412=CIRCLE('',#92710,0.0999999999999998) ;
#29413=CIRCLE('',#92712,0.0999999999999998) ;
#29414=CIRCLE('',#92714,0.0999999999999994) ;
#29415=CIRCLE('',#92716,0.0999999999999998) ;
#29416=CIRCLE('',#92718,0.0999999999999994) ;
#29417=CIRCLE('',#92721,0.0999999999999998) ;
#29418=CIRCLE('',#92722,0.0999999999999998) ;
#29419=CIRCLE('',#92724,0.0999999999999994) ;
#29420=CIRCLE('',#92725,0.0999999999999994) ;
#29421=CIRCLE('',#92727,0.0999999999999994) ;
#29422=CIRCLE('',#92728,0.0999999999999994) ;
#29423=CIRCLE('',#92730,0.0999999999999994) ;
#29424=CIRCLE('',#92732,0.0999999999999994) ;
#29425=CIRCLE('',#92734,0.0999999999999998) ;
#29426=CIRCLE('',#92735,0.0999999999999998) ;
#29427=CIRCLE('',#92737,0.0999999999999994) ;
#29428=CIRCLE('',#92739,0.0999999999999994) ;
#29429=CIRCLE('',#92741,0.1) ;
#29430=CIRCLE('',#92742,0.1) ;
#29431=CIRCLE('',#92744,0.0999999999999994) ;
#29432=CIRCLE('',#92746,0.0999999999999994) ;
#29433=CIRCLE('',#92748,0.0999999999999994) ;
#29434=CIRCLE('',#92750,0.0999999999999994) ;
#29435=CIRCLE('',#92752,0.0999999999999994) ;
#29436=CIRCLE('',#92754,0.0999999999999994) ;
#29437=CIRCLE('',#92756,0.0999999999999994) ;
#29438=CIRCLE('',#92758,0.0999999999999994) ;
#29439=CIRCLE('',#92760,0.1) ;
#29440=CIRCLE('',#92762,0.1) ;
#29441=CIRCLE('',#92765,0.1) ;
#29442=CIRCLE('',#92766,0.0999999999999998) ;
#29443=CIRCLE('',#92768,0.0999999999999994) ;
#29444=CIRCLE('',#92769,0.0999999999999994) ;
#29445=CIRCLE('',#92771,0.0999999999999994) ;
#29446=CIRCLE('',#92772,0.0999999999999994) ;
#29447=CIRCLE('',#92774,0.0999999999999994) ;
#29448=CIRCLE('',#92776,0.0999999999999994) ;
#29449=CIRCLE('',#92778,0.0999999999999998) ;
#29450=CIRCLE('',#92779,0.0999999999999998) ;
#29451=CIRCLE('',#92781,0.0999999999999994) ;
#29452=CIRCLE('',#92783,0.0999999999999994) ;
#29453=CIRCLE('',#92785,0.0999999999999998) ;
#29454=CIRCLE('',#92786,0.0999999999999998) ;
#29455=CIRCLE('',#92788,0.0999999999999994) ;
#29456=CIRCLE('',#92790,0.0999999999999994) ;
#29457=CIRCLE('',#92792,0.0999999999999994) ;
#29458=CIRCLE('',#92794,0.0999999999999994) ;
#29459=CIRCLE('',#92796,0.0999999999999994) ;
#29460=CIRCLE('',#92798,0.0999999999999994) ;
#29461=CIRCLE('',#92800,0.0999999999999994) ;
#29462=CIRCLE('',#92802,0.0999999999999994) ;
#29463=CIRCLE('',#92804,0.0999999999999998) ;
#29464=CIRCLE('',#92806,0.0999999999999998) ;
#29465=CIRCLE('',#92809,0.0999999999999997) ;
#29466=CIRCLE('',#92811,0.1) ;
#29467=CIRCLE('',#92813,0.0999999999999994) ;
#29468=CIRCLE('',#92815,0.0999999999999994) ;
#29469=CIRCLE('',#92817,0.0999999999999994) ;
#29470=CIRCLE('',#92819,0.1) ;
#29471=CIRCLE('',#92821,0.099999999999999) ;
#29472=CIRCLE('',#92823,0.0999999999999994) ;
#29473=CIRCLE('',#92825,0.0999999999999994) ;
#29474=CIRCLE('',#92827,0.099999999999999) ;
#29475=CIRCLE('',#92834,0.0999999999999994) ;
#29476=CIRCLE('',#92836,0.0999999999999994) ;
#29477=CIRCLE('',#92838,0.0999999999999993) ;
#29478=CIRCLE('',#92839,0.1) ;
#29479=CIRCLE('',#92840,0.1) ;
#29480=CIRCLE('',#92842,0.0999999999999998) ;
#29481=CIRCLE('',#92844,0.0999999999999994) ;
#29482=CIRCLE('',#92848,0.1) ;
#29483=CIRCLE('',#92849,0.0999999999999995) ;
#29484=CIRCLE('',#92850,0.0999999999999998) ;
#29485=CIRCLE('',#92851,0.100000000000001) ;
#29486=CIRCLE('',#92853,0.0999999999999995) ;
#29487=CIRCLE('',#92854,0.0999999999999994) ;
#29488=CIRCLE('',#92856,0.0999999999999994) ;
#29489=CIRCLE('',#92857,0.0999999999999995) ;
#29490=CIRCLE('',#92859,0.0999999999999994) ;
#29491=CIRCLE('',#92861,0.1) ;
#29492=CIRCLE('',#92863,0.1) ;
#29493=CIRCLE('',#92865,0.0999999999999994) ;
#29494=CIRCLE('',#92867,0.1) ;
#29495=CIRCLE('',#92869,0.0999999999999999) ;
#29496=CIRCLE('',#92871,0.0999999999999999) ;
#29497=CIRCLE('',#92873,0.1) ;
#29498=CIRCLE('',#92875,0.1) ;
#29499=CIRCLE('',#92878,0.1) ;
#29500=CIRCLE('',#92879,0.1) ;
#29501=CIRCLE('',#92882,0.1) ;
#29502=CIRCLE('',#92884,0.0999999999999994) ;
#29503=CIRCLE('',#92885,0.0999999999999994) ;
#29504=CIRCLE('',#92886,0.0999999999999994) ;
#29505=CIRCLE('',#92888,0.0999999999999994) ;
#29506=CIRCLE('',#92890,0.0999999999999994) ;
#29507=CIRCLE('',#92892,0.0999999999999994) ;
#29508=CIRCLE('',#92894,0.0999999999999994) ;
#29509=CIRCLE('',#92896,0.0999999999999994) ;
#29510=CIRCLE('',#92898,0.1) ;
#29511=CIRCLE('',#92900,0.1) ;
#29512=CIRCLE('',#92903,0.200000000000001) ;
#29513=CIRCLE('',#92904,0.0999999999999994) ;
#29514=CIRCLE('',#92905,0.0999999999999994) ;
#29515=CIRCLE('',#92906,0.0999999999999993) ;
#29516=CIRCLE('',#92908,0.1) ;
#29517=CIRCLE('',#92909,0.1) ;
#29518=CIRCLE('',#92911,2.) ;
#29519=CIRCLE('',#92912,0.1) ;
#29520=CIRCLE('',#92913,1.9) ;
#29521=CIRCLE('',#92914,1.9) ;
#29522=CIRCLE('',#92916,1.47071067811865) ;
#29523=CIRCLE('',#92917,0.1) ;
#29524=CIRCLE('',#92918,1.5) ;
#29525=CIRCLE('',#92920,1.6) ;
#29526=CIRCLE('',#92921,0.1) ;
#29527=CIRCLE('',#92922,1.5) ;
#29528=CIRCLE('',#92923,1.5) ;
#29529=CIRCLE('',#92925,0.0999999999999994) ;
#29530=CIRCLE('',#92926,0.0999999999999994) ;
#29531=CIRCLE('',#92927,0.200000000000001) ;
#29532=CIRCLE('',#92928,0.0999999999999994) ;
#29533=CIRCLE('',#92930,0.0999999999999994) ;
#29534=CIRCLE('',#92931,0.0999999999999994) ;
#29535=CIRCLE('',#92932,0.0999999999999994) ;
#29536=CIRCLE('',#92934,0.0999999999999994) ;
#29537=CIRCLE('',#92936,0.0999999999999994) ;
#29538=CIRCLE('',#92937,0.0999999999999994) ;
#29539=CIRCLE('',#92938,0.0999999999999994) ;
#29540=CIRCLE('',#92940,0.749999999999997) ;
#29541=CIRCLE('',#92943,1.9) ;
#29542=CIRCLE('',#92944,1.9) ;
#29543=CIRCLE('',#92945,1.9) ;
#29544=CIRCLE('',#92946,1.9) ;
#29545=CIRCLE('',#92947,1.9) ;
#29546=CIRCLE('',#92949,3.1) ;
#29547=CIRCLE('',#92954,0.200000000000001) ;
#29548=CIRCLE('',#92955,2.9) ;
#29549=CIRCLE('',#92956,0.200000000000001) ;
#29550=CIRCLE('',#92957,0.200000000000001) ;
#29551=CIRCLE('',#92969,0.200000000000001) ;
#29552=CIRCLE('',#92970,0.200000000000001) ;
#29553=CIRCLE('',#92971,0.200000000000001) ;
#29554=CIRCLE('',#92972,0.200000000000001) ;
#29555=CIRCLE('',#92978,0.200000000000001) ;
#29556=CIRCLE('',#92979,0.200000000000001) ;
#29557=CIRCLE('',#92980,0.200000000000001) ;
#29558=CIRCLE('',#92981,0.200000000000001) ;
#29559=CIRCLE('',#92985,3.1) ;
#29560=CIRCLE('',#92988,0.1) ;
#29561=CIRCLE('',#92989,0.1) ;
#29562=CIRCLE('',#92990,0.0999999999999994) ;
#29563=CIRCLE('',#92991,0.0999999999999994) ;
#29564=CIRCLE('',#92992,0.1) ;
#29565=CIRCLE('',#92993,0.1) ;
#29566=CIRCLE('',#92994,0.0999999999999998) ;
#29567=CIRCLE('',#92995,0.0999999999999998) ;
#29568=CIRCLE('',#92996,0.0999999999999998) ;
#29569=CIRCLE('',#92997,0.0999999999999998) ;
#29570=CIRCLE('',#92998,0.0999999999999998) ;
#29571=CIRCLE('',#92999,0.0999999999999998) ;
#29572=CIRCLE('',#93000,0.1) ;
#29573=CIRCLE('',#93001,0.1) ;
#29574=CIRCLE('',#93002,0.1) ;
#29575=CIRCLE('',#93003,0.1) ;
#29576=CIRCLE('',#93004,0.0999999999999998) ;
#29577=CIRCLE('',#93005,0.0999999999999998) ;
#29578=CIRCLE('',#93007,0.1) ;
#29579=CIRCLE('',#93008,0.0999999999999998) ;
#29580=CIRCLE('',#93009,0.0999999999999998) ;
#29581=CIRCLE('',#93010,0.1) ;
#29582=CIRCLE('',#93011,0.1) ;
#29583=CIRCLE('',#93012,0.1) ;
#29584=CIRCLE('',#93013,0.1) ;
#29585=CIRCLE('',#93014,0.0999999999999998) ;
#29586=CIRCLE('',#93015,0.0999999999999998) ;
#29587=CIRCLE('',#93016,0.0999999999999998) ;
#29588=CIRCLE('',#93017,0.0999999999999998) ;
#29589=CIRCLE('',#93018,0.0999999999999998) ;
#29590=CIRCLE('',#93019,0.0999999999999998) ;
#29591=CIRCLE('',#93020,0.1) ;
#29592=CIRCLE('',#93021,0.1) ;
#29593=CIRCLE('',#93022,0.0999999999999994) ;
#29594=CIRCLE('',#93023,0.0999999999999994) ;
#29595=CIRCLE('',#93024,0.1) ;
#29596=CIRCLE('',#93047,0.0999999999999994) ;
#29597=CIRCLE('',#93048,0.0999999999999994) ;
#29598=CIRCLE('',#93049,0.0999999999999994) ;
#29599=CIRCLE('',#93050,0.0999999999999994) ;
#29600=CIRCLE('',#93052,0.0999999999999994) ;
#29601=CIRCLE('',#93055,0.0999999999999994) ;
#29602=CIRCLE('',#93058,0.0999999999999994) ;
#29603=CIRCLE('',#93061,0.0999999999999994) ;
#29604=CIRCLE('',#93073,0.0999999999999994) ;
#29605=CIRCLE('',#93074,0.0999999999999994) ;
#29606=CIRCLE('',#93075,0.0999999999999994) ;
#29607=CIRCLE('',#93076,0.0999999999999994) ;
#29608=CIRCLE('',#93078,0.0999999999999994) ;
#29609=CIRCLE('',#93081,0.0999999999999994) ;
#29610=CIRCLE('',#93084,0.0999999999999994) ;
#29611=CIRCLE('',#93087,0.0999999999999994) ;
#29612=CIRCLE('',#93094,0.200000000000001) ;
#29613=CIRCLE('',#93097,3.) ;
#29614=CIRCLE('',#93098,3.) ;
#29615=CIRCLE('',#93099,3.) ;
#29616=CIRCLE('',#93100,3.) ;
#29617=CIRCLE('',#93101,0.1) ;
#29618=CIRCLE('',#93102,0.0999999999999994) ;
#29619=CIRCLE('',#93104,0.0999999999999999) ;
#29620=CIRCLE('',#93105,0.1) ;
#29621=CIRCLE('',#93108,0.1) ;
#29622=CIRCLE('',#93110,0.0999999999999997) ;
#29623=CIRCLE('',#93112,0.0999999999999994) ;
#29624=CIRCLE('',#93114,0.1) ;
#29625=CIRCLE('',#93118,0.0999999999999999) ;
#29626=CIRCLE('',#93120,0.1) ;
#29627=CIRCLE('',#93122,0.1) ;
#29628=CIRCLE('',#93123,0.0999999999999994) ;
#29629=CIRCLE('',#93124,0.1) ;
#29630=CIRCLE('',#93126,0.1) ;
#29631=CIRCLE('',#93128,0.1) ;
#29632=CIRCLE('',#93130,0.1) ;
#29633=CIRCLE('',#93132,0.0999999999999994) ;
#29634=CIRCLE('',#93134,0.1) ;
#29635=CIRCLE('',#93136,0.0999999999999998) ;
#29636=CIRCLE('',#93138,0.1) ;
#29637=CIRCLE('',#93141,0.1) ;
#29638=CIRCLE('',#93143,0.0999999999999999) ;
#29639=CIRCLE('',#93145,0.0999999999999999) ;
#29640=CIRCLE('',#93147,0.1) ;
#29641=CIRCLE('',#93149,0.1) ;
#29642=CIRCLE('',#93152,0.1) ;
#29643=CIRCLE('',#93156,0.0999999999999999) ;
#29644=CIRCLE('',#93157,0.0999999999999999) ;
#29645=CIRCLE('',#93163,0.0999999999999994) ;
#29646=CIRCLE('',#93164,0.0999999999999994) ;
#29647=CIRCLE('',#93166,0.0999999999999994) ;
#29648=CIRCLE('',#93169,0.1) ;
#29649=CIRCLE('',#93170,0.1) ;
#29650=CIRCLE('',#93172,0.0999999999999994) ;
#29651=CIRCLE('',#93176,0.0999999999999994) ;
#29652=CIRCLE('',#93180,0.0999999999999998) ;
#29653=CIRCLE('',#93181,0.0999999999999994) ;
#29654=CIRCLE('',#93183,0.0999999999999994) ;
#29655=CIRCLE('',#93185,0.0999999999999998) ;
#29656=CIRCLE('',#93187,0.0999999999999998) ;
#29657=CIRCLE('',#93189,0.0999999999999994) ;
#29658=CIRCLE('',#93191,0.0999999999999998) ;
#29659=CIRCLE('',#93193,0.0999999999999994) ;
#29660=CIRCLE('',#93196,0.0999999999999998) ;
#29661=CIRCLE('',#93197,0.0999999999999998) ;
#29662=CIRCLE('',#93199,0.0999999999999994) ;
#29663=CIRCLE('',#93200,0.0999999999999994) ;
#29664=CIRCLE('',#93202,0.0999999999999994) ;
#29665=CIRCLE('',#93203,0.0999999999999994) ;
#29666=CIRCLE('',#93205,0.0999999999999994) ;
#29667=CIRCLE('',#93207,0.0999999999999994) ;
#29668=CIRCLE('',#93209,0.0999999999999998) ;
#29669=CIRCLE('',#93210,0.0999999999999998) ;
#29670=CIRCLE('',#93212,0.0999999999999994) ;
#29671=CIRCLE('',#93214,0.0999999999999994) ;
#29672=CIRCLE('',#93216,0.1) ;
#29673=CIRCLE('',#93217,0.1) ;
#29674=CIRCLE('',#93219,0.0999999999999994) ;
#29675=CIRCLE('',#93221,0.0999999999999994) ;
#29676=CIRCLE('',#93223,0.0999999999999994) ;
#29677=CIRCLE('',#93225,0.0999999999999994) ;
#29678=CIRCLE('',#93227,0.0999999999999994) ;
#29679=CIRCLE('',#93229,0.0999999999999994) ;
#29680=CIRCLE('',#93231,0.0999999999999994) ;
#29681=CIRCLE('',#93233,0.0999999999999994) ;
#29682=CIRCLE('',#93235,0.1) ;
#29683=CIRCLE('',#93237,0.1) ;
#29684=CIRCLE('',#93240,0.1) ;
#29685=CIRCLE('',#93241,0.0999999999999998) ;
#29686=CIRCLE('',#93243,0.0999999999999994) ;
#29687=CIRCLE('',#93244,0.0999999999999994) ;
#29688=CIRCLE('',#93246,0.0999999999999994) ;
#29689=CIRCLE('',#93247,0.0999999999999994) ;
#29690=CIRCLE('',#93249,0.0999999999999994) ;
#29691=CIRCLE('',#93251,0.0999999999999994) ;
#29692=CIRCLE('',#93253,0.0999999999999998) ;
#29693=CIRCLE('',#93254,0.0999999999999998) ;
#29694=CIRCLE('',#93256,0.0999999999999994) ;
#29695=CIRCLE('',#93258,0.0999999999999994) ;
#29696=CIRCLE('',#93260,0.0999999999999998) ;
#29697=CIRCLE('',#93261,0.0999999999999998) ;
#29698=CIRCLE('',#93263,0.0999999999999994) ;
#29699=CIRCLE('',#93265,0.0999999999999994) ;
#29700=CIRCLE('',#93267,0.0999999999999994) ;
#29701=CIRCLE('',#93269,0.0999999999999994) ;
#29702=CIRCLE('',#93271,0.0999999999999994) ;
#29703=CIRCLE('',#93273,0.0999999999999994) ;
#29704=CIRCLE('',#93275,0.0999999999999994) ;
#29705=CIRCLE('',#93277,0.0999999999999994) ;
#29706=CIRCLE('',#93279,0.0999999999999998) ;
#29707=CIRCLE('',#93281,0.0999999999999998) ;
#29708=CIRCLE('',#93284,0.0999999999999997) ;
#29709=CIRCLE('',#93286,0.1) ;
#29710=CIRCLE('',#93288,0.0999999999999994) ;
#29711=CIRCLE('',#93290,0.0999999999999994) ;
#29712=CIRCLE('',#93292,0.0999999999999994) ;
#29713=CIRCLE('',#93294,0.1) ;
#29714=CIRCLE('',#93296,0.1) ;
#29715=CIRCLE('',#93298,0.0999999999999994) ;
#29716=CIRCLE('',#93300,0.0999999999999994) ;
#29717=CIRCLE('',#93302,0.0999999999999994) ;
#29718=CIRCLE('',#93304,0.0999999999999998) ;
#29719=CIRCLE('',#93306,0.1) ;
#29720=CIRCLE('',#93326,0.0999999999999994) ;
#29721=CIRCLE('',#93328,0.0999999999999994) ;
#29722=CIRCLE('',#93330,0.0999999999999993) ;
#29723=CIRCLE('',#93331,0.1) ;
#29724=CIRCLE('',#93332,0.1) ;
#29725=CIRCLE('',#93335,0.1) ;
#29726=CIRCLE('',#93336,0.0999999999999998) ;
#29727=CIRCLE('',#93338,0.0999999999999994) ;
#29728=CIRCLE('',#93342,0.1) ;
#29729=CIRCLE('',#93344,0.1) ;
#29730=CIRCLE('',#93345,0.0999999999999995) ;
#29731=CIRCLE('',#93346,0.0999999999999998) ;
#29732=CIRCLE('',#93347,0.0999999999999993) ;
#34714=VERTEX_POINT('',#132553) ;
#34715=VERTEX_POINT('',#132554) ;
#34716=VERTEX_POINT('',#132556) ;
#34717=VERTEX_POINT('',#132558) ;
#34718=VERTEX_POINT('',#132562) ;
#34719=VERTEX_POINT('',#132564) ;
#34720=VERTEX_POINT('',#132566) ;
#34721=VERTEX_POINT('',#132570) ;
#34722=VERTEX_POINT('',#132572) ;
#34723=VERTEX_POINT('',#132576) ;
#34724=VERTEX_POINT('',#132578) ;
#34725=VERTEX_POINT('',#132580) ;
#34726=VERTEX_POINT('',#132584) ;
#34727=VERTEX_POINT('',#132585) ;
#34728=VERTEX_POINT('',#132587) ;
#34729=VERTEX_POINT('',#132589) ;
#34730=VERTEX_POINT('',#132593) ;
#34731=VERTEX_POINT('',#132594) ;
#34732=VERTEX_POINT('',#132596) ;
#34733=VERTEX_POINT('',#132600) ;
#34734=VERTEX_POINT('',#132602) ;
#34735=VERTEX_POINT('',#132606) ;
#34736=VERTEX_POINT('',#132607) ;
#34737=VERTEX_POINT('',#132609) ;
#34738=VERTEX_POINT('',#132613) ;
#34739=VERTEX_POINT('',#132619) ;
#34740=VERTEX_POINT('',#132620) ;
#34741=VERTEX_POINT('',#132622) ;
#34742=VERTEX_POINT('',#132633) ;
#34743=VERTEX_POINT('',#132635) ;
#34744=VERTEX_POINT('',#132646) ;
#34745=VERTEX_POINT('',#132648) ;
#34746=VERTEX_POINT('',#132659) ;
#34747=VERTEX_POINT('',#132661) ;
#34748=VERTEX_POINT('',#132693) ;
#34749=VERTEX_POINT('',#132695) ;
#34750=VERTEX_POINT('',#132706) ;
#34751=VERTEX_POINT('',#132708) ;
#34752=VERTEX_POINT('',#132719) ;
#34753=VERTEX_POINT('',#132721) ;
#34754=VERTEX_POINT('',#132732) ;
#34755=VERTEX_POINT('',#132734) ;
#34756=VERTEX_POINT('',#132769) ;
#34757=VERTEX_POINT('',#132770) ;
#34758=VERTEX_POINT('',#132772) ;
#34759=VERTEX_POINT('',#132774) ;
#34760=VERTEX_POINT('',#132778) ;
#34761=VERTEX_POINT('',#132779) ;
#34762=VERTEX_POINT('',#132781) ;
#34763=VERTEX_POINT('',#132783) ;
#34764=VERTEX_POINT('',#132787) ;
#34765=VERTEX_POINT('',#132789) ;
#34766=VERTEX_POINT('',#132791) ;
#34767=VERTEX_POINT('',#132795) ;
#34768=VERTEX_POINT('',#132797) ;
#34769=VERTEX_POINT('',#132801) ;
#34770=VERTEX_POINT('',#132803) ;
#34771=VERTEX_POINT('',#132805) ;
#34772=VERTEX_POINT('',#132809) ;
#34773=VERTEX_POINT('',#132810) ;
#34774=VERTEX_POINT('',#132812) ;
#34775=VERTEX_POINT('',#132814) ;
#34776=VERTEX_POINT('',#132818) ;
#34777=VERTEX_POINT('',#132819) ;
#34778=VERTEX_POINT('',#132821) ;
#34779=VERTEX_POINT('',#132825) ;
#34780=VERTEX_POINT('',#132827) ;
#34781=VERTEX_POINT('',#132831) ;
#34782=VERTEX_POINT('',#132832) ;
#34783=VERTEX_POINT('',#132834) ;
#34784=VERTEX_POINT('',#132838) ;
#34785=VERTEX_POINT('',#132844) ;
#34786=VERTEX_POINT('',#132845) ;
#34787=VERTEX_POINT('',#132847) ;
#34788=VERTEX_POINT('',#132858) ;
#34789=VERTEX_POINT('',#132860) ;
#34790=VERTEX_POINT('',#132871) ;
#34791=VERTEX_POINT('',#132873) ;
#34792=VERTEX_POINT('',#132884) ;
#34793=VERTEX_POINT('',#132886) ;
#34794=VERTEX_POINT('',#132918) ;
#34795=VERTEX_POINT('',#132920) ;
#34796=VERTEX_POINT('',#132931) ;
#34797=VERTEX_POINT('',#132933) ;
#34798=VERTEX_POINT('',#132944) ;
#34799=VERTEX_POINT('',#132946) ;
#34800=VERTEX_POINT('',#132957) ;
#34801=VERTEX_POINT('',#132959) ;
#34802=VERTEX_POINT('',#132994) ;
#34803=VERTEX_POINT('',#132995) ;
#34804=VERTEX_POINT('',#132997) ;
#34805=VERTEX_POINT('',#132999) ;
#34806=VERTEX_POINT('',#133002) ;
#34807=VERTEX_POINT('',#133003) ;
#34808=VERTEX_POINT('',#133005) ;
#34809=VERTEX_POINT('',#133007) ;
#34810=VERTEX_POINT('',#133012) ;
#34811=VERTEX_POINT('',#133014) ;
#34812=VERTEX_POINT('',#133019) ;
#34813=VERTEX_POINT('',#133021) ;
#34814=VERTEX_POINT('',#133025) ;
#34815=VERTEX_POINT('',#133026) ;
#34816=VERTEX_POINT('',#133028) ;
#34817=VERTEX_POINT('',#133030) ;
#34818=VERTEX_POINT('',#133034) ;
#34819=VERTEX_POINT('',#133035) ;
#34820=VERTEX_POINT('',#133037) ;
#34821=VERTEX_POINT('',#133039) ;
#34822=VERTEX_POINT('',#133043) ;
#34823=VERTEX_POINT('',#133044) ;
#34824=VERTEX_POINT('',#133046) ;
#34825=VERTEX_POINT('',#133048) ;
#34826=VERTEX_POINT('',#133052) ;
#34827=VERTEX_POINT('',#133053) ;
#34828=VERTEX_POINT('',#133064) ;
#34829=VERTEX_POINT('',#133066) ;
#34830=VERTEX_POINT('',#133068) ;
#34831=VERTEX_POINT('',#133070) ;
#34832=VERTEX_POINT('',#133074) ;
#34833=VERTEX_POINT('',#133075) ;
#34834=VERTEX_POINT('',#133077) ;
#34835=VERTEX_POINT('',#133079) ;
#34836=VERTEX_POINT('',#133083) ;
#34837=VERTEX_POINT('',#133084) ;
#34838=VERTEX_POINT('',#133086) ;
#34839=VERTEX_POINT('',#133088) ;
#34840=VERTEX_POINT('',#133093) ;
#34841=VERTEX_POINT('',#133095) ;
#34842=VERTEX_POINT('',#133102) ;
#34843=VERTEX_POINT('',#133104) ;
#34844=VERTEX_POINT('',#133106) ;
#34845=VERTEX_POINT('',#133108) ;
#34846=VERTEX_POINT('',#133110) ;
#34847=VERTEX_POINT('',#133112) ;
#34848=VERTEX_POINT('',#133114) ;
#34849=VERTEX_POINT('',#133116) ;
#34850=VERTEX_POINT('',#133118) ;
#34851=VERTEX_POINT('',#133120) ;
#34852=VERTEX_POINT('',#133122) ;
#34853=VERTEX_POINT('',#133124) ;
#34854=VERTEX_POINT('',#133127) ;
#34855=VERTEX_POINT('',#133129) ;
#34856=VERTEX_POINT('',#133134) ;
#34857=VERTEX_POINT('',#133136) ;
#34858=VERTEX_POINT('',#133140) ;
#34859=VERTEX_POINT('',#133142) ;
#34860=VERTEX_POINT('',#133144) ;
#34861=VERTEX_POINT('',#133148) ;
#34862=VERTEX_POINT('',#133149) ;
#34863=VERTEX_POINT('',#133151) ;
#34864=VERTEX_POINT('',#133153) ;
#34865=VERTEX_POINT('',#133155) ;
#34866=VERTEX_POINT('',#133157) ;
#34867=VERTEX_POINT('',#133159) ;
#34868=VERTEX_POINT('',#133161) ;
#34869=VERTEX_POINT('',#133163) ;
#34870=VERTEX_POINT('',#133165) ;
#34871=VERTEX_POINT('',#133167) ;
#34872=VERTEX_POINT('',#133169) ;
#34873=VERTEX_POINT('',#133173) ;
#34874=VERTEX_POINT('',#133174) ;
#34875=VERTEX_POINT('',#133179) ;
#34876=VERTEX_POINT('',#133181) ;
#34877=VERTEX_POINT('',#133186) ;
#34878=VERTEX_POINT('',#133187) ;
#34879=VERTEX_POINT('',#133189) ;
#34880=VERTEX_POINT('',#133191) ;
#34881=VERTEX_POINT('',#133194) ;
#34882=VERTEX_POINT('',#133195) ;
#34883=VERTEX_POINT('',#133197) ;
#34884=VERTEX_POINT('',#133199) ;
#34885=VERTEX_POINT('',#133201) ;
#34886=VERTEX_POINT('',#133203) ;
#34887=VERTEX_POINT('',#133205) ;
#34888=VERTEX_POINT('',#133207) ;
#34889=VERTEX_POINT('',#133210) ;
#34890=VERTEX_POINT('',#133211) ;
#34891=VERTEX_POINT('',#133213) ;
#34892=VERTEX_POINT('',#133215) ;
#34893=VERTEX_POINT('',#133217) ;
#34894=VERTEX_POINT('',#133219) ;
#34895=VERTEX_POINT('',#133221) ;
#34896=VERTEX_POINT('',#133223) ;
#34897=VERTEX_POINT('',#133227) ;
#34898=VERTEX_POINT('',#133228) ;
#34899=VERTEX_POINT('',#133230) ;
#34900=VERTEX_POINT('',#133232) ;
#34901=VERTEX_POINT('',#133236) ;
#34902=VERTEX_POINT('',#133237) ;
#34903=VERTEX_POINT('',#133242) ;
#34904=VERTEX_POINT('',#133244) ;
#34905=VERTEX_POINT('',#133248) ;
#34906=VERTEX_POINT('',#133249) ;
#34907=VERTEX_POINT('',#133251) ;
#34908=VERTEX_POINT('',#133253) ;
#34909=VERTEX_POINT('',#133256) ;
#34910=VERTEX_POINT('',#133257) ;
#34911=VERTEX_POINT('',#133259) ;
#34912=VERTEX_POINT('',#133266) ;
#34913=VERTEX_POINT('',#133268) ;
#34914=VERTEX_POINT('',#133275) ;
#34915=VERTEX_POINT('',#133277) ;
#34916=VERTEX_POINT('',#133284) ;
#34917=VERTEX_POINT('',#133292) ;
#34918=VERTEX_POINT('',#133293) ;
#34919=VERTEX_POINT('',#133295) ;
#34920=VERTEX_POINT('',#133302) ;
#34921=VERTEX_POINT('',#133304) ;
#34922=VERTEX_POINT('',#133311) ;
#34923=VERTEX_POINT('',#133313) ;
#34924=VERTEX_POINT('',#133320) ;
#34925=VERTEX_POINT('',#133329) ;
#34926=VERTEX_POINT('',#133330) ;
#34927=VERTEX_POINT('',#133332) ;
#34928=VERTEX_POINT('',#133334) ;
#34929=VERTEX_POINT('',#133337) ;
#34930=VERTEX_POINT('',#133338) ;
#34931=VERTEX_POINT('',#133340) ;
#34932=VERTEX_POINT('',#133342) ;
#34933=VERTEX_POINT('',#133344) ;
#34934=VERTEX_POINT('',#133346) ;
#34935=VERTEX_POINT('',#133348) ;
#34936=VERTEX_POINT('',#133350) ;
#34937=VERTEX_POINT('',#133353) ;
#34938=VERTEX_POINT('',#133354) ;
#34939=VERTEX_POINT('',#133356) ;
#34940=VERTEX_POINT('',#133358) ;
#34941=VERTEX_POINT('',#133360) ;
#34942=VERTEX_POINT('',#133362) ;
#34943=VERTEX_POINT('',#133364) ;
#34944=VERTEX_POINT('',#133366) ;
#34945=VERTEX_POINT('',#133370) ;
#34946=VERTEX_POINT('',#133371) ;
#34947=VERTEX_POINT('',#133373) ;
#34948=VERTEX_POINT('',#133375) ;
#34949=VERTEX_POINT('',#133379) ;
#34950=VERTEX_POINT('',#133380) ;
#34951=VERTEX_POINT('',#133409) ;
#34952=VERTEX_POINT('',#133420) ;
#34953=VERTEX_POINT('',#133446) ;
#34954=VERTEX_POINT('',#133463) ;
#34955=VERTEX_POINT('',#133465) ;
#34956=VERTEX_POINT('',#133467) ;
#34957=VERTEX_POINT('',#133469) ;
#34958=VERTEX_POINT('',#133471) ;
#34959=VERTEX_POINT('',#133473) ;
#34960=VERTEX_POINT('',#133502) ;
#34961=VERTEX_POINT('',#133513) ;
#34962=VERTEX_POINT('',#133539) ;
#34963=VERTEX_POINT('',#133558) ;
#34964=VERTEX_POINT('',#133559) ;
#34965=VERTEX_POINT('',#133561) ;
#34966=VERTEX_POINT('',#133563) ;
#34967=VERTEX_POINT('',#133567) ;
#34968=VERTEX_POINT('',#133568) ;
#34969=VERTEX_POINT('',#133570) ;
#34970=VERTEX_POINT('',#133572) ;
#34971=VERTEX_POINT('',#133591) ;
#34972=VERTEX_POINT('',#133592) ;
#34973=VERTEX_POINT('',#133594) ;
#34974=VERTEX_POINT('',#133596) ;
#34975=VERTEX_POINT('',#133600) ;
#34976=VERTEX_POINT('',#133601) ;
#34977=VERTEX_POINT('',#133603) ;
#34978=VERTEX_POINT('',#133605) ;
#34979=VERTEX_POINT('',#133609) ;
#34980=VERTEX_POINT('',#133610) ;
#34981=VERTEX_POINT('',#133612) ;
#34982=VERTEX_POINT('',#133614) ;
#34983=VERTEX_POINT('',#133616) ;
#34984=VERTEX_POINT('',#133618) ;
#34985=VERTEX_POINT('',#133620) ;
#34986=VERTEX_POINT('',#133622) ;
#34987=VERTEX_POINT('',#133626) ;
#34988=VERTEX_POINT('',#133627) ;
#34989=VERTEX_POINT('',#133629) ;
#34990=VERTEX_POINT('',#133631) ;
#34991=VERTEX_POINT('',#133634) ;
#34992=VERTEX_POINT('',#133636) ;
#34993=VERTEX_POINT('',#133640) ;
#34994=VERTEX_POINT('',#133641) ;
#34995=VERTEX_POINT('',#133644) ;
#34996=VERTEX_POINT('',#133646) ;
#34997=VERTEX_POINT('',#133648) ;
#34998=VERTEX_POINT('',#133650) ;
#34999=VERTEX_POINT('',#133654) ;
#35000=VERTEX_POINT('',#133656) ;
#35001=VERTEX_POINT('',#133660) ;
#35002=VERTEX_POINT('',#133662) ;
#35003=VERTEX_POINT('',#133666) ;
#35004=VERTEX_POINT('',#133667) ;
#35005=VERTEX_POINT('',#133669) ;
#35006=VERTEX_POINT('',#133671) ;
#35007=VERTEX_POINT('',#133673) ;
#35008=VERTEX_POINT('',#133675) ;
#35009=VERTEX_POINT('',#133679) ;
#35010=VERTEX_POINT('',#133680) ;
#35011=VERTEX_POINT('',#133682) ;
#35012=VERTEX_POINT('',#133684) ;
#35013=VERTEX_POINT('',#133686) ;
#35014=VERTEX_POINT('',#133688) ;
#35015=VERTEX_POINT('',#133692) ;
#35016=VERTEX_POINT('',#133693) ;
#35017=VERTEX_POINT('',#133695) ;
#35018=VERTEX_POINT('',#133697) ;
#35019=VERTEX_POINT('',#133701) ;
#35020=VERTEX_POINT('',#133702) ;
#35021=VERTEX_POINT('',#133704) ;
#35022=VERTEX_POINT('',#133706) ;
#35023=VERTEX_POINT('',#133710) ;
#35024=VERTEX_POINT('',#133711) ;
#35025=VERTEX_POINT('',#133713) ;
#35026=VERTEX_POINT('',#133715) ;
#35027=VERTEX_POINT('',#133719) ;
#35028=VERTEX_POINT('',#133720) ;
#35029=VERTEX_POINT('',#133722) ;
#35030=VERTEX_POINT('',#133724) ;
#35031=VERTEX_POINT('',#133728) ;
#35032=VERTEX_POINT('',#133729) ;
#35033=VERTEX_POINT('',#133731) ;
#35034=VERTEX_POINT('',#133733) ;
#35035=VERTEX_POINT('',#133736) ;
#35036=VERTEX_POINT('',#133737) ;
#35037=VERTEX_POINT('',#133739) ;
#35038=VERTEX_POINT('',#133741) ;
#35039=VERTEX_POINT('',#133743) ;
#35040=VERTEX_POINT('',#133745) ;
#35041=VERTEX_POINT('',#133747) ;
#35042=VERTEX_POINT('',#133749) ;
#35043=VERTEX_POINT('',#133753) ;
#35044=VERTEX_POINT('',#133754) ;
#35045=VERTEX_POINT('',#133759) ;
#35046=VERTEX_POINT('',#133763) ;
#35047=VERTEX_POINT('',#133767) ;
#35048=VERTEX_POINT('',#133771) ;
#35049=VERTEX_POINT('',#133775) ;
#35050=VERTEX_POINT('',#133779) ;
#35051=VERTEX_POINT('',#133797) ;
#35052=VERTEX_POINT('',#133798) ;
#35053=VERTEX_POINT('',#133800) ;
#35054=VERTEX_POINT('',#133802) ;
#35055=VERTEX_POINT('',#133806) ;
#35056=VERTEX_POINT('',#133807) ;
#35057=VERTEX_POINT('',#133809) ;
#35058=VERTEX_POINT('',#133811) ;
#35059=VERTEX_POINT('',#133815) ;
#35060=VERTEX_POINT('',#133816) ;
#35061=VERTEX_POINT('',#133818) ;
#35062=VERTEX_POINT('',#133820) ;
#35063=VERTEX_POINT('',#133824) ;
#35064=VERTEX_POINT('',#133825) ;
#35065=VERTEX_POINT('',#133827) ;
#35066=VERTEX_POINT('',#133829) ;
#35067=VERTEX_POINT('',#133833) ;
#35068=VERTEX_POINT('',#133834) ;
#35069=VERTEX_POINT('',#133836) ;
#35070=VERTEX_POINT('',#133838) ;
#35071=VERTEX_POINT('',#133841) ;
#35072=VERTEX_POINT('',#133842) ;
#35073=VERTEX_POINT('',#133844) ;
#35074=VERTEX_POINT('',#133846) ;
#35075=VERTEX_POINT('',#133848) ;
#35076=VERTEX_POINT('',#133850) ;
#35077=VERTEX_POINT('',#133852) ;
#35078=VERTEX_POINT('',#133854) ;
#35079=VERTEX_POINT('',#133858) ;
#35080=VERTEX_POINT('',#133860) ;
#35081=VERTEX_POINT('',#133864) ;
#35082=VERTEX_POINT('',#133868) ;
#35083=VERTEX_POINT('',#133872) ;
#35084=VERTEX_POINT('',#133876) ;
#35085=VERTEX_POINT('',#133880) ;
#35086=VERTEX_POINT('',#133884) ;
#35087=VERTEX_POINT('',#133890) ;
#35088=VERTEX_POINT('',#133891) ;
#35089=VERTEX_POINT('',#133893) ;
#35090=VERTEX_POINT('',#133895) ;
#35091=VERTEX_POINT('',#133900) ;
#35092=VERTEX_POINT('',#133902) ;
#35093=VERTEX_POINT('',#133906) ;
#35094=VERTEX_POINT('',#133908) ;
#35095=VERTEX_POINT('',#133912) ;
#35096=VERTEX_POINT('',#133917) ;
#35097=VERTEX_POINT('',#133919) ;
#35098=VERTEX_POINT('',#133921) ;
#35099=VERTEX_POINT('',#133923) ;
#35100=VERTEX_POINT('',#133928) ;
#35101=VERTEX_POINT('',#133929) ;
#35102=VERTEX_POINT('',#133931) ;
#35103=VERTEX_POINT('',#133933) ;
#35104=VERTEX_POINT('',#133935) ;
#35105=VERTEX_POINT('',#133937) ;
#35106=VERTEX_POINT('',#134132) ;
#35107=VERTEX_POINT('',#134194) ;
#35108=VERTEX_POINT('',#134195) ;
#35109=VERTEX_POINT('',#134461) ;
#35110=VERTEX_POINT('',#134462) ;
#35111=VERTEX_POINT('',#134503) ;
#35112=VERTEX_POINT('',#134838) ;
#35113=VERTEX_POINT('',#134839) ;
#35114=VERTEX_POINT('',#134841) ;
#35115=VERTEX_POINT('',#134843) ;
#35116=VERTEX_POINT('',#134847) ;
#35117=VERTEX_POINT('',#134849) ;
#35118=VERTEX_POINT('',#134853) ;
#35119=VERTEX_POINT('',#134855) ;
#35120=VERTEX_POINT('',#134859) ;
#35121=VERTEX_POINT('',#134861) ;
#35122=VERTEX_POINT('',#134865) ;
#35123=VERTEX_POINT('',#134867) ;
#35124=VERTEX_POINT('',#134871) ;
#35125=VERTEX_POINT('',#134873) ;
#35126=VERTEX_POINT('',#134877) ;
#35127=VERTEX_POINT('',#134879) ;
#35128=VERTEX_POINT('',#134883) ;
#35129=VERTEX_POINT('',#134885) ;
#35130=VERTEX_POINT('',#134889) ;
#35131=VERTEX_POINT('',#134891) ;
#35132=VERTEX_POINT('',#134895) ;
#35133=VERTEX_POINT('',#134896) ;
#35134=VERTEX_POINT('',#134898) ;
#35135=VERTEX_POINT('',#134900) ;
#35136=VERTEX_POINT('',#134902) ;
#35137=VERTEX_POINT('',#134904) ;
#35138=VERTEX_POINT('',#134906) ;
#35139=VERTEX_POINT('',#134910) ;
#35140=VERTEX_POINT('',#134911) ;
#35141=VERTEX_POINT('',#134913) ;
#35142=VERTEX_POINT('',#134915) ;
#35143=VERTEX_POINT('',#134917) ;
#35144=VERTEX_POINT('',#134919) ;
#35145=VERTEX_POINT('',#134921) ;
#35146=VERTEX_POINT('',#134925) ;
#35147=VERTEX_POINT('',#134926) ;
#35148=VERTEX_POINT('',#134928) ;
#35149=VERTEX_POINT('',#134930) ;
#35150=VERTEX_POINT('',#134934) ;
#35151=VERTEX_POINT('',#134935) ;
#35152=VERTEX_POINT('',#134937) ;
#35153=VERTEX_POINT('',#134944) ;
#35154=VERTEX_POINT('',#134945) ;
#35155=VERTEX_POINT('',#134947) ;
#35156=VERTEX_POINT('',#134949) ;
#35157=VERTEX_POINT('',#134959) ;
#35158=VERTEX_POINT('',#134960) ;
#35159=VERTEX_POINT('',#134962) ;
#35160=VERTEX_POINT('',#134964) ;
#35161=VERTEX_POINT('',#134968) ;
#35162=VERTEX_POINT('',#134969) ;
#35163=VERTEX_POINT('',#134971) ;
#35164=VERTEX_POINT('',#134973) ;
#35165=VERTEX_POINT('',#134977) ;
#35166=VERTEX_POINT('',#134978) ;
#35167=VERTEX_POINT('',#134980) ;
#35168=VERTEX_POINT('',#134982) ;
#35169=VERTEX_POINT('',#134984) ;
#35170=VERTEX_POINT('',#134986) ;
#35171=VERTEX_POINT('',#134988) ;
#35172=VERTEX_POINT('',#134990) ;
#35173=VERTEX_POINT('',#134994) ;
#35174=VERTEX_POINT('',#134995) ;
#35175=VERTEX_POINT('',#134997) ;
#35176=VERTEX_POINT('',#134999) ;
#35177=VERTEX_POINT('',#135002) ;
#35178=VERTEX_POINT('',#135004) ;
#35179=VERTEX_POINT('',#135008) ;
#35180=VERTEX_POINT('',#135009) ;
#35181=VERTEX_POINT('',#135012) ;
#35182=VERTEX_POINT('',#135014) ;
#35183=VERTEX_POINT('',#135016) ;
#35184=VERTEX_POINT('',#135018) ;
#35185=VERTEX_POINT('',#135022) ;
#35186=VERTEX_POINT('',#135024) ;
#35187=VERTEX_POINT('',#135028) ;
#35188=VERTEX_POINT('',#135030) ;
#35189=VERTEX_POINT('',#135034) ;
#35190=VERTEX_POINT('',#135035) ;
#35191=VERTEX_POINT('',#135037) ;
#35192=VERTEX_POINT('',#135039) ;
#35193=VERTEX_POINT('',#135041) ;
#35194=VERTEX_POINT('',#135043) ;
#35195=VERTEX_POINT('',#135047) ;
#35196=VERTEX_POINT('',#135048) ;
#35197=VERTEX_POINT('',#135050) ;
#35198=VERTEX_POINT('',#135052) ;
#35199=VERTEX_POINT('',#135054) ;
#35200=VERTEX_POINT('',#135056) ;
#35201=VERTEX_POINT('',#135060) ;
#35202=VERTEX_POINT('',#135061) ;
#35203=VERTEX_POINT('',#135063) ;
#35204=VERTEX_POINT('',#135065) ;
#35205=VERTEX_POINT('',#135069) ;
#35206=VERTEX_POINT('',#135070) ;
#35207=VERTEX_POINT('',#135072) ;
#35208=VERTEX_POINT('',#135074) ;
#35209=VERTEX_POINT('',#135078) ;
#35210=VERTEX_POINT('',#135079) ;
#35211=VERTEX_POINT('',#135081) ;
#35212=VERTEX_POINT('',#135083) ;
#35213=VERTEX_POINT('',#135087) ;
#35214=VERTEX_POINT('',#135088) ;
#35215=VERTEX_POINT('',#135090) ;
#35216=VERTEX_POINT('',#135092) ;
#35217=VERTEX_POINT('',#135096) ;
#35218=VERTEX_POINT('',#135097) ;
#35219=VERTEX_POINT('',#135099) ;
#35220=VERTEX_POINT('',#135101) ;
#35221=VERTEX_POINT('',#135104) ;
#35222=VERTEX_POINT('',#135105) ;
#35223=VERTEX_POINT('',#135107) ;
#35224=VERTEX_POINT('',#135109) ;
#35225=VERTEX_POINT('',#135111) ;
#35226=VERTEX_POINT('',#135113) ;
#35227=VERTEX_POINT('',#135115) ;
#35228=VERTEX_POINT('',#135117) ;
#35229=VERTEX_POINT('',#135121) ;
#35230=VERTEX_POINT('',#135122) ;
#35231=VERTEX_POINT('',#135127) ;
#35232=VERTEX_POINT('',#135131) ;
#35233=VERTEX_POINT('',#135135) ;
#35234=VERTEX_POINT('',#135139) ;
#35235=VERTEX_POINT('',#135143) ;
#35236=VERTEX_POINT('',#135147) ;
#35237=VERTEX_POINT('',#135165) ;
#35238=VERTEX_POINT('',#135166) ;
#35239=VERTEX_POINT('',#135168) ;
#35240=VERTEX_POINT('',#135170) ;
#35241=VERTEX_POINT('',#135174) ;
#35242=VERTEX_POINT('',#135175) ;
#35243=VERTEX_POINT('',#135177) ;
#35244=VERTEX_POINT('',#135179) ;
#35245=VERTEX_POINT('',#135183) ;
#35246=VERTEX_POINT('',#135184) ;
#35247=VERTEX_POINT('',#135186) ;
#35248=VERTEX_POINT('',#135188) ;
#35249=VERTEX_POINT('',#135192) ;
#35250=VERTEX_POINT('',#135193) ;
#35251=VERTEX_POINT('',#135195) ;
#35252=VERTEX_POINT('',#135197) ;
#35253=VERTEX_POINT('',#135201) ;
#35254=VERTEX_POINT('',#135202) ;
#35255=VERTEX_POINT('',#135204) ;
#35256=VERTEX_POINT('',#135206) ;
#35257=VERTEX_POINT('',#135209) ;
#35258=VERTEX_POINT('',#135210) ;
#35259=VERTEX_POINT('',#135212) ;
#35260=VERTEX_POINT('',#135214) ;
#35261=VERTEX_POINT('',#135216) ;
#35262=VERTEX_POINT('',#135218) ;
#35263=VERTEX_POINT('',#135220) ;
#35264=VERTEX_POINT('',#135222) ;
#35265=VERTEX_POINT('',#135226) ;
#35266=VERTEX_POINT('',#135228) ;
#35267=VERTEX_POINT('',#135232) ;
#35268=VERTEX_POINT('',#135236) ;
#35269=VERTEX_POINT('',#135240) ;
#35270=VERTEX_POINT('',#135244) ;
#35271=VERTEX_POINT('',#135248) ;
#35272=VERTEX_POINT('',#135252) ;
#35273=VERTEX_POINT('',#135258) ;
#35274=VERTEX_POINT('',#135259) ;
#35275=VERTEX_POINT('',#135261) ;
#35276=VERTEX_POINT('',#135263) ;
#35277=VERTEX_POINT('',#135268) ;
#35278=VERTEX_POINT('',#135270) ;
#35279=VERTEX_POINT('',#135274) ;
#35280=VERTEX_POINT('',#135276) ;
#35281=VERTEX_POINT('',#135280) ;
#35282=VERTEX_POINT('',#135285) ;
#35283=VERTEX_POINT('',#135287) ;
#35284=VERTEX_POINT('',#135289) ;
#35285=VERTEX_POINT('',#135291) ;
#35286=VERTEX_POINT('',#135296) ;
#35287=VERTEX_POINT('',#135297) ;
#35288=VERTEX_POINT('',#135299) ;
#35289=VERTEX_POINT('',#135301) ;
#35290=VERTEX_POINT('',#135303) ;
#35291=VERTEX_POINT('',#135305) ;
#35292=VERTEX_POINT('',#135500) ;
#35293=VERTEX_POINT('',#135561) ;
#35294=VERTEX_POINT('',#135562) ;
#35295=VERTEX_POINT('',#135801) ;
#35296=VERTEX_POINT('',#135802) ;
#35297=VERTEX_POINT('',#135843) ;
#35298=VERTEX_POINT('',#136256) ;
#35299=VERTEX_POINT('',#136257) ;
#35300=VERTEX_POINT('',#136259) ;
#35301=VERTEX_POINT('',#136261) ;
#35302=VERTEX_POINT('',#136265) ;
#35303=VERTEX_POINT('',#136267) ;
#35304=VERTEX_POINT('',#136269) ;
#35305=VERTEX_POINT('',#136273) ;
#35306=VERTEX_POINT('',#136275) ;
#35307=VERTEX_POINT('',#136279) ;
#35308=VERTEX_POINT('',#136281) ;
#35309=VERTEX_POINT('',#136283) ;
#35310=VERTEX_POINT('',#136287) ;
#35311=VERTEX_POINT('',#136288) ;
#35312=VERTEX_POINT('',#136290) ;
#35313=VERTEX_POINT('',#136292) ;
#35314=VERTEX_POINT('',#136296) ;
#35315=VERTEX_POINT('',#136297) ;
#35316=VERTEX_POINT('',#136299) ;
#35317=VERTEX_POINT('',#136303) ;
#35318=VERTEX_POINT('',#136305) ;
#35319=VERTEX_POINT('',#136309) ;
#35320=VERTEX_POINT('',#136310) ;
#35321=VERTEX_POINT('',#136312) ;
#35322=VERTEX_POINT('',#136316) ;
#35323=VERTEX_POINT('',#136322) ;
#35324=VERTEX_POINT('',#136323) ;
#35325=VERTEX_POINT('',#136325) ;
#35326=VERTEX_POINT('',#136336) ;
#35327=VERTEX_POINT('',#136338) ;
#35328=VERTEX_POINT('',#136349) ;
#35329=VERTEX_POINT('',#136351) ;
#35330=VERTEX_POINT('',#136362) ;
#35331=VERTEX_POINT('',#136364) ;
#35332=VERTEX_POINT('',#136396) ;
#35333=VERTEX_POINT('',#136398) ;
#35334=VERTEX_POINT('',#136409) ;
#35335=VERTEX_POINT('',#136411) ;
#35336=VERTEX_POINT('',#136422) ;
#35337=VERTEX_POINT('',#136424) ;
#35338=VERTEX_POINT('',#136435) ;
#35339=VERTEX_POINT('',#136437) ;
#35340=VERTEX_POINT('',#136472) ;
#35341=VERTEX_POINT('',#136473) ;
#35342=VERTEX_POINT('',#136475) ;
#35343=VERTEX_POINT('',#136477) ;
#35344=VERTEX_POINT('',#136481) ;
#35345=VERTEX_POINT('',#136482) ;
#35346=VERTEX_POINT('',#136484) ;
#35347=VERTEX_POINT('',#136486) ;
#35348=VERTEX_POINT('',#136490) ;
#35349=VERTEX_POINT('',#136492) ;
#35350=VERTEX_POINT('',#136494) ;
#35351=VERTEX_POINT('',#136498) ;
#35352=VERTEX_POINT('',#136500) ;
#35353=VERTEX_POINT('',#136504) ;
#35354=VERTEX_POINT('',#136506) ;
#35355=VERTEX_POINT('',#136508) ;
#35356=VERTEX_POINT('',#136512) ;
#35357=VERTEX_POINT('',#136513) ;
#35358=VERTEX_POINT('',#136515) ;
#35359=VERTEX_POINT('',#136517) ;
#35360=VERTEX_POINT('',#136521) ;
#35361=VERTEX_POINT('',#136522) ;
#35362=VERTEX_POINT('',#136524) ;
#35363=VERTEX_POINT('',#136528) ;
#35364=VERTEX_POINT('',#136530) ;
#35365=VERTEX_POINT('',#136534) ;
#35366=VERTEX_POINT('',#136535) ;
#35367=VERTEX_POINT('',#136537) ;
#35368=VERTEX_POINT('',#136541) ;
#35369=VERTEX_POINT('',#136547) ;
#35370=VERTEX_POINT('',#136548) ;
#35371=VERTEX_POINT('',#136550) ;
#35372=VERTEX_POINT('',#136561) ;
#35373=VERTEX_POINT('',#136563) ;
#35374=VERTEX_POINT('',#136574) ;
#35375=VERTEX_POINT('',#136576) ;
#35376=VERTEX_POINT('',#136587) ;
#35377=VERTEX_POINT('',#136589) ;
#35378=VERTEX_POINT('',#136621) ;
#35379=VERTEX_POINT('',#136623) ;
#35380=VERTEX_POINT('',#136634) ;
#35381=VERTEX_POINT('',#136636) ;
#35382=VERTEX_POINT('',#136647) ;
#35383=VERTEX_POINT('',#136649) ;
#35384=VERTEX_POINT('',#136660) ;
#35385=VERTEX_POINT('',#136662) ;
#35386=VERTEX_POINT('',#136697) ;
#35387=VERTEX_POINT('',#136698) ;
#35388=VERTEX_POINT('',#136700) ;
#35389=VERTEX_POINT('',#136702) ;
#35390=VERTEX_POINT('',#136705) ;
#35391=VERTEX_POINT('',#136706) ;
#35392=VERTEX_POINT('',#136708) ;
#35393=VERTEX_POINT('',#136710) ;
#35394=VERTEX_POINT('',#136715) ;
#35395=VERTEX_POINT('',#136717) ;
#35396=VERTEX_POINT('',#136722) ;
#35397=VERTEX_POINT('',#136724) ;
#35398=VERTEX_POINT('',#136728) ;
#35399=VERTEX_POINT('',#136729) ;
#35400=VERTEX_POINT('',#136731) ;
#35401=VERTEX_POINT('',#136733) ;
#35402=VERTEX_POINT('',#136737) ;
#35403=VERTEX_POINT('',#136738) ;
#35404=VERTEX_POINT('',#136740) ;
#35405=VERTEX_POINT('',#136742) ;
#35406=VERTEX_POINT('',#136746) ;
#35407=VERTEX_POINT('',#136747) ;
#35408=VERTEX_POINT('',#136749) ;
#35409=VERTEX_POINT('',#136751) ;
#35410=VERTEX_POINT('',#136755) ;
#35411=VERTEX_POINT('',#136757) ;
#35412=VERTEX_POINT('',#136767) ;
#35413=VERTEX_POINT('',#136768) ;
#35414=VERTEX_POINT('',#136770) ;
#35415=VERTEX_POINT('',#136773) ;
#35416=VERTEX_POINT('',#136777) ;
#35417=VERTEX_POINT('',#136778) ;
#35418=VERTEX_POINT('',#136780) ;
#35419=VERTEX_POINT('',#136782) ;
#35420=VERTEX_POINT('',#136786) ;
#35421=VERTEX_POINT('',#136787) ;
#35422=VERTEX_POINT('',#136789) ;
#35423=VERTEX_POINT('',#136791) ;
#35424=VERTEX_POINT('',#136795) ;
#35425=VERTEX_POINT('',#136796) ;
#35426=VERTEX_POINT('',#136798) ;
#35427=VERTEX_POINT('',#136807) ;
#35428=VERTEX_POINT('',#136809) ;
#35429=VERTEX_POINT('',#136813) ;
#35430=VERTEX_POINT('',#136815) ;
#35431=VERTEX_POINT('',#136817) ;
#35432=VERTEX_POINT('',#136819) ;
#35433=VERTEX_POINT('',#136821) ;
#35434=VERTEX_POINT('',#136823) ;
#35435=VERTEX_POINT('',#136825) ;
#35436=VERTEX_POINT('',#136827) ;
#35437=VERTEX_POINT('',#136829) ;
#35438=VERTEX_POINT('',#136831) ;
#35439=VERTEX_POINT('',#136833) ;
#35440=VERTEX_POINT('',#136835) ;
#35441=VERTEX_POINT('',#136838) ;
#35442=VERTEX_POINT('',#136840) ;
#35443=VERTEX_POINT('',#136844) ;
#35444=VERTEX_POINT('',#136846) ;
#35445=VERTEX_POINT('',#136851) ;
#35446=VERTEX_POINT('',#136852) ;
#35447=VERTEX_POINT('',#136854) ;
#35448=VERTEX_POINT('',#136856) ;
#35449=VERTEX_POINT('',#136858) ;
#35450=VERTEX_POINT('',#136860) ;
#35451=VERTEX_POINT('',#136862) ;
#35452=VERTEX_POINT('',#136864) ;
#35453=VERTEX_POINT('',#136866) ;
#35454=VERTEX_POINT('',#136868) ;
#35455=VERTEX_POINT('',#136870) ;
#35456=VERTEX_POINT('',#136872) ;
#35457=VERTEX_POINT('',#136876) ;
#35458=VERTEX_POINT('',#136878) ;
#35459=VERTEX_POINT('',#136882) ;
#35460=VERTEX_POINT('',#136884) ;
#35461=VERTEX_POINT('',#136889) ;
#35462=VERTEX_POINT('',#136890) ;
#35463=VERTEX_POINT('',#136892) ;
#35464=VERTEX_POINT('',#136894) ;
#35465=VERTEX_POINT('',#136897) ;
#35466=VERTEX_POINT('',#136898) ;
#35467=VERTEX_POINT('',#136900) ;
#35468=VERTEX_POINT('',#136902) ;
#35469=VERTEX_POINT('',#136904) ;
#35470=VERTEX_POINT('',#136906) ;
#35471=VERTEX_POINT('',#136908) ;
#35472=VERTEX_POINT('',#136910) ;
#35473=VERTEX_POINT('',#136913) ;
#35474=VERTEX_POINT('',#136914) ;
#35475=VERTEX_POINT('',#136916) ;
#35476=VERTEX_POINT('',#136918) ;
#35477=VERTEX_POINT('',#136920) ;
#35478=VERTEX_POINT('',#136922) ;
#35479=VERTEX_POINT('',#136924) ;
#35480=VERTEX_POINT('',#136926) ;
#35481=VERTEX_POINT('',#136930) ;
#35482=VERTEX_POINT('',#136931) ;
#35483=VERTEX_POINT('',#136933) ;
#35484=VERTEX_POINT('',#136935) ;
#35485=VERTEX_POINT('',#136939) ;
#35486=VERTEX_POINT('',#136941) ;
#35487=VERTEX_POINT('',#136945) ;
#35488=VERTEX_POINT('',#136947) ;
#35489=VERTEX_POINT('',#136951) ;
#35490=VERTEX_POINT('',#136952) ;
#35491=VERTEX_POINT('',#136954) ;
#35492=VERTEX_POINT('',#136956) ;
#35493=VERTEX_POINT('',#136959) ;
#35494=VERTEX_POINT('',#136960) ;
#35495=VERTEX_POINT('',#136962) ;
#35496=VERTEX_POINT('',#136969) ;
#35497=VERTEX_POINT('',#136971) ;
#35498=VERTEX_POINT('',#136978) ;
#35499=VERTEX_POINT('',#136980) ;
#35500=VERTEX_POINT('',#136987) ;
#35501=VERTEX_POINT('',#136995) ;
#35502=VERTEX_POINT('',#136996) ;
#35503=VERTEX_POINT('',#136998) ;
#35504=VERTEX_POINT('',#137005) ;
#35505=VERTEX_POINT('',#137007) ;
#35506=VERTEX_POINT('',#137014) ;
#35507=VERTEX_POINT('',#137016) ;
#35508=VERTEX_POINT('',#137023) ;
#35509=VERTEX_POINT('',#137032) ;
#35510=VERTEX_POINT('',#137033) ;
#35511=VERTEX_POINT('',#137035) ;
#35512=VERTEX_POINT('',#137037) ;
#35513=VERTEX_POINT('',#137040) ;
#35514=VERTEX_POINT('',#137041) ;
#35515=VERTEX_POINT('',#137043) ;
#35516=VERTEX_POINT('',#137045) ;
#35517=VERTEX_POINT('',#137047) ;
#35518=VERTEX_POINT('',#137049) ;
#35519=VERTEX_POINT('',#137051) ;
#35520=VERTEX_POINT('',#137053) ;
#35521=VERTEX_POINT('',#137056) ;
#35522=VERTEX_POINT('',#137057) ;
#35523=VERTEX_POINT('',#137059) ;
#35524=VERTEX_POINT('',#137061) ;
#35525=VERTEX_POINT('',#137063) ;
#35526=VERTEX_POINT('',#137065) ;
#35527=VERTEX_POINT('',#137067) ;
#35528=VERTEX_POINT('',#137069) ;
#35529=VERTEX_POINT('',#137073) ;
#35530=VERTEX_POINT('',#137074) ;
#35531=VERTEX_POINT('',#137076) ;
#35532=VERTEX_POINT('',#137078) ;
#35533=VERTEX_POINT('',#137082) ;
#35534=VERTEX_POINT('',#137083) ;
#35535=VERTEX_POINT('',#137112) ;
#35536=VERTEX_POINT('',#137123) ;
#35537=VERTEX_POINT('',#137149) ;
#35538=VERTEX_POINT('',#137166) ;
#35539=VERTEX_POINT('',#137168) ;
#35540=VERTEX_POINT('',#137197) ;
#35541=VERTEX_POINT('',#137208) ;
#35542=VERTEX_POINT('',#137234) ;
#35543=VERTEX_POINT('',#137251) ;
#35544=VERTEX_POINT('',#137253) ;
#35545=VERTEX_POINT('',#137255) ;
#35546=VERTEX_POINT('',#137257) ;
#35547=VERTEX_POINT('',#137261) ;
#35548=VERTEX_POINT('',#137262) ;
#35549=VERTEX_POINT('',#137264) ;
#35550=VERTEX_POINT('',#137266) ;
#35551=VERTEX_POINT('',#137270) ;
#35552=VERTEX_POINT('',#137271) ;
#35553=VERTEX_POINT('',#137273) ;
#35554=VERTEX_POINT('',#137275) ;
#35555=VERTEX_POINT('',#137294) ;
#35556=VERTEX_POINT('',#137295) ;
#35557=VERTEX_POINT('',#137297) ;
#35558=VERTEX_POINT('',#137299) ;
#35559=VERTEX_POINT('',#137303) ;
#35560=VERTEX_POINT('',#137304) ;
#35561=VERTEX_POINT('',#137306) ;
#35562=VERTEX_POINT('',#137308) ;
#35563=VERTEX_POINT('',#137312) ;
#35564=VERTEX_POINT('',#137313) ;
#35565=VERTEX_POINT('',#137315) ;
#35566=VERTEX_POINT('',#137317) ;
#35567=VERTEX_POINT('',#137319) ;
#35568=VERTEX_POINT('',#137321) ;
#35569=VERTEX_POINT('',#137323) ;
#35570=VERTEX_POINT('',#137325) ;
#35571=VERTEX_POINT('',#137329) ;
#35572=VERTEX_POINT('',#137330) ;
#35573=VERTEX_POINT('',#137332) ;
#35574=VERTEX_POINT('',#137334) ;
#35575=VERTEX_POINT('',#137337) ;
#35576=VERTEX_POINT('',#137339) ;
#35577=VERTEX_POINT('',#137343) ;
#35578=VERTEX_POINT('',#137344) ;
#35579=VERTEX_POINT('',#137347) ;
#35580=VERTEX_POINT('',#137349) ;
#35581=VERTEX_POINT('',#137351) ;
#35582=VERTEX_POINT('',#137353) ;
#35583=VERTEX_POINT('',#137357) ;
#35584=VERTEX_POINT('',#137359) ;
#35585=VERTEX_POINT('',#137363) ;
#35586=VERTEX_POINT('',#137365) ;
#35587=VERTEX_POINT('',#137369) ;
#35588=VERTEX_POINT('',#137370) ;
#35589=VERTEX_POINT('',#137372) ;
#35590=VERTEX_POINT('',#137374) ;
#35591=VERTEX_POINT('',#137376) ;
#35592=VERTEX_POINT('',#137378) ;
#35593=VERTEX_POINT('',#137382) ;
#35594=VERTEX_POINT('',#137383) ;
#35595=VERTEX_POINT('',#137385) ;
#35596=VERTEX_POINT('',#137387) ;
#35597=VERTEX_POINT('',#137389) ;
#35598=VERTEX_POINT('',#137391) ;
#35599=VERTEX_POINT('',#137395) ;
#35600=VERTEX_POINT('',#137396) ;
#35601=VERTEX_POINT('',#137398) ;
#35602=VERTEX_POINT('',#137400) ;
#35603=VERTEX_POINT('',#137404) ;
#35604=VERTEX_POINT('',#137405) ;
#35605=VERTEX_POINT('',#137407) ;
#35606=VERTEX_POINT('',#137409) ;
#35607=VERTEX_POINT('',#137413) ;
#35608=VERTEX_POINT('',#137414) ;
#35609=VERTEX_POINT('',#137416) ;
#35610=VERTEX_POINT('',#137418) ;
#35611=VERTEX_POINT('',#137422) ;
#35612=VERTEX_POINT('',#137423) ;
#35613=VERTEX_POINT('',#137425) ;
#35614=VERTEX_POINT('',#137427) ;
#35615=VERTEX_POINT('',#137431) ;
#35616=VERTEX_POINT('',#137432) ;
#35617=VERTEX_POINT('',#137434) ;
#35618=VERTEX_POINT('',#137436) ;
#35619=VERTEX_POINT('',#137439) ;
#35620=VERTEX_POINT('',#137440) ;
#35621=VERTEX_POINT('',#137442) ;
#35622=VERTEX_POINT('',#137444) ;
#35623=VERTEX_POINT('',#137446) ;
#35624=VERTEX_POINT('',#137448) ;
#35625=VERTEX_POINT('',#137450) ;
#35626=VERTEX_POINT('',#137452) ;
#35627=VERTEX_POINT('',#137456) ;
#35628=VERTEX_POINT('',#137457) ;
#35629=VERTEX_POINT('',#137462) ;
#35630=VERTEX_POINT('',#137466) ;
#35631=VERTEX_POINT('',#137470) ;
#35632=VERTEX_POINT('',#137474) ;
#35633=VERTEX_POINT('',#137478) ;
#35634=VERTEX_POINT('',#137482) ;
#35635=VERTEX_POINT('',#137500) ;
#35636=VERTEX_POINT('',#137501) ;
#35637=VERTEX_POINT('',#137503) ;
#35638=VERTEX_POINT('',#137505) ;
#35639=VERTEX_POINT('',#137509) ;
#35640=VERTEX_POINT('',#137510) ;
#35641=VERTEX_POINT('',#137512) ;
#35642=VERTEX_POINT('',#137514) ;
#35643=VERTEX_POINT('',#137518) ;
#35644=VERTEX_POINT('',#137519) ;
#35645=VERTEX_POINT('',#137521) ;
#35646=VERTEX_POINT('',#137523) ;
#35647=VERTEX_POINT('',#137527) ;
#35648=VERTEX_POINT('',#137528) ;
#35649=VERTEX_POINT('',#137530) ;
#35650=VERTEX_POINT('',#137532) ;
#35651=VERTEX_POINT('',#137536) ;
#35652=VERTEX_POINT('',#137537) ;
#35653=VERTEX_POINT('',#137539) ;
#35654=VERTEX_POINT('',#137541) ;
#35655=VERTEX_POINT('',#137544) ;
#35656=VERTEX_POINT('',#137545) ;
#35657=VERTEX_POINT('',#137547) ;
#35658=VERTEX_POINT('',#137549) ;
#35659=VERTEX_POINT('',#137551) ;
#35660=VERTEX_POINT('',#137553) ;
#35661=VERTEX_POINT('',#137555) ;
#35662=VERTEX_POINT('',#137557) ;
#35663=VERTEX_POINT('',#137561) ;
#35664=VERTEX_POINT('',#137563) ;
#35665=VERTEX_POINT('',#137567) ;
#35666=VERTEX_POINT('',#137571) ;
#35667=VERTEX_POINT('',#137575) ;
#35668=VERTEX_POINT('',#137579) ;
#35669=VERTEX_POINT('',#137583) ;
#35670=VERTEX_POINT('',#137587) ;
#35671=VERTEX_POINT('',#137593) ;
#35672=VERTEX_POINT('',#137594) ;
#35673=VERTEX_POINT('',#137596) ;
#35674=VERTEX_POINT('',#137598) ;
#35675=VERTEX_POINT('',#137603) ;
#35676=VERTEX_POINT('',#137605) ;
#35677=VERTEX_POINT('',#137609) ;
#35678=VERTEX_POINT('',#137611) ;
#35679=VERTEX_POINT('',#137615) ;
#35680=VERTEX_POINT('',#137620) ;
#35681=VERTEX_POINT('',#137622) ;
#35682=VERTEX_POINT('',#137624) ;
#35683=VERTEX_POINT('',#137626) ;
#35684=VERTEX_POINT('',#137631) ;
#35685=VERTEX_POINT('',#137632) ;
#35686=VERTEX_POINT('',#137634) ;
#35687=VERTEX_POINT('',#137636) ;
#35688=VERTEX_POINT('',#137638) ;
#35689=VERTEX_POINT('',#137640) ;
#35690=VERTEX_POINT('',#137835) ;
#35691=VERTEX_POINT('',#137897) ;
#35692=VERTEX_POINT('',#137898) ;
#35693=VERTEX_POINT('',#138164) ;
#35694=VERTEX_POINT('',#138165) ;
#35695=VERTEX_POINT('',#138206) ;
#35696=VERTEX_POINT('',#138541) ;
#35697=VERTEX_POINT('',#138542) ;
#35698=VERTEX_POINT('',#138544) ;
#35699=VERTEX_POINT('',#138546) ;
#35700=VERTEX_POINT('',#138550) ;
#35701=VERTEX_POINT('',#138552) ;
#35702=VERTEX_POINT('',#138556) ;
#35703=VERTEX_POINT('',#138558) ;
#35704=VERTEX_POINT('',#138562) ;
#35705=VERTEX_POINT('',#138564) ;
#35706=VERTEX_POINT('',#138568) ;
#35707=VERTEX_POINT('',#138570) ;
#35708=VERTEX_POINT('',#138574) ;
#35709=VERTEX_POINT('',#138576) ;
#35710=VERTEX_POINT('',#138580) ;
#35711=VERTEX_POINT('',#138582) ;
#35712=VERTEX_POINT('',#138586) ;
#35713=VERTEX_POINT('',#138588) ;
#35714=VERTEX_POINT('',#138592) ;
#35715=VERTEX_POINT('',#138594) ;
#35716=VERTEX_POINT('',#138598) ;
#35717=VERTEX_POINT('',#138599) ;
#35718=VERTEX_POINT('',#138601) ;
#35719=VERTEX_POINT('',#138603) ;
#35720=VERTEX_POINT('',#138605) ;
#35721=VERTEX_POINT('',#138607) ;
#35722=VERTEX_POINT('',#138609) ;
#35723=VERTEX_POINT('',#138613) ;
#35724=VERTEX_POINT('',#138614) ;
#35725=VERTEX_POINT('',#138616) ;
#35726=VERTEX_POINT('',#138618) ;
#35727=VERTEX_POINT('',#138620) ;
#35728=VERTEX_POINT('',#138622) ;
#35729=VERTEX_POINT('',#138624) ;
#35730=VERTEX_POINT('',#138628) ;
#35731=VERTEX_POINT('',#138629) ;
#35732=VERTEX_POINT('',#138631) ;
#35733=VERTEX_POINT('',#138633) ;
#35734=VERTEX_POINT('',#138639) ;
#35735=VERTEX_POINT('',#138641) ;
#35736=VERTEX_POINT('',#138643) ;
#35737=VERTEX_POINT('',#138647) ;
#35738=VERTEX_POINT('',#138648) ;
#35739=VERTEX_POINT('',#138650) ;
#35740=VERTEX_POINT('',#138652) ;
#35741=VERTEX_POINT('',#138662) ;
#35742=VERTEX_POINT('',#138663) ;
#35743=VERTEX_POINT('',#138665) ;
#35744=VERTEX_POINT('',#138667) ;
#35745=VERTEX_POINT('',#138671) ;
#35746=VERTEX_POINT('',#138672) ;
#35747=VERTEX_POINT('',#138674) ;
#35748=VERTEX_POINT('',#138676) ;
#35749=VERTEX_POINT('',#138680) ;
#35750=VERTEX_POINT('',#138681) ;
#35751=VERTEX_POINT('',#138683) ;
#35752=VERTEX_POINT('',#138685) ;
#35753=VERTEX_POINT('',#138687) ;
#35754=VERTEX_POINT('',#138689) ;
#35755=VERTEX_POINT('',#138691) ;
#35756=VERTEX_POINT('',#138693) ;
#35757=VERTEX_POINT('',#138697) ;
#35758=VERTEX_POINT('',#138698) ;
#35759=VERTEX_POINT('',#138700) ;
#35760=VERTEX_POINT('',#138702) ;
#35761=VERTEX_POINT('',#138705) ;
#35762=VERTEX_POINT('',#138707) ;
#35763=VERTEX_POINT('',#138711) ;
#35764=VERTEX_POINT('',#138712) ;
#35765=VERTEX_POINT('',#138715) ;
#35766=VERTEX_POINT('',#138717) ;
#35767=VERTEX_POINT('',#138719) ;
#35768=VERTEX_POINT('',#138721) ;
#35769=VERTEX_POINT('',#138725) ;
#35770=VERTEX_POINT('',#138727) ;
#35771=VERTEX_POINT('',#138731) ;
#35772=VERTEX_POINT('',#138733) ;
#35773=VERTEX_POINT('',#138737) ;
#35774=VERTEX_POINT('',#138738) ;
#35775=VERTEX_POINT('',#138740) ;
#35776=VERTEX_POINT('',#138742) ;
#35777=VERTEX_POINT('',#138744) ;
#35778=VERTEX_POINT('',#138746) ;
#35779=VERTEX_POINT('',#138750) ;
#35780=VERTEX_POINT('',#138751) ;
#35781=VERTEX_POINT('',#138753) ;
#35782=VERTEX_POINT('',#138755) ;
#35783=VERTEX_POINT('',#138757) ;
#35784=VERTEX_POINT('',#138759) ;
#35785=VERTEX_POINT('',#138763) ;
#35786=VERTEX_POINT('',#138764) ;
#35787=VERTEX_POINT('',#138766) ;
#35788=VERTEX_POINT('',#138768) ;
#35789=VERTEX_POINT('',#138772) ;
#35790=VERTEX_POINT('',#138773) ;
#35791=VERTEX_POINT('',#138775) ;
#35792=VERTEX_POINT('',#138777) ;
#35793=VERTEX_POINT('',#138781) ;
#35794=VERTEX_POINT('',#138782) ;
#35795=VERTEX_POINT('',#138784) ;
#35796=VERTEX_POINT('',#138786) ;
#35797=VERTEX_POINT('',#138790) ;
#35798=VERTEX_POINT('',#138791) ;
#35799=VERTEX_POINT('',#138793) ;
#35800=VERTEX_POINT('',#138795) ;
#35801=VERTEX_POINT('',#138799) ;
#35802=VERTEX_POINT('',#138800) ;
#35803=VERTEX_POINT('',#138802) ;
#35804=VERTEX_POINT('',#138804) ;
#35805=VERTEX_POINT('',#138807) ;
#35806=VERTEX_POINT('',#138808) ;
#35807=VERTEX_POINT('',#138810) ;
#35808=VERTEX_POINT('',#138812) ;
#35809=VERTEX_POINT('',#138814) ;
#35810=VERTEX_POINT('',#138816) ;
#35811=VERTEX_POINT('',#138818) ;
#35812=VERTEX_POINT('',#138820) ;
#35813=VERTEX_POINT('',#138824) ;
#35814=VERTEX_POINT('',#138825) ;
#35815=VERTEX_POINT('',#138830) ;
#35816=VERTEX_POINT('',#138834) ;
#35817=VERTEX_POINT('',#138838) ;
#35818=VERTEX_POINT('',#138842) ;
#35819=VERTEX_POINT('',#138846) ;
#35820=VERTEX_POINT('',#138850) ;
#35821=VERTEX_POINT('',#138868) ;
#35822=VERTEX_POINT('',#138869) ;
#35823=VERTEX_POINT('',#138871) ;
#35824=VERTEX_POINT('',#138873) ;
#35825=VERTEX_POINT('',#138877) ;
#35826=VERTEX_POINT('',#138878) ;
#35827=VERTEX_POINT('',#138880) ;
#35828=VERTEX_POINT('',#138882) ;
#35829=VERTEX_POINT('',#138886) ;
#35830=VERTEX_POINT('',#138887) ;
#35831=VERTEX_POINT('',#138889) ;
#35832=VERTEX_POINT('',#138891) ;
#35833=VERTEX_POINT('',#138895) ;
#35834=VERTEX_POINT('',#138896) ;
#35835=VERTEX_POINT('',#138898) ;
#35836=VERTEX_POINT('',#138900) ;
#35837=VERTEX_POINT('',#138904) ;
#35838=VERTEX_POINT('',#138905) ;
#35839=VERTEX_POINT('',#138907) ;
#35840=VERTEX_POINT('',#138909) ;
#35841=VERTEX_POINT('',#138912) ;
#35842=VERTEX_POINT('',#138913) ;
#35843=VERTEX_POINT('',#138915) ;
#35844=VERTEX_POINT('',#138917) ;
#35845=VERTEX_POINT('',#138919) ;
#35846=VERTEX_POINT('',#138921) ;
#35847=VERTEX_POINT('',#138923) ;
#35848=VERTEX_POINT('',#138925) ;
#35849=VERTEX_POINT('',#138929) ;
#35850=VERTEX_POINT('',#138931) ;
#35851=VERTEX_POINT('',#138935) ;
#35852=VERTEX_POINT('',#138939) ;
#35853=VERTEX_POINT('',#138943) ;
#35854=VERTEX_POINT('',#138947) ;
#35855=VERTEX_POINT('',#138951) ;
#35856=VERTEX_POINT('',#138955) ;
#35857=VERTEX_POINT('',#138961) ;
#35858=VERTEX_POINT('',#138962) ;
#35859=VERTEX_POINT('',#138964) ;
#35860=VERTEX_POINT('',#138966) ;
#35861=VERTEX_POINT('',#138971) ;
#35862=VERTEX_POINT('',#138973) ;
#35863=VERTEX_POINT('',#138977) ;
#35864=VERTEX_POINT('',#138979) ;
#35865=VERTEX_POINT('',#138983) ;
#35866=VERTEX_POINT('',#138988) ;
#35867=VERTEX_POINT('',#138990) ;
#35868=VERTEX_POINT('',#138992) ;
#35869=VERTEX_POINT('',#138994) ;
#35870=VERTEX_POINT('',#138999) ;
#35871=VERTEX_POINT('',#139000) ;
#35872=VERTEX_POINT('',#139002) ;
#35873=VERTEX_POINT('',#139004) ;
#35874=VERTEX_POINT('',#139006) ;
#35875=VERTEX_POINT('',#139008) ;
#35876=VERTEX_POINT('',#139202) ;
#35877=VERTEX_POINT('',#139264) ;
#35878=VERTEX_POINT('',#139265) ;
#35879=VERTEX_POINT('',#139504) ;
#35880=VERTEX_POINT('',#139505) ;
#35881=VERTEX_POINT('',#139546) ;
#35882=VERTEX_POINT('',#139959) ;
#35883=VERTEX_POINT('',#139960) ;
#35884=VERTEX_POINT('',#139962) ;
#35885=VERTEX_POINT('',#139964) ;
#35886=VERTEX_POINT('',#139968) ;
#35887=VERTEX_POINT('',#139969) ;
#35888=VERTEX_POINT('',#139971) ;
#35889=VERTEX_POINT('',#139973) ;
#35890=VERTEX_POINT('',#139977) ;
#35891=VERTEX_POINT('',#139979) ;
#35892=VERTEX_POINT('',#139981) ;
#35893=VERTEX_POINT('',#139985) ;
#35894=VERTEX_POINT('',#139987) ;
#35895=VERTEX_POINT('',#139991) ;
#35896=VERTEX_POINT('',#139993) ;
#35897=VERTEX_POINT('',#139995) ;
#35898=VERTEX_POINT('',#139999) ;
#35899=VERTEX_POINT('',#140000) ;
#35900=VERTEX_POINT('',#140002) ;
#35901=VERTEX_POINT('',#140004) ;
#35902=VERTEX_POINT('',#140008) ;
#35903=VERTEX_POINT('',#140009) ;
#35904=VERTEX_POINT('',#140011) ;
#35905=VERTEX_POINT('',#140015) ;
#35906=VERTEX_POINT('',#140017) ;
#35907=VERTEX_POINT('',#140021) ;
#35908=VERTEX_POINT('',#140022) ;
#35909=VERTEX_POINT('',#140024) ;
#35910=VERTEX_POINT('',#140028) ;
#35911=VERTEX_POINT('',#140034) ;
#35912=VERTEX_POINT('',#140035) ;
#35913=VERTEX_POINT('',#140037) ;
#35914=VERTEX_POINT('',#140048) ;
#35915=VERTEX_POINT('',#140050) ;
#35916=VERTEX_POINT('',#140061) ;
#35917=VERTEX_POINT('',#140063) ;
#35918=VERTEX_POINT('',#140074) ;
#35919=VERTEX_POINT('',#140076) ;
#35920=VERTEX_POINT('',#140108) ;
#35921=VERTEX_POINT('',#140110) ;
#35922=VERTEX_POINT('',#140121) ;
#35923=VERTEX_POINT('',#140123) ;
#35924=VERTEX_POINT('',#140134) ;
#35925=VERTEX_POINT('',#140136) ;
#35926=VERTEX_POINT('',#140147) ;
#35927=VERTEX_POINT('',#140149) ;
#35928=VERTEX_POINT('',#140184) ;
#35929=VERTEX_POINT('',#140185) ;
#35930=VERTEX_POINT('',#140187) ;
#35931=VERTEX_POINT('',#140189) ;
#35932=VERTEX_POINT('',#140193) ;
#35933=VERTEX_POINT('',#140194) ;
#35934=VERTEX_POINT('',#140196) ;
#35935=VERTEX_POINT('',#140198) ;
#35936=VERTEX_POINT('',#140202) ;
#35937=VERTEX_POINT('',#140203) ;
#35938=VERTEX_POINT('',#140205) ;
#35939=VERTEX_POINT('',#140213) ;
#35940=VERTEX_POINT('',#140215) ;
#35941=VERTEX_POINT('',#140217) ;
#35942=VERTEX_POINT('',#140219) ;
#35943=VERTEX_POINT('',#140221) ;
#35944=VERTEX_POINT('',#140223) ;
#35945=VERTEX_POINT('',#140225) ;
#35946=VERTEX_POINT('',#140227) ;
#35947=VERTEX_POINT('',#140230) ;
#35948=VERTEX_POINT('',#140232) ;
#35949=VERTEX_POINT('',#140236) ;
#35950=VERTEX_POINT('',#140238) ;
#35951=VERTEX_POINT('',#140240) ;
#35952=VERTEX_POINT('',#140244) ;
#35953=VERTEX_POINT('',#140245) ;
#35954=VERTEX_POINT('',#140247) ;
#35955=VERTEX_POINT('',#140249) ;
#35956=VERTEX_POINT('',#140251) ;
#35957=VERTEX_POINT('',#140253) ;
#35958=VERTEX_POINT('',#140255) ;
#35959=VERTEX_POINT('',#140257) ;
#35960=VERTEX_POINT('',#140261) ;
#35961=VERTEX_POINT('',#140262) ;
#35962=VERTEX_POINT('',#140264) ;
#35963=VERTEX_POINT('',#140266) ;
#35964=VERTEX_POINT('',#140270) ;
#35965=VERTEX_POINT('',#140271) ;
#35966=VERTEX_POINT('',#140273) ;
#35967=VERTEX_POINT('',#140275) ;
#35968=VERTEX_POINT('',#140279) ;
#35969=VERTEX_POINT('',#140280) ;
#35970=VERTEX_POINT('',#140282) ;
#35971=VERTEX_POINT('',#140284) ;
#35972=VERTEX_POINT('',#140288) ;
#35973=VERTEX_POINT('',#140289) ;
#35974=VERTEX_POINT('',#140291) ;
#35975=VERTEX_POINT('',#140293) ;
#35976=VERTEX_POINT('',#140297) ;
#35977=VERTEX_POINT('',#140298) ;
#35978=VERTEX_POINT('',#140300) ;
#35979=VERTEX_POINT('',#140302) ;
#35980=VERTEX_POINT('',#140306) ;
#35981=VERTEX_POINT('',#140307) ;
#35982=VERTEX_POINT('',#140309) ;
#35983=VERTEX_POINT('',#140311) ;
#35984=VERTEX_POINT('',#140315) ;
#35985=VERTEX_POINT('',#140316) ;
#35986=VERTEX_POINT('',#140318) ;
#35987=VERTEX_POINT('',#140320) ;
#35988=VERTEX_POINT('',#140323) ;
#35989=VERTEX_POINT('',#140324) ;
#35990=VERTEX_POINT('',#140326) ;
#35991=VERTEX_POINT('',#140328) ;
#35992=VERTEX_POINT('',#140330) ;
#35993=VERTEX_POINT('',#140332) ;
#35994=VERTEX_POINT('',#140334) ;
#35995=VERTEX_POINT('',#140336) ;
#35996=VERTEX_POINT('',#140340) ;
#35997=VERTEX_POINT('',#140341) ;
#35998=VERTEX_POINT('',#140343) ;
#35999=VERTEX_POINT('',#140345) ;
#36000=VERTEX_POINT('',#140349) ;
#36001=VERTEX_POINT('',#140351) ;
#36002=VERTEX_POINT('',#140355) ;
#36003=VERTEX_POINT('',#140357) ;
#36004=VERTEX_POINT('',#140361) ;
#36005=VERTEX_POINT('',#140362) ;
#36006=VERTEX_POINT('',#140364) ;
#36007=VERTEX_POINT('',#140366) ;
#36008=VERTEX_POINT('',#140369) ;
#36009=VERTEX_POINT('',#140370) ;
#36010=VERTEX_POINT('',#140372) ;
#36011=VERTEX_POINT('',#140379) ;
#36012=VERTEX_POINT('',#140381) ;
#36013=VERTEX_POINT('',#140388) ;
#36014=VERTEX_POINT('',#140390) ;
#36015=VERTEX_POINT('',#140397) ;
#36016=VERTEX_POINT('',#140406) ;
#36017=VERTEX_POINT('',#140407) ;
#36018=VERTEX_POINT('',#140409) ;
#36019=VERTEX_POINT('',#140411) ;
#36020=VERTEX_POINT('',#140414) ;
#36021=VERTEX_POINT('',#140415) ;
#36022=VERTEX_POINT('',#140417) ;
#36023=VERTEX_POINT('',#140419) ;
#36024=VERTEX_POINT('',#140421) ;
#36025=VERTEX_POINT('',#140423) ;
#36026=VERTEX_POINT('',#140425) ;
#36027=VERTEX_POINT('',#140427) ;
#36028=VERTEX_POINT('',#140431) ;
#36029=VERTEX_POINT('',#140432) ;
#36030=VERTEX_POINT('',#140434) ;
#36031=VERTEX_POINT('',#140436) ;
#36032=VERTEX_POINT('',#140440) ;
#36033=VERTEX_POINT('',#140441) ;
#36034=VERTEX_POINT('',#140470) ;
#36035=VERTEX_POINT('',#140481) ;
#36036=VERTEX_POINT('',#140507) ;
#36037=VERTEX_POINT('',#140524) ;
#36038=VERTEX_POINT('',#140526) ;
#36039=VERTEX_POINT('',#140528) ;
#36040=VERTEX_POINT('',#140530) ;
#36041=VERTEX_POINT('',#140534) ;
#36042=VERTEX_POINT('',#140535) ;
#36043=VERTEX_POINT('',#140537) ;
#36044=VERTEX_POINT('',#140539) ;
#36045=VERTEX_POINT('',#140543) ;
#36046=VERTEX_POINT('',#140544) ;
#36047=VERTEX_POINT('',#140546) ;
#36048=VERTEX_POINT('',#140548) ;
#36049=VERTEX_POINT('',#140590) ;
#36050=VERTEX_POINT('',#140591) ;
#36051=VERTEX_POINT('',#140593) ;
#36052=VERTEX_POINT('',#140595) ;
#36053=VERTEX_POINT('',#140599) ;
#36054=VERTEX_POINT('',#140600) ;
#36055=VERTEX_POINT('',#140602) ;
#36056=VERTEX_POINT('',#140604) ;
#36057=VERTEX_POINT('',#140608) ;
#36058=VERTEX_POINT('',#140609) ;
#36059=VERTEX_POINT('',#140611) ;
#36060=VERTEX_POINT('',#140613) ;
#36061=VERTEX_POINT('',#140615) ;
#36062=VERTEX_POINT('',#140617) ;
#36063=VERTEX_POINT('',#140619) ;
#36064=VERTEX_POINT('',#140621) ;
#36065=VERTEX_POINT('',#140625) ;
#36066=VERTEX_POINT('',#140626) ;
#36067=VERTEX_POINT('',#140628) ;
#36068=VERTEX_POINT('',#140630) ;
#36069=VERTEX_POINT('',#140633) ;
#36070=VERTEX_POINT('',#140635) ;
#36071=VERTEX_POINT('',#140639) ;
#36072=VERTEX_POINT('',#140640) ;
#36073=VERTEX_POINT('',#140643) ;
#36074=VERTEX_POINT('',#140645) ;
#36075=VERTEX_POINT('',#140647) ;
#36076=VERTEX_POINT('',#140649) ;
#36077=VERTEX_POINT('',#140653) ;
#36078=VERTEX_POINT('',#140655) ;
#36079=VERTEX_POINT('',#140659) ;
#36080=VERTEX_POINT('',#140661) ;
#36081=VERTEX_POINT('',#140665) ;
#36082=VERTEX_POINT('',#140666) ;
#36083=VERTEX_POINT('',#140668) ;
#36084=VERTEX_POINT('',#140670) ;
#36085=VERTEX_POINT('',#140672) ;
#36086=VERTEX_POINT('',#140674) ;
#36087=VERTEX_POINT('',#140678) ;
#36088=VERTEX_POINT('',#140679) ;
#36089=VERTEX_POINT('',#140681) ;
#36090=VERTEX_POINT('',#140683) ;
#36091=VERTEX_POINT('',#140685) ;
#36092=VERTEX_POINT('',#140687) ;
#36093=VERTEX_POINT('',#140691) ;
#36094=VERTEX_POINT('',#140692) ;
#36095=VERTEX_POINT('',#140694) ;
#36096=VERTEX_POINT('',#140696) ;
#36097=VERTEX_POINT('',#140700) ;
#36098=VERTEX_POINT('',#140701) ;
#36099=VERTEX_POINT('',#140703) ;
#36100=VERTEX_POINT('',#140705) ;
#36101=VERTEX_POINT('',#140709) ;
#36102=VERTEX_POINT('',#140710) ;
#36103=VERTEX_POINT('',#140712) ;
#36104=VERTEX_POINT('',#140714) ;
#36105=VERTEX_POINT('',#140718) ;
#36106=VERTEX_POINT('',#140719) ;
#36107=VERTEX_POINT('',#140721) ;
#36108=VERTEX_POINT('',#140723) ;
#36109=VERTEX_POINT('',#140727) ;
#36110=VERTEX_POINT('',#140728) ;
#36111=VERTEX_POINT('',#140730) ;
#36112=VERTEX_POINT('',#140732) ;
#36113=VERTEX_POINT('',#140735) ;
#36114=VERTEX_POINT('',#140736) ;
#36115=VERTEX_POINT('',#140738) ;
#36116=VERTEX_POINT('',#140740) ;
#36117=VERTEX_POINT('',#140742) ;
#36118=VERTEX_POINT('',#140744) ;
#36119=VERTEX_POINT('',#140746) ;
#36120=VERTEX_POINT('',#140748) ;
#36121=VERTEX_POINT('',#140752) ;
#36122=VERTEX_POINT('',#140753) ;
#36123=VERTEX_POINT('',#140758) ;
#36124=VERTEX_POINT('',#140762) ;
#36125=VERTEX_POINT('',#140766) ;
#36126=VERTEX_POINT('',#140770) ;
#36127=VERTEX_POINT('',#140774) ;
#36128=VERTEX_POINT('',#140778) ;
#36129=VERTEX_POINT('',#140796) ;
#36130=VERTEX_POINT('',#140797) ;
#36131=VERTEX_POINT('',#140799) ;
#36132=VERTEX_POINT('',#140801) ;
#36133=VERTEX_POINT('',#140805) ;
#36134=VERTEX_POINT('',#140806) ;
#36135=VERTEX_POINT('',#140808) ;
#36136=VERTEX_POINT('',#140810) ;
#36137=VERTEX_POINT('',#140814) ;
#36138=VERTEX_POINT('',#140815) ;
#36139=VERTEX_POINT('',#140817) ;
#36140=VERTEX_POINT('',#140819) ;
#36141=VERTEX_POINT('',#140823) ;
#36142=VERTEX_POINT('',#140824) ;
#36143=VERTEX_POINT('',#140826) ;
#36144=VERTEX_POINT('',#140828) ;
#36145=VERTEX_POINT('',#140832) ;
#36146=VERTEX_POINT('',#140833) ;
#36147=VERTEX_POINT('',#140835) ;
#36148=VERTEX_POINT('',#140837) ;
#36149=VERTEX_POINT('',#140840) ;
#36150=VERTEX_POINT('',#140841) ;
#36151=VERTEX_POINT('',#140843) ;
#36152=VERTEX_POINT('',#140845) ;
#36153=VERTEX_POINT('',#140847) ;
#36154=VERTEX_POINT('',#140849) ;
#36155=VERTEX_POINT('',#140851) ;
#36156=VERTEX_POINT('',#140853) ;
#36157=VERTEX_POINT('',#140857) ;
#36158=VERTEX_POINT('',#140859) ;
#36159=VERTEX_POINT('',#140863) ;
#36160=VERTEX_POINT('',#140867) ;
#36161=VERTEX_POINT('',#140871) ;
#36162=VERTEX_POINT('',#140875) ;
#36163=VERTEX_POINT('',#140879) ;
#36164=VERTEX_POINT('',#140883) ;
#36165=VERTEX_POINT('',#140889) ;
#36166=VERTEX_POINT('',#140890) ;
#36167=VERTEX_POINT('',#140892) ;
#36168=VERTEX_POINT('',#140894) ;
#36169=VERTEX_POINT('',#140899) ;
#36170=VERTEX_POINT('',#140901) ;
#36171=VERTEX_POINT('',#140905) ;
#36172=VERTEX_POINT('',#140907) ;
#36173=VERTEX_POINT('',#140911) ;
#36174=VERTEX_POINT('',#140916) ;
#36175=VERTEX_POINT('',#140918) ;
#36176=VERTEX_POINT('',#140920) ;
#36177=VERTEX_POINT('',#140922) ;
#36178=VERTEX_POINT('',#140927) ;
#36179=VERTEX_POINT('',#140928) ;
#36180=VERTEX_POINT('',#140930) ;
#36181=VERTEX_POINT('',#140932) ;
#36182=VERTEX_POINT('',#140934) ;
#36183=VERTEX_POINT('',#140936) ;
#36184=VERTEX_POINT('',#141131) ;
#36185=VERTEX_POINT('',#141193) ;
#36186=VERTEX_POINT('',#141194) ;
#36187=VERTEX_POINT('',#141452) ;
#36188=VERTEX_POINT('',#141453) ;
#36189=VERTEX_POINT('',#141494) ;
#41593=EDGE_CURVE('',#34714,#34715,#28626,.T.) ;
#41594=EDGE_CURVE('',#34716,#34714,#28627,.T.) ;
#41595=EDGE_CURVE('',#34717,#34716,#28628,.T.) ;
#41596=EDGE_CURVE('',#34717,#34715,#28629,.T.) ;
#41597=EDGE_CURVE('',#34718,#34718,#28630,.T.) ;
#41598=EDGE_CURVE('',#34718,#34719,#28631,.T.) ;
#41599=EDGE_CURVE('',#34720,#34719,#28632,.T.) ;
#41600=EDGE_CURVE('',#34719,#34720,#28633,.T.) ;
#41601=EDGE_CURVE('',#34721,#34721,#28634,.T.) ;
#41602=EDGE_CURVE('',#34721,#34722,#28635,.T.) ;
#41603=EDGE_CURVE('',#34722,#34722,#28636,.T.) ;
#41604=EDGE_CURVE('',#34723,#34723,#28637,.T.) ;
#41605=EDGE_CURVE('',#34723,#34724,#28638,.T.) ;
#41606=EDGE_CURVE('',#34725,#34724,#28639,.T.) ;
#41607=EDGE_CURVE('',#34724,#34725,#28640,.T.) ;
#41608=EDGE_CURVE('',#34726,#34727,#28641,.T.) ;
#41609=EDGE_CURVE('',#34728,#34727,#28642,.T.) ;
#41610=EDGE_CURVE('',#34728,#34729,#28643,.T.) ;
#41611=EDGE_CURVE('',#34729,#34726,#28644,.T.) ;
#41612=EDGE_CURVE('',#34730,#34731,#28645,.T.) ;
#41613=EDGE_CURVE('',#34731,#34732,#28646,.T.) ;
#41614=EDGE_CURVE('',#34730,#34732,#28647,.T.) ;
#41615=EDGE_CURVE('',#34733,#34726,#2430,.T.) ;
#41616=EDGE_CURVE('',#34733,#34734,#28648,.T.) ;
#41617=EDGE_CURVE('',#34727,#34734,#2431,.T.) ;
#41618=EDGE_CURVE('',#34735,#34736,#28649,.T.) ;
#41619=EDGE_CURVE('',#34735,#34737,#28650,.T.) ;
#41620=EDGE_CURVE('',#34736,#34737,#28651,.T.) ;
#41621=EDGE_CURVE('',#34738,#34738,#28652,.T.) ;
#41622=EDGE_CURVE('',#34738,#34721,#2432,.T.) ;
#41623=EDGE_CURVE('',#34722,#34725,#2433,.T.) ;
#41624=EDGE_CURVE('',#34739,#34740,#28653,.T.) ;
#41625=EDGE_CURVE('',#34739,#34741,#1999,.T.) ;
#41626=EDGE_CURVE('',#34742,#34741,#2434,.T.) ;
#41627=EDGE_CURVE('',#34742,#34743,#2000,.T.) ;
#41628=EDGE_CURVE('',#34744,#34743,#28654,.T.) ;
#41629=EDGE_CURVE('',#34744,#34745,#2001,.T.) ;
#41630=EDGE_CURVE('',#34745,#34746,#2435,.T.) ;
#41631=EDGE_CURVE('',#34746,#34747,#2002,.T.) ;
#41632=EDGE_CURVE('',#34748,#34747,#28655,.T.) ;
#41633=EDGE_CURVE('',#34748,#34749,#2003,.T.) ;
#41634=EDGE_CURVE('',#34750,#34749,#2436,.T.) ;
#41635=EDGE_CURVE('',#34750,#34751,#2004,.T.) ;
#41636=EDGE_CURVE('',#34752,#34751,#28656,.T.) ;
#41637=EDGE_CURVE('',#34752,#34753,#2005,.T.) ;
#41638=EDGE_CURVE('',#34753,#34754,#2437,.T.) ;
#41639=EDGE_CURVE('',#34754,#34755,#2006,.T.) ;
#41640=EDGE_CURVE('',#34740,#34755,#28657,.T.) ;
#41641=EDGE_CURVE('',#34740,#34720,#2438,.T.) ;
#41642=EDGE_CURVE('',#34756,#34757,#28658,.T.) ;
#41643=EDGE_CURVE('',#34758,#34756,#28659,.T.) ;
#41644=EDGE_CURVE('',#34759,#34758,#28660,.T.) ;
#41645=EDGE_CURVE('',#34759,#34757,#28661,.T.) ;
#41646=EDGE_CURVE('',#34760,#34761,#28662,.T.) ;
#41647=EDGE_CURVE('',#34762,#34760,#2439,.T.) ;
#41648=EDGE_CURVE('',#34763,#34762,#28663,.T.) ;
#41649=EDGE_CURVE('',#34761,#34763,#2440,.T.) ;
#41650=EDGE_CURVE('',#34764,#34764,#28664,.T.) ;
#41651=EDGE_CURVE('',#34764,#34765,#28665,.T.) ;
#41652=EDGE_CURVE('',#34766,#34765,#28666,.T.) ;
#41653=EDGE_CURVE('',#34765,#34766,#28667,.T.) ;
#41654=EDGE_CURVE('',#34767,#34767,#28668,.T.) ;
#41655=EDGE_CURVE('',#34767,#34768,#28669,.T.) ;
#41656=EDGE_CURVE('',#34768,#34768,#28670,.T.) ;
#41657=EDGE_CURVE('',#34769,#34769,#28671,.T.) ;
#41658=EDGE_CURVE('',#34769,#34770,#28672,.T.) ;
#41659=EDGE_CURVE('',#34771,#34770,#28673,.T.) ;
#41660=EDGE_CURVE('',#34770,#34771,#28674,.T.) ;
#41661=EDGE_CURVE('',#34772,#34773,#28675,.T.) ;
#41662=EDGE_CURVE('',#34774,#34773,#28676,.T.) ;
#41663=EDGE_CURVE('',#34774,#34775,#28677,.T.) ;
#41664=EDGE_CURVE('',#34775,#34772,#28678,.T.) ;
#41665=EDGE_CURVE('',#34776,#34777,#28679,.T.) ;
#41666=EDGE_CURVE('',#34777,#34778,#28680,.T.) ;
#41667=EDGE_CURVE('',#34776,#34778,#28681,.T.) ;
#41668=EDGE_CURVE('',#34779,#34772,#2441,.T.) ;
#41669=EDGE_CURVE('',#34779,#34780,#28682,.T.) ;
#41670=EDGE_CURVE('',#34773,#34780,#2442,.T.) ;
#41671=EDGE_CURVE('',#34781,#34782,#28683,.T.) ;
#41672=EDGE_CURVE('',#34781,#34783,#28684,.T.) ;
#41673=EDGE_CURVE('',#34782,#34783,#28685,.T.) ;
#41674=EDGE_CURVE('',#34784,#34784,#28686,.T.) ;
#41675=EDGE_CURVE('',#34784,#34767,#2443,.T.) ;
#41676=EDGE_CURVE('',#34768,#34771,#2444,.T.) ;
#41677=EDGE_CURVE('',#34785,#34786,#28687,.T.) ;
#41678=EDGE_CURVE('',#34785,#34787,#2007,.T.) ;
#41679=EDGE_CURVE('',#34788,#34787,#2445,.T.) ;
#41680=EDGE_CURVE('',#34788,#34789,#2008,.T.) ;
#41681=EDGE_CURVE('',#34790,#34789,#28688,.T.) ;
#41682=EDGE_CURVE('',#34790,#34791,#2009,.T.) ;
#41683=EDGE_CURVE('',#34791,#34792,#2446,.T.) ;
#41684=EDGE_CURVE('',#34792,#34793,#2010,.T.) ;
#41685=EDGE_CURVE('',#34794,#34793,#28689,.T.) ;
#41686=EDGE_CURVE('',#34794,#34795,#2011,.T.) ;
#41687=EDGE_CURVE('',#34796,#34795,#2447,.T.) ;
#41688=EDGE_CURVE('',#34796,#34797,#2012,.T.) ;
#41689=EDGE_CURVE('',#34798,#34797,#28690,.T.) ;
#41690=EDGE_CURVE('',#34798,#34799,#2013,.T.) ;
#41691=EDGE_CURVE('',#34799,#34800,#2448,.T.) ;
#41692=EDGE_CURVE('',#34800,#34801,#2014,.T.) ;
#41693=EDGE_CURVE('',#34786,#34801,#28691,.T.) ;
#41694=EDGE_CURVE('',#34786,#34766,#2449,.T.) ;
#41695=EDGE_CURVE('',#34802,#34803,#2450,.T.) ;
#41696=EDGE_CURVE('',#34803,#34804,#2451,.T.) ;
#41697=EDGE_CURVE('',#34805,#34804,#2452,.T.) ;
#41698=EDGE_CURVE('',#34805,#34802,#2453,.T.) ;
#41699=EDGE_CURVE('',#34806,#34807,#28692,.T.) ;
#41700=EDGE_CURVE('',#34806,#34808,#2454,.T.) ;
#41701=EDGE_CURVE('',#34809,#34808,#2015,.T.) ;
#41702=EDGE_CURVE('',#34809,#34810,#2455,.T.) ;
#41703=EDGE_CURVE('',#34811,#34810,#2016,.T.) ;
#41704=EDGE_CURVE('',#34811,#34812,#2456,.T.) ;
#41705=EDGE_CURVE('',#34813,#34812,#28693,.T.) ;
#41706=EDGE_CURVE('',#34813,#34807,#2457,.T.) ;
#41707=EDGE_CURVE('',#34814,#34815,#2458,.T.) ;
#41708=EDGE_CURVE('',#34814,#34816,#2459,.T.) ;
#41709=EDGE_CURVE('',#34816,#34817,#2460,.T.) ;
#41710=EDGE_CURVE('',#34817,#34815,#2461,.T.) ;
#41711=EDGE_CURVE('',#34818,#34819,#2462,.T.) ;
#41712=EDGE_CURVE('',#34818,#34820,#2463,.T.) ;
#41713=EDGE_CURVE('',#34820,#34821,#2464,.T.) ;
#41714=EDGE_CURVE('',#34821,#34819,#2465,.T.) ;
#41715=EDGE_CURVE('',#34822,#34823,#2466,.T.) ;
#41716=EDGE_CURVE('',#34822,#34824,#2467,.T.) ;
#41717=EDGE_CURVE('',#34824,#34825,#2468,.T.) ;
#41718=EDGE_CURVE('',#34825,#34823,#2469,.T.) ;
#41719=EDGE_CURVE('',#34826,#34827,#2470,.T.) ;
#41720=EDGE_CURVE('',#34826,#34823,#28694,.T.) ;
#41721=EDGE_CURVE('',#34827,#34825,#28695,.T.) ;
#41722=EDGE_CURVE('',#34819,#34822,#28696,.T.) ;
#41723=EDGE_CURVE('',#34824,#34821,#28697,.T.) ;
#41724=EDGE_CURVE('',#34815,#34818,#28698,.T.) ;
#41725=EDGE_CURVE('',#34820,#34817,#28699,.T.) ;
#41726=EDGE_CURVE('',#34814,#34828,#28700,.T.) ;
#41727=EDGE_CURVE('',#34828,#34829,#2471,.T.) ;
#41728=EDGE_CURVE('',#34830,#34829,#28701,.T.) ;
#41729=EDGE_CURVE('',#34831,#34830,#2472,.T.) ;
#41730=EDGE_CURVE('',#34816,#34831,#28702,.T.) ;
#41731=EDGE_CURVE('',#34832,#34833,#28703,.T.) ;
#41732=EDGE_CURVE('',#34833,#34834,#2473,.T.) ;
#41733=EDGE_CURVE('',#34834,#34835,#28704,.T.) ;
#41734=EDGE_CURVE('',#34835,#34832,#2474,.T.) ;
#41735=EDGE_CURVE('',#34836,#34837,#2475,.T.) ;
#41736=EDGE_CURVE('',#34836,#34838,#2476,.T.) ;
#41737=EDGE_CURVE('',#34838,#34839,#2477,.T.) ;
#41738=EDGE_CURVE('',#34839,#34837,#2478,.T.) ;
#41739=EDGE_CURVE('',#34783,#34731,#2479,.T.) ;
#41740=EDGE_CURVE('',#34731,#34840,#2480,.T.) ;
#41741=EDGE_CURVE('',#34840,#34841,#2481,.T.) ;
#41742=EDGE_CURVE('',#34841,#34783,#2482,.T.) ;
#41743=EDGE_CURVE('',#34801,#34785,#2483,.T.) ;
#41744=EDGE_CURVE('',#34774,#34778,#2484,.T.) ;
#41745=EDGE_CURVE('',#34778,#34842,#2485,.T.) ;
#41746=EDGE_CURVE('',#34843,#34842,#2486,.T.) ;
#41747=EDGE_CURVE('',#34843,#34844,#2487,.T.) ;
#41748=EDGE_CURVE('',#34845,#34844,#28705,.T.) ;
#41749=EDGE_CURVE('',#34845,#34846,#28706,.T.) ;
#41750=EDGE_CURVE('',#34847,#34846,#28707,.T.) ;
#41751=EDGE_CURVE('',#34847,#34848,#2488,.T.) ;
#41752=EDGE_CURVE('',#34849,#34848,#28708,.T.) ;
#41753=EDGE_CURVE('',#34849,#34850,#28709,.T.) ;
#41754=EDGE_CURVE('',#34851,#34850,#28710,.T.) ;
#41755=EDGE_CURVE('',#34851,#34852,#2489,.T.) ;
#41756=EDGE_CURVE('',#34852,#34853,#2490,.T.) ;
#41757=EDGE_CURVE('',#34853,#34735,#2491,.T.) ;
#41758=EDGE_CURVE('',#34735,#34854,#2492,.T.) ;
#41759=EDGE_CURVE('',#34855,#34854,#28711,.T.) ;
#41760=EDGE_CURVE('',#34855,#34729,#2493,.T.) ;
#41761=EDGE_CURVE('',#34728,#34732,#2494,.T.) ;
#41762=EDGE_CURVE('',#34732,#34781,#2495,.T.) ;
#41763=EDGE_CURVE('',#34781,#34856,#2496,.T.) ;
#41764=EDGE_CURVE('',#34857,#34856,#28712,.T.) ;
#41765=EDGE_CURVE('',#34857,#34775,#2497,.T.) ;
#41766=EDGE_CURVE('',#34777,#34858,#2498,.T.) ;
#41767=EDGE_CURVE('',#34858,#34859,#2499,.T.) ;
#41768=EDGE_CURVE('',#34860,#34859,#2500,.T.) ;
#41769=EDGE_CURVE('',#34860,#34777,#2501,.T.) ;
#41770=EDGE_CURVE('',#34861,#34862,#2502,.T.) ;
#41771=EDGE_CURVE('',#34861,#34863,#2503,.T.) ;
#41772=EDGE_CURVE('',#34863,#34864,#267,.T.) ;
#41773=EDGE_CURVE('',#34864,#34865,#2504,.T.) ;
#41774=EDGE_CURVE('',#34865,#34866,#268,.T.) ;
#41775=EDGE_CURVE('',#34866,#34867,#2505,.T.) ;
#41776=EDGE_CURVE('',#34867,#34868,#269,.T.) ;
#41777=EDGE_CURVE('',#34868,#34869,#2506,.T.) ;
#41778=EDGE_CURVE('',#34869,#34870,#270,.T.) ;
#41779=EDGE_CURVE('',#34870,#34871,#2507,.T.) ;
#41780=EDGE_CURVE('',#34871,#34872,#2508,.T.) ;
#41781=EDGE_CURVE('',#34872,#34862,#2509,.T.) ;
#41782=EDGE_CURVE('',#34873,#34874,#2510,.T.) ;
#41783=EDGE_CURVE('',#34874,#34831,#2511,.T.) ;
#41784=EDGE_CURVE('',#34873,#34830,#2512,.T.) ;
#41785=EDGE_CURVE('',#34827,#34875,#2513,.T.) ;
#41786=EDGE_CURVE('',#34875,#34876,#2514,.T.) ;
#41787=EDGE_CURVE('',#34829,#34876,#2515,.T.) ;
#41788=EDGE_CURVE('',#34826,#34828,#2516,.T.) ;
#41789=EDGE_CURVE('',#34877,#34878,#2517,.T.) ;
#41790=EDGE_CURVE('',#34878,#34879,#2518,.T.) ;
#41791=EDGE_CURVE('',#34879,#34880,#2519,.T.) ;
#41792=EDGE_CURVE('',#34877,#34880,#2520,.T.) ;
#41793=EDGE_CURVE('',#34881,#34882,#28713,.T.) ;
#41794=EDGE_CURVE('',#34881,#34883,#2521,.T.) ;
#41795=EDGE_CURVE('',#34884,#34883,#28714,.T.) ;
#41796=EDGE_CURVE('',#34884,#34885,#2522,.T.) ;
#41797=EDGE_CURVE('',#34886,#34885,#28715,.T.) ;
#41798=EDGE_CURVE('',#34886,#34887,#2523,.T.) ;
#41799=EDGE_CURVE('',#34888,#34887,#28716,.T.) ;
#41800=EDGE_CURVE('',#34888,#34882,#2524,.T.) ;
#41801=EDGE_CURVE('',#34889,#34890,#28717,.T.) ;
#41802=EDGE_CURVE('',#34889,#34891,#2525,.T.) ;
#41803=EDGE_CURVE('',#34892,#34891,#28718,.T.) ;
#41804=EDGE_CURVE('',#34892,#34893,#2526,.T.) ;
#41805=EDGE_CURVE('',#34894,#34893,#28719,.T.) ;
#41806=EDGE_CURVE('',#34894,#34895,#2527,.T.) ;
#41807=EDGE_CURVE('',#34896,#34895,#28720,.T.) ;
#41808=EDGE_CURVE('',#34896,#34890,#2528,.T.) ;
#41809=EDGE_CURVE('',#34897,#34898,#2529,.T.) ;
#41810=EDGE_CURVE('',#34898,#34899,#2530,.T.) ;
#41811=EDGE_CURVE('',#34899,#34900,#2531,.T.) ;
#41812=EDGE_CURVE('',#34897,#34900,#2532,.T.) ;
#41813=EDGE_CURVE('',#34901,#34902,#2533,.T.) ;
#41814=EDGE_CURVE('',#34902,#34761,#2534,.T.) ;
#41815=EDGE_CURVE('',#34901,#34763,#2535,.T.) ;
#41816=EDGE_CURVE('',#34760,#34903,#2536,.T.) ;
#41817=EDGE_CURVE('',#34903,#34904,#2537,.T.) ;
#41818=EDGE_CURVE('',#34762,#34904,#2538,.T.) ;
#41819=EDGE_CURVE('',#34905,#34906,#2539,.T.) ;
#41820=EDGE_CURVE('',#34906,#34907,#2540,.T.) ;
#41821=EDGE_CURVE('',#34907,#34908,#2541,.T.) ;
#41822=EDGE_CURVE('',#34905,#34908,#2542,.T.) ;
#41823=EDGE_CURVE('',#34909,#34910,#2543,.T.) ;
#41824=EDGE_CURVE('',#34910,#34911,#2017,.T.) ;
#41825=EDGE_CURVE('',#34911,#34912,#2544,.T.) ;
#41826=EDGE_CURVE('',#34913,#34912,#2018,.T.) ;
#41827=EDGE_CURVE('',#34913,#34914,#2545,.T.) ;
#41828=EDGE_CURVE('',#34915,#34914,#2019,.T.) ;
#41829=EDGE_CURVE('',#34915,#34916,#2546,.T.) ;
#41830=EDGE_CURVE('',#34916,#34909,#2020,.T.) ;
#41831=EDGE_CURVE('',#34917,#34918,#2547,.T.) ;
#41832=EDGE_CURVE('',#34918,#34919,#2021,.T.) ;
#41833=EDGE_CURVE('',#34919,#34920,#2548,.T.) ;
#41834=EDGE_CURVE('',#34921,#34920,#2022,.T.) ;
#41835=EDGE_CURVE('',#34921,#34922,#2549,.T.) ;
#41836=EDGE_CURVE('',#34923,#34922,#2023,.T.) ;
#41837=EDGE_CURVE('',#34923,#34924,#2550,.T.) ;
#41838=EDGE_CURVE('',#34924,#34917,#2024,.T.) ;
#41839=EDGE_CURVE('',#34925,#34926,#2551,.T.) ;
#41840=EDGE_CURVE('',#34926,#34927,#2552,.T.) ;
#41841=EDGE_CURVE('',#34927,#34928,#2553,.T.) ;
#41842=EDGE_CURVE('',#34925,#34928,#2554,.T.) ;
#41843=EDGE_CURVE('',#34929,#34930,#28721,.T.) ;
#41844=EDGE_CURVE('',#34929,#34931,#2555,.T.) ;
#41845=EDGE_CURVE('',#34932,#34931,#28722,.T.) ;
#41846=EDGE_CURVE('',#34932,#34933,#2556,.T.) ;
#41847=EDGE_CURVE('',#34934,#34933,#28723,.T.) ;
#41848=EDGE_CURVE('',#34934,#34935,#2557,.T.) ;
#41849=EDGE_CURVE('',#34936,#34935,#28724,.T.) ;
#41850=EDGE_CURVE('',#34936,#34930,#2558,.T.) ;
#41851=EDGE_CURVE('',#34937,#34938,#28725,.T.) ;
#41852=EDGE_CURVE('',#34937,#34939,#2559,.T.) ;
#41853=EDGE_CURVE('',#34940,#34939,#28726,.T.) ;
#41854=EDGE_CURVE('',#34940,#34941,#2560,.T.) ;
#41855=EDGE_CURVE('',#34942,#34941,#28727,.T.) ;
#41856=EDGE_CURVE('',#34942,#34943,#2561,.T.) ;
#41857=EDGE_CURVE('',#34944,#34943,#28728,.T.) ;
#41858=EDGE_CURVE('',#34944,#34938,#2562,.T.) ;
#41859=EDGE_CURVE('',#34945,#34946,#2563,.T.) ;
#41860=EDGE_CURVE('',#34946,#34947,#2564,.T.) ;
#41861=EDGE_CURVE('',#34947,#34948,#2565,.T.) ;
#41862=EDGE_CURVE('',#34945,#34948,#2566,.T.) ;
#41863=EDGE_CURVE('',#34949,#34950,#2025,.T.) ;
#41864=EDGE_CURVE('',#34950,#34951,#2026,.T.) ;
#41865=EDGE_CURVE('',#34951,#34952,#2027,.T.) ;
#41866=EDGE_CURVE('',#34952,#34953,#2028,.T.) ;
#41867=EDGE_CURVE('',#34953,#34954,#2567,.T.) ;
#41868=EDGE_CURVE('',#34955,#34954,#2568,.T.) ;
#41869=EDGE_CURVE('',#34955,#34956,#2569,.T.) ;
#41870=EDGE_CURVE('',#34956,#34957,#2570,.T.) ;
#41871=EDGE_CURVE('',#34957,#34958,#2571,.T.) ;
#41872=EDGE_CURVE('',#34958,#34959,#2029,.T.) ;
#41873=EDGE_CURVE('',#34959,#34960,#2030,.T.) ;
#41874=EDGE_CURVE('',#34960,#34961,#2031,.T.) ;
#41875=EDGE_CURVE('',#34961,#34962,#2032,.T.) ;
#41876=EDGE_CURVE('',#34962,#34949,#2572,.T.) ;
#41877=EDGE_CURVE('',#34963,#34964,#2573,.T.) ;
#41878=EDGE_CURVE('',#34963,#34965,#2574,.T.) ;
#41879=EDGE_CURVE('',#34965,#34966,#28729,.T.) ;
#41880=EDGE_CURVE('',#34966,#34964,#2575,.T.) ;
#41881=EDGE_CURVE('',#34967,#34968,#2576,.T.) ;
#41882=EDGE_CURVE('',#34968,#34969,#2577,.T.) ;
#41883=EDGE_CURVE('',#34969,#34970,#2578,.T.) ;
#41884=EDGE_CURVE('',#34970,#34967,#2579,.T.) ;
#41885=EDGE_CURVE('',#34876,#34877,#28730,.T.) ;
#41886=EDGE_CURVE('',#34880,#34897,#28731,.T.) ;
#41887=EDGE_CURVE('',#34900,#34901,#28732,.T.) ;
#41888=EDGE_CURVE('',#34904,#34905,#28733,.T.) ;
#41889=EDGE_CURVE('',#34908,#34925,#28734,.T.) ;
#41890=EDGE_CURVE('',#34928,#34945,#28735,.T.) ;
#41891=EDGE_CURVE('',#34948,#34955,#28736,.T.) ;
#41892=EDGE_CURVE('',#34954,#34963,#28737,.T.) ;
#41893=EDGE_CURVE('',#34964,#34836,#28738,.T.) ;
#41894=EDGE_CURVE('',#34837,#34843,#28739,.T.) ;
#41895=EDGE_CURVE('',#34842,#34860,#28740,.T.) ;
#41896=EDGE_CURVE('',#34859,#34861,#28741,.T.) ;
#41897=EDGE_CURVE('',#34862,#34805,#28742,.T.) ;
#41898=EDGE_CURVE('',#34804,#34873,#28743,.T.) ;
#41899=EDGE_CURVE('',#34971,#34972,#2580,.T.) ;
#41900=EDGE_CURVE('',#34972,#34973,#2581,.T.) ;
#41901=EDGE_CURVE('',#34973,#34974,#2582,.T.) ;
#41902=EDGE_CURVE('',#34974,#34971,#2583,.T.) ;
#41903=EDGE_CURVE('',#34975,#34976,#2584,.T.) ;
#41904=EDGE_CURVE('',#34976,#34977,#2585,.T.) ;
#41905=EDGE_CURVE('',#34977,#34978,#2586,.T.) ;
#41906=EDGE_CURVE('',#34978,#34975,#2587,.T.) ;
#41907=EDGE_CURVE('',#34979,#34980,#271,.T.) ;
#41908=EDGE_CURVE('',#34979,#34981,#2588,.T.) ;
#41909=EDGE_CURVE('',#34981,#34982,#2589,.T.) ;
#41910=EDGE_CURVE('',#34982,#34983,#2590,.T.) ;
#41911=EDGE_CURVE('',#34984,#34983,#272,.T.) ;
#41912=EDGE_CURVE('',#34984,#34985,#2591,.T.) ;
#41913=EDGE_CURVE('',#34985,#34986,#2592,.T.) ;
#41914=EDGE_CURVE('',#34986,#34980,#2593,.T.) ;
#41915=EDGE_CURVE('',#34987,#34988,#2594,.T.) ;
#41916=EDGE_CURVE('',#34988,#34989,#273,.T.) ;
#41917=EDGE_CURVE('',#34990,#34989,#2595,.T.) ;
#41918=EDGE_CURVE('',#34990,#34982,#274,.T.) ;
#41919=EDGE_CURVE('',#34981,#34991,#275,.T.) ;
#41920=EDGE_CURVE('',#34991,#34992,#2596,.T.) ;
#41921=EDGE_CURVE('',#34992,#34987,#276,.T.) ;
#41922=EDGE_CURVE('',#34993,#34994,#277,.T.) ;
#41923=EDGE_CURVE('',#34993,#34988,#2597,.T.) ;
#41924=EDGE_CURVE('',#34987,#34995,#2598,.T.) ;
#41925=EDGE_CURVE('',#34996,#34995,#278,.T.) ;
#41926=EDGE_CURVE('',#34996,#34997,#2599,.T.) ;
#41927=EDGE_CURVE('',#34997,#34998,#2600,.T.) ;
#41928=EDGE_CURVE('',#34998,#34994,#2601,.T.) ;
#41929=EDGE_CURVE('',#34991,#34999,#2602,.T.) ;
#41930=EDGE_CURVE('',#34999,#35000,#2603,.T.) ;
#41931=EDGE_CURVE('',#35000,#34992,#2604,.T.) ;
#41932=EDGE_CURVE('',#34989,#35001,#2605,.T.) ;
#41933=EDGE_CURVE('',#35001,#35002,#2606,.T.) ;
#41934=EDGE_CURVE('',#35002,#34990,#2607,.T.) ;
#41935=EDGE_CURVE('',#35003,#35004,#2608,.T.) ;
#41936=EDGE_CURVE('',#35004,#35005,#2609,.T.) ;
#41937=EDGE_CURVE('',#35005,#35006,#2610,.T.) ;
#41938=EDGE_CURVE('',#35006,#35007,#2611,.T.) ;
#41939=EDGE_CURVE('',#35007,#35008,#2612,.T.) ;
#41940=EDGE_CURVE('',#35008,#35003,#2613,.T.) ;
#41941=EDGE_CURVE('',#35009,#35010,#2614,.T.) ;
#41942=EDGE_CURVE('',#35010,#35011,#2615,.T.) ;
#41943=EDGE_CURVE('',#35011,#35012,#2616,.T.) ;
#41944=EDGE_CURVE('',#35012,#35013,#2617,.T.) ;
#41945=EDGE_CURVE('',#35013,#35014,#2618,.T.) ;
#41946=EDGE_CURVE('',#35014,#35009,#2619,.T.) ;
#41947=EDGE_CURVE('',#35015,#35016,#2620,.T.) ;
#41948=EDGE_CURVE('',#35016,#35017,#2621,.T.) ;
#41949=EDGE_CURVE('',#35017,#35018,#2622,.T.) ;
#41950=EDGE_CURVE('',#35018,#35015,#2623,.T.) ;
#41951=EDGE_CURVE('',#35019,#35020,#2624,.T.) ;
#41952=EDGE_CURVE('',#35020,#35021,#2625,.T.) ;
#41953=EDGE_CURVE('',#35021,#35022,#2626,.T.) ;
#41954=EDGE_CURVE('',#35022,#35019,#2627,.T.) ;
#41955=EDGE_CURVE('',#35023,#35024,#2628,.T.) ;
#41956=EDGE_CURVE('',#35024,#35025,#2629,.T.) ;
#41957=EDGE_CURVE('',#35025,#35026,#2630,.T.) ;
#41958=EDGE_CURVE('',#35026,#35023,#2631,.T.) ;
#41959=EDGE_CURVE('',#35027,#35028,#2632,.T.) ;
#41960=EDGE_CURVE('',#35028,#35029,#2633,.T.) ;
#41961=EDGE_CURVE('',#35029,#35030,#2634,.T.) ;
#41962=EDGE_CURVE('',#35030,#35027,#2635,.T.) ;
#41963=EDGE_CURVE('',#35031,#35032,#2636,.T.) ;
#41964=EDGE_CURVE('',#35032,#35033,#2637,.T.) ;
#41965=EDGE_CURVE('',#35033,#35034,#2638,.T.) ;
#41966=EDGE_CURVE('',#35034,#35031,#2639,.T.) ;
#41967=EDGE_CURVE('',#35035,#35036,#2640,.T.) ;
#41968=EDGE_CURVE('',#35037,#35035,#28744,.T.) ;
#41969=EDGE_CURVE('',#35038,#35037,#2641,.T.) ;
#41970=EDGE_CURVE('',#35039,#35038,#28745,.T.) ;
#41971=EDGE_CURVE('',#35040,#35039,#2642,.T.) ;
#41972=EDGE_CURVE('',#35041,#35040,#28746,.T.) ;
#41973=EDGE_CURVE('',#35042,#35041,#2643,.T.) ;
#41974=EDGE_CURVE('',#35036,#35042,#28747,.T.) ;
#41975=EDGE_CURVE('',#35043,#35044,#28748,.T.) ;
#41976=EDGE_CURVE('',#35036,#35043,#2644,.T.) ;
#41977=EDGE_CURVE('',#35042,#35044,#2645,.T.) ;
#41978=EDGE_CURVE('',#35045,#35043,#2646,.T.) ;
#41979=EDGE_CURVE('',#35035,#35045,#2647,.T.) ;
#41980=EDGE_CURVE('',#35046,#35045,#28749,.T.) ;
#41981=EDGE_CURVE('',#35037,#35046,#2648,.T.) ;
#41982=EDGE_CURVE('',#35047,#35046,#2649,.T.) ;
#41983=EDGE_CURVE('',#35038,#35047,#2650,.T.) ;
#41984=EDGE_CURVE('',#35048,#35047,#28750,.T.) ;
#41985=EDGE_CURVE('',#35039,#35048,#2651,.T.) ;
#41986=EDGE_CURVE('',#35049,#35048,#2652,.T.) ;
#41987=EDGE_CURVE('',#35040,#35049,#2653,.T.) ;
#41988=EDGE_CURVE('',#35050,#35049,#28751,.T.) ;
#41989=EDGE_CURVE('',#35041,#35050,#2654,.T.) ;
#41990=EDGE_CURVE('',#35044,#35050,#2655,.T.) ;
#41991=EDGE_CURVE('',#34793,#34794,#2656,.T.) ;
#41992=EDGE_CURVE('',#34791,#34796,#2657,.T.) ;
#41993=EDGE_CURVE('',#34795,#34792,#2658,.T.) ;
#41994=EDGE_CURVE('',#34799,#34788,#2659,.T.) ;
#41995=EDGE_CURVE('',#34787,#34800,#2660,.T.) ;
#41996=EDGE_CURVE('',#34789,#34798,#2661,.T.) ;
#41997=EDGE_CURVE('',#34797,#34790,#2662,.T.) ;
#41998=EDGE_CURVE('',#35051,#35052,#2663,.T.) ;
#41999=EDGE_CURVE('',#35052,#35053,#2664,.T.) ;
#42000=EDGE_CURVE('',#35053,#35054,#2665,.T.) ;
#42001=EDGE_CURVE('',#35054,#35051,#2666,.T.) ;
#42002=EDGE_CURVE('',#35055,#35056,#2667,.T.) ;
#42003=EDGE_CURVE('',#35056,#35057,#2668,.T.) ;
#42004=EDGE_CURVE('',#35057,#35058,#2669,.T.) ;
#42005=EDGE_CURVE('',#35058,#35055,#2670,.T.) ;
#42006=EDGE_CURVE('',#35059,#35060,#2671,.T.) ;
#42007=EDGE_CURVE('',#35060,#35061,#2672,.T.) ;
#42008=EDGE_CURVE('',#35061,#35062,#2673,.T.) ;
#42009=EDGE_CURVE('',#35062,#35059,#2674,.T.) ;
#42010=EDGE_CURVE('',#35063,#35064,#2675,.T.) ;
#42011=EDGE_CURVE('',#35064,#35065,#2676,.T.) ;
#42012=EDGE_CURVE('',#35065,#35066,#2677,.T.) ;
#42013=EDGE_CURVE('',#35066,#35063,#2678,.T.) ;
#42014=EDGE_CURVE('',#35067,#35068,#2679,.T.) ;
#42015=EDGE_CURVE('',#35068,#35069,#2680,.T.) ;
#42016=EDGE_CURVE('',#35069,#35070,#2681,.T.) ;
#42017=EDGE_CURVE('',#35070,#35067,#2682,.T.) ;
#42018=EDGE_CURVE('',#35071,#35072,#2683,.T.) ;
#42019=EDGE_CURVE('',#35073,#35071,#28752,.T.) ;
#42020=EDGE_CURVE('',#35074,#35073,#2684,.T.) ;
#42021=EDGE_CURVE('',#35075,#35074,#28753,.T.) ;
#42022=EDGE_CURVE('',#35076,#35075,#2685,.T.) ;
#42023=EDGE_CURVE('',#35077,#35076,#28754,.T.) ;
#42024=EDGE_CURVE('',#35078,#35077,#2686,.T.) ;
#42025=EDGE_CURVE('',#35072,#35078,#28755,.T.) ;
#42026=EDGE_CURVE('',#35078,#35079,#2687,.T.) ;
#42027=EDGE_CURVE('',#35079,#35080,#28756,.T.) ;
#42028=EDGE_CURVE('',#35072,#35080,#2688,.T.) ;
#42029=EDGE_CURVE('',#35080,#35081,#2689,.T.) ;
#42030=EDGE_CURVE('',#35071,#35081,#2690,.T.) ;
#42031=EDGE_CURVE('',#35081,#35082,#28757,.T.) ;
#42032=EDGE_CURVE('',#35073,#35082,#2691,.T.) ;
#42033=EDGE_CURVE('',#35082,#35083,#2692,.T.) ;
#42034=EDGE_CURVE('',#35074,#35083,#2693,.T.) ;
#42035=EDGE_CURVE('',#35083,#35084,#28758,.T.) ;
#42036=EDGE_CURVE('',#35075,#35084,#2694,.T.) ;
#42037=EDGE_CURVE('',#35084,#35085,#2695,.T.) ;
#42038=EDGE_CURVE('',#35076,#35085,#2696,.T.) ;
#42039=EDGE_CURVE('',#35085,#35086,#28759,.T.) ;
#42040=EDGE_CURVE('',#35077,#35086,#2697,.T.) ;
#42041=EDGE_CURVE('',#35086,#35079,#2698,.T.) ;
#42042=EDGE_CURVE('',#35087,#35088,#2699,.T.) ;
#42043=EDGE_CURVE('',#35088,#35089,#2700,.T.) ;
#42044=EDGE_CURVE('',#35089,#35090,#2701,.T.) ;
#42045=EDGE_CURVE('',#35090,#35087,#2702,.T.) ;
#42046=EDGE_CURVE('',#34782,#34758,#2703,.T.) ;
#42047=EDGE_CURVE('',#34758,#35091,#2704,.T.) ;
#42048=EDGE_CURVE('',#35091,#35092,#2705,.T.) ;
#42049=EDGE_CURVE('',#35092,#34782,#2706,.T.) ;
#42050=EDGE_CURVE('',#35093,#34779,#2707,.T.) ;
#42051=EDGE_CURVE('',#34772,#35094,#2708,.T.) ;
#42052=EDGE_CURVE('',#35094,#35093,#2709,.T.) ;
#42053=EDGE_CURVE('',#34780,#35095,#2710,.T.) ;
#42054=EDGE_CURVE('',#35095,#34776,#2711,.T.) ;
#42055=EDGE_CURVE('',#34776,#34773,#2712,.T.) ;
#42056=EDGE_CURVE('',#34757,#35096,#2713,.T.) ;
#42057=EDGE_CURVE('',#35096,#35097,#28760,.T.) ;
#42058=EDGE_CURVE('',#35097,#35098,#2714,.T.) ;
#42059=EDGE_CURVE('',#35098,#35099,#2715,.T.) ;
#42060=EDGE_CURVE('',#35099,#34756,#2716,.T.) ;
#42061=EDGE_CURVE('',#35100,#35101,#28761,.T.) ;
#42062=EDGE_CURVE('',#35101,#35102,#28762,.T.) ;
#42063=EDGE_CURVE('',#35102,#35103,#28763,.T.) ;
#42064=EDGE_CURVE('',#35103,#35104,#2717,.T.) ;
#42065=EDGE_CURVE('',#35104,#35105,#28764,.T.) ;
#42066=EDGE_CURVE('',#35105,#35100,#2718,.T.) ;
#42067=EDGE_CURVE('',#35009,#34918,#28765,.T.) ;
#42068=EDGE_CURVE('',#34977,#35009,#2033,.T.) ;
#42069=EDGE_CURVE('',#34919,#34977,#28766,.T.) ;
#42070=EDGE_CURVE('',#34999,#34979,#28767,.T.) ;
#42071=EDGE_CURVE('',#35013,#34980,#28768,.T.) ;
#42072=EDGE_CURVE('',#34999,#35013,#279,.T.) ;
#42073=EDGE_CURVE('',#35014,#34986,#28769,.T.) ;
#42074=EDGE_CURVE('',#34978,#35014,#28770,.T.) ;
#42075=EDGE_CURVE('',#34920,#34976,#28771,.T.) ;
#42076=EDGE_CURVE('',#35010,#34917,#28772,.T.) ;
#42077=EDGE_CURVE('',#35000,#35012,#280,.T.) ;
#42078=EDGE_CURVE('',#34995,#35000,#28773,.T.) ;
#42079=EDGE_CURVE('',#34978,#34986,#28774,.T.) ;
#42080=EDGE_CURVE('',#35007,#34976,#281,.T.) ;
#42081=EDGE_CURVE('',#34921,#35007,#28775,.T.) ;
#42082=EDGE_CURVE('',#34972,#34924,#28776,.T.) ;
#42083=EDGE_CURVE('',#35010,#34972,#2034,.T.) ;
#42084=EDGE_CURVE('',#34996,#35012,#28777,.T.) ;
#42085=EDGE_CURVE('',#34975,#34985,#28778,.T.) ;
#42086=EDGE_CURVE('',#35008,#34975,#28779,.T.) ;
#42087=EDGE_CURVE('',#34922,#35006,#28780,.T.) ;
#42088=EDGE_CURVE('',#34973,#34923,#28781,.T.) ;
#42089=EDGE_CURVE('',#35011,#34971,#28782,.T.) ;
#42090=EDGE_CURVE('',#34997,#35011,#28783,.T.) ;
#42091=EDGE_CURVE('',#35008,#34985,#28784,.T.) ;
#42092=EDGE_CURVE('',#34973,#35006,#282,.T.) ;
#42093=EDGE_CURVE('',#34997,#34971,#28785,.T.) ;
#42094=EDGE_CURVE('',#34983,#35002,#28786,.T.) ;
#42095=EDGE_CURVE('',#35003,#34984,#28787,.T.) ;
#42096=EDGE_CURVE('',#34974,#35005,#28788,.T.) ;
#42097=EDGE_CURVE('',#34998,#34974,#28789,.T.) ;
#42098=EDGE_CURVE('',#35003,#35002,#283,.T.) ;
#42099=EDGE_CURVE('',#34998,#35005,#28790,.T.) ;
#42100=EDGE_CURVE('',#35004,#35001,#284,.T.) ;
#42101=EDGE_CURVE('',#34994,#35004,#28791,.T.) ;
#42102=EDGE_CURVE('',#34993,#35001,#28792,.T.) ;
#42103=EDGE_CURVE('',#34841,#35106,#285,.T.) ;
#42104=EDGE_CURVE('',#35106,#34759,#2035,.T.) ;
#42105=EDGE_CURVE('',#35091,#35093,#28793,.T.) ;
#42106=EDGE_CURVE('',#35092,#35094,#28794,.T.) ;
#42107=EDGE_CURVE('',#34856,#35092,#28795,.T.) ;
#42108=EDGE_CURVE('',#34864,#35096,#2036,.T.) ;
#42109=EDGE_CURVE('',#34757,#34865,#2037,.T.) ;
#42110=EDGE_CURVE('',#35098,#34779,#28796,.T.) ;
#42111=EDGE_CURVE('',#35093,#35099,#28797,.T.) ;
#42112=EDGE_CURVE('',#34857,#35094,#28798,.T.) ;
#42113=EDGE_CURVE('',#35107,#35108,#2038,.T.) ;
#42114=EDGE_CURVE('',#35108,#34858,#286,.T.) ;
#42115=EDGE_CURVE('',#35095,#35107,#28799,.T.) ;
#42116=EDGE_CURVE('',#35082,#35087,#28800,.T.) ;
#42117=EDGE_CURVE('',#35087,#35081,#28801,.T.) ;
#42118=EDGE_CURVE('',#35088,#35080,#28802,.T.) ;
#42119=EDGE_CURVE('',#35083,#35090,#28803,.T.) ;
#42120=EDGE_CURVE('',#35088,#35079,#28804,.T.) ;
#42121=EDGE_CURVE('',#35084,#35090,#28805,.T.) ;
#42122=EDGE_CURVE('',#35089,#35086,#28806,.T.) ;
#42123=EDGE_CURVE('',#35085,#35089,#28807,.T.) ;
#42124=EDGE_CURVE('',#34943,#35018,#28808,.T.) ;
#42125=EDGE_CURVE('',#35015,#34942,#28809,.T.) ;
#42126=EDGE_CURVE('',#35030,#34941,#28810,.T.) ;
#42127=EDGE_CURVE('',#35015,#35030,#28811,.T.) ;
#42128=EDGE_CURVE('',#35022,#35018,#28812,.T.) ;
#42129=EDGE_CURVE('',#34944,#35022,#28813,.T.) ;
#42130=EDGE_CURVE('',#35027,#34940,#28814,.T.) ;
#42131=EDGE_CURVE('',#35016,#35029,#28815,.T.) ;
#42132=EDGE_CURVE('',#35017,#35034,#28816,.T.) ;
#42133=EDGE_CURVE('',#35031,#35016,#28817,.T.) ;
#42134=EDGE_CURVE('',#35019,#35017,#28818,.T.) ;
#42135=EDGE_CURVE('',#34938,#35021,#28819,.T.) ;
#42136=EDGE_CURVE('',#34939,#35025,#28820,.T.) ;
#42137=EDGE_CURVE('',#35026,#34937,#28821,.T.) ;
#42138=EDGE_CURVE('',#35027,#35025,#28822,.T.) ;
#42139=EDGE_CURVE('',#35031,#35029,#28823,.T.) ;
#42140=EDGE_CURVE('',#35019,#35034,#28824,.T.) ;
#42141=EDGE_CURVE('',#35026,#35021,#28825,.T.) ;
#42142=EDGE_CURVE('',#35028,#35024,#28826,.T.) ;
#42143=EDGE_CURVE('',#35032,#35028,#28827,.T.) ;
#42144=EDGE_CURVE('',#35020,#35033,#28828,.T.) ;
#42145=EDGE_CURVE('',#35023,#35020,#28829,.T.) ;
#42146=EDGE_CURVE('',#35032,#35024,#28830,.T.) ;
#42147=EDGE_CURVE('',#35023,#35033,#28831,.T.) ;
#42148=EDGE_CURVE('',#34895,#35062,#28832,.T.) ;
#42149=EDGE_CURVE('',#35059,#34894,#28833,.T.) ;
#42150=EDGE_CURVE('',#35058,#34893,#28834,.T.) ;
#42151=EDGE_CURVE('',#35059,#35058,#28835,.T.) ;
#42152=EDGE_CURVE('',#35066,#35062,#28836,.T.) ;
#42153=EDGE_CURVE('',#34896,#35066,#28837,.T.) ;
#42154=EDGE_CURVE('',#35055,#34892,#28838,.T.) ;
#42155=EDGE_CURVE('',#35060,#35057,#28839,.T.) ;
#42156=EDGE_CURVE('',#35061,#35070,#28840,.T.) ;
#42157=EDGE_CURVE('',#35067,#35060,#28841,.T.) ;
#42158=EDGE_CURVE('',#35063,#35061,#28842,.T.) ;
#42159=EDGE_CURVE('',#34890,#35065,#28843,.T.) ;
#42160=EDGE_CURVE('',#34891,#35053,#28844,.T.) ;
#42161=EDGE_CURVE('',#35054,#34889,#28845,.T.) ;
#42162=EDGE_CURVE('',#35055,#35053,#28846,.T.) ;
#42163=EDGE_CURVE('',#35067,#35057,#28847,.T.) ;
#42164=EDGE_CURVE('',#35063,#35070,#28848,.T.) ;
#42165=EDGE_CURVE('',#35054,#35065,#28849,.T.) ;
#42166=EDGE_CURVE('',#35056,#35052,#28850,.T.) ;
#42167=EDGE_CURVE('',#35068,#35056,#28851,.T.) ;
#42168=EDGE_CURVE('',#35064,#35069,#28852,.T.) ;
#42169=EDGE_CURVE('',#35051,#35064,#28853,.T.) ;
#42170=EDGE_CURVE('',#35068,#35052,#28854,.T.) ;
#42171=EDGE_CURVE('',#35051,#35069,#28855,.T.) ;
#42172=EDGE_CURVE('',#34965,#35101,#2039,.T.) ;
#42173=EDGE_CURVE('',#34966,#35100,#28856,.T.) ;
#42174=EDGE_CURVE('',#34838,#34966,#28857,.T.) ;
#42175=EDGE_CURVE('',#34838,#35100,#28858,.T.) ;
#42176=EDGE_CURVE('',#34839,#35105,#28859,.T.) ;
#42177=EDGE_CURVE('',#34844,#34839,#28860,.T.) ;
#42178=EDGE_CURVE('',#34845,#35105,#28861,.T.) ;
#42179=EDGE_CURVE('',#34846,#35104,#28862,.T.) ;
#42180=EDGE_CURVE('',#34848,#34970,#28863,.T.) ;
#42181=EDGE_CURVE('',#34967,#34847,#28864,.T.) ;
#42182=EDGE_CURVE('',#34967,#35104,#28865,.T.) ;
#42183=EDGE_CURVE('',#34968,#35103,#28866,.T.) ;
#42184=EDGE_CURVE('',#34969,#34835,#28867,.T.) ;
#42185=EDGE_CURVE('',#34832,#34968,#28868,.T.) ;
#42186=EDGE_CURVE('',#34832,#35103,#28869,.T.) ;
#42187=EDGE_CURVE('',#35102,#34833,#2040,.T.) ;
#42188=EDGE_CURVE('',#34956,#34947,#28870,.T.) ;
#42189=EDGE_CURVE('',#34946,#34927,#28871,.T.) ;
#42190=EDGE_CURVE('',#34926,#34907,#28872,.T.) ;
#42191=EDGE_CURVE('',#34906,#34903,#28873,.T.) ;
#42192=EDGE_CURVE('',#34902,#34899,#28874,.T.) ;
#42193=EDGE_CURVE('',#34898,#34879,#28875,.T.) ;
#42194=EDGE_CURVE('',#34878,#34875,#28876,.T.) ;
#42195=EDGE_CURVE('',#34874,#34803,#28877,.T.) ;
#42196=EDGE_CURVE('',#34802,#34872,#28878,.T.) ;
#42197=EDGE_CURVE('',#34780,#35098,#28879,.T.) ;
#42198=EDGE_CURVE('',#35095,#35097,#28880,.T.) ;
#42199=EDGE_CURVE('',#35107,#35096,#28881,.T.) ;
#42200=EDGE_CURVE('',#35108,#34864,#28882,.T.) ;
#42201=EDGE_CURVE('',#34858,#34863,#28883,.T.) ;
#42202=EDGE_CURVE('',#34840,#34867,#28884,.T.) ;
#42203=EDGE_CURVE('',#34841,#34866,#28885,.T.) ;
#42204=EDGE_CURVE('',#35106,#34865,#28886,.T.) ;
#42205=EDGE_CURVE('',#35091,#35099,#28887,.T.) ;
#42206=EDGE_CURVE('',#35109,#35110,#2041,.T.) ;
#42207=EDGE_CURVE('',#35110,#35102,#2042,.T.) ;
#42208=EDGE_CURVE('',#35101,#35111,#2043,.T.) ;
#42209=EDGE_CURVE('',#35111,#35109,#2044,.T.) ;
#42210=EDGE_CURVE('',#34965,#34953,#28888,.T.) ;
#42211=EDGE_CURVE('',#34952,#35101,#2045,.T.) ;
#42212=EDGE_CURVE('',#34834,#34962,#28889,.T.) ;
#42213=EDGE_CURVE('',#34949,#34833,#28890,.T.) ;
#42214=EDGE_CURVE('',#35102,#34950,#2046,.T.) ;
#42215=EDGE_CURVE('',#35111,#34952,#28891,.T.) ;
#42216=EDGE_CURVE('',#35109,#34951,#28892,.T.) ;
#42217=EDGE_CURVE('',#35110,#34950,#28893,.T.) ;
#42218=EDGE_CURVE('',#35112,#35113,#2719,.T.) ;
#42219=EDGE_CURVE('',#35113,#35114,#2720,.T.) ;
#42220=EDGE_CURVE('',#35115,#35114,#2721,.T.) ;
#42221=EDGE_CURVE('',#35115,#35112,#2722,.T.) ;
#42222=EDGE_CURVE('',#35114,#35116,#28894,.T.) ;
#42223=EDGE_CURVE('',#35117,#35116,#2723,.T.) ;
#42224=EDGE_CURVE('',#35117,#35115,#28895,.T.) ;
#42225=EDGE_CURVE('',#35116,#35118,#2724,.T.) ;
#42226=EDGE_CURVE('',#35119,#35118,#2725,.T.) ;
#42227=EDGE_CURVE('',#35119,#35117,#2726,.T.) ;
#42228=EDGE_CURVE('',#35118,#35120,#28896,.T.) ;
#42229=EDGE_CURVE('',#35121,#35120,#2727,.T.) ;
#42230=EDGE_CURVE('',#35121,#35119,#28897,.T.) ;
#42231=EDGE_CURVE('',#35120,#35122,#2728,.T.) ;
#42232=EDGE_CURVE('',#35123,#35122,#2729,.T.) ;
#42233=EDGE_CURVE('',#35123,#35121,#2730,.T.) ;
#42234=EDGE_CURVE('',#35122,#35124,#28898,.T.) ;
#42235=EDGE_CURVE('',#35125,#35124,#2731,.T.) ;
#42236=EDGE_CURVE('',#35125,#35123,#28899,.T.) ;
#42237=EDGE_CURVE('',#35124,#35126,#2732,.T.) ;
#42238=EDGE_CURVE('',#35127,#35126,#2733,.T.) ;
#42239=EDGE_CURVE('',#35127,#35125,#2734,.T.) ;
#42240=EDGE_CURVE('',#35126,#35128,#28900,.T.) ;
#42241=EDGE_CURVE('',#35129,#35128,#2735,.T.) ;
#42242=EDGE_CURVE('',#35129,#35127,#28901,.T.) ;
#42243=EDGE_CURVE('',#35128,#35130,#2736,.T.) ;
#42244=EDGE_CURVE('',#35130,#35131,#2737,.T.) ;
#42245=EDGE_CURVE('',#35131,#35129,#2738,.T.) ;
#42246=EDGE_CURVE('',#35132,#35133,#28902,.T.) ;
#42247=EDGE_CURVE('',#35133,#35134,#2739,.T.) ;
#42248=EDGE_CURVE('',#35134,#35135,#2740,.T.) ;
#42249=EDGE_CURVE('',#35135,#35136,#2741,.T.) ;
#42250=EDGE_CURVE('',#35136,#35137,#2742,.T.) ;
#42251=EDGE_CURVE('',#35137,#35138,#2743,.T.) ;
#42252=EDGE_CURVE('',#35138,#35132,#2744,.T.) ;
#42253=EDGE_CURVE('',#35139,#35140,#2745,.T.) ;
#42254=EDGE_CURVE('',#35140,#35141,#2746,.T.) ;
#42255=EDGE_CURVE('',#35141,#35142,#2747,.T.) ;
#42256=EDGE_CURVE('',#35142,#35143,#2748,.T.) ;
#42257=EDGE_CURVE('',#35143,#35144,#28903,.T.) ;
#42258=EDGE_CURVE('',#35144,#35145,#2749,.T.) ;
#42259=EDGE_CURVE('',#35145,#35139,#2750,.T.) ;
#42260=EDGE_CURVE('',#35146,#35147,#28904,.T.) ;
#42261=EDGE_CURVE('',#35147,#35148,#2751,.T.) ;
#42262=EDGE_CURVE('',#35148,#35149,#2752,.T.) ;
#42263=EDGE_CURVE('',#35149,#35146,#2753,.T.) ;
#42264=EDGE_CURVE('',#35150,#35151,#2754,.T.) ;
#42265=EDGE_CURVE('',#35151,#35152,#2755,.T.) ;
#42266=EDGE_CURVE('',#35152,#34737,#2756,.T.) ;
#42267=EDGE_CURVE('',#34737,#35150,#2757,.T.) ;
#42268=EDGE_CURVE('',#34755,#34739,#2758,.T.) ;
#42269=EDGE_CURVE('',#35153,#35154,#2759,.T.) ;
#42270=EDGE_CURVE('',#35154,#35155,#2760,.T.) ;
#42271=EDGE_CURVE('',#35155,#35156,#2761,.T.) ;
#42272=EDGE_CURVE('',#35156,#35153,#2762,.T.) ;
#42273=EDGE_CURVE('',#35148,#34957,#28905,.T.) ;
#42274=EDGE_CURVE('',#34871,#35151,#28906,.T.) ;
#42275=EDGE_CURVE('',#35150,#34853,#28907,.T.) ;
#42276=EDGE_CURVE('',#34852,#35156,#28908,.T.) ;
#42277=EDGE_CURVE('',#35155,#35149,#28909,.T.) ;
#42278=EDGE_CURVE('',#35157,#35158,#2763,.T.) ;
#42279=EDGE_CURVE('',#35158,#35159,#2764,.T.) ;
#42280=EDGE_CURVE('',#35159,#35160,#2765,.T.) ;
#42281=EDGE_CURVE('',#35160,#35157,#2766,.T.) ;
#42282=EDGE_CURVE('',#35161,#35162,#2767,.T.) ;
#42283=EDGE_CURVE('',#35162,#35163,#2768,.T.) ;
#42284=EDGE_CURVE('',#35163,#35164,#2769,.T.) ;
#42285=EDGE_CURVE('',#35164,#35161,#2770,.T.) ;
#42286=EDGE_CURVE('',#35165,#35166,#287,.T.) ;
#42287=EDGE_CURVE('',#35165,#35167,#2771,.T.) ;
#42288=EDGE_CURVE('',#35167,#35168,#2772,.T.) ;
#42289=EDGE_CURVE('',#35168,#35169,#2773,.T.) ;
#42290=EDGE_CURVE('',#35170,#35169,#288,.T.) ;
#42291=EDGE_CURVE('',#35170,#35171,#2774,.T.) ;
#42292=EDGE_CURVE('',#35171,#35172,#2775,.T.) ;
#42293=EDGE_CURVE('',#35172,#35166,#2776,.T.) ;
#42294=EDGE_CURVE('',#35173,#35174,#2777,.T.) ;
#42295=EDGE_CURVE('',#35174,#35175,#289,.T.) ;
#42296=EDGE_CURVE('',#35176,#35175,#2778,.T.) ;
#42297=EDGE_CURVE('',#35176,#35168,#290,.T.) ;
#42298=EDGE_CURVE('',#35167,#35177,#291,.T.) ;
#42299=EDGE_CURVE('',#35177,#35178,#2779,.T.) ;
#42300=EDGE_CURVE('',#35178,#35173,#292,.T.) ;
#42301=EDGE_CURVE('',#35179,#35180,#293,.T.) ;
#42302=EDGE_CURVE('',#35179,#35174,#2780,.T.) ;
#42303=EDGE_CURVE('',#35173,#35181,#2781,.T.) ;
#42304=EDGE_CURVE('',#35182,#35181,#294,.T.) ;
#42305=EDGE_CURVE('',#35182,#35183,#2782,.T.) ;
#42306=EDGE_CURVE('',#35183,#35184,#2783,.T.) ;
#42307=EDGE_CURVE('',#35184,#35180,#2784,.T.) ;
#42308=EDGE_CURVE('',#35177,#35185,#2785,.T.) ;
#42309=EDGE_CURVE('',#35185,#35186,#2786,.T.) ;
#42310=EDGE_CURVE('',#35186,#35178,#2787,.T.) ;
#42311=EDGE_CURVE('',#35175,#35187,#2788,.T.) ;
#42312=EDGE_CURVE('',#35187,#35188,#2789,.T.) ;
#42313=EDGE_CURVE('',#35188,#35176,#2790,.T.) ;
#42314=EDGE_CURVE('',#35189,#35190,#2791,.T.) ;
#42315=EDGE_CURVE('',#35190,#35191,#2792,.T.) ;
#42316=EDGE_CURVE('',#35191,#35192,#2793,.T.) ;
#42317=EDGE_CURVE('',#35192,#35193,#2794,.T.) ;
#42318=EDGE_CURVE('',#35193,#35194,#2795,.T.) ;
#42319=EDGE_CURVE('',#35194,#35189,#2796,.T.) ;
#42320=EDGE_CURVE('',#35195,#35196,#2797,.T.) ;
#42321=EDGE_CURVE('',#35196,#35197,#2798,.T.) ;
#42322=EDGE_CURVE('',#35197,#35198,#2799,.T.) ;
#42323=EDGE_CURVE('',#35198,#35199,#2800,.T.) ;
#42324=EDGE_CURVE('',#35199,#35200,#2801,.T.) ;
#42325=EDGE_CURVE('',#35200,#35195,#2802,.T.) ;
#42326=EDGE_CURVE('',#35201,#35202,#2803,.T.) ;
#42327=EDGE_CURVE('',#35202,#35203,#2804,.T.) ;
#42328=EDGE_CURVE('',#35203,#35204,#2805,.T.) ;
#42329=EDGE_CURVE('',#35204,#35201,#2806,.T.) ;
#42330=EDGE_CURVE('',#35205,#35206,#2807,.T.) ;
#42331=EDGE_CURVE('',#35206,#35207,#2808,.T.) ;
#42332=EDGE_CURVE('',#35207,#35208,#2809,.T.) ;
#42333=EDGE_CURVE('',#35208,#35205,#2810,.T.) ;
#42334=EDGE_CURVE('',#35209,#35210,#2811,.T.) ;
#42335=EDGE_CURVE('',#35210,#35211,#2812,.T.) ;
#42336=EDGE_CURVE('',#35211,#35212,#2813,.T.) ;
#42337=EDGE_CURVE('',#35212,#35209,#2814,.T.) ;
#42338=EDGE_CURVE('',#35213,#35214,#2815,.T.) ;
#42339=EDGE_CURVE('',#35214,#35215,#2816,.T.) ;
#42340=EDGE_CURVE('',#35215,#35216,#2817,.T.) ;
#42341=EDGE_CURVE('',#35216,#35213,#2818,.T.) ;
#42342=EDGE_CURVE('',#35217,#35218,#2819,.T.) ;
#42343=EDGE_CURVE('',#35218,#35219,#2820,.T.) ;
#42344=EDGE_CURVE('',#35219,#35220,#2821,.T.) ;
#42345=EDGE_CURVE('',#35220,#35217,#2822,.T.) ;
#42346=EDGE_CURVE('',#35221,#35222,#2823,.T.) ;
#42347=EDGE_CURVE('',#35223,#35221,#28910,.T.) ;
#42348=EDGE_CURVE('',#35224,#35223,#2824,.T.) ;
#42349=EDGE_CURVE('',#35225,#35224,#28911,.T.) ;
#42350=EDGE_CURVE('',#35226,#35225,#2825,.T.) ;
#42351=EDGE_CURVE('',#35227,#35226,#28912,.T.) ;
#42352=EDGE_CURVE('',#35228,#35227,#2826,.T.) ;
#42353=EDGE_CURVE('',#35222,#35228,#28913,.T.) ;
#42354=EDGE_CURVE('',#35229,#35230,#28914,.T.) ;
#42355=EDGE_CURVE('',#35222,#35229,#2827,.T.) ;
#42356=EDGE_CURVE('',#35228,#35230,#2828,.T.) ;
#42357=EDGE_CURVE('',#35231,#35229,#2829,.T.) ;
#42358=EDGE_CURVE('',#35221,#35231,#2830,.T.) ;
#42359=EDGE_CURVE('',#35232,#35231,#28915,.T.) ;
#42360=EDGE_CURVE('',#35223,#35232,#2831,.T.) ;
#42361=EDGE_CURVE('',#35233,#35232,#2832,.T.) ;
#42362=EDGE_CURVE('',#35224,#35233,#2833,.T.) ;
#42363=EDGE_CURVE('',#35234,#35233,#28916,.T.) ;
#42364=EDGE_CURVE('',#35225,#35234,#2834,.T.) ;
#42365=EDGE_CURVE('',#35235,#35234,#2835,.T.) ;
#42366=EDGE_CURVE('',#35226,#35235,#2836,.T.) ;
#42367=EDGE_CURVE('',#35236,#35235,#28917,.T.) ;
#42368=EDGE_CURVE('',#35227,#35236,#2837,.T.) ;
#42369=EDGE_CURVE('',#35230,#35236,#2838,.T.) ;
#42370=EDGE_CURVE('',#34747,#34748,#2839,.T.) ;
#42371=EDGE_CURVE('',#34745,#34750,#2840,.T.) ;
#42372=EDGE_CURVE('',#34749,#34746,#2841,.T.) ;
#42373=EDGE_CURVE('',#34753,#34742,#2842,.T.) ;
#42374=EDGE_CURVE('',#34741,#34754,#2843,.T.) ;
#42375=EDGE_CURVE('',#34743,#34752,#2844,.T.) ;
#42376=EDGE_CURVE('',#34751,#34744,#2845,.T.) ;
#42377=EDGE_CURVE('',#35237,#35238,#2846,.T.) ;
#42378=EDGE_CURVE('',#35238,#35239,#2847,.T.) ;
#42379=EDGE_CURVE('',#35239,#35240,#2848,.T.) ;
#42380=EDGE_CURVE('',#35240,#35237,#2849,.T.) ;
#42381=EDGE_CURVE('',#35241,#35242,#2850,.T.) ;
#42382=EDGE_CURVE('',#35242,#35243,#2851,.T.) ;
#42383=EDGE_CURVE('',#35243,#35244,#2852,.T.) ;
#42384=EDGE_CURVE('',#35244,#35241,#2853,.T.) ;
#42385=EDGE_CURVE('',#35245,#35246,#2854,.T.) ;
#42386=EDGE_CURVE('',#35246,#35247,#2855,.T.) ;
#42387=EDGE_CURVE('',#35247,#35248,#2856,.T.) ;
#42388=EDGE_CURVE('',#35248,#35245,#2857,.T.) ;
#42389=EDGE_CURVE('',#35249,#35250,#2858,.T.) ;
#42390=EDGE_CURVE('',#35250,#35251,#2859,.T.) ;
#42391=EDGE_CURVE('',#35251,#35252,#2860,.T.) ;
#42392=EDGE_CURVE('',#35252,#35249,#2861,.T.) ;
#42393=EDGE_CURVE('',#35253,#35254,#2862,.T.) ;
#42394=EDGE_CURVE('',#35254,#35255,#2863,.T.) ;
#42395=EDGE_CURVE('',#35255,#35256,#2864,.T.) ;
#42396=EDGE_CURVE('',#35256,#35253,#2865,.T.) ;
#42397=EDGE_CURVE('',#35257,#35258,#2866,.T.) ;
#42398=EDGE_CURVE('',#35259,#35257,#28918,.T.) ;
#42399=EDGE_CURVE('',#35260,#35259,#2867,.T.) ;
#42400=EDGE_CURVE('',#35261,#35260,#28919,.T.) ;
#42401=EDGE_CURVE('',#35262,#35261,#2868,.T.) ;
#42402=EDGE_CURVE('',#35263,#35262,#28920,.T.) ;
#42403=EDGE_CURVE('',#35264,#35263,#2869,.T.) ;
#42404=EDGE_CURVE('',#35258,#35264,#28921,.T.) ;
#42405=EDGE_CURVE('',#35264,#35265,#2870,.T.) ;
#42406=EDGE_CURVE('',#35265,#35266,#28922,.T.) ;
#42407=EDGE_CURVE('',#35258,#35266,#2871,.T.) ;
#42408=EDGE_CURVE('',#35266,#35267,#2872,.T.) ;
#42409=EDGE_CURVE('',#35257,#35267,#2873,.T.) ;
#42410=EDGE_CURVE('',#35267,#35268,#28923,.T.) ;
#42411=EDGE_CURVE('',#35259,#35268,#2874,.T.) ;
#42412=EDGE_CURVE('',#35268,#35269,#2875,.T.) ;
#42413=EDGE_CURVE('',#35260,#35269,#2876,.T.) ;
#42414=EDGE_CURVE('',#35269,#35270,#28924,.T.) ;
#42415=EDGE_CURVE('',#35261,#35270,#2877,.T.) ;
#42416=EDGE_CURVE('',#35270,#35271,#2878,.T.) ;
#42417=EDGE_CURVE('',#35262,#35271,#2879,.T.) ;
#42418=EDGE_CURVE('',#35271,#35272,#28925,.T.) ;
#42419=EDGE_CURVE('',#35263,#35272,#2880,.T.) ;
#42420=EDGE_CURVE('',#35272,#35265,#2881,.T.) ;
#42421=EDGE_CURVE('',#35273,#35274,#2882,.T.) ;
#42422=EDGE_CURVE('',#35274,#35275,#2883,.T.) ;
#42423=EDGE_CURVE('',#35275,#35276,#2884,.T.) ;
#42424=EDGE_CURVE('',#35276,#35273,#2885,.T.) ;
#42425=EDGE_CURVE('',#34736,#34716,#2886,.T.) ;
#42426=EDGE_CURVE('',#34716,#35277,#2887,.T.) ;
#42427=EDGE_CURVE('',#35277,#35278,#2888,.T.) ;
#42428=EDGE_CURVE('',#35278,#34736,#2889,.T.) ;
#42429=EDGE_CURVE('',#35279,#34733,#2890,.T.) ;
#42430=EDGE_CURVE('',#34726,#35280,#2891,.T.) ;
#42431=EDGE_CURVE('',#35280,#35279,#2892,.T.) ;
#42432=EDGE_CURVE('',#34734,#35281,#2893,.T.) ;
#42433=EDGE_CURVE('',#35281,#34730,#2894,.T.) ;
#42434=EDGE_CURVE('',#34730,#34727,#2895,.T.) ;
#42435=EDGE_CURVE('',#34715,#35282,#2896,.T.) ;
#42436=EDGE_CURVE('',#35282,#35283,#28926,.T.) ;
#42437=EDGE_CURVE('',#35283,#35284,#2897,.T.) ;
#42438=EDGE_CURVE('',#35284,#35285,#2898,.T.) ;
#42439=EDGE_CURVE('',#35285,#34714,#2899,.T.) ;
#42440=EDGE_CURVE('',#35286,#35287,#28927,.T.) ;
#42441=EDGE_CURVE('',#35287,#35288,#28928,.T.) ;
#42442=EDGE_CURVE('',#35288,#35289,#28929,.T.) ;
#42443=EDGE_CURVE('',#35289,#35290,#2900,.T.) ;
#42444=EDGE_CURVE('',#35290,#35291,#28930,.T.) ;
#42445=EDGE_CURVE('',#35291,#35286,#2901,.T.) ;
#42446=EDGE_CURVE('',#35195,#34910,#28931,.T.) ;
#42447=EDGE_CURVE('',#35163,#35195,#2047,.T.) ;
#42448=EDGE_CURVE('',#34911,#35163,#28932,.T.) ;
#42449=EDGE_CURVE('',#35185,#35165,#28933,.T.) ;
#42450=EDGE_CURVE('',#35199,#35166,#28934,.T.) ;
#42451=EDGE_CURVE('',#35185,#35199,#295,.T.) ;
#42452=EDGE_CURVE('',#35200,#35172,#28935,.T.) ;
#42453=EDGE_CURVE('',#35164,#35200,#28936,.T.) ;
#42454=EDGE_CURVE('',#34912,#35162,#28937,.T.) ;
#42455=EDGE_CURVE('',#35196,#34909,#28938,.T.) ;
#42456=EDGE_CURVE('',#35186,#35198,#296,.T.) ;
#42457=EDGE_CURVE('',#35181,#35186,#28939,.T.) ;
#42458=EDGE_CURVE('',#35164,#35172,#28940,.T.) ;
#42459=EDGE_CURVE('',#35193,#35162,#297,.T.) ;
#42460=EDGE_CURVE('',#34913,#35193,#28941,.T.) ;
#42461=EDGE_CURVE('',#35158,#34916,#28942,.T.) ;
#42462=EDGE_CURVE('',#35196,#35158,#2048,.T.) ;
#42463=EDGE_CURVE('',#35182,#35198,#28943,.T.) ;
#42464=EDGE_CURVE('',#35161,#35171,#28944,.T.) ;
#42465=EDGE_CURVE('',#35194,#35161,#28945,.T.) ;
#42466=EDGE_CURVE('',#34914,#35192,#28946,.T.) ;
#42467=EDGE_CURVE('',#35159,#34915,#28947,.T.) ;
#42468=EDGE_CURVE('',#35197,#35157,#28948,.T.) ;
#42469=EDGE_CURVE('',#35183,#35197,#28949,.T.) ;
#42470=EDGE_CURVE('',#35194,#35171,#28950,.T.) ;
#42471=EDGE_CURVE('',#35159,#35192,#298,.T.) ;
#42472=EDGE_CURVE('',#35183,#35157,#28951,.T.) ;
#42473=EDGE_CURVE('',#35169,#35188,#28952,.T.) ;
#42474=EDGE_CURVE('',#35189,#35170,#28953,.T.) ;
#42475=EDGE_CURVE('',#35160,#35191,#28954,.T.) ;
#42476=EDGE_CURVE('',#35184,#35160,#28955,.T.) ;
#42477=EDGE_CURVE('',#35189,#35188,#299,.T.) ;
#42478=EDGE_CURVE('',#35184,#35191,#28956,.T.) ;
#42479=EDGE_CURVE('',#35190,#35187,#300,.T.) ;
#42480=EDGE_CURVE('',#35180,#35190,#28957,.T.) ;
#42481=EDGE_CURVE('',#35179,#35187,#28958,.T.) ;
#42482=EDGE_CURVE('',#35152,#35292,#301,.T.) ;
#42483=EDGE_CURVE('',#35292,#34717,#2049,.T.) ;
#42484=EDGE_CURVE('',#35277,#35279,#28959,.T.) ;
#42485=EDGE_CURVE('',#35278,#35280,#28960,.T.) ;
#42486=EDGE_CURVE('',#34854,#35278,#28961,.T.) ;
#42487=EDGE_CURVE('',#34868,#35282,#2050,.T.) ;
#42488=EDGE_CURVE('',#34715,#34869,#2051,.T.) ;
#42489=EDGE_CURVE('',#35284,#34733,#28962,.T.) ;
#42490=EDGE_CURVE('',#35279,#35285,#28963,.T.) ;
#42491=EDGE_CURVE('',#34855,#35280,#28964,.T.) ;
#42492=EDGE_CURVE('',#35293,#35294,#2052,.T.) ;
#42493=EDGE_CURVE('',#35294,#34840,#302,.T.) ;
#42494=EDGE_CURVE('',#35281,#35293,#28965,.T.) ;
#42495=EDGE_CURVE('',#35268,#35273,#28966,.T.) ;
#42496=EDGE_CURVE('',#35273,#35267,#28967,.T.) ;
#42497=EDGE_CURVE('',#35274,#35266,#28968,.T.) ;
#42498=EDGE_CURVE('',#35269,#35276,#28969,.T.) ;
#42499=EDGE_CURVE('',#35274,#35265,#28970,.T.) ;
#42500=EDGE_CURVE('',#35270,#35276,#28971,.T.) ;
#42501=EDGE_CURVE('',#35275,#35272,#28972,.T.) ;
#42502=EDGE_CURVE('',#35271,#35275,#28973,.T.) ;
#42503=EDGE_CURVE('',#34935,#35204,#28974,.T.) ;
#42504=EDGE_CURVE('',#35201,#34934,#28975,.T.) ;
#42505=EDGE_CURVE('',#35216,#34933,#28976,.T.) ;
#42506=EDGE_CURVE('',#35201,#35216,#28977,.T.) ;
#42507=EDGE_CURVE('',#35208,#35204,#28978,.T.) ;
#42508=EDGE_CURVE('',#34936,#35208,#28979,.T.) ;
#42509=EDGE_CURVE('',#35213,#34932,#28980,.T.) ;
#42510=EDGE_CURVE('',#35202,#35215,#28981,.T.) ;
#42511=EDGE_CURVE('',#35203,#35220,#28982,.T.) ;
#42512=EDGE_CURVE('',#35217,#35202,#28983,.T.) ;
#42513=EDGE_CURVE('',#35205,#35203,#28984,.T.) ;
#42514=EDGE_CURVE('',#34930,#35207,#28985,.T.) ;
#42515=EDGE_CURVE('',#34931,#35211,#28986,.T.) ;
#42516=EDGE_CURVE('',#35212,#34929,#28987,.T.) ;
#42517=EDGE_CURVE('',#35213,#35211,#28988,.T.) ;
#42518=EDGE_CURVE('',#35217,#35215,#28989,.T.) ;
#42519=EDGE_CURVE('',#35205,#35220,#28990,.T.) ;
#42520=EDGE_CURVE('',#35212,#35207,#28991,.T.) ;
#42521=EDGE_CURVE('',#35214,#35210,#28992,.T.) ;
#42522=EDGE_CURVE('',#35218,#35214,#28993,.T.) ;
#42523=EDGE_CURVE('',#35206,#35219,#28994,.T.) ;
#42524=EDGE_CURVE('',#35209,#35206,#28995,.T.) ;
#42525=EDGE_CURVE('',#35218,#35210,#28996,.T.) ;
#42526=EDGE_CURVE('',#35209,#35219,#28997,.T.) ;
#42527=EDGE_CURVE('',#34887,#35248,#28998,.T.) ;
#42528=EDGE_CURVE('',#35245,#34886,#28999,.T.) ;
#42529=EDGE_CURVE('',#35244,#34885,#29000,.T.) ;
#42530=EDGE_CURVE('',#35245,#35244,#29001,.T.) ;
#42531=EDGE_CURVE('',#35252,#35248,#29002,.T.) ;
#42532=EDGE_CURVE('',#34888,#35252,#29003,.T.) ;
#42533=EDGE_CURVE('',#35241,#34884,#29004,.T.) ;
#42534=EDGE_CURVE('',#35246,#35243,#29005,.T.) ;
#42535=EDGE_CURVE('',#35247,#35256,#29006,.T.) ;
#42536=EDGE_CURVE('',#35253,#35246,#29007,.T.) ;
#42537=EDGE_CURVE('',#35249,#35247,#29008,.T.) ;
#42538=EDGE_CURVE('',#34882,#35251,#29009,.T.) ;
#42539=EDGE_CURVE('',#34883,#35239,#29010,.T.) ;
#42540=EDGE_CURVE('',#35240,#34881,#29011,.T.) ;
#42541=EDGE_CURVE('',#35241,#35239,#29012,.T.) ;
#42542=EDGE_CURVE('',#35253,#35243,#29013,.T.) ;
#42543=EDGE_CURVE('',#35249,#35256,#29014,.T.) ;
#42544=EDGE_CURVE('',#35240,#35251,#29015,.T.) ;
#42545=EDGE_CURVE('',#35242,#35238,#29016,.T.) ;
#42546=EDGE_CURVE('',#35254,#35242,#29017,.T.) ;
#42547=EDGE_CURVE('',#35250,#35255,#29018,.T.) ;
#42548=EDGE_CURVE('',#35237,#35250,#29019,.T.) ;
#42549=EDGE_CURVE('',#35254,#35238,#29020,.T.) ;
#42550=EDGE_CURVE('',#35237,#35255,#29021,.T.) ;
#42551=EDGE_CURVE('',#34834,#35287,#2053,.T.) ;
#42552=EDGE_CURVE('',#34835,#35286,#29022,.T.) ;
#42553=EDGE_CURVE('',#34969,#35286,#29023,.T.) ;
#42554=EDGE_CURVE('',#34970,#35291,#29024,.T.) ;
#42555=EDGE_CURVE('',#34849,#35291,#29025,.T.) ;
#42556=EDGE_CURVE('',#34850,#35290,#29026,.T.) ;
#42557=EDGE_CURVE('',#35153,#34851,#29027,.T.) ;
#42558=EDGE_CURVE('',#35153,#35290,#29028,.T.) ;
#42559=EDGE_CURVE('',#35154,#35289,#29029,.T.) ;
#42560=EDGE_CURVE('',#35146,#35154,#29030,.T.) ;
#42561=EDGE_CURVE('',#35146,#35289,#29031,.T.) ;
#42562=EDGE_CURVE('',#35288,#35147,#2054,.T.) ;
#42563=EDGE_CURVE('',#34734,#35284,#29032,.T.) ;
#42564=EDGE_CURVE('',#35281,#35283,#29033,.T.) ;
#42565=EDGE_CURVE('',#35293,#35282,#29034,.T.) ;
#42566=EDGE_CURVE('',#35294,#34868,#29035,.T.) ;
#42567=EDGE_CURVE('',#35152,#34870,#29036,.T.) ;
#42568=EDGE_CURVE('',#35292,#34869,#29037,.T.) ;
#42569=EDGE_CURVE('',#35277,#35285,#29038,.T.) ;
#42570=EDGE_CURVE('',#35295,#35296,#2055,.T.) ;
#42571=EDGE_CURVE('',#35296,#35288,#2056,.T.) ;
#42572=EDGE_CURVE('',#35287,#35297,#2057,.T.) ;
#42573=EDGE_CURVE('',#35297,#35295,#2058,.T.) ;
#42574=EDGE_CURVE('',#34961,#35287,#2059,.T.) ;
#42575=EDGE_CURVE('',#34958,#35147,#29039,.T.) ;
#42576=EDGE_CURVE('',#35288,#34959,#2060,.T.) ;
#42577=EDGE_CURVE('',#35297,#34961,#29040,.T.) ;
#42578=EDGE_CURVE('',#35295,#34960,#29041,.T.) ;
#42579=EDGE_CURVE('',#35296,#34959,#29042,.T.) ;
#42580=EDGE_CURVE('',#35119,#35137,#29043,.T.) ;
#42581=EDGE_CURVE('',#35137,#35121,#29044,.T.) ;
#42582=EDGE_CURVE('',#35120,#35139,#29045,.T.) ;
#42583=EDGE_CURVE('',#35139,#35118,#29046,.T.) ;
#42584=EDGE_CURVE('',#35138,#35123,#29047,.T.) ;
#42585=EDGE_CURVE('',#35117,#35136,#29048,.T.) ;
#42586=EDGE_CURVE('',#35140,#35116,#29049,.T.) ;
#42587=EDGE_CURVE('',#35122,#35145,#29050,.T.) ;
#42588=EDGE_CURVE('',#35138,#35125,#29051,.T.) ;
#42589=EDGE_CURVE('',#35115,#35136,#29052,.T.) ;
#42590=EDGE_CURVE('',#35140,#35114,#29053,.T.) ;
#42591=EDGE_CURVE('',#35124,#35145,#29054,.T.) ;
#42592=EDGE_CURVE('',#35132,#35127,#29055,.T.) ;
#42593=EDGE_CURVE('',#35112,#35135,#2061,.T.) ;
#42594=EDGE_CURVE('',#35113,#34809,#29056,.T.) ;
#42595=EDGE_CURVE('',#34810,#35112,#29057,.T.) ;
#42596=EDGE_CURVE('',#35141,#35113,#2062,.T.) ;
#42597=EDGE_CURVE('',#35126,#35144,#29058,.T.) ;
#42598=EDGE_CURVE('',#35133,#35129,#29059,.T.) ;
#42599=EDGE_CURVE('',#34811,#35135,#29060,.T.) ;
#42600=EDGE_CURVE('',#35141,#34808,#29061,.T.) ;
#42601=EDGE_CURVE('',#35128,#35143,#29062,.T.) ;
#42602=EDGE_CURVE('',#35134,#35131,#29063,.T.) ;
#42603=EDGE_CURVE('',#34812,#35134,#29064,.T.) ;
#42604=EDGE_CURVE('',#35142,#34806,#29065,.T.) ;
#42605=EDGE_CURVE('',#35130,#35142,#29066,.T.) ;
#42606=EDGE_CURVE('',#34813,#35131,#29067,.T.) ;
#42607=EDGE_CURVE('',#35130,#34807,#29068,.T.) ;
#42608=EDGE_CURVE('',#35298,#35299,#29069,.T.) ;
#42609=EDGE_CURVE('',#35300,#35298,#29070,.T.) ;
#42610=EDGE_CURVE('',#35301,#35300,#29071,.T.) ;
#42611=EDGE_CURVE('',#35301,#35299,#29072,.T.) ;
#42612=EDGE_CURVE('',#35302,#35302,#29073,.T.) ;
#42613=EDGE_CURVE('',#35302,#35303,#29074,.T.) ;
#42614=EDGE_CURVE('',#35304,#35303,#29075,.T.) ;
#42615=EDGE_CURVE('',#35303,#35304,#29076,.T.) ;
#42616=EDGE_CURVE('',#35305,#35305,#29077,.T.) ;
#42617=EDGE_CURVE('',#35305,#35306,#29078,.T.) ;
#42618=EDGE_CURVE('',#35306,#35306,#29079,.T.) ;
#42619=EDGE_CURVE('',#35307,#35307,#29080,.T.) ;
#42620=EDGE_CURVE('',#35307,#35308,#29081,.T.) ;
#42621=EDGE_CURVE('',#35309,#35308,#29082,.T.) ;
#42622=EDGE_CURVE('',#35308,#35309,#29083,.T.) ;
#42623=EDGE_CURVE('',#35310,#35311,#29084,.T.) ;
#42624=EDGE_CURVE('',#35312,#35311,#29085,.T.) ;
#42625=EDGE_CURVE('',#35312,#35313,#29086,.T.) ;
#42626=EDGE_CURVE('',#35313,#35310,#29087,.T.) ;
#42627=EDGE_CURVE('',#35314,#35315,#29088,.T.) ;
#42628=EDGE_CURVE('',#35315,#35316,#29089,.T.) ;
#42629=EDGE_CURVE('',#35314,#35316,#29090,.T.) ;
#42630=EDGE_CURVE('',#35317,#35310,#2902,.T.) ;
#42631=EDGE_CURVE('',#35317,#35318,#29091,.T.) ;
#42632=EDGE_CURVE('',#35311,#35318,#2903,.T.) ;
#42633=EDGE_CURVE('',#35319,#35320,#29092,.T.) ;
#42634=EDGE_CURVE('',#35319,#35321,#29093,.T.) ;
#42635=EDGE_CURVE('',#35320,#35321,#29094,.T.) ;
#42636=EDGE_CURVE('',#35322,#35322,#29095,.T.) ;
#42637=EDGE_CURVE('',#35322,#35305,#2904,.T.) ;
#42638=EDGE_CURVE('',#35306,#35309,#2905,.T.) ;
#42639=EDGE_CURVE('',#35323,#35324,#29096,.T.) ;
#42640=EDGE_CURVE('',#35323,#35325,#2063,.T.) ;
#42641=EDGE_CURVE('',#35326,#35325,#2906,.T.) ;
#42642=EDGE_CURVE('',#35326,#35327,#2064,.T.) ;
#42643=EDGE_CURVE('',#35328,#35327,#29097,.T.) ;
#42644=EDGE_CURVE('',#35328,#35329,#2065,.T.) ;
#42645=EDGE_CURVE('',#35329,#35330,#2907,.T.) ;
#42646=EDGE_CURVE('',#35330,#35331,#2066,.T.) ;
#42647=EDGE_CURVE('',#35332,#35331,#29098,.T.) ;
#42648=EDGE_CURVE('',#35332,#35333,#2067,.T.) ;
#42649=EDGE_CURVE('',#35334,#35333,#2908,.T.) ;
#42650=EDGE_CURVE('',#35334,#35335,#2068,.T.) ;
#42651=EDGE_CURVE('',#35336,#35335,#29099,.T.) ;
#42652=EDGE_CURVE('',#35336,#35337,#2069,.T.) ;
#42653=EDGE_CURVE('',#35337,#35338,#2909,.T.) ;
#42654=EDGE_CURVE('',#35338,#35339,#2070,.T.) ;
#42655=EDGE_CURVE('',#35324,#35339,#29100,.T.) ;
#42656=EDGE_CURVE('',#35324,#35304,#2910,.T.) ;
#42657=EDGE_CURVE('',#35340,#35341,#29101,.T.) ;
#42658=EDGE_CURVE('',#35342,#35340,#29102,.T.) ;
#42659=EDGE_CURVE('',#35343,#35342,#29103,.T.) ;
#42660=EDGE_CURVE('',#35343,#35341,#29104,.T.) ;
#42661=EDGE_CURVE('',#35344,#35345,#29105,.T.) ;
#42662=EDGE_CURVE('',#35346,#35344,#2911,.T.) ;
#42663=EDGE_CURVE('',#35347,#35346,#29106,.T.) ;
#42664=EDGE_CURVE('',#35345,#35347,#2912,.T.) ;
#42665=EDGE_CURVE('',#35348,#35348,#29107,.T.) ;
#42666=EDGE_CURVE('',#35348,#35349,#29108,.T.) ;
#42667=EDGE_CURVE('',#35350,#35349,#29109,.T.) ;
#42668=EDGE_CURVE('',#35349,#35350,#29110,.T.) ;
#42669=EDGE_CURVE('',#35351,#35351,#29111,.T.) ;
#42670=EDGE_CURVE('',#35351,#35352,#29112,.T.) ;
#42671=EDGE_CURVE('',#35352,#35352,#29113,.T.) ;
#42672=EDGE_CURVE('',#35353,#35353,#29114,.T.) ;
#42673=EDGE_CURVE('',#35353,#35354,#29115,.T.) ;
#42674=EDGE_CURVE('',#35355,#35354,#29116,.T.) ;
#42675=EDGE_CURVE('',#35354,#35355,#29117,.T.) ;
#42676=EDGE_CURVE('',#35356,#35357,#29118,.T.) ;
#42677=EDGE_CURVE('',#35358,#35357,#29119,.T.) ;
#42678=EDGE_CURVE('',#35358,#35359,#29120,.T.) ;
#42679=EDGE_CURVE('',#35359,#35356,#29121,.T.) ;
#42680=EDGE_CURVE('',#35360,#35361,#29122,.T.) ;
#42681=EDGE_CURVE('',#35361,#35362,#29123,.T.) ;
#42682=EDGE_CURVE('',#35360,#35362,#29124,.T.) ;
#42683=EDGE_CURVE('',#35363,#35356,#2913,.T.) ;
#42684=EDGE_CURVE('',#35363,#35364,#29125,.T.) ;
#42685=EDGE_CURVE('',#35357,#35364,#2914,.T.) ;
#42686=EDGE_CURVE('',#35365,#35366,#29126,.T.) ;
#42687=EDGE_CURVE('',#35365,#35367,#29127,.T.) ;
#42688=EDGE_CURVE('',#35366,#35367,#29128,.T.) ;
#42689=EDGE_CURVE('',#35368,#35368,#29129,.T.) ;
#42690=EDGE_CURVE('',#35368,#35351,#2915,.T.) ;
#42691=EDGE_CURVE('',#35352,#35355,#2916,.T.) ;
#42692=EDGE_CURVE('',#35369,#35370,#29130,.T.) ;
#42693=EDGE_CURVE('',#35369,#35371,#2071,.T.) ;
#42694=EDGE_CURVE('',#35372,#35371,#2917,.T.) ;
#42695=EDGE_CURVE('',#35372,#35373,#2072,.T.) ;
#42696=EDGE_CURVE('',#35374,#35373,#29131,.T.) ;
#42697=EDGE_CURVE('',#35374,#35375,#2073,.T.) ;
#42698=EDGE_CURVE('',#35375,#35376,#2918,.T.) ;
#42699=EDGE_CURVE('',#35376,#35377,#2074,.T.) ;
#42700=EDGE_CURVE('',#35378,#35377,#29132,.T.) ;
#42701=EDGE_CURVE('',#35378,#35379,#2075,.T.) ;
#42702=EDGE_CURVE('',#35380,#35379,#2919,.T.) ;
#42703=EDGE_CURVE('',#35380,#35381,#2076,.T.) ;
#42704=EDGE_CURVE('',#35382,#35381,#29133,.T.) ;
#42705=EDGE_CURVE('',#35382,#35383,#2077,.T.) ;
#42706=EDGE_CURVE('',#35383,#35384,#2920,.T.) ;
#42707=EDGE_CURVE('',#35384,#35385,#2078,.T.) ;
#42708=EDGE_CURVE('',#35370,#35385,#29134,.T.) ;
#42709=EDGE_CURVE('',#35370,#35350,#2921,.T.) ;
#42710=EDGE_CURVE('',#35386,#35387,#2922,.T.) ;
#42711=EDGE_CURVE('',#35388,#35387,#2923,.T.) ;
#42712=EDGE_CURVE('',#35388,#35389,#2924,.T.) ;
#42713=EDGE_CURVE('',#35389,#35386,#2925,.T.) ;
#42714=EDGE_CURVE('',#35390,#35391,#29135,.T.) ;
#42715=EDGE_CURVE('',#35390,#35392,#2926,.T.) ;
#42716=EDGE_CURVE('',#35393,#35392,#2079,.T.) ;
#42717=EDGE_CURVE('',#35393,#35394,#2927,.T.) ;
#42718=EDGE_CURVE('',#35395,#35394,#2080,.T.) ;
#42719=EDGE_CURVE('',#35395,#35396,#2928,.T.) ;
#42720=EDGE_CURVE('',#35397,#35396,#29136,.T.) ;
#42721=EDGE_CURVE('',#35397,#35391,#2929,.T.) ;
#42722=EDGE_CURVE('',#35398,#35399,#2930,.T.) ;
#42723=EDGE_CURVE('',#35398,#35400,#2931,.T.) ;
#42724=EDGE_CURVE('',#35401,#35400,#2932,.T.) ;
#42725=EDGE_CURVE('',#35401,#35399,#2933,.T.) ;
#42726=EDGE_CURVE('',#35402,#35403,#2934,.T.) ;
#42727=EDGE_CURVE('',#35402,#35404,#2935,.T.) ;
#42728=EDGE_CURVE('',#35405,#35404,#2936,.T.) ;
#42729=EDGE_CURVE('',#35405,#35403,#2937,.T.) ;
#42730=EDGE_CURVE('',#35406,#35407,#2938,.T.) ;
#42731=EDGE_CURVE('',#35406,#35408,#2939,.T.) ;
#42732=EDGE_CURVE('',#35409,#35408,#2940,.T.) ;
#42733=EDGE_CURVE('',#35409,#35407,#2941,.T.) ;
#42734=EDGE_CURVE('',#35406,#35410,#29137,.T.) ;
#42735=EDGE_CURVE('',#35411,#35410,#2942,.T.) ;
#42736=EDGE_CURVE('',#35408,#35411,#29138,.T.) ;
#42737=EDGE_CURVE('',#35407,#35402,#29139,.T.) ;
#42738=EDGE_CURVE('',#35404,#35409,#29140,.T.) ;
#42739=EDGE_CURVE('',#35403,#35398,#29141,.T.) ;
#42740=EDGE_CURVE('',#35400,#35405,#29142,.T.) ;
#42741=EDGE_CURVE('',#35412,#35413,#29143,.T.) ;
#42742=EDGE_CURVE('',#35412,#35414,#2943,.T.) ;
#42743=EDGE_CURVE('',#35414,#35399,#29144,.T.) ;
#42744=EDGE_CURVE('',#35415,#35401,#29145,.T.) ;
#42745=EDGE_CURVE('',#35413,#35415,#2944,.T.) ;
#42746=EDGE_CURVE('',#35416,#35417,#29146,.T.) ;
#42747=EDGE_CURVE('',#35417,#35418,#2945,.T.) ;
#42748=EDGE_CURVE('',#35418,#35419,#2946,.T.) ;
#42749=EDGE_CURVE('',#35419,#35416,#2947,.T.) ;
#42750=EDGE_CURVE('',#35420,#35421,#2948,.T.) ;
#42751=EDGE_CURVE('',#35421,#35422,#2949,.T.) ;
#42752=EDGE_CURVE('',#35422,#35423,#2950,.T.) ;
#42753=EDGE_CURVE('',#35423,#35420,#2951,.T.) ;
#42754=EDGE_CURVE('',#35424,#35425,#2952,.T.) ;
#42755=EDGE_CURVE('',#35425,#35426,#2953,.T.) ;
#42756=EDGE_CURVE('',#35426,#35367,#2954,.T.) ;
#42757=EDGE_CURVE('',#35367,#35424,#2955,.T.) ;
#42758=EDGE_CURVE('',#35385,#35369,#2956,.T.) ;
#42759=EDGE_CURVE('',#35358,#35362,#2957,.T.) ;
#42760=EDGE_CURVE('',#35362,#35319,#2958,.T.) ;
#42761=EDGE_CURVE('',#35319,#35427,#2959,.T.) ;
#42762=EDGE_CURVE('',#35428,#35427,#29147,.T.) ;
#42763=EDGE_CURVE('',#35428,#35313,#2960,.T.) ;
#42764=EDGE_CURVE('',#35312,#35316,#2961,.T.) ;
#42765=EDGE_CURVE('',#35316,#35429,#2962,.T.) ;
#42766=EDGE_CURVE('',#35430,#35429,#2963,.T.) ;
#42767=EDGE_CURVE('',#35430,#35431,#2964,.T.) ;
#42768=EDGE_CURVE('',#35432,#35431,#29148,.T.) ;
#42769=EDGE_CURVE('',#35432,#35433,#29149,.T.) ;
#42770=EDGE_CURVE('',#35434,#35433,#29150,.T.) ;
#42771=EDGE_CURVE('',#35434,#35435,#2965,.T.) ;
#42772=EDGE_CURVE('',#35436,#35435,#29151,.T.) ;
#42773=EDGE_CURVE('',#35436,#35437,#29152,.T.) ;
#42774=EDGE_CURVE('',#35438,#35437,#29153,.T.) ;
#42775=EDGE_CURVE('',#35438,#35439,#2966,.T.) ;
#42776=EDGE_CURVE('',#35439,#35440,#2967,.T.) ;
#42777=EDGE_CURVE('',#35440,#35365,#2968,.T.) ;
#42778=EDGE_CURVE('',#35365,#35441,#2969,.T.) ;
#42779=EDGE_CURVE('',#35442,#35441,#29154,.T.) ;
#42780=EDGE_CURVE('',#35442,#35359,#2970,.T.) ;
#42781=EDGE_CURVE('',#35361,#35443,#2971,.T.) ;
#42782=EDGE_CURVE('',#35443,#35444,#2972,.T.) ;
#42783=EDGE_CURVE('',#35444,#35321,#2973,.T.) ;
#42784=EDGE_CURVE('',#35321,#35361,#2974,.T.) ;
#42785=EDGE_CURVE('',#35445,#35446,#2975,.T.) ;
#42786=EDGE_CURVE('',#35447,#35446,#2976,.T.) ;
#42787=EDGE_CURVE('',#35447,#35448,#2977,.T.) ;
#42788=EDGE_CURVE('',#35448,#35449,#303,.T.) ;
#42789=EDGE_CURVE('',#35449,#35450,#2978,.T.) ;
#42790=EDGE_CURVE('',#35450,#35451,#304,.T.) ;
#42791=EDGE_CURVE('',#35451,#35452,#2979,.T.) ;
#42792=EDGE_CURVE('',#35452,#35453,#305,.T.) ;
#42793=EDGE_CURVE('',#35453,#35454,#2980,.T.) ;
#42794=EDGE_CURVE('',#35454,#35455,#306,.T.) ;
#42795=EDGE_CURVE('',#35455,#35456,#2981,.T.) ;
#42796=EDGE_CURVE('',#35456,#35445,#2982,.T.) ;
#42797=EDGE_CURVE('',#35457,#35413,#2983,.T.) ;
#42798=EDGE_CURVE('',#35458,#35415,#2984,.T.) ;
#42799=EDGE_CURVE('',#35458,#35457,#2985,.T.) ;
#42800=EDGE_CURVE('',#35412,#35459,#2986,.T.) ;
#42801=EDGE_CURVE('',#35459,#35460,#2987,.T.) ;
#42802=EDGE_CURVE('',#35411,#35460,#2988,.T.) ;
#42803=EDGE_CURVE('',#35414,#35410,#2989,.T.) ;
#42804=EDGE_CURVE('',#35461,#35462,#2990,.T.) ;
#42805=EDGE_CURVE('',#35462,#35463,#2991,.T.) ;
#42806=EDGE_CURVE('',#35464,#35463,#2992,.T.) ;
#42807=EDGE_CURVE('',#35464,#35461,#2993,.T.) ;
#42808=EDGE_CURVE('',#35465,#35466,#29155,.T.) ;
#42809=EDGE_CURVE('',#35465,#35467,#2994,.T.) ;
#42810=EDGE_CURVE('',#35468,#35467,#29156,.T.) ;
#42811=EDGE_CURVE('',#35468,#35469,#2995,.T.) ;
#42812=EDGE_CURVE('',#35470,#35469,#29157,.T.) ;
#42813=EDGE_CURVE('',#35470,#35471,#2996,.T.) ;
#42814=EDGE_CURVE('',#35472,#35471,#29158,.T.) ;
#42815=EDGE_CURVE('',#35472,#35466,#2997,.T.) ;
#42816=EDGE_CURVE('',#35473,#35474,#29159,.T.) ;
#42817=EDGE_CURVE('',#35473,#35475,#2998,.T.) ;
#42818=EDGE_CURVE('',#35476,#35475,#29160,.T.) ;
#42819=EDGE_CURVE('',#35476,#35477,#2999,.T.) ;
#42820=EDGE_CURVE('',#35478,#35477,#29161,.T.) ;
#42821=EDGE_CURVE('',#35478,#35479,#3000,.T.) ;
#42822=EDGE_CURVE('',#35480,#35479,#29162,.T.) ;
#42823=EDGE_CURVE('',#35480,#35474,#3001,.T.) ;
#42824=EDGE_CURVE('',#35481,#35482,#3002,.T.) ;
#42825=EDGE_CURVE('',#35482,#35483,#3003,.T.) ;
#42826=EDGE_CURVE('',#35484,#35483,#3004,.T.) ;
#42827=EDGE_CURVE('',#35484,#35481,#3005,.T.) ;
#42828=EDGE_CURVE('',#35485,#35345,#3006,.T.) ;
#42829=EDGE_CURVE('',#35486,#35347,#3007,.T.) ;
#42830=EDGE_CURVE('',#35486,#35485,#3008,.T.) ;
#42831=EDGE_CURVE('',#35344,#35487,#3009,.T.) ;
#42832=EDGE_CURVE('',#35487,#35488,#3010,.T.) ;
#42833=EDGE_CURVE('',#35346,#35488,#3011,.T.) ;
#42834=EDGE_CURVE('',#35489,#35490,#3012,.T.) ;
#42835=EDGE_CURVE('',#35490,#35491,#3013,.T.) ;
#42836=EDGE_CURVE('',#35492,#35491,#3014,.T.) ;
#42837=EDGE_CURVE('',#35492,#35489,#3015,.T.) ;
#42838=EDGE_CURVE('',#35493,#35494,#3016,.T.) ;
#42839=EDGE_CURVE('',#35494,#35495,#2081,.T.) ;
#42840=EDGE_CURVE('',#35495,#35496,#3017,.T.) ;
#42841=EDGE_CURVE('',#35497,#35496,#2082,.T.) ;
#42842=EDGE_CURVE('',#35497,#35498,#3018,.T.) ;
#42843=EDGE_CURVE('',#35499,#35498,#2083,.T.) ;
#42844=EDGE_CURVE('',#35499,#35500,#3019,.T.) ;
#42845=EDGE_CURVE('',#35500,#35493,#2084,.T.) ;
#42846=EDGE_CURVE('',#35501,#35502,#3020,.T.) ;
#42847=EDGE_CURVE('',#35502,#35503,#2085,.T.) ;
#42848=EDGE_CURVE('',#35503,#35504,#3021,.T.) ;
#42849=EDGE_CURVE('',#35505,#35504,#2086,.T.) ;
#42850=EDGE_CURVE('',#35505,#35506,#3022,.T.) ;
#42851=EDGE_CURVE('',#35507,#35506,#2087,.T.) ;
#42852=EDGE_CURVE('',#35507,#35508,#3023,.T.) ;
#42853=EDGE_CURVE('',#35508,#35501,#2088,.T.) ;
#42854=EDGE_CURVE('',#35509,#35510,#3024,.T.) ;
#42855=EDGE_CURVE('',#35510,#35511,#3025,.T.) ;
#42856=EDGE_CURVE('',#35512,#35511,#3026,.T.) ;
#42857=EDGE_CURVE('',#35512,#35509,#3027,.T.) ;
#42858=EDGE_CURVE('',#35513,#35514,#29163,.T.) ;
#42859=EDGE_CURVE('',#35513,#35515,#3028,.T.) ;
#42860=EDGE_CURVE('',#35516,#35515,#29164,.T.) ;
#42861=EDGE_CURVE('',#35516,#35517,#3029,.T.) ;
#42862=EDGE_CURVE('',#35518,#35517,#29165,.T.) ;
#42863=EDGE_CURVE('',#35518,#35519,#3030,.T.) ;
#42864=EDGE_CURVE('',#35520,#35519,#29166,.T.) ;
#42865=EDGE_CURVE('',#35520,#35514,#3031,.T.) ;
#42866=EDGE_CURVE('',#35521,#35522,#29167,.T.) ;
#42867=EDGE_CURVE('',#35521,#35523,#3032,.T.) ;
#42868=EDGE_CURVE('',#35524,#35523,#29168,.T.) ;
#42869=EDGE_CURVE('',#35524,#35525,#3033,.T.) ;
#42870=EDGE_CURVE('',#35526,#35525,#29169,.T.) ;
#42871=EDGE_CURVE('',#35526,#35527,#3034,.T.) ;
#42872=EDGE_CURVE('',#35528,#35527,#29170,.T.) ;
#42873=EDGE_CURVE('',#35528,#35522,#3035,.T.) ;
#42874=EDGE_CURVE('',#35529,#35530,#3036,.T.) ;
#42875=EDGE_CURVE('',#35530,#35531,#3037,.T.) ;
#42876=EDGE_CURVE('',#35532,#35531,#3038,.T.) ;
#42877=EDGE_CURVE('',#35532,#35529,#3039,.T.) ;
#42878=EDGE_CURVE('',#35533,#35534,#2089,.T.) ;
#42879=EDGE_CURVE('',#35534,#35535,#2090,.T.) ;
#42880=EDGE_CURVE('',#35535,#35536,#2091,.T.) ;
#42881=EDGE_CURVE('',#35536,#35537,#2092,.T.) ;
#42882=EDGE_CURVE('',#35537,#35538,#3040,.T.) ;
#42883=EDGE_CURVE('',#35538,#35539,#2093,.T.) ;
#42884=EDGE_CURVE('',#35539,#35540,#2094,.T.) ;
#42885=EDGE_CURVE('',#35540,#35541,#2095,.T.) ;
#42886=EDGE_CURVE('',#35541,#35542,#2096,.T.) ;
#42887=EDGE_CURVE('',#35542,#35543,#3041,.T.) ;
#42888=EDGE_CURVE('',#35544,#35543,#3042,.T.) ;
#42889=EDGE_CURVE('',#35544,#35545,#3043,.T.) ;
#42890=EDGE_CURVE('',#35545,#35546,#3044,.T.) ;
#42891=EDGE_CURVE('',#35546,#35533,#3045,.T.) ;
#42892=EDGE_CURVE('',#35547,#35548,#3046,.T.) ;
#42893=EDGE_CURVE('',#35548,#35549,#29171,.T.) ;
#42894=EDGE_CURVE('',#35549,#35550,#3047,.T.) ;
#42895=EDGE_CURVE('',#35550,#35547,#29172,.T.) ;
#42896=EDGE_CURVE('',#35551,#35552,#3048,.T.) ;
#42897=EDGE_CURVE('',#35552,#35553,#3049,.T.) ;
#42898=EDGE_CURVE('',#35553,#35554,#3050,.T.) ;
#42899=EDGE_CURVE('',#35554,#35551,#3051,.T.) ;
#42900=EDGE_CURVE('',#35461,#35459,#29173,.T.) ;
#42901=EDGE_CURVE('',#35457,#35386,#29174,.T.) ;
#42902=EDGE_CURVE('',#35389,#35445,#29175,.T.) ;
#42903=EDGE_CURVE('',#35456,#35425,#29176,.T.) ;
#42904=EDGE_CURVE('',#35424,#35440,#29177,.T.) ;
#42905=EDGE_CURVE('',#35439,#35554,#29178,.T.) ;
#42906=EDGE_CURVE('',#35553,#35419,#29179,.T.) ;
#42907=EDGE_CURVE('',#35418,#35546,#29180,.T.) ;
#42908=EDGE_CURVE('',#35545,#35530,#29181,.T.) ;
#42909=EDGE_CURVE('',#35529,#35510,#29182,.T.) ;
#42910=EDGE_CURVE('',#35509,#35490,#29183,.T.) ;
#42911=EDGE_CURVE('',#35489,#35487,#29184,.T.) ;
#42912=EDGE_CURVE('',#35485,#35482,#29185,.T.) ;
#42913=EDGE_CURVE('',#35481,#35462,#29186,.T.) ;
#42914=EDGE_CURVE('',#35555,#35556,#3052,.T.) ;
#42915=EDGE_CURVE('',#35556,#35557,#3053,.T.) ;
#42916=EDGE_CURVE('',#35557,#35558,#3054,.T.) ;
#42917=EDGE_CURVE('',#35558,#35555,#3055,.T.) ;
#42918=EDGE_CURVE('',#35559,#35560,#3056,.T.) ;
#42919=EDGE_CURVE('',#35560,#35561,#3057,.T.) ;
#42920=EDGE_CURVE('',#35561,#35562,#3058,.T.) ;
#42921=EDGE_CURVE('',#35562,#35559,#3059,.T.) ;
#42922=EDGE_CURVE('',#35563,#35564,#307,.T.) ;
#42923=EDGE_CURVE('',#35563,#35565,#3060,.T.) ;
#42924=EDGE_CURVE('',#35565,#35566,#3061,.T.) ;
#42925=EDGE_CURVE('',#35566,#35567,#3062,.T.) ;
#42926=EDGE_CURVE('',#35568,#35567,#308,.T.) ;
#42927=EDGE_CURVE('',#35568,#35569,#3063,.T.) ;
#42928=EDGE_CURVE('',#35569,#35570,#3064,.T.) ;
#42929=EDGE_CURVE('',#35570,#35564,#3065,.T.) ;
#42930=EDGE_CURVE('',#35571,#35572,#3066,.T.) ;
#42931=EDGE_CURVE('',#35572,#35573,#309,.T.) ;
#42932=EDGE_CURVE('',#35574,#35573,#3067,.T.) ;
#42933=EDGE_CURVE('',#35574,#35566,#310,.T.) ;
#42934=EDGE_CURVE('',#35565,#35575,#311,.T.) ;
#42935=EDGE_CURVE('',#35575,#35576,#3068,.T.) ;
#42936=EDGE_CURVE('',#35576,#35571,#312,.T.) ;
#42937=EDGE_CURVE('',#35577,#35578,#313,.T.) ;
#42938=EDGE_CURVE('',#35577,#35572,#3069,.T.) ;
#42939=EDGE_CURVE('',#35571,#35579,#3070,.T.) ;
#42940=EDGE_CURVE('',#35580,#35579,#314,.T.) ;
#42941=EDGE_CURVE('',#35580,#35581,#3071,.T.) ;
#42942=EDGE_CURVE('',#35581,#35582,#3072,.T.) ;
#42943=EDGE_CURVE('',#35582,#35578,#3073,.T.) ;
#42944=EDGE_CURVE('',#35575,#35583,#3074,.T.) ;
#42945=EDGE_CURVE('',#35583,#35584,#3075,.T.) ;
#42946=EDGE_CURVE('',#35584,#35576,#3076,.T.) ;
#42947=EDGE_CURVE('',#35573,#35585,#3077,.T.) ;
#42948=EDGE_CURVE('',#35585,#35586,#3078,.T.) ;
#42949=EDGE_CURVE('',#35586,#35574,#3079,.T.) ;
#42950=EDGE_CURVE('',#35587,#35588,#3080,.T.) ;
#42951=EDGE_CURVE('',#35588,#35589,#3081,.T.) ;
#42952=EDGE_CURVE('',#35589,#35590,#3082,.T.) ;
#42953=EDGE_CURVE('',#35590,#35591,#3083,.T.) ;
#42954=EDGE_CURVE('',#35591,#35592,#3084,.T.) ;
#42955=EDGE_CURVE('',#35592,#35587,#3085,.T.) ;
#42956=EDGE_CURVE('',#35593,#35594,#3086,.T.) ;
#42957=EDGE_CURVE('',#35594,#35595,#3087,.T.) ;
#42958=EDGE_CURVE('',#35595,#35596,#3088,.T.) ;
#42959=EDGE_CURVE('',#35596,#35597,#3089,.T.) ;
#42960=EDGE_CURVE('',#35597,#35598,#3090,.T.) ;
#42961=EDGE_CURVE('',#35598,#35593,#3091,.T.) ;
#42962=EDGE_CURVE('',#35599,#35600,#3092,.T.) ;
#42963=EDGE_CURVE('',#35600,#35601,#3093,.T.) ;
#42964=EDGE_CURVE('',#35601,#35602,#3094,.T.) ;
#42965=EDGE_CURVE('',#35602,#35599,#3095,.T.) ;
#42966=EDGE_CURVE('',#35603,#35604,#3096,.T.) ;
#42967=EDGE_CURVE('',#35604,#35605,#3097,.T.) ;
#42968=EDGE_CURVE('',#35605,#35606,#3098,.T.) ;
#42969=EDGE_CURVE('',#35606,#35603,#3099,.T.) ;
#42970=EDGE_CURVE('',#35607,#35608,#3100,.T.) ;
#42971=EDGE_CURVE('',#35608,#35609,#3101,.T.) ;
#42972=EDGE_CURVE('',#35609,#35610,#3102,.T.) ;
#42973=EDGE_CURVE('',#35610,#35607,#3103,.T.) ;
#42974=EDGE_CURVE('',#35611,#35612,#3104,.T.) ;
#42975=EDGE_CURVE('',#35612,#35613,#3105,.T.) ;
#42976=EDGE_CURVE('',#35613,#35614,#3106,.T.) ;
#42977=EDGE_CURVE('',#35614,#35611,#3107,.T.) ;
#42978=EDGE_CURVE('',#35615,#35616,#3108,.T.) ;
#42979=EDGE_CURVE('',#35616,#35617,#3109,.T.) ;
#42980=EDGE_CURVE('',#35617,#35618,#3110,.T.) ;
#42981=EDGE_CURVE('',#35618,#35615,#3111,.T.) ;
#42982=EDGE_CURVE('',#35619,#35620,#3112,.T.) ;
#42983=EDGE_CURVE('',#35621,#35619,#29187,.T.) ;
#42984=EDGE_CURVE('',#35622,#35621,#3113,.T.) ;
#42985=EDGE_CURVE('',#35623,#35622,#29188,.T.) ;
#42986=EDGE_CURVE('',#35624,#35623,#3114,.T.) ;
#42987=EDGE_CURVE('',#35625,#35624,#29189,.T.) ;
#42988=EDGE_CURVE('',#35626,#35625,#3115,.T.) ;
#42989=EDGE_CURVE('',#35620,#35626,#29190,.T.) ;
#42990=EDGE_CURVE('',#35627,#35628,#29191,.T.) ;
#42991=EDGE_CURVE('',#35620,#35627,#3116,.T.) ;
#42992=EDGE_CURVE('',#35626,#35628,#3117,.T.) ;
#42993=EDGE_CURVE('',#35629,#35627,#3118,.T.) ;
#42994=EDGE_CURVE('',#35619,#35629,#3119,.T.) ;
#42995=EDGE_CURVE('',#35630,#35629,#29192,.T.) ;
#42996=EDGE_CURVE('',#35621,#35630,#3120,.T.) ;
#42997=EDGE_CURVE('',#35631,#35630,#3121,.T.) ;
#42998=EDGE_CURVE('',#35622,#35631,#3122,.T.) ;
#42999=EDGE_CURVE('',#35632,#35631,#29193,.T.) ;
#43000=EDGE_CURVE('',#35623,#35632,#3123,.T.) ;
#43001=EDGE_CURVE('',#35633,#35632,#3124,.T.) ;
#43002=EDGE_CURVE('',#35624,#35633,#3125,.T.) ;
#43003=EDGE_CURVE('',#35634,#35633,#29194,.T.) ;
#43004=EDGE_CURVE('',#35625,#35634,#3126,.T.) ;
#43005=EDGE_CURVE('',#35628,#35634,#3127,.T.) ;
#43006=EDGE_CURVE('',#35377,#35378,#3128,.T.) ;
#43007=EDGE_CURVE('',#35375,#35380,#3129,.T.) ;
#43008=EDGE_CURVE('',#35379,#35376,#3130,.T.) ;
#43009=EDGE_CURVE('',#35383,#35372,#3131,.T.) ;
#43010=EDGE_CURVE('',#35371,#35384,#3132,.T.) ;
#43011=EDGE_CURVE('',#35373,#35382,#3133,.T.) ;
#43012=EDGE_CURVE('',#35381,#35374,#3134,.T.) ;
#43013=EDGE_CURVE('',#35635,#35636,#3135,.T.) ;
#43014=EDGE_CURVE('',#35636,#35637,#3136,.T.) ;
#43015=EDGE_CURVE('',#35637,#35638,#3137,.T.) ;
#43016=EDGE_CURVE('',#35638,#35635,#3138,.T.) ;
#43017=EDGE_CURVE('',#35639,#35640,#3139,.T.) ;
#43018=EDGE_CURVE('',#35640,#35641,#3140,.T.) ;
#43019=EDGE_CURVE('',#35641,#35642,#3141,.T.) ;
#43020=EDGE_CURVE('',#35642,#35639,#3142,.T.) ;
#43021=EDGE_CURVE('',#35643,#35644,#3143,.T.) ;
#43022=EDGE_CURVE('',#35644,#35645,#3144,.T.) ;
#43023=EDGE_CURVE('',#35645,#35646,#3145,.T.) ;
#43024=EDGE_CURVE('',#35646,#35643,#3146,.T.) ;
#43025=EDGE_CURVE('',#35647,#35648,#3147,.T.) ;
#43026=EDGE_CURVE('',#35648,#35649,#3148,.T.) ;
#43027=EDGE_CURVE('',#35649,#35650,#3149,.T.) ;
#43028=EDGE_CURVE('',#35650,#35647,#3150,.T.) ;
#43029=EDGE_CURVE('',#35651,#35652,#3151,.T.) ;
#43030=EDGE_CURVE('',#35652,#35653,#3152,.T.) ;
#43031=EDGE_CURVE('',#35653,#35654,#3153,.T.) ;
#43032=EDGE_CURVE('',#35654,#35651,#3154,.T.) ;
#43033=EDGE_CURVE('',#35655,#35656,#3155,.T.) ;
#43034=EDGE_CURVE('',#35657,#35655,#29195,.T.) ;
#43035=EDGE_CURVE('',#35658,#35657,#3156,.T.) ;
#43036=EDGE_CURVE('',#35659,#35658,#29196,.T.) ;
#43037=EDGE_CURVE('',#35660,#35659,#3157,.T.) ;
#43038=EDGE_CURVE('',#35661,#35660,#29197,.T.) ;
#43039=EDGE_CURVE('',#35662,#35661,#3158,.T.) ;
#43040=EDGE_CURVE('',#35656,#35662,#29198,.T.) ;
#43041=EDGE_CURVE('',#35662,#35663,#3159,.T.) ;
#43042=EDGE_CURVE('',#35663,#35664,#29199,.T.) ;
#43043=EDGE_CURVE('',#35656,#35664,#3160,.T.) ;
#43044=EDGE_CURVE('',#35664,#35665,#3161,.T.) ;
#43045=EDGE_CURVE('',#35655,#35665,#3162,.T.) ;
#43046=EDGE_CURVE('',#35665,#35666,#29200,.T.) ;
#43047=EDGE_CURVE('',#35657,#35666,#3163,.T.) ;
#43048=EDGE_CURVE('',#35666,#35667,#3164,.T.) ;
#43049=EDGE_CURVE('',#35658,#35667,#3165,.T.) ;
#43050=EDGE_CURVE('',#35667,#35668,#29201,.T.) ;
#43051=EDGE_CURVE('',#35659,#35668,#3166,.T.) ;
#43052=EDGE_CURVE('',#35668,#35669,#3167,.T.) ;
#43053=EDGE_CURVE('',#35660,#35669,#3168,.T.) ;
#43054=EDGE_CURVE('',#35669,#35670,#29202,.T.) ;
#43055=EDGE_CURVE('',#35661,#35670,#3169,.T.) ;
#43056=EDGE_CURVE('',#35670,#35663,#3170,.T.) ;
#43057=EDGE_CURVE('',#35671,#35672,#3171,.T.) ;
#43058=EDGE_CURVE('',#35672,#35673,#3172,.T.) ;
#43059=EDGE_CURVE('',#35673,#35674,#3173,.T.) ;
#43060=EDGE_CURVE('',#35674,#35671,#3174,.T.) ;
#43061=EDGE_CURVE('',#35366,#35342,#3175,.T.) ;
#43062=EDGE_CURVE('',#35342,#35675,#3176,.T.) ;
#43063=EDGE_CURVE('',#35675,#35676,#3177,.T.) ;
#43064=EDGE_CURVE('',#35676,#35366,#3178,.T.) ;
#43065=EDGE_CURVE('',#35677,#35363,#3179,.T.) ;
#43066=EDGE_CURVE('',#35356,#35678,#3180,.T.) ;
#43067=EDGE_CURVE('',#35678,#35677,#3181,.T.) ;
#43068=EDGE_CURVE('',#35364,#35679,#3182,.T.) ;
#43069=EDGE_CURVE('',#35679,#35360,#3183,.T.) ;
#43070=EDGE_CURVE('',#35360,#35357,#3184,.T.) ;
#43071=EDGE_CURVE('',#35341,#35680,#3185,.T.) ;
#43072=EDGE_CURVE('',#35680,#35681,#29203,.T.) ;
#43073=EDGE_CURVE('',#35681,#35682,#3186,.T.) ;
#43074=EDGE_CURVE('',#35682,#35683,#3187,.T.) ;
#43075=EDGE_CURVE('',#35683,#35340,#3188,.T.) ;
#43076=EDGE_CURVE('',#35684,#35685,#29204,.T.) ;
#43077=EDGE_CURVE('',#35685,#35686,#29205,.T.) ;
#43078=EDGE_CURVE('',#35686,#35687,#29206,.T.) ;
#43079=EDGE_CURVE('',#35687,#35688,#3189,.T.) ;
#43080=EDGE_CURVE('',#35688,#35689,#29207,.T.) ;
#43081=EDGE_CURVE('',#35689,#35684,#3190,.T.) ;
#43082=EDGE_CURVE('',#35593,#35502,#29208,.T.) ;
#43083=EDGE_CURVE('',#35561,#35593,#2097,.T.) ;
#43084=EDGE_CURVE('',#35503,#35561,#29209,.T.) ;
#43085=EDGE_CURVE('',#35583,#35563,#29210,.T.) ;
#43086=EDGE_CURVE('',#35597,#35564,#29211,.T.) ;
#43087=EDGE_CURVE('',#35583,#35597,#315,.T.) ;
#43088=EDGE_CURVE('',#35598,#35570,#29212,.T.) ;
#43089=EDGE_CURVE('',#35562,#35598,#29213,.T.) ;
#43090=EDGE_CURVE('',#35504,#35560,#29214,.T.) ;
#43091=EDGE_CURVE('',#35594,#35501,#29215,.T.) ;
#43092=EDGE_CURVE('',#35584,#35596,#316,.T.) ;
#43093=EDGE_CURVE('',#35579,#35584,#29216,.T.) ;
#43094=EDGE_CURVE('',#35562,#35570,#29217,.T.) ;
#43095=EDGE_CURVE('',#35591,#35560,#317,.T.) ;
#43096=EDGE_CURVE('',#35505,#35591,#29218,.T.) ;
#43097=EDGE_CURVE('',#35556,#35508,#29219,.T.) ;
#43098=EDGE_CURVE('',#35594,#35556,#2098,.T.) ;
#43099=EDGE_CURVE('',#35580,#35596,#29220,.T.) ;
#43100=EDGE_CURVE('',#35559,#35569,#29221,.T.) ;
#43101=EDGE_CURVE('',#35592,#35559,#29222,.T.) ;
#43102=EDGE_CURVE('',#35506,#35590,#29223,.T.) ;
#43103=EDGE_CURVE('',#35557,#35507,#29224,.T.) ;
#43104=EDGE_CURVE('',#35595,#35555,#29225,.T.) ;
#43105=EDGE_CURVE('',#35581,#35595,#29226,.T.) ;
#43106=EDGE_CURVE('',#35592,#35569,#29227,.T.) ;
#43107=EDGE_CURVE('',#35557,#35590,#318,.T.) ;
#43108=EDGE_CURVE('',#35581,#35555,#29228,.T.) ;
#43109=EDGE_CURVE('',#35567,#35586,#29229,.T.) ;
#43110=EDGE_CURVE('',#35587,#35568,#29230,.T.) ;
#43111=EDGE_CURVE('',#35558,#35589,#29231,.T.) ;
#43112=EDGE_CURVE('',#35582,#35558,#29232,.T.) ;
#43113=EDGE_CURVE('',#35587,#35586,#319,.T.) ;
#43114=EDGE_CURVE('',#35582,#35589,#29233,.T.) ;
#43115=EDGE_CURVE('',#35588,#35585,#320,.T.) ;
#43116=EDGE_CURVE('',#35578,#35588,#29234,.T.) ;
#43117=EDGE_CURVE('',#35577,#35585,#29235,.T.) ;
#43118=EDGE_CURVE('',#35426,#35690,#321,.T.) ;
#43119=EDGE_CURVE('',#35690,#35343,#2099,.T.) ;
#43120=EDGE_CURVE('',#35675,#35677,#29236,.T.) ;
#43121=EDGE_CURVE('',#35676,#35678,#29237,.T.) ;
#43122=EDGE_CURVE('',#35441,#35676,#29238,.T.) ;
#43123=EDGE_CURVE('',#35453,#35680,#2100,.T.) ;
#43124=EDGE_CURVE('',#35341,#35454,#2101,.T.) ;
#43125=EDGE_CURVE('',#35682,#35363,#29239,.T.) ;
#43126=EDGE_CURVE('',#35677,#35683,#29240,.T.) ;
#43127=EDGE_CURVE('',#35442,#35678,#29241,.T.) ;
#43128=EDGE_CURVE('',#35691,#35692,#2102,.T.) ;
#43129=EDGE_CURVE('',#35692,#35443,#322,.T.) ;
#43130=EDGE_CURVE('',#35679,#35691,#29242,.T.) ;
#43131=EDGE_CURVE('',#35666,#35671,#29243,.T.) ;
#43132=EDGE_CURVE('',#35671,#35665,#29244,.T.) ;
#43133=EDGE_CURVE('',#35672,#35664,#29245,.T.) ;
#43134=EDGE_CURVE('',#35667,#35674,#29246,.T.) ;
#43135=EDGE_CURVE('',#35672,#35663,#29247,.T.) ;
#43136=EDGE_CURVE('',#35668,#35674,#29248,.T.) ;
#43137=EDGE_CURVE('',#35673,#35670,#29249,.T.) ;
#43138=EDGE_CURVE('',#35669,#35673,#29250,.T.) ;
#43139=EDGE_CURVE('',#35527,#35602,#29251,.T.) ;
#43140=EDGE_CURVE('',#35599,#35526,#29252,.T.) ;
#43141=EDGE_CURVE('',#35614,#35525,#29253,.T.) ;
#43142=EDGE_CURVE('',#35599,#35614,#29254,.T.) ;
#43143=EDGE_CURVE('',#35606,#35602,#29255,.T.) ;
#43144=EDGE_CURVE('',#35528,#35606,#29256,.T.) ;
#43145=EDGE_CURVE('',#35611,#35524,#29257,.T.) ;
#43146=EDGE_CURVE('',#35600,#35613,#29258,.T.) ;
#43147=EDGE_CURVE('',#35601,#35618,#29259,.T.) ;
#43148=EDGE_CURVE('',#35615,#35600,#29260,.T.) ;
#43149=EDGE_CURVE('',#35603,#35601,#29261,.T.) ;
#43150=EDGE_CURVE('',#35522,#35605,#29262,.T.) ;
#43151=EDGE_CURVE('',#35523,#35609,#29263,.T.) ;
#43152=EDGE_CURVE('',#35610,#35521,#29264,.T.) ;
#43153=EDGE_CURVE('',#35611,#35609,#29265,.T.) ;
#43154=EDGE_CURVE('',#35615,#35613,#29266,.T.) ;
#43155=EDGE_CURVE('',#35603,#35618,#29267,.T.) ;
#43156=EDGE_CURVE('',#35610,#35605,#29268,.T.) ;
#43157=EDGE_CURVE('',#35612,#35608,#29269,.T.) ;
#43158=EDGE_CURVE('',#35616,#35612,#29270,.T.) ;
#43159=EDGE_CURVE('',#35604,#35617,#29271,.T.) ;
#43160=EDGE_CURVE('',#35607,#35604,#29272,.T.) ;
#43161=EDGE_CURVE('',#35616,#35608,#29273,.T.) ;
#43162=EDGE_CURVE('',#35607,#35617,#29274,.T.) ;
#43163=EDGE_CURVE('',#35479,#35646,#29275,.T.) ;
#43164=EDGE_CURVE('',#35643,#35478,#29276,.T.) ;
#43165=EDGE_CURVE('',#35642,#35477,#29277,.T.) ;
#43166=EDGE_CURVE('',#35643,#35642,#29278,.T.) ;
#43167=EDGE_CURVE('',#35650,#35646,#29279,.T.) ;
#43168=EDGE_CURVE('',#35480,#35650,#29280,.T.) ;
#43169=EDGE_CURVE('',#35639,#35476,#29281,.T.) ;
#43170=EDGE_CURVE('',#35644,#35641,#29282,.T.) ;
#43171=EDGE_CURVE('',#35645,#35654,#29283,.T.) ;
#43172=EDGE_CURVE('',#35651,#35644,#29284,.T.) ;
#43173=EDGE_CURVE('',#35647,#35645,#29285,.T.) ;
#43174=EDGE_CURVE('',#35474,#35649,#29286,.T.) ;
#43175=EDGE_CURVE('',#35475,#35637,#29287,.T.) ;
#43176=EDGE_CURVE('',#35638,#35473,#29288,.T.) ;
#43177=EDGE_CURVE('',#35639,#35637,#29289,.T.) ;
#43178=EDGE_CURVE('',#35651,#35641,#29290,.T.) ;
#43179=EDGE_CURVE('',#35647,#35654,#29291,.T.) ;
#43180=EDGE_CURVE('',#35638,#35649,#29292,.T.) ;
#43181=EDGE_CURVE('',#35640,#35636,#29293,.T.) ;
#43182=EDGE_CURVE('',#35652,#35640,#29294,.T.) ;
#43183=EDGE_CURVE('',#35648,#35653,#29295,.T.) ;
#43184=EDGE_CURVE('',#35635,#35648,#29296,.T.) ;
#43185=EDGE_CURVE('',#35652,#35636,#29297,.T.) ;
#43186=EDGE_CURVE('',#35635,#35653,#29298,.T.) ;
#43187=EDGE_CURVE('',#35550,#35685,#2103,.T.) ;
#43188=EDGE_CURVE('',#35547,#35684,#29299,.T.) ;
#43189=EDGE_CURVE('',#35548,#35422,#29300,.T.) ;
#43190=EDGE_CURVE('',#35423,#35547,#29301,.T.) ;
#43191=EDGE_CURVE('',#35423,#35684,#29302,.T.) ;
#43192=EDGE_CURVE('',#35420,#35689,#29303,.T.) ;
#43193=EDGE_CURVE('',#35421,#35434,#29304,.T.) ;
#43194=EDGE_CURVE('',#35435,#35420,#29305,.T.) ;
#43195=EDGE_CURVE('',#35436,#35689,#29306,.T.) ;
#43196=EDGE_CURVE('',#35437,#35688,#29307,.T.) ;
#43197=EDGE_CURVE('',#35551,#35438,#29308,.T.) ;
#43198=EDGE_CURVE('',#35551,#35688,#29309,.T.) ;
#43199=EDGE_CURVE('',#35552,#35687,#29310,.T.) ;
#43200=EDGE_CURVE('',#35416,#35552,#29311,.T.) ;
#43201=EDGE_CURVE('',#35416,#35687,#29312,.T.) ;
#43202=EDGE_CURVE('',#35686,#35417,#2104,.T.) ;
#43203=EDGE_CURVE('',#35531,#35544,#29313,.T.) ;
#43204=EDGE_CURVE('',#35511,#35532,#29314,.T.) ;
#43205=EDGE_CURVE('',#35491,#35512,#29315,.T.) ;
#43206=EDGE_CURVE('',#35488,#35492,#29316,.T.) ;
#43207=EDGE_CURVE('',#35483,#35486,#29317,.T.) ;
#43208=EDGE_CURVE('',#35463,#35484,#29318,.T.) ;
#43209=EDGE_CURVE('',#35460,#35464,#29319,.T.) ;
#43210=EDGE_CURVE('',#35387,#35458,#29320,.T.) ;
#43211=EDGE_CURVE('',#35446,#35388,#29321,.T.) ;
#43212=EDGE_CURVE('',#35364,#35682,#29322,.T.) ;
#43213=EDGE_CURVE('',#35679,#35681,#29323,.T.) ;
#43214=EDGE_CURVE('',#35691,#35680,#29324,.T.) ;
#43215=EDGE_CURVE('',#35692,#35453,#29325,.T.) ;
#43216=EDGE_CURVE('',#35443,#35452,#29326,.T.) ;
#43217=EDGE_CURVE('',#35444,#35451,#29327,.T.) ;
#43218=EDGE_CURVE('',#35426,#35455,#29328,.T.) ;
#43219=EDGE_CURVE('',#35690,#35454,#29329,.T.) ;
#43220=EDGE_CURVE('',#35675,#35683,#29330,.T.) ;
#43221=EDGE_CURVE('',#35693,#35694,#2105,.T.) ;
#43222=EDGE_CURVE('',#35694,#35686,#2106,.T.) ;
#43223=EDGE_CURVE('',#35685,#35695,#2107,.T.) ;
#43224=EDGE_CURVE('',#35695,#35693,#2108,.T.) ;
#43225=EDGE_CURVE('',#35538,#35549,#29331,.T.) ;
#43226=EDGE_CURVE('',#35550,#35537,#29332,.T.) ;
#43227=EDGE_CURVE('',#35536,#35685,#2109,.T.) ;
#43228=EDGE_CURVE('',#35533,#35417,#29333,.T.) ;
#43229=EDGE_CURVE('',#35686,#35534,#2110,.T.) ;
#43230=EDGE_CURVE('',#35695,#35536,#29334,.T.) ;
#43231=EDGE_CURVE('',#35693,#35535,#29335,.T.) ;
#43232=EDGE_CURVE('',#35694,#35534,#29336,.T.) ;
#43233=EDGE_CURVE('',#35696,#35697,#3191,.T.) ;
#43234=EDGE_CURVE('',#35697,#35698,#3192,.T.) ;
#43235=EDGE_CURVE('',#35699,#35698,#3193,.T.) ;
#43236=EDGE_CURVE('',#35699,#35696,#3194,.T.) ;
#43237=EDGE_CURVE('',#35698,#35700,#29337,.T.) ;
#43238=EDGE_CURVE('',#35701,#35700,#3195,.T.) ;
#43239=EDGE_CURVE('',#35701,#35699,#29338,.T.) ;
#43240=EDGE_CURVE('',#35700,#35702,#3196,.T.) ;
#43241=EDGE_CURVE('',#35703,#35702,#3197,.T.) ;
#43242=EDGE_CURVE('',#35703,#35701,#3198,.T.) ;
#43243=EDGE_CURVE('',#35702,#35704,#29339,.T.) ;
#43244=EDGE_CURVE('',#35705,#35704,#3199,.T.) ;
#43245=EDGE_CURVE('',#35705,#35703,#29340,.T.) ;
#43246=EDGE_CURVE('',#35704,#35706,#3200,.T.) ;
#43247=EDGE_CURVE('',#35707,#35706,#3201,.T.) ;
#43248=EDGE_CURVE('',#35707,#35705,#3202,.T.) ;
#43249=EDGE_CURVE('',#35706,#35708,#29341,.T.) ;
#43250=EDGE_CURVE('',#35709,#35708,#3203,.T.) ;
#43251=EDGE_CURVE('',#35709,#35707,#29342,.T.) ;
#43252=EDGE_CURVE('',#35708,#35710,#3204,.T.) ;
#43253=EDGE_CURVE('',#35711,#35710,#3205,.T.) ;
#43254=EDGE_CURVE('',#35711,#35709,#3206,.T.) ;
#43255=EDGE_CURVE('',#35710,#35712,#29343,.T.) ;
#43256=EDGE_CURVE('',#35713,#35712,#3207,.T.) ;
#43257=EDGE_CURVE('',#35713,#35711,#29344,.T.) ;
#43258=EDGE_CURVE('',#35712,#35714,#3208,.T.) ;
#43259=EDGE_CURVE('',#35714,#35715,#3209,.T.) ;
#43260=EDGE_CURVE('',#35715,#35713,#3210,.T.) ;
#43261=EDGE_CURVE('',#35716,#35717,#29345,.T.) ;
#43262=EDGE_CURVE('',#35717,#35718,#3211,.T.) ;
#43263=EDGE_CURVE('',#35718,#35719,#3212,.T.) ;
#43264=EDGE_CURVE('',#35719,#35720,#3213,.T.) ;
#43265=EDGE_CURVE('',#35720,#35721,#3214,.T.) ;
#43266=EDGE_CURVE('',#35721,#35722,#3215,.T.) ;
#43267=EDGE_CURVE('',#35722,#35716,#3216,.T.) ;
#43268=EDGE_CURVE('',#35723,#35724,#3217,.T.) ;
#43269=EDGE_CURVE('',#35724,#35725,#3218,.T.) ;
#43270=EDGE_CURVE('',#35725,#35726,#3219,.T.) ;
#43271=EDGE_CURVE('',#35726,#35727,#3220,.T.) ;
#43272=EDGE_CURVE('',#35727,#35728,#29346,.T.) ;
#43273=EDGE_CURVE('',#35728,#35729,#3221,.T.) ;
#43274=EDGE_CURVE('',#35729,#35723,#3222,.T.) ;
#43275=EDGE_CURVE('',#35730,#35731,#3223,.T.) ;
#43276=EDGE_CURVE('',#35730,#35732,#3224,.T.) ;
#43277=EDGE_CURVE('',#35732,#35733,#3225,.T.) ;
#43278=EDGE_CURVE('',#35733,#35731,#3226,.T.) ;
#43279=EDGE_CURVE('',#35339,#35323,#3227,.T.) ;
#43280=EDGE_CURVE('',#35315,#35734,#3228,.T.) ;
#43281=EDGE_CURVE('',#35734,#35735,#3229,.T.) ;
#43282=EDGE_CURVE('',#35736,#35735,#3230,.T.) ;
#43283=EDGE_CURVE('',#35736,#35315,#3231,.T.) ;
#43284=EDGE_CURVE('',#35737,#35738,#3232,.T.) ;
#43285=EDGE_CURVE('',#35737,#35739,#3233,.T.) ;
#43286=EDGE_CURVE('',#35739,#35740,#29347,.T.) ;
#43287=EDGE_CURVE('',#35740,#35738,#3234,.T.) ;
#43288=EDGE_CURVE('',#35543,#35737,#29348,.T.) ;
#43289=EDGE_CURVE('',#35738,#35730,#29349,.T.) ;
#43290=EDGE_CURVE('',#35731,#35430,#29350,.T.) ;
#43291=EDGE_CURVE('',#35429,#35736,#29351,.T.) ;
#43292=EDGE_CURVE('',#35735,#35447,#29352,.T.) ;
#43293=EDGE_CURVE('',#35741,#35742,#3235,.T.) ;
#43294=EDGE_CURVE('',#35742,#35743,#3236,.T.) ;
#43295=EDGE_CURVE('',#35743,#35744,#3237,.T.) ;
#43296=EDGE_CURVE('',#35744,#35741,#3238,.T.) ;
#43297=EDGE_CURVE('',#35745,#35746,#3239,.T.) ;
#43298=EDGE_CURVE('',#35746,#35747,#3240,.T.) ;
#43299=EDGE_CURVE('',#35747,#35748,#3241,.T.) ;
#43300=EDGE_CURVE('',#35748,#35745,#3242,.T.) ;
#43301=EDGE_CURVE('',#35749,#35750,#323,.T.) ;
#43302=EDGE_CURVE('',#35749,#35751,#3243,.T.) ;
#43303=EDGE_CURVE('',#35751,#35752,#3244,.T.) ;
#43304=EDGE_CURVE('',#35752,#35753,#3245,.T.) ;
#43305=EDGE_CURVE('',#35754,#35753,#324,.T.) ;
#43306=EDGE_CURVE('',#35754,#35755,#3246,.T.) ;
#43307=EDGE_CURVE('',#35755,#35756,#3247,.T.) ;
#43308=EDGE_CURVE('',#35756,#35750,#3248,.T.) ;
#43309=EDGE_CURVE('',#35757,#35758,#3249,.T.) ;
#43310=EDGE_CURVE('',#35758,#35759,#325,.T.) ;
#43311=EDGE_CURVE('',#35760,#35759,#3250,.T.) ;
#43312=EDGE_CURVE('',#35760,#35752,#326,.T.) ;
#43313=EDGE_CURVE('',#35751,#35761,#327,.T.) ;
#43314=EDGE_CURVE('',#35761,#35762,#3251,.T.) ;
#43315=EDGE_CURVE('',#35762,#35757,#328,.T.) ;
#43316=EDGE_CURVE('',#35763,#35764,#329,.T.) ;
#43317=EDGE_CURVE('',#35763,#35758,#3252,.T.) ;
#43318=EDGE_CURVE('',#35757,#35765,#3253,.T.) ;
#43319=EDGE_CURVE('',#35766,#35765,#330,.T.) ;
#43320=EDGE_CURVE('',#35766,#35767,#3254,.T.) ;
#43321=EDGE_CURVE('',#35767,#35768,#3255,.T.) ;
#43322=EDGE_CURVE('',#35768,#35764,#3256,.T.) ;
#43323=EDGE_CURVE('',#35761,#35769,#3257,.T.) ;
#43324=EDGE_CURVE('',#35769,#35770,#3258,.T.) ;
#43325=EDGE_CURVE('',#35770,#35762,#3259,.T.) ;
#43326=EDGE_CURVE('',#35759,#35771,#3260,.T.) ;
#43327=EDGE_CURVE('',#35771,#35772,#3261,.T.) ;
#43328=EDGE_CURVE('',#35772,#35760,#3262,.T.) ;
#43329=EDGE_CURVE('',#35773,#35774,#3263,.T.) ;
#43330=EDGE_CURVE('',#35774,#35775,#3264,.T.) ;
#43331=EDGE_CURVE('',#35775,#35776,#3265,.T.) ;
#43332=EDGE_CURVE('',#35776,#35777,#3266,.T.) ;
#43333=EDGE_CURVE('',#35777,#35778,#3267,.T.) ;
#43334=EDGE_CURVE('',#35778,#35773,#3268,.T.) ;
#43335=EDGE_CURVE('',#35779,#35780,#3269,.T.) ;
#43336=EDGE_CURVE('',#35780,#35781,#3270,.T.) ;
#43337=EDGE_CURVE('',#35781,#35782,#3271,.T.) ;
#43338=EDGE_CURVE('',#35782,#35783,#3272,.T.) ;
#43339=EDGE_CURVE('',#35783,#35784,#3273,.T.) ;
#43340=EDGE_CURVE('',#35784,#35779,#3274,.T.) ;
#43341=EDGE_CURVE('',#35785,#35786,#3275,.T.) ;
#43342=EDGE_CURVE('',#35786,#35787,#3276,.T.) ;
#43343=EDGE_CURVE('',#35787,#35788,#3277,.T.) ;
#43344=EDGE_CURVE('',#35788,#35785,#3278,.T.) ;
#43345=EDGE_CURVE('',#35789,#35790,#3279,.T.) ;
#43346=EDGE_CURVE('',#35790,#35791,#3280,.T.) ;
#43347=EDGE_CURVE('',#35791,#35792,#3281,.T.) ;
#43348=EDGE_CURVE('',#35792,#35789,#3282,.T.) ;
#43349=EDGE_CURVE('',#35793,#35794,#3283,.T.) ;
#43350=EDGE_CURVE('',#35794,#35795,#3284,.T.) ;
#43351=EDGE_CURVE('',#35795,#35796,#3285,.T.) ;
#43352=EDGE_CURVE('',#35796,#35793,#3286,.T.) ;
#43353=EDGE_CURVE('',#35797,#35798,#3287,.T.) ;
#43354=EDGE_CURVE('',#35798,#35799,#3288,.T.) ;
#43355=EDGE_CURVE('',#35799,#35800,#3289,.T.) ;
#43356=EDGE_CURVE('',#35800,#35797,#3290,.T.) ;
#43357=EDGE_CURVE('',#35801,#35802,#3291,.T.) ;
#43358=EDGE_CURVE('',#35802,#35803,#3292,.T.) ;
#43359=EDGE_CURVE('',#35803,#35804,#3293,.T.) ;
#43360=EDGE_CURVE('',#35804,#35801,#3294,.T.) ;
#43361=EDGE_CURVE('',#35805,#35806,#3295,.T.) ;
#43362=EDGE_CURVE('',#35807,#35805,#29353,.T.) ;
#43363=EDGE_CURVE('',#35808,#35807,#3296,.T.) ;
#43364=EDGE_CURVE('',#35809,#35808,#29354,.T.) ;
#43365=EDGE_CURVE('',#35810,#35809,#3297,.T.) ;
#43366=EDGE_CURVE('',#35811,#35810,#29355,.T.) ;
#43367=EDGE_CURVE('',#35812,#35811,#3298,.T.) ;
#43368=EDGE_CURVE('',#35806,#35812,#29356,.T.) ;
#43369=EDGE_CURVE('',#35813,#35814,#29357,.T.) ;
#43370=EDGE_CURVE('',#35806,#35813,#3299,.T.) ;
#43371=EDGE_CURVE('',#35812,#35814,#3300,.T.) ;
#43372=EDGE_CURVE('',#35815,#35813,#3301,.T.) ;
#43373=EDGE_CURVE('',#35805,#35815,#3302,.T.) ;
#43374=EDGE_CURVE('',#35816,#35815,#29358,.T.) ;
#43375=EDGE_CURVE('',#35807,#35816,#3303,.T.) ;
#43376=EDGE_CURVE('',#35817,#35816,#3304,.T.) ;
#43377=EDGE_CURVE('',#35808,#35817,#3305,.T.) ;
#43378=EDGE_CURVE('',#35818,#35817,#29359,.T.) ;
#43379=EDGE_CURVE('',#35809,#35818,#3306,.T.) ;
#43380=EDGE_CURVE('',#35819,#35818,#3307,.T.) ;
#43381=EDGE_CURVE('',#35810,#35819,#3308,.T.) ;
#43382=EDGE_CURVE('',#35820,#35819,#29360,.T.) ;
#43383=EDGE_CURVE('',#35811,#35820,#3309,.T.) ;
#43384=EDGE_CURVE('',#35814,#35820,#3310,.T.) ;
#43385=EDGE_CURVE('',#35331,#35332,#3311,.T.) ;
#43386=EDGE_CURVE('',#35329,#35334,#3312,.T.) ;
#43387=EDGE_CURVE('',#35333,#35330,#3313,.T.) ;
#43388=EDGE_CURVE('',#35337,#35326,#3314,.T.) ;
#43389=EDGE_CURVE('',#35325,#35338,#3315,.T.) ;
#43390=EDGE_CURVE('',#35327,#35336,#3316,.T.) ;
#43391=EDGE_CURVE('',#35335,#35328,#3317,.T.) ;
#43392=EDGE_CURVE('',#35821,#35822,#3318,.T.) ;
#43393=EDGE_CURVE('',#35822,#35823,#3319,.T.) ;
#43394=EDGE_CURVE('',#35823,#35824,#3320,.T.) ;
#43395=EDGE_CURVE('',#35824,#35821,#3321,.T.) ;
#43396=EDGE_CURVE('',#35825,#35826,#3322,.T.) ;
#43397=EDGE_CURVE('',#35826,#35827,#3323,.T.) ;
#43398=EDGE_CURVE('',#35827,#35828,#3324,.T.) ;
#43399=EDGE_CURVE('',#35828,#35825,#3325,.T.) ;
#43400=EDGE_CURVE('',#35829,#35830,#3326,.T.) ;
#43401=EDGE_CURVE('',#35830,#35831,#3327,.T.) ;
#43402=EDGE_CURVE('',#35831,#35832,#3328,.T.) ;
#43403=EDGE_CURVE('',#35832,#35829,#3329,.T.) ;
#43404=EDGE_CURVE('',#35833,#35834,#3330,.T.) ;
#43405=EDGE_CURVE('',#35834,#35835,#3331,.T.) ;
#43406=EDGE_CURVE('',#35835,#35836,#3332,.T.) ;
#43407=EDGE_CURVE('',#35836,#35833,#3333,.T.) ;
#43408=EDGE_CURVE('',#35837,#35838,#3334,.T.) ;
#43409=EDGE_CURVE('',#35838,#35839,#3335,.T.) ;
#43410=EDGE_CURVE('',#35839,#35840,#3336,.T.) ;
#43411=EDGE_CURVE('',#35840,#35837,#3337,.T.) ;
#43412=EDGE_CURVE('',#35841,#35842,#3338,.T.) ;
#43413=EDGE_CURVE('',#35843,#35841,#29361,.T.) ;
#43414=EDGE_CURVE('',#35844,#35843,#3339,.T.) ;
#43415=EDGE_CURVE('',#35845,#35844,#29362,.T.) ;
#43416=EDGE_CURVE('',#35846,#35845,#3340,.T.) ;
#43417=EDGE_CURVE('',#35847,#35846,#29363,.T.) ;
#43418=EDGE_CURVE('',#35848,#35847,#3341,.T.) ;
#43419=EDGE_CURVE('',#35842,#35848,#29364,.T.) ;
#43420=EDGE_CURVE('',#35848,#35849,#3342,.T.) ;
#43421=EDGE_CURVE('',#35849,#35850,#29365,.T.) ;
#43422=EDGE_CURVE('',#35842,#35850,#3343,.T.) ;
#43423=EDGE_CURVE('',#35850,#35851,#3344,.T.) ;
#43424=EDGE_CURVE('',#35841,#35851,#3345,.T.) ;
#43425=EDGE_CURVE('',#35851,#35852,#29366,.T.) ;
#43426=EDGE_CURVE('',#35843,#35852,#3346,.T.) ;
#43427=EDGE_CURVE('',#35852,#35853,#3347,.T.) ;
#43428=EDGE_CURVE('',#35844,#35853,#3348,.T.) ;
#43429=EDGE_CURVE('',#35853,#35854,#29367,.T.) ;
#43430=EDGE_CURVE('',#35845,#35854,#3349,.T.) ;
#43431=EDGE_CURVE('',#35854,#35855,#3350,.T.) ;
#43432=EDGE_CURVE('',#35846,#35855,#3351,.T.) ;
#43433=EDGE_CURVE('',#35855,#35856,#29368,.T.) ;
#43434=EDGE_CURVE('',#35847,#35856,#3352,.T.) ;
#43435=EDGE_CURVE('',#35856,#35849,#3353,.T.) ;
#43436=EDGE_CURVE('',#35857,#35858,#3354,.T.) ;
#43437=EDGE_CURVE('',#35858,#35859,#3355,.T.) ;
#43438=EDGE_CURVE('',#35859,#35860,#3356,.T.) ;
#43439=EDGE_CURVE('',#35860,#35857,#3357,.T.) ;
#43440=EDGE_CURVE('',#35320,#35300,#3358,.T.) ;
#43441=EDGE_CURVE('',#35300,#35861,#3359,.T.) ;
#43442=EDGE_CURVE('',#35861,#35862,#3360,.T.) ;
#43443=EDGE_CURVE('',#35862,#35320,#3361,.T.) ;
#43444=EDGE_CURVE('',#35863,#35317,#3362,.T.) ;
#43445=EDGE_CURVE('',#35310,#35864,#3363,.T.) ;
#43446=EDGE_CURVE('',#35864,#35863,#3364,.T.) ;
#43447=EDGE_CURVE('',#35318,#35865,#3365,.T.) ;
#43448=EDGE_CURVE('',#35865,#35314,#3366,.T.) ;
#43449=EDGE_CURVE('',#35314,#35311,#3367,.T.) ;
#43450=EDGE_CURVE('',#35299,#35866,#3368,.T.) ;
#43451=EDGE_CURVE('',#35866,#35867,#29369,.T.) ;
#43452=EDGE_CURVE('',#35867,#35868,#3369,.T.) ;
#43453=EDGE_CURVE('',#35868,#35869,#3370,.T.) ;
#43454=EDGE_CURVE('',#35869,#35298,#3371,.T.) ;
#43455=EDGE_CURVE('',#35870,#35871,#29370,.T.) ;
#43456=EDGE_CURVE('',#35871,#35872,#29371,.T.) ;
#43457=EDGE_CURVE('',#35872,#35873,#29372,.T.) ;
#43458=EDGE_CURVE('',#35873,#35874,#3372,.T.) ;
#43459=EDGE_CURVE('',#35874,#35875,#29373,.T.) ;
#43460=EDGE_CURVE('',#35875,#35870,#3373,.T.) ;
#43461=EDGE_CURVE('',#35779,#35494,#29374,.T.) ;
#43462=EDGE_CURVE('',#35747,#35779,#2111,.T.) ;
#43463=EDGE_CURVE('',#35495,#35747,#29375,.T.) ;
#43464=EDGE_CURVE('',#35769,#35749,#29376,.T.) ;
#43465=EDGE_CURVE('',#35783,#35750,#29377,.T.) ;
#43466=EDGE_CURVE('',#35769,#35783,#331,.T.) ;
#43467=EDGE_CURVE('',#35784,#35756,#29378,.T.) ;
#43468=EDGE_CURVE('',#35748,#35784,#29379,.T.) ;
#43469=EDGE_CURVE('',#35496,#35746,#29380,.T.) ;
#43470=EDGE_CURVE('',#35780,#35493,#29381,.T.) ;
#43471=EDGE_CURVE('',#35770,#35782,#332,.T.) ;
#43472=EDGE_CURVE('',#35765,#35770,#29382,.T.) ;
#43473=EDGE_CURVE('',#35748,#35756,#29383,.T.) ;
#43474=EDGE_CURVE('',#35777,#35746,#333,.T.) ;
#43475=EDGE_CURVE('',#35497,#35777,#29384,.T.) ;
#43476=EDGE_CURVE('',#35742,#35500,#29385,.T.) ;
#43477=EDGE_CURVE('',#35780,#35742,#2112,.T.) ;
#43478=EDGE_CURVE('',#35766,#35782,#29386,.T.) ;
#43479=EDGE_CURVE('',#35745,#35755,#29387,.T.) ;
#43480=EDGE_CURVE('',#35778,#35745,#29388,.T.) ;
#43481=EDGE_CURVE('',#35498,#35776,#29389,.T.) ;
#43482=EDGE_CURVE('',#35743,#35499,#29390,.T.) ;
#43483=EDGE_CURVE('',#35781,#35741,#29391,.T.) ;
#43484=EDGE_CURVE('',#35767,#35781,#29392,.T.) ;
#43485=EDGE_CURVE('',#35778,#35755,#29393,.T.) ;
#43486=EDGE_CURVE('',#35743,#35776,#334,.T.) ;
#43487=EDGE_CURVE('',#35767,#35741,#29394,.T.) ;
#43488=EDGE_CURVE('',#35753,#35772,#29395,.T.) ;
#43489=EDGE_CURVE('',#35773,#35754,#29396,.T.) ;
#43490=EDGE_CURVE('',#35744,#35775,#29397,.T.) ;
#43491=EDGE_CURVE('',#35768,#35744,#29398,.T.) ;
#43492=EDGE_CURVE('',#35773,#35772,#335,.T.) ;
#43493=EDGE_CURVE('',#35768,#35775,#29399,.T.) ;
#43494=EDGE_CURVE('',#35774,#35771,#336,.T.) ;
#43495=EDGE_CURVE('',#35764,#35774,#29400,.T.) ;
#43496=EDGE_CURVE('',#35763,#35771,#29401,.T.) ;
#43497=EDGE_CURVE('',#35444,#35876,#337,.T.) ;
#43498=EDGE_CURVE('',#35876,#35301,#2113,.T.) ;
#43499=EDGE_CURVE('',#35861,#35863,#29402,.T.) ;
#43500=EDGE_CURVE('',#35862,#35864,#29403,.T.) ;
#43501=EDGE_CURVE('',#35427,#35862,#29404,.T.) ;
#43502=EDGE_CURVE('',#35449,#35866,#2114,.T.) ;
#43503=EDGE_CURVE('',#35299,#35450,#2115,.T.) ;
#43504=EDGE_CURVE('',#35868,#35317,#29405,.T.) ;
#43505=EDGE_CURVE('',#35863,#35869,#29406,.T.) ;
#43506=EDGE_CURVE('',#35428,#35864,#29407,.T.) ;
#43507=EDGE_CURVE('',#35877,#35878,#2116,.T.) ;
#43508=EDGE_CURVE('',#35878,#35734,#338,.T.) ;
#43509=EDGE_CURVE('',#35865,#35877,#29408,.T.) ;
#43510=EDGE_CURVE('',#35852,#35857,#29409,.T.) ;
#43511=EDGE_CURVE('',#35857,#35851,#29410,.T.) ;
#43512=EDGE_CURVE('',#35858,#35850,#29411,.T.) ;
#43513=EDGE_CURVE('',#35853,#35860,#29412,.T.) ;
#43514=EDGE_CURVE('',#35858,#35849,#29413,.T.) ;
#43515=EDGE_CURVE('',#35854,#35860,#29414,.T.) ;
#43516=EDGE_CURVE('',#35859,#35856,#29415,.T.) ;
#43517=EDGE_CURVE('',#35855,#35859,#29416,.T.) ;
#43518=EDGE_CURVE('',#35519,#35788,#29417,.T.) ;
#43519=EDGE_CURVE('',#35785,#35518,#29418,.T.) ;
#43520=EDGE_CURVE('',#35800,#35517,#29419,.T.) ;
#43521=EDGE_CURVE('',#35785,#35800,#29420,.T.) ;
#43522=EDGE_CURVE('',#35792,#35788,#29421,.T.) ;
#43523=EDGE_CURVE('',#35520,#35792,#29422,.T.) ;
#43524=EDGE_CURVE('',#35797,#35516,#29423,.T.) ;
#43525=EDGE_CURVE('',#35786,#35799,#29424,.T.) ;
#43526=EDGE_CURVE('',#35787,#35804,#29425,.T.) ;
#43527=EDGE_CURVE('',#35801,#35786,#29426,.T.) ;
#43528=EDGE_CURVE('',#35789,#35787,#29427,.T.) ;
#43529=EDGE_CURVE('',#35514,#35791,#29428,.T.) ;
#43530=EDGE_CURVE('',#35515,#35795,#29429,.T.) ;
#43531=EDGE_CURVE('',#35796,#35513,#29430,.T.) ;
#43532=EDGE_CURVE('',#35797,#35795,#29431,.T.) ;
#43533=EDGE_CURVE('',#35801,#35799,#29432,.T.) ;
#43534=EDGE_CURVE('',#35789,#35804,#29433,.T.) ;
#43535=EDGE_CURVE('',#35796,#35791,#29434,.T.) ;
#43536=EDGE_CURVE('',#35798,#35794,#29435,.T.) ;
#43537=EDGE_CURVE('',#35802,#35798,#29436,.T.) ;
#43538=EDGE_CURVE('',#35790,#35803,#29437,.T.) ;
#43539=EDGE_CURVE('',#35793,#35790,#29438,.T.) ;
#43540=EDGE_CURVE('',#35802,#35794,#29439,.T.) ;
#43541=EDGE_CURVE('',#35793,#35803,#29440,.T.) ;
#43542=EDGE_CURVE('',#35471,#35832,#29441,.T.) ;
#43543=EDGE_CURVE('',#35829,#35470,#29442,.T.) ;
#43544=EDGE_CURVE('',#35828,#35469,#29443,.T.) ;
#43545=EDGE_CURVE('',#35829,#35828,#29444,.T.) ;
#43546=EDGE_CURVE('',#35836,#35832,#29445,.T.) ;
#43547=EDGE_CURVE('',#35472,#35836,#29446,.T.) ;
#43548=EDGE_CURVE('',#35825,#35468,#29447,.T.) ;
#43549=EDGE_CURVE('',#35830,#35827,#29448,.T.) ;
#43550=EDGE_CURVE('',#35831,#35840,#29449,.T.) ;
#43551=EDGE_CURVE('',#35837,#35830,#29450,.T.) ;
#43552=EDGE_CURVE('',#35833,#35831,#29451,.T.) ;
#43553=EDGE_CURVE('',#35466,#35835,#29452,.T.) ;
#43554=EDGE_CURVE('',#35467,#35823,#29453,.T.) ;
#43555=EDGE_CURVE('',#35824,#35465,#29454,.T.) ;
#43556=EDGE_CURVE('',#35825,#35823,#29455,.T.) ;
#43557=EDGE_CURVE('',#35837,#35827,#29456,.T.) ;
#43558=EDGE_CURVE('',#35833,#35840,#29457,.T.) ;
#43559=EDGE_CURVE('',#35824,#35835,#29458,.T.) ;
#43560=EDGE_CURVE('',#35826,#35822,#29459,.T.) ;
#43561=EDGE_CURVE('',#35838,#35826,#29460,.T.) ;
#43562=EDGE_CURVE('',#35834,#35839,#29461,.T.) ;
#43563=EDGE_CURVE('',#35821,#35834,#29462,.T.) ;
#43564=EDGE_CURVE('',#35838,#35822,#29463,.T.) ;
#43565=EDGE_CURVE('',#35821,#35839,#29464,.T.) ;
#43566=EDGE_CURVE('',#35739,#35871,#2117,.T.) ;
#43567=EDGE_CURVE('',#35740,#35870,#29465,.T.) ;
#43568=EDGE_CURVE('',#35732,#35740,#29466,.T.) ;
#43569=EDGE_CURVE('',#35732,#35870,#29467,.T.) ;
#43570=EDGE_CURVE('',#35733,#35875,#29468,.T.) ;
#43571=EDGE_CURVE('',#35431,#35733,#29469,.T.) ;
#43572=EDGE_CURVE('',#35432,#35875,#29470,.T.) ;
#43573=EDGE_CURVE('',#35433,#35874,#29471,.T.) ;
#43574=EDGE_CURVE('',#35421,#35874,#29472,.T.) ;
#43575=EDGE_CURVE('',#35422,#35873,#29473,.T.) ;
#43576=EDGE_CURVE('',#35548,#35873,#29474,.T.) ;
#43577=EDGE_CURVE('',#35872,#35549,#2118,.T.) ;
#43578=EDGE_CURVE('',#35318,#35868,#29475,.T.) ;
#43579=EDGE_CURVE('',#35865,#35867,#29476,.T.) ;
#43580=EDGE_CURVE('',#35877,#35866,#29477,.T.) ;
#43581=EDGE_CURVE('',#35878,#35449,#29478,.T.) ;
#43582=EDGE_CURVE('',#35734,#35448,#29479,.T.) ;
#43583=EDGE_CURVE('',#35876,#35450,#29480,.T.) ;
#43584=EDGE_CURVE('',#35861,#35869,#29481,.T.) ;
#43585=EDGE_CURVE('',#35879,#35880,#2119,.T.) ;
#43586=EDGE_CURVE('',#35880,#35872,#2120,.T.) ;
#43587=EDGE_CURVE('',#35871,#35881,#2121,.T.) ;
#43588=EDGE_CURVE('',#35881,#35879,#2122,.T.) ;
#43589=EDGE_CURVE('',#35739,#35542,#29482,.T.) ;
#43590=EDGE_CURVE('',#35541,#35871,#2123,.T.) ;
#43591=EDGE_CURVE('',#35872,#35539,#2124,.T.) ;
#43592=EDGE_CURVE('',#35881,#35541,#29483,.T.) ;
#43593=EDGE_CURVE('',#35879,#35540,#29484,.T.) ;
#43594=EDGE_CURVE('',#35880,#35539,#29485,.T.) ;
#43595=EDGE_CURVE('',#35703,#35721,#29486,.T.) ;
#43596=EDGE_CURVE('',#35721,#35705,#29487,.T.) ;
#43597=EDGE_CURVE('',#35704,#35723,#29488,.T.) ;
#43598=EDGE_CURVE('',#35723,#35702,#29489,.T.) ;
#43599=EDGE_CURVE('',#35722,#35707,#29490,.T.) ;
#43600=EDGE_CURVE('',#35701,#35720,#29491,.T.) ;
#43601=EDGE_CURVE('',#35724,#35700,#29492,.T.) ;
#43602=EDGE_CURVE('',#35706,#35729,#29493,.T.) ;
#43603=EDGE_CURVE('',#35722,#35709,#29494,.T.) ;
#43604=EDGE_CURVE('',#35699,#35720,#29495,.T.) ;
#43605=EDGE_CURVE('',#35724,#35698,#29496,.T.) ;
#43606=EDGE_CURVE('',#35708,#35729,#29497,.T.) ;
#43607=EDGE_CURVE('',#35716,#35711,#29498,.T.) ;
#43608=EDGE_CURVE('',#35696,#35719,#2125,.T.) ;
#43609=EDGE_CURVE('',#35697,#35393,#29499,.T.) ;
#43610=EDGE_CURVE('',#35394,#35696,#29500,.T.) ;
#43611=EDGE_CURVE('',#35725,#35697,#2126,.T.) ;
#43612=EDGE_CURVE('',#35710,#35728,#29501,.T.) ;
#43613=EDGE_CURVE('',#35717,#35713,#29502,.T.) ;
#43614=EDGE_CURVE('',#35395,#35719,#29503,.T.) ;
#43615=EDGE_CURVE('',#35725,#35392,#29504,.T.) ;
#43616=EDGE_CURVE('',#35712,#35727,#29505,.T.) ;
#43617=EDGE_CURVE('',#35718,#35715,#29506,.T.) ;
#43618=EDGE_CURVE('',#35396,#35718,#29507,.T.) ;
#43619=EDGE_CURVE('',#35726,#35390,#29508,.T.) ;
#43620=EDGE_CURVE('',#35714,#35726,#29509,.T.) ;
#43621=EDGE_CURVE('',#35397,#35715,#29510,.T.) ;
#43622=EDGE_CURVE('',#35714,#35391,#29511,.T.) ;
#43623=EDGE_CURVE('',#35882,#35883,#29512,.T.) ;
#43624=EDGE_CURVE('',#35884,#35882,#29513,.T.) ;
#43625=EDGE_CURVE('',#35885,#35884,#29514,.T.) ;
#43626=EDGE_CURVE('',#35885,#35883,#29515,.T.) ;
#43627=EDGE_CURVE('',#35886,#35887,#29516,.T.) ;
#43628=EDGE_CURVE('',#35888,#35886,#3374,.T.) ;
#43629=EDGE_CURVE('',#35889,#35888,#29517,.T.) ;
#43630=EDGE_CURVE('',#35887,#35889,#3375,.T.) ;
#43631=EDGE_CURVE('',#35890,#35890,#29518,.T.) ;
#43632=EDGE_CURVE('',#35890,#35891,#29519,.T.) ;
#43633=EDGE_CURVE('',#35892,#35891,#29520,.T.) ;
#43634=EDGE_CURVE('',#35891,#35892,#29521,.T.) ;
#43635=EDGE_CURVE('',#35893,#35893,#29522,.T.) ;
#43636=EDGE_CURVE('',#35893,#35894,#29523,.T.) ;
#43637=EDGE_CURVE('',#35894,#35894,#29524,.T.) ;
#43638=EDGE_CURVE('',#35895,#35895,#29525,.T.) ;
#43639=EDGE_CURVE('',#35895,#35896,#29526,.T.) ;
#43640=EDGE_CURVE('',#35897,#35896,#29527,.T.) ;
#43641=EDGE_CURVE('',#35896,#35897,#29528,.T.) ;
#43642=EDGE_CURVE('',#35898,#35899,#29529,.T.) ;
#43643=EDGE_CURVE('',#35900,#35899,#29530,.T.) ;
#43644=EDGE_CURVE('',#35900,#35901,#29531,.T.) ;
#43645=EDGE_CURVE('',#35901,#35898,#29532,.T.) ;
#43646=EDGE_CURVE('',#35902,#35903,#29533,.T.) ;
#43647=EDGE_CURVE('',#35903,#35904,#29534,.T.) ;
#43648=EDGE_CURVE('',#35902,#35904,#29535,.T.) ;
#43649=EDGE_CURVE('',#35905,#35898,#3376,.T.) ;
#43650=EDGE_CURVE('',#35905,#35906,#29536,.T.) ;
#43651=EDGE_CURVE('',#35899,#35906,#3377,.T.) ;
#43652=EDGE_CURVE('',#35907,#35908,#29537,.T.) ;
#43653=EDGE_CURVE('',#35907,#35909,#29538,.T.) ;
#43654=EDGE_CURVE('',#35908,#35909,#29539,.T.) ;
#43655=EDGE_CURVE('',#35910,#35910,#29540,.T.) ;
#43656=EDGE_CURVE('',#35910,#35893,#3378,.T.) ;
#43657=EDGE_CURVE('',#35894,#35897,#3379,.T.) ;
#43658=EDGE_CURVE('',#35911,#35912,#29541,.T.) ;
#43659=EDGE_CURVE('',#35911,#35913,#2127,.T.) ;
#43660=EDGE_CURVE('',#35914,#35913,#3380,.T.) ;
#43661=EDGE_CURVE('',#35914,#35915,#2128,.T.) ;
#43662=EDGE_CURVE('',#35916,#35915,#29542,.T.) ;
#43663=EDGE_CURVE('',#35916,#35917,#2129,.T.) ;
#43664=EDGE_CURVE('',#35917,#35918,#3381,.T.) ;
#43665=EDGE_CURVE('',#35918,#35919,#2130,.T.) ;
#43666=EDGE_CURVE('',#35920,#35919,#29543,.T.) ;
#43667=EDGE_CURVE('',#35920,#35921,#2131,.T.) ;
#43668=EDGE_CURVE('',#35922,#35921,#3382,.T.) ;
#43669=EDGE_CURVE('',#35922,#35923,#2132,.T.) ;
#43670=EDGE_CURVE('',#35924,#35923,#29544,.T.) ;
#43671=EDGE_CURVE('',#35924,#35925,#2133,.T.) ;
#43672=EDGE_CURVE('',#35925,#35926,#3383,.T.) ;
#43673=EDGE_CURVE('',#35926,#35927,#2134,.T.) ;
#43674=EDGE_CURVE('',#35912,#35927,#29545,.T.) ;
#43675=EDGE_CURVE('',#35912,#35892,#3384,.T.) ;
#43676=EDGE_CURVE('',#35928,#35929,#29546,.T.) ;
#43677=EDGE_CURVE('',#35929,#35930,#3385,.T.) ;
#43678=EDGE_CURVE('',#35930,#35931,#3386,.T.) ;
#43679=EDGE_CURVE('',#35931,#35928,#3387,.T.) ;
#43680=EDGE_CURVE('',#35932,#35933,#3388,.T.) ;
#43681=EDGE_CURVE('',#35932,#35934,#3389,.T.) ;
#43682=EDGE_CURVE('',#35934,#35935,#3390,.T.) ;
#43683=EDGE_CURVE('',#35935,#35933,#3391,.T.) ;
#43684=EDGE_CURVE('',#35936,#35937,#3392,.T.) ;
#43685=EDGE_CURVE('',#35937,#35938,#3393,.T.) ;
#43686=EDGE_CURVE('',#35938,#35909,#3394,.T.) ;
#43687=EDGE_CURVE('',#35909,#35936,#3395,.T.) ;
#43688=EDGE_CURVE('',#35927,#35911,#3396,.T.) ;
#43689=EDGE_CURVE('',#35900,#35904,#3397,.T.) ;
#43690=EDGE_CURVE('',#35904,#35939,#3398,.T.) ;
#43691=EDGE_CURVE('',#35940,#35939,#3399,.T.) ;
#43692=EDGE_CURVE('',#35940,#35941,#3400,.T.) ;
#43693=EDGE_CURVE('',#35942,#35941,#29547,.T.) ;
#43694=EDGE_CURVE('',#35942,#35943,#29548,.T.) ;
#43695=EDGE_CURVE('',#35944,#35943,#29549,.T.) ;
#43696=EDGE_CURVE('',#35944,#35945,#3401,.T.) ;
#43697=EDGE_CURVE('',#35945,#35946,#3402,.T.) ;
#43698=EDGE_CURVE('',#35946,#35907,#3403,.T.) ;
#43699=EDGE_CURVE('',#35907,#35947,#3404,.T.) ;
#43700=EDGE_CURVE('',#35948,#35947,#29550,.T.) ;
#43701=EDGE_CURVE('',#35948,#35901,#3405,.T.) ;
#43702=EDGE_CURVE('',#35903,#35949,#3406,.T.) ;
#43703=EDGE_CURVE('',#35949,#35950,#3407,.T.) ;
#43704=EDGE_CURVE('',#35951,#35950,#3408,.T.) ;
#43705=EDGE_CURVE('',#35951,#35903,#3409,.T.) ;
#43706=EDGE_CURVE('',#35952,#35953,#3410,.T.) ;
#43707=EDGE_CURVE('',#35952,#35954,#3411,.T.) ;
#43708=EDGE_CURVE('',#35954,#35955,#339,.T.) ;
#43709=EDGE_CURVE('',#35955,#35956,#3412,.T.) ;
#43710=EDGE_CURVE('',#35956,#35957,#340,.T.) ;
#43711=EDGE_CURVE('',#35957,#35958,#3413,.T.) ;
#43712=EDGE_CURVE('',#35958,#35959,#3414,.T.) ;
#43713=EDGE_CURVE('',#35959,#35953,#3415,.T.) ;
#43714=EDGE_CURVE('',#35960,#35961,#3416,.T.) ;
#43715=EDGE_CURVE('',#35961,#35962,#3417,.T.) ;
#43716=EDGE_CURVE('',#35963,#35962,#3418,.T.) ;
#43717=EDGE_CURVE('',#35963,#35960,#3419,.T.) ;
#43718=EDGE_CURVE('',#35964,#35965,#3420,.T.) ;
#43719=EDGE_CURVE('',#35965,#35966,#3421,.T.) ;
#43720=EDGE_CURVE('',#35967,#35966,#3422,.T.) ;
#43721=EDGE_CURVE('',#35967,#35964,#3423,.T.) ;
#43722=EDGE_CURVE('',#35968,#35969,#3424,.T.) ;
#43723=EDGE_CURVE('',#35969,#35970,#3425,.T.) ;
#43724=EDGE_CURVE('',#35971,#35970,#3426,.T.) ;
#43725=EDGE_CURVE('',#35971,#35968,#3427,.T.) ;
#43726=EDGE_CURVE('',#35972,#35973,#3428,.T.) ;
#43727=EDGE_CURVE('',#35973,#35974,#3429,.T.) ;
#43728=EDGE_CURVE('',#35975,#35974,#3430,.T.) ;
#43729=EDGE_CURVE('',#35975,#35972,#3431,.T.) ;
#43730=EDGE_CURVE('',#35976,#35977,#3432,.T.) ;
#43731=EDGE_CURVE('',#35977,#35978,#3433,.T.) ;
#43732=EDGE_CURVE('',#35979,#35978,#3434,.T.) ;
#43733=EDGE_CURVE('',#35979,#35976,#3435,.T.) ;
#43734=EDGE_CURVE('',#35980,#35981,#3436,.T.) ;
#43735=EDGE_CURVE('',#35981,#35982,#3437,.T.) ;
#43736=EDGE_CURVE('',#35983,#35982,#3438,.T.) ;
#43737=EDGE_CURVE('',#35983,#35980,#3439,.T.) ;
#43738=EDGE_CURVE('',#35984,#35985,#3440,.T.) ;
#43739=EDGE_CURVE('',#35985,#35986,#3441,.T.) ;
#43740=EDGE_CURVE('',#35987,#35986,#3442,.T.) ;
#43741=EDGE_CURVE('',#35987,#35984,#3443,.T.) ;
#43742=EDGE_CURVE('',#35988,#35989,#29551,.T.) ;
#43743=EDGE_CURVE('',#35988,#35990,#3444,.T.) ;
#43744=EDGE_CURVE('',#35991,#35990,#29552,.T.) ;
#43745=EDGE_CURVE('',#35991,#35992,#3445,.T.) ;
#43746=EDGE_CURVE('',#35993,#35992,#29553,.T.) ;
#43747=EDGE_CURVE('',#35993,#35994,#3446,.T.) ;
#43748=EDGE_CURVE('',#35995,#35994,#29554,.T.) ;
#43749=EDGE_CURVE('',#35995,#35989,#3447,.T.) ;
#43750=EDGE_CURVE('',#35996,#35997,#3448,.T.) ;
#43751=EDGE_CURVE('',#35997,#35998,#3449,.T.) ;
#43752=EDGE_CURVE('',#35999,#35998,#3450,.T.) ;
#43753=EDGE_CURVE('',#35999,#35996,#3451,.T.) ;
#43754=EDGE_CURVE('',#36000,#35887,#3452,.T.) ;
#43755=EDGE_CURVE('',#36001,#35889,#3453,.T.) ;
#43756=EDGE_CURVE('',#36001,#36000,#3454,.T.) ;
#43757=EDGE_CURVE('',#35886,#36002,#3455,.T.) ;
#43758=EDGE_CURVE('',#36002,#36003,#3456,.T.) ;
#43759=EDGE_CURVE('',#35888,#36003,#3457,.T.) ;
#43760=EDGE_CURVE('',#36004,#36005,#3458,.T.) ;
#43761=EDGE_CURVE('',#36005,#36006,#3459,.T.) ;
#43762=EDGE_CURVE('',#36007,#36006,#3460,.T.) ;
#43763=EDGE_CURVE('',#36007,#36004,#3461,.T.) ;
#43764=EDGE_CURVE('',#36008,#36009,#3462,.T.) ;
#43765=EDGE_CURVE('',#36009,#36010,#2135,.T.) ;
#43766=EDGE_CURVE('',#36010,#36011,#3463,.T.) ;
#43767=EDGE_CURVE('',#36012,#36011,#2136,.T.) ;
#43768=EDGE_CURVE('',#36012,#36013,#3464,.T.) ;
#43769=EDGE_CURVE('',#36014,#36013,#2137,.T.) ;
#43770=EDGE_CURVE('',#36014,#36015,#3465,.T.) ;
#43771=EDGE_CURVE('',#36015,#36008,#2138,.T.) ;
#43772=EDGE_CURVE('',#36016,#36017,#3466,.T.) ;
#43773=EDGE_CURVE('',#36017,#36018,#3467,.T.) ;
#43774=EDGE_CURVE('',#36019,#36018,#3468,.T.) ;
#43775=EDGE_CURVE('',#36019,#36016,#3469,.T.) ;
#43776=EDGE_CURVE('',#36020,#36021,#29555,.T.) ;
#43777=EDGE_CURVE('',#36020,#36022,#3470,.T.) ;
#43778=EDGE_CURVE('',#36023,#36022,#29556,.T.) ;
#43779=EDGE_CURVE('',#36023,#36024,#3471,.T.) ;
#43780=EDGE_CURVE('',#36025,#36024,#29557,.T.) ;
#43781=EDGE_CURVE('',#36025,#36026,#3472,.T.) ;
#43782=EDGE_CURVE('',#36027,#36026,#29558,.T.) ;
#43783=EDGE_CURVE('',#36027,#36021,#3473,.T.) ;
#43784=EDGE_CURVE('',#36028,#36029,#3474,.T.) ;
#43785=EDGE_CURVE('',#36029,#36030,#3475,.T.) ;
#43786=EDGE_CURVE('',#36031,#36030,#3476,.T.) ;
#43787=EDGE_CURVE('',#36031,#36028,#3477,.T.) ;
#43788=EDGE_CURVE('',#36032,#36033,#2139,.T.) ;
#43789=EDGE_CURVE('',#36033,#36034,#2140,.T.) ;
#43790=EDGE_CURVE('',#36034,#36035,#2141,.T.) ;
#43791=EDGE_CURVE('',#36035,#36036,#2142,.T.) ;
#43792=EDGE_CURVE('',#36036,#36037,#3478,.T.) ;
#43793=EDGE_CURVE('',#36038,#36037,#3479,.T.) ;
#43794=EDGE_CURVE('',#36038,#36039,#3480,.T.) ;
#43795=EDGE_CURVE('',#36039,#36040,#3481,.T.) ;
#43796=EDGE_CURVE('',#36040,#36032,#3482,.T.) ;
#43797=EDGE_CURVE('',#36041,#36042,#3483,.T.) ;
#43798=EDGE_CURVE('',#36041,#36043,#3484,.T.) ;
#43799=EDGE_CURVE('',#36043,#36044,#29559,.T.) ;
#43800=EDGE_CURVE('',#36044,#36042,#3485,.T.) ;
#43801=EDGE_CURVE('',#36045,#36046,#3486,.T.) ;
#43802=EDGE_CURVE('',#36046,#36047,#3487,.T.) ;
#43803=EDGE_CURVE('',#36047,#36048,#3488,.T.) ;
#43804=EDGE_CURVE('',#36048,#36045,#3489,.T.) ;
#43805=EDGE_CURVE('',#36037,#36041,#29560,.T.) ;
#43806=EDGE_CURVE('',#36042,#35932,#29561,.T.) ;
#43807=EDGE_CURVE('',#35933,#35940,#29562,.T.) ;
#43808=EDGE_CURVE('',#35939,#35951,#29563,.T.) ;
#43809=EDGE_CURVE('',#35950,#35952,#29564,.T.) ;
#43810=EDGE_CURVE('',#35953,#35963,#29565,.T.) ;
#43811=EDGE_CURVE('',#35962,#35967,#29566,.T.) ;
#43812=EDGE_CURVE('',#35966,#35971,#29567,.T.) ;
#43813=EDGE_CURVE('',#35970,#35975,#29568,.T.) ;
#43814=EDGE_CURVE('',#35974,#35979,#29569,.T.) ;
#43815=EDGE_CURVE('',#35978,#35983,#29570,.T.) ;
#43816=EDGE_CURVE('',#35982,#35987,#29571,.T.) ;
#43817=EDGE_CURVE('',#35986,#35999,#29572,.T.) ;
#43818=EDGE_CURVE('',#35998,#36001,#29573,.T.) ;
#43819=EDGE_CURVE('',#36003,#36007,#29574,.T.) ;
#43820=EDGE_CURVE('',#36006,#36019,#29575,.T.) ;
#43821=EDGE_CURVE('',#36018,#36031,#29576,.T.) ;
#43822=EDGE_CURVE('',#36030,#36038,#29577,.T.) ;
#43823=EDGE_CURVE('',#35930,#36040,#29578,.T.) ;
#43824=EDGE_CURVE('',#36039,#36029,#29579,.T.) ;
#43825=EDGE_CURVE('',#36028,#36017,#29580,.T.) ;
#43826=EDGE_CURVE('',#36016,#36005,#29581,.T.) ;
#43827=EDGE_CURVE('',#36004,#36002,#29582,.T.) ;
#43828=EDGE_CURVE('',#36000,#35997,#29583,.T.) ;
#43829=EDGE_CURVE('',#35996,#35985,#29584,.T.) ;
#43830=EDGE_CURVE('',#35984,#35981,#29585,.T.) ;
#43831=EDGE_CURVE('',#35980,#35977,#29586,.T.) ;
#43832=EDGE_CURVE('',#35976,#35973,#29587,.T.) ;
#43833=EDGE_CURVE('',#35972,#35969,#29588,.T.) ;
#43834=EDGE_CURVE('',#35968,#35965,#29589,.T.) ;
#43835=EDGE_CURVE('',#35964,#35961,#29590,.T.) ;
#43836=EDGE_CURVE('',#35960,#35959,#29591,.T.) ;
#43837=EDGE_CURVE('',#35958,#35937,#29592,.T.) ;
#43838=EDGE_CURVE('',#35936,#35946,#29593,.T.) ;
#43839=EDGE_CURVE('',#35945,#36048,#29594,.T.) ;
#43840=EDGE_CURVE('',#36047,#35931,#29595,.T.) ;
#43841=EDGE_CURVE('',#36049,#36050,#3490,.T.) ;
#43842=EDGE_CURVE('',#36050,#36051,#3491,.T.) ;
#43843=EDGE_CURVE('',#36051,#36052,#3492,.T.) ;
#43844=EDGE_CURVE('',#36052,#36049,#3493,.T.) ;
#43845=EDGE_CURVE('',#36053,#36054,#3494,.T.) ;
#43846=EDGE_CURVE('',#36054,#36055,#3495,.T.) ;
#43847=EDGE_CURVE('',#36055,#36056,#3496,.T.) ;
#43848=EDGE_CURVE('',#36056,#36053,#3497,.T.) ;
#43849=EDGE_CURVE('',#36057,#36058,#341,.T.) ;
#43850=EDGE_CURVE('',#36057,#36059,#3498,.T.) ;
#43851=EDGE_CURVE('',#36059,#36060,#3499,.T.) ;
#43852=EDGE_CURVE('',#36060,#36061,#3500,.T.) ;
#43853=EDGE_CURVE('',#36062,#36061,#342,.T.) ;
#43854=EDGE_CURVE('',#36062,#36063,#3501,.T.) ;
#43855=EDGE_CURVE('',#36063,#36064,#3502,.T.) ;
#43856=EDGE_CURVE('',#36064,#36058,#3503,.T.) ;
#43857=EDGE_CURVE('',#36065,#36066,#3504,.T.) ;
#43858=EDGE_CURVE('',#36066,#36067,#343,.T.) ;
#43859=EDGE_CURVE('',#36068,#36067,#3505,.T.) ;
#43860=EDGE_CURVE('',#36068,#36060,#344,.T.) ;
#43861=EDGE_CURVE('',#36059,#36069,#345,.T.) ;
#43862=EDGE_CURVE('',#36069,#36070,#3506,.T.) ;
#43863=EDGE_CURVE('',#36070,#36065,#346,.T.) ;
#43864=EDGE_CURVE('',#36071,#36072,#347,.T.) ;
#43865=EDGE_CURVE('',#36071,#36066,#3507,.T.) ;
#43866=EDGE_CURVE('',#36065,#36073,#3508,.T.) ;
#43867=EDGE_CURVE('',#36074,#36073,#348,.T.) ;
#43868=EDGE_CURVE('',#36074,#36075,#3509,.T.) ;
#43869=EDGE_CURVE('',#36075,#36076,#3510,.T.) ;
#43870=EDGE_CURVE('',#36076,#36072,#3511,.T.) ;
#43871=EDGE_CURVE('',#36069,#36077,#3512,.T.) ;
#43872=EDGE_CURVE('',#36077,#36078,#3513,.T.) ;
#43873=EDGE_CURVE('',#36078,#36070,#3514,.T.) ;
#43874=EDGE_CURVE('',#36067,#36079,#3515,.T.) ;
#43875=EDGE_CURVE('',#36079,#36080,#3516,.T.) ;
#43876=EDGE_CURVE('',#36080,#36068,#3517,.T.) ;
#43877=EDGE_CURVE('',#36081,#36082,#3518,.T.) ;
#43878=EDGE_CURVE('',#36082,#36083,#3519,.T.) ;
#43879=EDGE_CURVE('',#36083,#36084,#3520,.T.) ;
#43880=EDGE_CURVE('',#36084,#36085,#3521,.T.) ;
#43881=EDGE_CURVE('',#36085,#36086,#3522,.T.) ;
#43882=EDGE_CURVE('',#36086,#36081,#3523,.T.) ;
#43883=EDGE_CURVE('',#36087,#36088,#3524,.T.) ;
#43884=EDGE_CURVE('',#36088,#36089,#3525,.T.) ;
#43885=EDGE_CURVE('',#36089,#36090,#3526,.T.) ;
#43886=EDGE_CURVE('',#36090,#36091,#3527,.T.) ;
#43887=EDGE_CURVE('',#36091,#36092,#3528,.T.) ;
#43888=EDGE_CURVE('',#36092,#36087,#3529,.T.) ;
#43889=EDGE_CURVE('',#36093,#36094,#3530,.T.) ;
#43890=EDGE_CURVE('',#36094,#36095,#3531,.T.) ;
#43891=EDGE_CURVE('',#36095,#36096,#3532,.T.) ;
#43892=EDGE_CURVE('',#36096,#36093,#3533,.T.) ;
#43893=EDGE_CURVE('',#36097,#36098,#3534,.T.) ;
#43894=EDGE_CURVE('',#36098,#36099,#3535,.T.) ;
#43895=EDGE_CURVE('',#36099,#36100,#3536,.T.) ;
#43896=EDGE_CURVE('',#36100,#36097,#3537,.T.) ;
#43897=EDGE_CURVE('',#36101,#36102,#3538,.T.) ;
#43898=EDGE_CURVE('',#36102,#36103,#3539,.T.) ;
#43899=EDGE_CURVE('',#36103,#36104,#3540,.T.) ;
#43900=EDGE_CURVE('',#36104,#36101,#3541,.T.) ;
#43901=EDGE_CURVE('',#36105,#36106,#3542,.T.) ;
#43902=EDGE_CURVE('',#36106,#36107,#3543,.T.) ;
#43903=EDGE_CURVE('',#36107,#36108,#3544,.T.) ;
#43904=EDGE_CURVE('',#36108,#36105,#3545,.T.) ;
#43905=EDGE_CURVE('',#36109,#36110,#3546,.T.) ;
#43906=EDGE_CURVE('',#36110,#36111,#3547,.T.) ;
#43907=EDGE_CURVE('',#36111,#36112,#3548,.T.) ;
#43908=EDGE_CURVE('',#36112,#36109,#3549,.T.) ;
#43909=EDGE_CURVE('',#36113,#36114,#3550,.T.) ;
#43910=EDGE_CURVE('',#36115,#36113,#29596,.T.) ;
#43911=EDGE_CURVE('',#36116,#36115,#3551,.T.) ;
#43912=EDGE_CURVE('',#36117,#36116,#29597,.T.) ;
#43913=EDGE_CURVE('',#36118,#36117,#3552,.T.) ;
#43914=EDGE_CURVE('',#36119,#36118,#29598,.T.) ;
#43915=EDGE_CURVE('',#36120,#36119,#3553,.T.) ;
#43916=EDGE_CURVE('',#36114,#36120,#29599,.T.) ;
#43917=EDGE_CURVE('',#36121,#36122,#29600,.T.) ;
#43918=EDGE_CURVE('',#36114,#36121,#3554,.T.) ;
#43919=EDGE_CURVE('',#36120,#36122,#3555,.T.) ;
#43920=EDGE_CURVE('',#36123,#36121,#3556,.T.) ;
#43921=EDGE_CURVE('',#36113,#36123,#3557,.T.) ;
#43922=EDGE_CURVE('',#36124,#36123,#29601,.T.) ;
#43923=EDGE_CURVE('',#36115,#36124,#3558,.T.) ;
#43924=EDGE_CURVE('',#36125,#36124,#3559,.T.) ;
#43925=EDGE_CURVE('',#36116,#36125,#3560,.T.) ;
#43926=EDGE_CURVE('',#36126,#36125,#29602,.T.) ;
#43927=EDGE_CURVE('',#36117,#36126,#3561,.T.) ;
#43928=EDGE_CURVE('',#36127,#36126,#3562,.T.) ;
#43929=EDGE_CURVE('',#36118,#36127,#3563,.T.) ;
#43930=EDGE_CURVE('',#36128,#36127,#29603,.T.) ;
#43931=EDGE_CURVE('',#36119,#36128,#3564,.T.) ;
#43932=EDGE_CURVE('',#36122,#36128,#3565,.T.) ;
#43933=EDGE_CURVE('',#35919,#35920,#3566,.T.) ;
#43934=EDGE_CURVE('',#35917,#35922,#3567,.T.) ;
#43935=EDGE_CURVE('',#35921,#35918,#3568,.T.) ;
#43936=EDGE_CURVE('',#35925,#35914,#3569,.T.) ;
#43937=EDGE_CURVE('',#35913,#35926,#3570,.T.) ;
#43938=EDGE_CURVE('',#35915,#35924,#3571,.T.) ;
#43939=EDGE_CURVE('',#35923,#35916,#3572,.T.) ;
#43940=EDGE_CURVE('',#36129,#36130,#3573,.T.) ;
#43941=EDGE_CURVE('',#36130,#36131,#3574,.T.) ;
#43942=EDGE_CURVE('',#36131,#36132,#3575,.T.) ;
#43943=EDGE_CURVE('',#36132,#36129,#3576,.T.) ;
#43944=EDGE_CURVE('',#36133,#36134,#3577,.T.) ;
#43945=EDGE_CURVE('',#36134,#36135,#3578,.T.) ;
#43946=EDGE_CURVE('',#36135,#36136,#3579,.T.) ;
#43947=EDGE_CURVE('',#36136,#36133,#3580,.T.) ;
#43948=EDGE_CURVE('',#36137,#36138,#3581,.T.) ;
#43949=EDGE_CURVE('',#36138,#36139,#3582,.T.) ;
#43950=EDGE_CURVE('',#36139,#36140,#3583,.T.) ;
#43951=EDGE_CURVE('',#36140,#36137,#3584,.T.) ;
#43952=EDGE_CURVE('',#36141,#36142,#3585,.T.) ;
#43953=EDGE_CURVE('',#36142,#36143,#3586,.T.) ;
#43954=EDGE_CURVE('',#36143,#36144,#3587,.T.) ;
#43955=EDGE_CURVE('',#36144,#36141,#3588,.T.) ;
#43956=EDGE_CURVE('',#36145,#36146,#3589,.T.) ;
#43957=EDGE_CURVE('',#36146,#36147,#3590,.T.) ;
#43958=EDGE_CURVE('',#36147,#36148,#3591,.T.) ;
#43959=EDGE_CURVE('',#36148,#36145,#3592,.T.) ;
#43960=EDGE_CURVE('',#36149,#36150,#3593,.T.) ;
#43961=EDGE_CURVE('',#36151,#36149,#29604,.T.) ;
#43962=EDGE_CURVE('',#36152,#36151,#3594,.T.) ;
#43963=EDGE_CURVE('',#36153,#36152,#29605,.T.) ;
#43964=EDGE_CURVE('',#36154,#36153,#3595,.T.) ;
#43965=EDGE_CURVE('',#36155,#36154,#29606,.T.) ;
#43966=EDGE_CURVE('',#36156,#36155,#3596,.T.) ;
#43967=EDGE_CURVE('',#36150,#36156,#29607,.T.) ;
#43968=EDGE_CURVE('',#36156,#36157,#3597,.T.) ;
#43969=EDGE_CURVE('',#36157,#36158,#29608,.T.) ;
#43970=EDGE_CURVE('',#36150,#36158,#3598,.T.) ;
#43971=EDGE_CURVE('',#36158,#36159,#3599,.T.) ;
#43972=EDGE_CURVE('',#36149,#36159,#3600,.T.) ;
#43973=EDGE_CURVE('',#36159,#36160,#29609,.T.) ;
#43974=EDGE_CURVE('',#36151,#36160,#3601,.T.) ;
#43975=EDGE_CURVE('',#36160,#36161,#3602,.T.) ;
#43976=EDGE_CURVE('',#36152,#36161,#3603,.T.) ;
#43977=EDGE_CURVE('',#36161,#36162,#29610,.T.) ;
#43978=EDGE_CURVE('',#36153,#36162,#3604,.T.) ;
#43979=EDGE_CURVE('',#36162,#36163,#3605,.T.) ;
#43980=EDGE_CURVE('',#36154,#36163,#3606,.T.) ;
#43981=EDGE_CURVE('',#36163,#36164,#29611,.T.) ;
#43982=EDGE_CURVE('',#36155,#36164,#3607,.T.) ;
#43983=EDGE_CURVE('',#36164,#36157,#3608,.T.) ;
#43984=EDGE_CURVE('',#36165,#36166,#3609,.T.) ;
#43985=EDGE_CURVE('',#36166,#36167,#3610,.T.) ;
#43986=EDGE_CURVE('',#36167,#36168,#3611,.T.) ;
#43987=EDGE_CURVE('',#36168,#36165,#3612,.T.) ;
#43988=EDGE_CURVE('',#35908,#35884,#3613,.T.) ;
#43989=EDGE_CURVE('',#35884,#36169,#3614,.T.) ;
#43990=EDGE_CURVE('',#36169,#36170,#3615,.T.) ;
#43991=EDGE_CURVE('',#36170,#35908,#3616,.T.) ;
#43992=EDGE_CURVE('',#36171,#35905,#3617,.T.) ;
#43993=EDGE_CURVE('',#35898,#36172,#3618,.T.) ;
#43994=EDGE_CURVE('',#36172,#36171,#3619,.T.) ;
#43995=EDGE_CURVE('',#35906,#36173,#3620,.T.) ;
#43996=EDGE_CURVE('',#36173,#35902,#3621,.T.) ;
#43997=EDGE_CURVE('',#35902,#35899,#3622,.T.) ;
#43998=EDGE_CURVE('',#35883,#36174,#3623,.T.) ;
#43999=EDGE_CURVE('',#36174,#36175,#29612,.T.) ;
#44000=EDGE_CURVE('',#36175,#36176,#3624,.T.) ;
#44001=EDGE_CURVE('',#36176,#36177,#3625,.T.) ;
#44002=EDGE_CURVE('',#36177,#35882,#3626,.T.) ;
#44003=EDGE_CURVE('',#36178,#36179,#29613,.T.) ;
#44004=EDGE_CURVE('',#36179,#36180,#29614,.T.) ;
#44005=EDGE_CURVE('',#36180,#36181,#29615,.T.) ;
#44006=EDGE_CURVE('',#36181,#36182,#3627,.T.) ;
#44007=EDGE_CURVE('',#36182,#36183,#29616,.T.) ;
#44008=EDGE_CURVE('',#36183,#36178,#3628,.T.) ;
#44009=EDGE_CURVE('',#36087,#36009,#29617,.T.) ;
#44010=EDGE_CURVE('',#36055,#36087,#2143,.T.) ;
#44011=EDGE_CURVE('',#36010,#36055,#29618,.T.) ;
#44012=EDGE_CURVE('',#36077,#36057,#29619,.T.) ;
#44013=EDGE_CURVE('',#36091,#36058,#29620,.T.) ;
#44014=EDGE_CURVE('',#36077,#36091,#349,.T.) ;
#44015=EDGE_CURVE('',#36092,#36064,#29621,.T.) ;
#44016=EDGE_CURVE('',#36056,#36092,#29622,.T.) ;
#44017=EDGE_CURVE('',#36011,#36054,#29623,.T.) ;
#44018=EDGE_CURVE('',#36088,#36008,#29624,.T.) ;
#44019=EDGE_CURVE('',#36078,#36090,#350,.T.) ;
#44020=EDGE_CURVE('',#36073,#36078,#29625,.T.) ;
#44021=EDGE_CURVE('',#36056,#36064,#29626,.T.) ;
#44022=EDGE_CURVE('',#36085,#36054,#351,.T.) ;
#44023=EDGE_CURVE('',#36012,#36085,#29627,.T.) ;
#44024=EDGE_CURVE('',#36050,#36015,#29628,.T.) ;
#44025=EDGE_CURVE('',#36088,#36050,#2144,.T.) ;
#44026=EDGE_CURVE('',#36074,#36090,#29629,.T.) ;
#44027=EDGE_CURVE('',#36053,#36063,#29630,.T.) ;
#44028=EDGE_CURVE('',#36086,#36053,#29631,.T.) ;
#44029=EDGE_CURVE('',#36013,#36084,#29632,.T.) ;
#44030=EDGE_CURVE('',#36051,#36014,#29633,.T.) ;
#44031=EDGE_CURVE('',#36089,#36049,#29634,.T.) ;
#44032=EDGE_CURVE('',#36075,#36089,#29635,.T.) ;
#44033=EDGE_CURVE('',#36086,#36063,#29636,.T.) ;
#44034=EDGE_CURVE('',#36051,#36084,#352,.T.) ;
#44035=EDGE_CURVE('',#36075,#36049,#29637,.T.) ;
#44036=EDGE_CURVE('',#36061,#36080,#29638,.T.) ;
#44037=EDGE_CURVE('',#36081,#36062,#29639,.T.) ;
#44038=EDGE_CURVE('',#36052,#36083,#29640,.T.) ;
#44039=EDGE_CURVE('',#36076,#36052,#29641,.T.) ;
#44040=EDGE_CURVE('',#36081,#36080,#353,.T.) ;
#44041=EDGE_CURVE('',#36076,#36083,#29642,.T.) ;
#44042=EDGE_CURVE('',#36082,#36079,#354,.T.) ;
#44043=EDGE_CURVE('',#36072,#36082,#29643,.T.) ;
#44044=EDGE_CURVE('',#36071,#36079,#29644,.T.) ;
#44045=EDGE_CURVE('',#35938,#36184,#355,.T.) ;
#44046=EDGE_CURVE('',#36184,#35885,#2145,.T.) ;
#44047=EDGE_CURVE('',#36169,#36171,#29645,.T.) ;
#44048=EDGE_CURVE('',#36170,#36172,#29646,.T.) ;
#44049=EDGE_CURVE('',#35947,#36170,#29647,.T.) ;
#44050=EDGE_CURVE('',#35955,#36174,#2146,.T.) ;
#44051=EDGE_CURVE('',#35883,#35956,#2147,.T.) ;
#44052=EDGE_CURVE('',#36176,#35905,#29648,.T.) ;
#44053=EDGE_CURVE('',#36171,#36177,#29649,.T.) ;
#44054=EDGE_CURVE('',#35948,#36172,#29650,.T.) ;
#44055=EDGE_CURVE('',#36185,#36186,#2148,.T.) ;
#44056=EDGE_CURVE('',#36186,#35949,#356,.T.) ;
#44057=EDGE_CURVE('',#36173,#36185,#29651,.T.) ;
#44058=EDGE_CURVE('',#36160,#36165,#29652,.T.) ;
#44059=EDGE_CURVE('',#36165,#36159,#29653,.T.) ;
#44060=EDGE_CURVE('',#36166,#36158,#29654,.T.) ;
#44061=EDGE_CURVE('',#36161,#36168,#29655,.T.) ;
#44062=EDGE_CURVE('',#36166,#36157,#29656,.T.) ;
#44063=EDGE_CURVE('',#36162,#36168,#29657,.T.) ;
#44064=EDGE_CURVE('',#36167,#36164,#29658,.T.) ;
#44065=EDGE_CURVE('',#36163,#36167,#29659,.T.) ;
#44066=EDGE_CURVE('',#36026,#36096,#29660,.T.) ;
#44067=EDGE_CURVE('',#36093,#36025,#29661,.T.) ;
#44068=EDGE_CURVE('',#36108,#36024,#29662,.T.) ;
#44069=EDGE_CURVE('',#36093,#36108,#29663,.T.) ;
#44070=EDGE_CURVE('',#36100,#36096,#29664,.T.) ;
#44071=EDGE_CURVE('',#36027,#36100,#29665,.T.) ;
#44072=EDGE_CURVE('',#36105,#36023,#29666,.T.) ;
#44073=EDGE_CURVE('',#36094,#36107,#29667,.T.) ;
#44074=EDGE_CURVE('',#36095,#36112,#29668,.T.) ;
#44075=EDGE_CURVE('',#36109,#36094,#29669,.T.) ;
#44076=EDGE_CURVE('',#36097,#36095,#29670,.T.) ;
#44077=EDGE_CURVE('',#36021,#36099,#29671,.T.) ;
#44078=EDGE_CURVE('',#36022,#36103,#29672,.T.) ;
#44079=EDGE_CURVE('',#36104,#36020,#29673,.T.) ;
#44080=EDGE_CURVE('',#36105,#36103,#29674,.T.) ;
#44081=EDGE_CURVE('',#36109,#36107,#29675,.T.) ;
#44082=EDGE_CURVE('',#36097,#36112,#29676,.T.) ;
#44083=EDGE_CURVE('',#36104,#36099,#29677,.T.) ;
#44084=EDGE_CURVE('',#36106,#36102,#29678,.T.) ;
#44085=EDGE_CURVE('',#36110,#36106,#29679,.T.) ;
#44086=EDGE_CURVE('',#36098,#36111,#29680,.T.) ;
#44087=EDGE_CURVE('',#36101,#36098,#29681,.T.) ;
#44088=EDGE_CURVE('',#36110,#36102,#29682,.T.) ;
#44089=EDGE_CURVE('',#36101,#36111,#29683,.T.) ;
#44090=EDGE_CURVE('',#35994,#36140,#29684,.T.) ;
#44091=EDGE_CURVE('',#36137,#35993,#29685,.T.) ;
#44092=EDGE_CURVE('',#36136,#35992,#29686,.T.) ;
#44093=EDGE_CURVE('',#36137,#36136,#29687,.T.) ;
#44094=EDGE_CURVE('',#36144,#36140,#29688,.T.) ;
#44095=EDGE_CURVE('',#35995,#36144,#29689,.T.) ;
#44096=EDGE_CURVE('',#36133,#35991,#29690,.T.) ;
#44097=EDGE_CURVE('',#36138,#36135,#29691,.T.) ;
#44098=EDGE_CURVE('',#36139,#36148,#29692,.T.) ;
#44099=EDGE_CURVE('',#36145,#36138,#29693,.T.) ;
#44100=EDGE_CURVE('',#36141,#36139,#29694,.T.) ;
#44101=EDGE_CURVE('',#35989,#36143,#29695,.T.) ;
#44102=EDGE_CURVE('',#35990,#36131,#29696,.T.) ;
#44103=EDGE_CURVE('',#36132,#35988,#29697,.T.) ;
#44104=EDGE_CURVE('',#36133,#36131,#29698,.T.) ;
#44105=EDGE_CURVE('',#36145,#36135,#29699,.T.) ;
#44106=EDGE_CURVE('',#36141,#36148,#29700,.T.) ;
#44107=EDGE_CURVE('',#36132,#36143,#29701,.T.) ;
#44108=EDGE_CURVE('',#36134,#36130,#29702,.T.) ;
#44109=EDGE_CURVE('',#36146,#36134,#29703,.T.) ;
#44110=EDGE_CURVE('',#36142,#36147,#29704,.T.) ;
#44111=EDGE_CURVE('',#36129,#36142,#29705,.T.) ;
#44112=EDGE_CURVE('',#36146,#36130,#29706,.T.) ;
#44113=EDGE_CURVE('',#36129,#36147,#29707,.T.) ;
#44114=EDGE_CURVE('',#36043,#36179,#2149,.T.) ;
#44115=EDGE_CURVE('',#36044,#36178,#29708,.T.) ;
#44116=EDGE_CURVE('',#35934,#36044,#29709,.T.) ;
#44117=EDGE_CURVE('',#35934,#36178,#29710,.T.) ;
#44118=EDGE_CURVE('',#35935,#36183,#29711,.T.) ;
#44119=EDGE_CURVE('',#35941,#35935,#29712,.T.) ;
#44120=EDGE_CURVE('',#35942,#36183,#29713,.T.) ;
#44121=EDGE_CURVE('',#35943,#36182,#29714,.T.) ;
#44122=EDGE_CURVE('',#36045,#35944,#29715,.T.) ;
#44123=EDGE_CURVE('',#36045,#36182,#29716,.T.) ;
#44124=EDGE_CURVE('',#36046,#36181,#29717,.T.) ;
#44125=EDGE_CURVE('',#35928,#36046,#29718,.T.) ;
#44126=EDGE_CURVE('',#35928,#36181,#29719,.T.) ;
#44127=EDGE_CURVE('',#36180,#35929,#2150,.T.) ;
#44128=EDGE_CURVE('',#35906,#36176,#29720,.T.) ;
#44129=EDGE_CURVE('',#36173,#36175,#29721,.T.) ;
#44130=EDGE_CURVE('',#36185,#36174,#29722,.T.) ;
#44131=EDGE_CURVE('',#36186,#35955,#29723,.T.) ;
#44132=EDGE_CURVE('',#35949,#35954,#29724,.T.) ;
#44133=EDGE_CURVE('',#35938,#35957,#29725,.T.) ;
#44134=EDGE_CURVE('',#36184,#35956,#29726,.T.) ;
#44135=EDGE_CURVE('',#36169,#36177,#29727,.T.) ;
#44136=EDGE_CURVE('',#36187,#36188,#2151,.T.) ;
#44137=EDGE_CURVE('',#36188,#36180,#2152,.T.) ;
#44138=EDGE_CURVE('',#36179,#36189,#2153,.T.) ;
#44139=EDGE_CURVE('',#36189,#36187,#2154,.T.) ;
#44140=EDGE_CURVE('',#36043,#36036,#29728,.T.) ;
#44141=EDGE_CURVE('',#36035,#36179,#2155,.T.) ;
#44142=EDGE_CURVE('',#36032,#35929,#29729,.T.) ;
#44143=EDGE_CURVE('',#36180,#36033,#2156,.T.) ;
#44144=EDGE_CURVE('',#36189,#36035,#29730,.T.) ;
#44145=EDGE_CURVE('',#36187,#36034,#29731,.T.) ;
#44146=EDGE_CURVE('',#36188,#36033,#29732,.T.) ;
#54031=ORIENTED_EDGE('',*,*,#41593,.F.) ;
#54032=ORIENTED_EDGE('',*,*,#41594,.F.) ;
#54033=ORIENTED_EDGE('',*,*,#41595,.F.) ;
#54034=ORIENTED_EDGE('',*,*,#41596,.T.) ;
#54035=ORIENTED_EDGE('',*,*,#41597,.F.) ;
#54036=ORIENTED_EDGE('',*,*,#41598,.T.) ;
#54037=ORIENTED_EDGE('',*,*,#41599,.F.) ;
#54038=ORIENTED_EDGE('',*,*,#41600,.F.) ;
#54039=ORIENTED_EDGE('',*,*,#41598,.F.) ;
#54040=ORIENTED_EDGE('',*,*,#41601,.F.) ;
#54041=ORIENTED_EDGE('',*,*,#41602,.T.) ;
#54042=ORIENTED_EDGE('',*,*,#41603,.F.) ;
#54043=ORIENTED_EDGE('',*,*,#41602,.F.) ;
#54044=ORIENTED_EDGE('',*,*,#41604,.F.) ;
#54045=ORIENTED_EDGE('',*,*,#41605,.T.) ;
#54046=ORIENTED_EDGE('',*,*,#41606,.F.) ;
#54047=ORIENTED_EDGE('',*,*,#41607,.F.) ;
#54048=ORIENTED_EDGE('',*,*,#41605,.F.) ;
#54049=ORIENTED_EDGE('',*,*,#41608,.T.) ;
#54050=ORIENTED_EDGE('',*,*,#41609,.F.) ;
#54051=ORIENTED_EDGE('',*,*,#41610,.T.) ;
#54052=ORIENTED_EDGE('',*,*,#41611,.T.) ;
#54053=ORIENTED_EDGE('',*,*,#41612,.T.) ;
#54054=ORIENTED_EDGE('',*,*,#41613,.T.) ;
#54055=ORIENTED_EDGE('',*,*,#41614,.F.) ;
#54056=ORIENTED_EDGE('',*,*,#41608,.F.) ;
#54057=ORIENTED_EDGE('',*,*,#41615,.F.) ;
#54058=ORIENTED_EDGE('',*,*,#41616,.T.) ;
#54059=ORIENTED_EDGE('',*,*,#41617,.F.) ;
#54060=ORIENTED_EDGE('',*,*,#41618,.F.) ;
#54061=ORIENTED_EDGE('',*,*,#41619,.T.) ;
#54062=ORIENTED_EDGE('',*,*,#41620,.F.) ;
#54063=ORIENTED_EDGE('',*,*,#41621,.F.) ;
#54064=ORIENTED_EDGE('',*,*,#41622,.T.) ;
#54065=ORIENTED_EDGE('',*,*,#41601,.T.) ;
#54066=ORIENTED_EDGE('',*,*,#41622,.F.) ;
#54067=ORIENTED_EDGE('',*,*,#41603,.T.) ;
#54068=ORIENTED_EDGE('',*,*,#41623,.T.) ;
#54069=ORIENTED_EDGE('',*,*,#41606,.T.) ;
#54070=ORIENTED_EDGE('',*,*,#41607,.T.) ;
#54071=ORIENTED_EDGE('',*,*,#41623,.F.) ;
#54072=ORIENTED_EDGE('',*,*,#41624,.F.) ;
#54073=ORIENTED_EDGE('',*,*,#41625,.T.) ;
#54074=ORIENTED_EDGE('',*,*,#41626,.F.) ;
#54075=ORIENTED_EDGE('',*,*,#41627,.T.) ;
#54076=ORIENTED_EDGE('',*,*,#41628,.F.) ;
#54077=ORIENTED_EDGE('',*,*,#41629,.T.) ;
#54078=ORIENTED_EDGE('',*,*,#41630,.T.) ;
#54079=ORIENTED_EDGE('',*,*,#41631,.T.) ;
#54080=ORIENTED_EDGE('',*,*,#41632,.F.) ;
#54081=ORIENTED_EDGE('',*,*,#41633,.T.) ;
#54082=ORIENTED_EDGE('',*,*,#41634,.F.) ;
#54083=ORIENTED_EDGE('',*,*,#41635,.T.) ;
#54084=ORIENTED_EDGE('',*,*,#41636,.F.) ;
#54085=ORIENTED_EDGE('',*,*,#41637,.T.) ;
#54086=ORIENTED_EDGE('',*,*,#41638,.T.) ;
#54087=ORIENTED_EDGE('',*,*,#41639,.T.) ;
#54088=ORIENTED_EDGE('',*,*,#41640,.F.) ;
#54089=ORIENTED_EDGE('',*,*,#41641,.T.) ;
#54090=ORIENTED_EDGE('',*,*,#41599,.T.) ;
#54091=ORIENTED_EDGE('',*,*,#41600,.T.) ;
#54092=ORIENTED_EDGE('',*,*,#41641,.F.) ;
#54093=ORIENTED_EDGE('',*,*,#41642,.F.) ;
#54094=ORIENTED_EDGE('',*,*,#41643,.F.) ;
#54095=ORIENTED_EDGE('',*,*,#41644,.F.) ;
#54096=ORIENTED_EDGE('',*,*,#41645,.T.) ;
#54097=ORIENTED_EDGE('',*,*,#41646,.F.) ;
#54098=ORIENTED_EDGE('',*,*,#41647,.F.) ;
#54099=ORIENTED_EDGE('',*,*,#41648,.F.) ;
#54100=ORIENTED_EDGE('',*,*,#41649,.F.) ;
#54101=ORIENTED_EDGE('',*,*,#41650,.F.) ;
#54102=ORIENTED_EDGE('',*,*,#41651,.T.) ;
#54103=ORIENTED_EDGE('',*,*,#41652,.F.) ;
#54104=ORIENTED_EDGE('',*,*,#41653,.F.) ;
#54105=ORIENTED_EDGE('',*,*,#41651,.F.) ;
#54106=ORIENTED_EDGE('',*,*,#41654,.F.) ;
#54107=ORIENTED_EDGE('',*,*,#41655,.T.) ;
#54108=ORIENTED_EDGE('',*,*,#41656,.F.) ;
#54109=ORIENTED_EDGE('',*,*,#41655,.F.) ;
#54110=ORIENTED_EDGE('',*,*,#41657,.F.) ;
#54111=ORIENTED_EDGE('',*,*,#41658,.T.) ;
#54112=ORIENTED_EDGE('',*,*,#41659,.F.) ;
#54113=ORIENTED_EDGE('',*,*,#41660,.F.) ;
#54114=ORIENTED_EDGE('',*,*,#41658,.F.) ;
#54115=ORIENTED_EDGE('',*,*,#41661,.T.) ;
#54116=ORIENTED_EDGE('',*,*,#41662,.F.) ;
#54117=ORIENTED_EDGE('',*,*,#41663,.T.) ;
#54118=ORIENTED_EDGE('',*,*,#41664,.T.) ;
#54119=ORIENTED_EDGE('',*,*,#41665,.T.) ;
#54120=ORIENTED_EDGE('',*,*,#41666,.T.) ;
#54121=ORIENTED_EDGE('',*,*,#41667,.F.) ;
#54122=ORIENTED_EDGE('',*,*,#41661,.F.) ;
#54123=ORIENTED_EDGE('',*,*,#41668,.F.) ;
#54124=ORIENTED_EDGE('',*,*,#41669,.T.) ;
#54125=ORIENTED_EDGE('',*,*,#41670,.F.) ;
#54126=ORIENTED_EDGE('',*,*,#41671,.F.) ;
#54127=ORIENTED_EDGE('',*,*,#41672,.T.) ;
#54128=ORIENTED_EDGE('',*,*,#41673,.F.) ;
#54129=ORIENTED_EDGE('',*,*,#41674,.F.) ;
#54130=ORIENTED_EDGE('',*,*,#41675,.T.) ;
#54131=ORIENTED_EDGE('',*,*,#41654,.T.) ;
#54132=ORIENTED_EDGE('',*,*,#41675,.F.) ;
#54133=ORIENTED_EDGE('',*,*,#41656,.T.) ;
#54134=ORIENTED_EDGE('',*,*,#41676,.T.) ;
#54135=ORIENTED_EDGE('',*,*,#41659,.T.) ;
#54136=ORIENTED_EDGE('',*,*,#41660,.T.) ;
#54137=ORIENTED_EDGE('',*,*,#41676,.F.) ;
#54138=ORIENTED_EDGE('',*,*,#41677,.F.) ;
#54139=ORIENTED_EDGE('',*,*,#41678,.T.) ;
#54140=ORIENTED_EDGE('',*,*,#41679,.F.) ;
#54141=ORIENTED_EDGE('',*,*,#41680,.T.) ;
#54142=ORIENTED_EDGE('',*,*,#41681,.F.) ;
#54143=ORIENTED_EDGE('',*,*,#41682,.T.) ;
#54144=ORIENTED_EDGE('',*,*,#41683,.T.) ;
#54145=ORIENTED_EDGE('',*,*,#41684,.T.) ;
#54146=ORIENTED_EDGE('',*,*,#41685,.F.) ;
#54147=ORIENTED_EDGE('',*,*,#41686,.T.) ;
#54148=ORIENTED_EDGE('',*,*,#41687,.F.) ;
#54149=ORIENTED_EDGE('',*,*,#41688,.T.) ;
#54150=ORIENTED_EDGE('',*,*,#41689,.F.) ;
#54151=ORIENTED_EDGE('',*,*,#41690,.T.) ;
#54152=ORIENTED_EDGE('',*,*,#41691,.T.) ;
#54153=ORIENTED_EDGE('',*,*,#41692,.T.) ;
#54154=ORIENTED_EDGE('',*,*,#41693,.F.) ;
#54155=ORIENTED_EDGE('',*,*,#41694,.T.) ;
#54156=ORIENTED_EDGE('',*,*,#41652,.T.) ;
#54157=ORIENTED_EDGE('',*,*,#41653,.T.) ;
#54158=ORIENTED_EDGE('',*,*,#41694,.F.) ;
#54159=ORIENTED_EDGE('',*,*,#41695,.T.) ;
#54160=ORIENTED_EDGE('',*,*,#41696,.T.) ;
#54161=ORIENTED_EDGE('',*,*,#41697,.F.) ;
#54162=ORIENTED_EDGE('',*,*,#41698,.T.) ;
#54163=ORIENTED_EDGE('',*,*,#41699,.F.) ;
#54164=ORIENTED_EDGE('',*,*,#41700,.T.) ;
#54165=ORIENTED_EDGE('',*,*,#41701,.F.) ;
#54166=ORIENTED_EDGE('',*,*,#41702,.T.) ;
#54167=ORIENTED_EDGE('',*,*,#41703,.F.) ;
#54168=ORIENTED_EDGE('',*,*,#41704,.T.) ;
#54169=ORIENTED_EDGE('',*,*,#41705,.F.) ;
#54170=ORIENTED_EDGE('',*,*,#41706,.T.) ;
#54171=ORIENTED_EDGE('',*,*,#41707,.F.) ;
#54172=ORIENTED_EDGE('',*,*,#41708,.T.) ;
#54173=ORIENTED_EDGE('',*,*,#41709,.T.) ;
#54174=ORIENTED_EDGE('',*,*,#41710,.T.) ;
#54175=ORIENTED_EDGE('',*,*,#41711,.F.) ;
#54176=ORIENTED_EDGE('',*,*,#41712,.T.) ;
#54177=ORIENTED_EDGE('',*,*,#41713,.T.) ;
#54178=ORIENTED_EDGE('',*,*,#41714,.T.) ;
#54179=ORIENTED_EDGE('',*,*,#41715,.F.) ;
#54180=ORIENTED_EDGE('',*,*,#41716,.T.) ;
#54181=ORIENTED_EDGE('',*,*,#41717,.T.) ;
#54182=ORIENTED_EDGE('',*,*,#41718,.T.) ;
#54183=ORIENTED_EDGE('',*,*,#41719,.F.) ;
#54184=ORIENTED_EDGE('',*,*,#41720,.T.) ;
#54185=ORIENTED_EDGE('',*,*,#41718,.F.) ;
#54186=ORIENTED_EDGE('',*,*,#41721,.F.) ;
#54187=ORIENTED_EDGE('',*,*,#41722,.F.) ;
#54188=ORIENTED_EDGE('',*,*,#41714,.F.) ;
#54189=ORIENTED_EDGE('',*,*,#41723,.F.) ;
#54190=ORIENTED_EDGE('',*,*,#41716,.F.) ;
#54191=ORIENTED_EDGE('',*,*,#41724,.F.) ;
#54192=ORIENTED_EDGE('',*,*,#41710,.F.) ;
#54193=ORIENTED_EDGE('',*,*,#41725,.F.) ;
#54194=ORIENTED_EDGE('',*,*,#41712,.F.) ;
#54195=ORIENTED_EDGE('',*,*,#41708,.F.) ;
#54196=ORIENTED_EDGE('',*,*,#41726,.T.) ;
#54197=ORIENTED_EDGE('',*,*,#41727,.T.) ;
#54198=ORIENTED_EDGE('',*,*,#41728,.F.) ;
#54199=ORIENTED_EDGE('',*,*,#41729,.F.) ;
#54200=ORIENTED_EDGE('',*,*,#41730,.F.) ;
#54201=ORIENTED_EDGE('',*,*,#41731,.T.) ;
#54202=ORIENTED_EDGE('',*,*,#41732,.T.) ;
#54203=ORIENTED_EDGE('',*,*,#41733,.T.) ;
#54204=ORIENTED_EDGE('',*,*,#41734,.T.) ;
#54205=ORIENTED_EDGE('',*,*,#41735,.F.) ;
#54206=ORIENTED_EDGE('',*,*,#41736,.T.) ;
#54207=ORIENTED_EDGE('',*,*,#41737,.T.) ;
#54208=ORIENTED_EDGE('',*,*,#41738,.T.) ;
#54209=ORIENTED_EDGE('',*,*,#41739,.T.) ;
#54210=ORIENTED_EDGE('',*,*,#41740,.T.) ;
#54211=ORIENTED_EDGE('',*,*,#41741,.T.) ;
#54212=ORIENTED_EDGE('',*,*,#41742,.T.) ;
#54213=ORIENTED_EDGE('',*,*,#41677,.T.) ;
#54214=ORIENTED_EDGE('',*,*,#41693,.T.) ;
#54215=ORIENTED_EDGE('',*,*,#41743,.T.) ;
#54216=ORIENTED_EDGE('',*,*,#41744,.T.) ;
#54217=ORIENTED_EDGE('',*,*,#41745,.T.) ;
#54218=ORIENTED_EDGE('',*,*,#41746,.F.) ;
#54219=ORIENTED_EDGE('',*,*,#41747,.T.) ;
#54220=ORIENTED_EDGE('',*,*,#41748,.F.) ;
#54221=ORIENTED_EDGE('',*,*,#41749,.T.) ;
#54222=ORIENTED_EDGE('',*,*,#41750,.F.) ;
#54223=ORIENTED_EDGE('',*,*,#41751,.T.) ;
#54224=ORIENTED_EDGE('',*,*,#41752,.F.) ;
#54225=ORIENTED_EDGE('',*,*,#41753,.T.) ;
#54226=ORIENTED_EDGE('',*,*,#41754,.F.) ;
#54227=ORIENTED_EDGE('',*,*,#41755,.T.) ;
#54228=ORIENTED_EDGE('',*,*,#41756,.T.) ;
#54229=ORIENTED_EDGE('',*,*,#41757,.T.) ;
#54230=ORIENTED_EDGE('',*,*,#41758,.T.) ;
#54231=ORIENTED_EDGE('',*,*,#41759,.F.) ;
#54232=ORIENTED_EDGE('',*,*,#41760,.T.) ;
#54233=ORIENTED_EDGE('',*,*,#41610,.F.) ;
#54234=ORIENTED_EDGE('',*,*,#41761,.T.) ;
#54235=ORIENTED_EDGE('',*,*,#41762,.T.) ;
#54236=ORIENTED_EDGE('',*,*,#41763,.T.) ;
#54237=ORIENTED_EDGE('',*,*,#41764,.F.) ;
#54238=ORIENTED_EDGE('',*,*,#41765,.T.) ;
#54239=ORIENTED_EDGE('',*,*,#41663,.F.) ;
#54240=ORIENTED_EDGE('',*,*,#41604,.T.) ;
#54241=ORIENTED_EDGE('',*,*,#41657,.T.) ;
#54242=ORIENTED_EDGE('',*,*,#41766,.T.) ;
#54243=ORIENTED_EDGE('',*,*,#41767,.T.) ;
#54244=ORIENTED_EDGE('',*,*,#41768,.F.) ;
#54245=ORIENTED_EDGE('',*,*,#41769,.T.) ;
#54246=ORIENTED_EDGE('',*,*,#41770,.F.) ;
#54247=ORIENTED_EDGE('',*,*,#41771,.T.) ;
#54248=ORIENTED_EDGE('',*,*,#41772,.T.) ;
#54249=ORIENTED_EDGE('',*,*,#41773,.T.) ;
#54250=ORIENTED_EDGE('',*,*,#41774,.T.) ;
#54251=ORIENTED_EDGE('',*,*,#41775,.T.) ;
#54252=ORIENTED_EDGE('',*,*,#41776,.T.) ;
#54253=ORIENTED_EDGE('',*,*,#41777,.T.) ;
#54254=ORIENTED_EDGE('',*,*,#41778,.T.) ;
#54255=ORIENTED_EDGE('',*,*,#41779,.T.) ;
#54256=ORIENTED_EDGE('',*,*,#41780,.T.) ;
#54257=ORIENTED_EDGE('',*,*,#41781,.T.) ;
#54258=ORIENTED_EDGE('',*,*,#41782,.T.) ;
#54259=ORIENTED_EDGE('',*,*,#41783,.T.) ;
#54260=ORIENTED_EDGE('',*,*,#41729,.T.) ;
#54261=ORIENTED_EDGE('',*,*,#41784,.F.) ;
#54262=ORIENTED_EDGE('',*,*,#41719,.T.) ;
#54263=ORIENTED_EDGE('',*,*,#41785,.T.) ;
#54264=ORIENTED_EDGE('',*,*,#41786,.T.) ;
#54265=ORIENTED_EDGE('',*,*,#41787,.F.) ;
#54266=ORIENTED_EDGE('',*,*,#41727,.F.) ;
#54267=ORIENTED_EDGE('',*,*,#41788,.F.) ;
#54268=ORIENTED_EDGE('',*,*,#41789,.T.) ;
#54269=ORIENTED_EDGE('',*,*,#41790,.T.) ;
#54270=ORIENTED_EDGE('',*,*,#41791,.T.) ;
#54271=ORIENTED_EDGE('',*,*,#41792,.F.) ;
#54272=ORIENTED_EDGE('',*,*,#41793,.F.) ;
#54273=ORIENTED_EDGE('',*,*,#41794,.T.) ;
#54274=ORIENTED_EDGE('',*,*,#41795,.F.) ;
#54275=ORIENTED_EDGE('',*,*,#41796,.T.) ;
#54276=ORIENTED_EDGE('',*,*,#41797,.F.) ;
#54277=ORIENTED_EDGE('',*,*,#41798,.T.) ;
#54278=ORIENTED_EDGE('',*,*,#41799,.F.) ;
#54279=ORIENTED_EDGE('',*,*,#41800,.T.) ;
#54280=ORIENTED_EDGE('',*,*,#41597,.T.) ;
#54281=ORIENTED_EDGE('',*,*,#41801,.F.) ;
#54282=ORIENTED_EDGE('',*,*,#41802,.T.) ;
#54283=ORIENTED_EDGE('',*,*,#41803,.F.) ;
#54284=ORIENTED_EDGE('',*,*,#41804,.T.) ;
#54285=ORIENTED_EDGE('',*,*,#41805,.F.) ;
#54286=ORIENTED_EDGE('',*,*,#41806,.T.) ;
#54287=ORIENTED_EDGE('',*,*,#41807,.F.) ;
#54288=ORIENTED_EDGE('',*,*,#41808,.T.) ;
#54289=ORIENTED_EDGE('',*,*,#41650,.T.) ;
#54290=ORIENTED_EDGE('',*,*,#41809,.T.) ;
#54291=ORIENTED_EDGE('',*,*,#41810,.T.) ;
#54292=ORIENTED_EDGE('',*,*,#41811,.T.) ;
#54293=ORIENTED_EDGE('',*,*,#41812,.F.) ;
#54294=ORIENTED_EDGE('',*,*,#41813,.T.) ;
#54295=ORIENTED_EDGE('',*,*,#41814,.T.) ;
#54296=ORIENTED_EDGE('',*,*,#41649,.T.) ;
#54297=ORIENTED_EDGE('',*,*,#41815,.F.) ;
#54298=ORIENTED_EDGE('',*,*,#41647,.T.) ;
#54299=ORIENTED_EDGE('',*,*,#41816,.T.) ;
#54300=ORIENTED_EDGE('',*,*,#41817,.T.) ;
#54301=ORIENTED_EDGE('',*,*,#41818,.F.) ;
#54302=ORIENTED_EDGE('',*,*,#41819,.T.) ;
#54303=ORIENTED_EDGE('',*,*,#41820,.T.) ;
#54304=ORIENTED_EDGE('',*,*,#41821,.T.) ;
#54305=ORIENTED_EDGE('',*,*,#41822,.F.) ;
#54306=ORIENTED_EDGE('',*,*,#41823,.T.) ;
#54307=ORIENTED_EDGE('',*,*,#41824,.T.) ;
#54308=ORIENTED_EDGE('',*,*,#41825,.T.) ;
#54309=ORIENTED_EDGE('',*,*,#41826,.F.) ;
#54310=ORIENTED_EDGE('',*,*,#41827,.T.) ;
#54311=ORIENTED_EDGE('',*,*,#41828,.F.) ;
#54312=ORIENTED_EDGE('',*,*,#41829,.T.) ;
#54313=ORIENTED_EDGE('',*,*,#41830,.T.) ;
#54314=ORIENTED_EDGE('',*,*,#41831,.T.) ;
#54315=ORIENTED_EDGE('',*,*,#41832,.T.) ;
#54316=ORIENTED_EDGE('',*,*,#41833,.T.) ;
#54317=ORIENTED_EDGE('',*,*,#41834,.F.) ;
#54318=ORIENTED_EDGE('',*,*,#41835,.T.) ;
#54319=ORIENTED_EDGE('',*,*,#41836,.F.) ;
#54320=ORIENTED_EDGE('',*,*,#41837,.T.) ;
#54321=ORIENTED_EDGE('',*,*,#41838,.T.) ;
#54322=ORIENTED_EDGE('',*,*,#41839,.T.) ;
#54323=ORIENTED_EDGE('',*,*,#41840,.T.) ;
#54324=ORIENTED_EDGE('',*,*,#41841,.T.) ;
#54325=ORIENTED_EDGE('',*,*,#41842,.F.) ;
#54326=ORIENTED_EDGE('',*,*,#41843,.F.) ;
#54327=ORIENTED_EDGE('',*,*,#41844,.T.) ;
#54328=ORIENTED_EDGE('',*,*,#41845,.F.) ;
#54329=ORIENTED_EDGE('',*,*,#41846,.T.) ;
#54330=ORIENTED_EDGE('',*,*,#41847,.F.) ;
#54331=ORIENTED_EDGE('',*,*,#41848,.T.) ;
#54332=ORIENTED_EDGE('',*,*,#41849,.F.) ;
#54333=ORIENTED_EDGE('',*,*,#41850,.T.) ;
#54334=ORIENTED_EDGE('',*,*,#41851,.F.) ;
#54335=ORIENTED_EDGE('',*,*,#41852,.T.) ;
#54336=ORIENTED_EDGE('',*,*,#41853,.F.) ;
#54337=ORIENTED_EDGE('',*,*,#41854,.T.) ;
#54338=ORIENTED_EDGE('',*,*,#41855,.F.) ;
#54339=ORIENTED_EDGE('',*,*,#41856,.T.) ;
#54340=ORIENTED_EDGE('',*,*,#41857,.F.) ;
#54341=ORIENTED_EDGE('',*,*,#41858,.T.) ;
#54342=ORIENTED_EDGE('',*,*,#41859,.T.) ;
#54343=ORIENTED_EDGE('',*,*,#41860,.T.) ;
#54344=ORIENTED_EDGE('',*,*,#41861,.T.) ;
#54345=ORIENTED_EDGE('',*,*,#41862,.F.) ;
#54346=ORIENTED_EDGE('',*,*,#41863,.T.) ;
#54347=ORIENTED_EDGE('',*,*,#41864,.T.) ;
#54348=ORIENTED_EDGE('',*,*,#41865,.T.) ;
#54349=ORIENTED_EDGE('',*,*,#41866,.T.) ;
#54350=ORIENTED_EDGE('',*,*,#41867,.T.) ;
#54351=ORIENTED_EDGE('',*,*,#41868,.F.) ;
#54352=ORIENTED_EDGE('',*,*,#41869,.T.) ;
#54353=ORIENTED_EDGE('',*,*,#41870,.T.) ;
#54354=ORIENTED_EDGE('',*,*,#41871,.T.) ;
#54355=ORIENTED_EDGE('',*,*,#41872,.T.) ;
#54356=ORIENTED_EDGE('',*,*,#41873,.T.) ;
#54357=ORIENTED_EDGE('',*,*,#41874,.T.) ;
#54358=ORIENTED_EDGE('',*,*,#41875,.T.) ;
#54359=ORIENTED_EDGE('',*,*,#41876,.T.) ;
#54360=ORIENTED_EDGE('',*,*,#41877,.F.) ;
#54361=ORIENTED_EDGE('',*,*,#41878,.T.) ;
#54362=ORIENTED_EDGE('',*,*,#41879,.T.) ;
#54363=ORIENTED_EDGE('',*,*,#41880,.T.) ;
#54364=ORIENTED_EDGE('',*,*,#41881,.T.) ;
#54365=ORIENTED_EDGE('',*,*,#41882,.T.) ;
#54366=ORIENTED_EDGE('',*,*,#41883,.T.) ;
#54367=ORIENTED_EDGE('',*,*,#41884,.T.) ;
#54368=ORIENTED_EDGE('',*,*,#41728,.T.) ;
#54369=ORIENTED_EDGE('',*,*,#41787,.T.) ;
#54370=ORIENTED_EDGE('',*,*,#41885,.T.) ;
#54371=ORIENTED_EDGE('',*,*,#41792,.T.) ;
#54372=ORIENTED_EDGE('',*,*,#41886,.T.) ;
#54373=ORIENTED_EDGE('',*,*,#41812,.T.) ;
#54374=ORIENTED_EDGE('',*,*,#41887,.T.) ;
#54375=ORIENTED_EDGE('',*,*,#41815,.T.) ;
#54376=ORIENTED_EDGE('',*,*,#41648,.T.) ;
#54377=ORIENTED_EDGE('',*,*,#41818,.T.) ;
#54378=ORIENTED_EDGE('',*,*,#41888,.T.) ;
#54379=ORIENTED_EDGE('',*,*,#41822,.T.) ;
#54380=ORIENTED_EDGE('',*,*,#41889,.T.) ;
#54381=ORIENTED_EDGE('',*,*,#41842,.T.) ;
#54382=ORIENTED_EDGE('',*,*,#41890,.T.) ;
#54383=ORIENTED_EDGE('',*,*,#41862,.T.) ;
#54384=ORIENTED_EDGE('',*,*,#41891,.T.) ;
#54385=ORIENTED_EDGE('',*,*,#41868,.T.) ;
#54386=ORIENTED_EDGE('',*,*,#41892,.T.) ;
#54387=ORIENTED_EDGE('',*,*,#41877,.T.) ;
#54388=ORIENTED_EDGE('',*,*,#41893,.T.) ;
#54389=ORIENTED_EDGE('',*,*,#41735,.T.) ;
#54390=ORIENTED_EDGE('',*,*,#41894,.T.) ;
#54391=ORIENTED_EDGE('',*,*,#41746,.T.) ;
#54392=ORIENTED_EDGE('',*,*,#41895,.T.) ;
#54393=ORIENTED_EDGE('',*,*,#41768,.T.) ;
#54394=ORIENTED_EDGE('',*,*,#41896,.T.) ;
#54395=ORIENTED_EDGE('',*,*,#41770,.T.) ;
#54396=ORIENTED_EDGE('',*,*,#41897,.T.) ;
#54397=ORIENTED_EDGE('',*,*,#41697,.T.) ;
#54398=ORIENTED_EDGE('',*,*,#41898,.T.) ;
#54399=ORIENTED_EDGE('',*,*,#41784,.T.) ;
#54400=ORIENTED_EDGE('',*,*,#41899,.T.) ;
#54401=ORIENTED_EDGE('',*,*,#41900,.T.) ;
#54402=ORIENTED_EDGE('',*,*,#41901,.T.) ;
#54403=ORIENTED_EDGE('',*,*,#41902,.T.) ;
#54404=ORIENTED_EDGE('',*,*,#41903,.T.) ;
#54405=ORIENTED_EDGE('',*,*,#41904,.T.) ;
#54406=ORIENTED_EDGE('',*,*,#41905,.T.) ;
#54407=ORIENTED_EDGE('',*,*,#41906,.T.) ;
#54408=ORIENTED_EDGE('',*,*,#41907,.F.) ;
#54409=ORIENTED_EDGE('',*,*,#41908,.T.) ;
#54410=ORIENTED_EDGE('',*,*,#41909,.T.) ;
#54411=ORIENTED_EDGE('',*,*,#41910,.T.) ;
#54412=ORIENTED_EDGE('',*,*,#41911,.F.) ;
#54413=ORIENTED_EDGE('',*,*,#41912,.T.) ;
#54414=ORIENTED_EDGE('',*,*,#41913,.T.) ;
#54415=ORIENTED_EDGE('',*,*,#41914,.T.) ;
#54416=ORIENTED_EDGE('',*,*,#41915,.T.) ;
#54417=ORIENTED_EDGE('',*,*,#41916,.T.) ;
#54418=ORIENTED_EDGE('',*,*,#41917,.F.) ;
#54419=ORIENTED_EDGE('',*,*,#41918,.T.) ;
#54420=ORIENTED_EDGE('',*,*,#41909,.F.) ;
#54421=ORIENTED_EDGE('',*,*,#41919,.T.) ;
#54422=ORIENTED_EDGE('',*,*,#41920,.T.) ;
#54423=ORIENTED_EDGE('',*,*,#41921,.T.) ;
#54424=ORIENTED_EDGE('',*,*,#41922,.F.) ;
#54425=ORIENTED_EDGE('',*,*,#41923,.T.) ;
#54426=ORIENTED_EDGE('',*,*,#41915,.F.) ;
#54427=ORIENTED_EDGE('',*,*,#41924,.T.) ;
#54428=ORIENTED_EDGE('',*,*,#41925,.F.) ;
#54429=ORIENTED_EDGE('',*,*,#41926,.T.) ;
#54430=ORIENTED_EDGE('',*,*,#41927,.T.) ;
#54431=ORIENTED_EDGE('',*,*,#41928,.T.) ;
#54432=ORIENTED_EDGE('',*,*,#41920,.F.) ;
#54433=ORIENTED_EDGE('',*,*,#41929,.T.) ;
#54434=ORIENTED_EDGE('',*,*,#41930,.T.) ;
#54435=ORIENTED_EDGE('',*,*,#41931,.T.) ;
#54436=ORIENTED_EDGE('',*,*,#41917,.T.) ;
#54437=ORIENTED_EDGE('',*,*,#41932,.T.) ;
#54438=ORIENTED_EDGE('',*,*,#41933,.T.) ;
#54439=ORIENTED_EDGE('',*,*,#41934,.T.) ;
#54440=ORIENTED_EDGE('',*,*,#41935,.T.) ;
#54441=ORIENTED_EDGE('',*,*,#41936,.T.) ;
#54442=ORIENTED_EDGE('',*,*,#41937,.T.) ;
#54443=ORIENTED_EDGE('',*,*,#41938,.T.) ;
#54444=ORIENTED_EDGE('',*,*,#41939,.T.) ;
#54445=ORIENTED_EDGE('',*,*,#41940,.T.) ;
#54446=ORIENTED_EDGE('',*,*,#41941,.T.) ;
#54447=ORIENTED_EDGE('',*,*,#41942,.T.) ;
#54448=ORIENTED_EDGE('',*,*,#41943,.T.) ;
#54449=ORIENTED_EDGE('',*,*,#41944,.T.) ;
#54450=ORIENTED_EDGE('',*,*,#41945,.T.) ;
#54451=ORIENTED_EDGE('',*,*,#41946,.T.) ;
#54452=ORIENTED_EDGE('',*,*,#41947,.T.) ;
#54453=ORIENTED_EDGE('',*,*,#41948,.T.) ;
#54454=ORIENTED_EDGE('',*,*,#41949,.T.) ;
#54455=ORIENTED_EDGE('',*,*,#41950,.T.) ;
#54456=ORIENTED_EDGE('',*,*,#41951,.T.) ;
#54457=ORIENTED_EDGE('',*,*,#41952,.T.) ;
#54458=ORIENTED_EDGE('',*,*,#41953,.T.) ;
#54459=ORIENTED_EDGE('',*,*,#41954,.T.) ;
#54460=ORIENTED_EDGE('',*,*,#41955,.T.) ;
#54461=ORIENTED_EDGE('',*,*,#41956,.T.) ;
#54462=ORIENTED_EDGE('',*,*,#41957,.T.) ;
#54463=ORIENTED_EDGE('',*,*,#41958,.T.) ;
#54464=ORIENTED_EDGE('',*,*,#41959,.T.) ;
#54465=ORIENTED_EDGE('',*,*,#41960,.T.) ;
#54466=ORIENTED_EDGE('',*,*,#41961,.T.) ;
#54467=ORIENTED_EDGE('',*,*,#41962,.T.) ;
#54468=ORIENTED_EDGE('',*,*,#41963,.T.) ;
#54469=ORIENTED_EDGE('',*,*,#41964,.T.) ;
#54470=ORIENTED_EDGE('',*,*,#41965,.T.) ;
#54471=ORIENTED_EDGE('',*,*,#41966,.T.) ;
#54472=ORIENTED_EDGE('',*,*,#41967,.F.) ;
#54473=ORIENTED_EDGE('',*,*,#41968,.F.) ;
#54474=ORIENTED_EDGE('',*,*,#41969,.F.) ;
#54475=ORIENTED_EDGE('',*,*,#41970,.F.) ;
#54476=ORIENTED_EDGE('',*,*,#41971,.F.) ;
#54477=ORIENTED_EDGE('',*,*,#41972,.F.) ;
#54478=ORIENTED_EDGE('',*,*,#41973,.F.) ;
#54479=ORIENTED_EDGE('',*,*,#41974,.F.) ;
#54480=ORIENTED_EDGE('',*,*,#41975,.F.) ;
#54481=ORIENTED_EDGE('',*,*,#41976,.F.) ;
#54482=ORIENTED_EDGE('',*,*,#41974,.T.) ;
#54483=ORIENTED_EDGE('',*,*,#41977,.T.) ;
#54484=ORIENTED_EDGE('',*,*,#41978,.F.) ;
#54485=ORIENTED_EDGE('',*,*,#41979,.F.) ;
#54486=ORIENTED_EDGE('',*,*,#41967,.T.) ;
#54487=ORIENTED_EDGE('',*,*,#41976,.T.) ;
#54488=ORIENTED_EDGE('',*,*,#41980,.F.) ;
#54489=ORIENTED_EDGE('',*,*,#41981,.F.) ;
#54490=ORIENTED_EDGE('',*,*,#41968,.T.) ;
#54491=ORIENTED_EDGE('',*,*,#41979,.T.) ;
#54492=ORIENTED_EDGE('',*,*,#41982,.F.) ;
#54493=ORIENTED_EDGE('',*,*,#41983,.F.) ;
#54494=ORIENTED_EDGE('',*,*,#41969,.T.) ;
#54495=ORIENTED_EDGE('',*,*,#41981,.T.) ;
#54496=ORIENTED_EDGE('',*,*,#41984,.F.) ;
#54497=ORIENTED_EDGE('',*,*,#41985,.F.) ;
#54498=ORIENTED_EDGE('',*,*,#41970,.T.) ;
#54499=ORIENTED_EDGE('',*,*,#41983,.T.) ;
#54500=ORIENTED_EDGE('',*,*,#41986,.F.) ;
#54501=ORIENTED_EDGE('',*,*,#41987,.F.) ;
#54502=ORIENTED_EDGE('',*,*,#41971,.T.) ;
#54503=ORIENTED_EDGE('',*,*,#41985,.T.) ;
#54504=ORIENTED_EDGE('',*,*,#41988,.F.) ;
#54505=ORIENTED_EDGE('',*,*,#41989,.F.) ;
#54506=ORIENTED_EDGE('',*,*,#41972,.T.) ;
#54507=ORIENTED_EDGE('',*,*,#41987,.T.) ;
#54508=ORIENTED_EDGE('',*,*,#41990,.F.) ;
#54509=ORIENTED_EDGE('',*,*,#41977,.F.) ;
#54510=ORIENTED_EDGE('',*,*,#41973,.T.) ;
#54511=ORIENTED_EDGE('',*,*,#41989,.T.) ;
#54512=ORIENTED_EDGE('',*,*,#41978,.T.) ;
#54513=ORIENTED_EDGE('',*,*,#41975,.T.) ;
#54514=ORIENTED_EDGE('',*,*,#41990,.T.) ;
#54515=ORIENTED_EDGE('',*,*,#41988,.T.) ;
#54516=ORIENTED_EDGE('',*,*,#41986,.T.) ;
#54517=ORIENTED_EDGE('',*,*,#41984,.T.) ;
#54518=ORIENTED_EDGE('',*,*,#41982,.T.) ;
#54519=ORIENTED_EDGE('',*,*,#41980,.T.) ;
#54520=ORIENTED_EDGE('',*,*,#41685,.T.) ;
#54521=ORIENTED_EDGE('',*,*,#41991,.T.) ;
#54522=ORIENTED_EDGE('',*,*,#41683,.F.) ;
#54523=ORIENTED_EDGE('',*,*,#41992,.T.) ;
#54524=ORIENTED_EDGE('',*,*,#41687,.T.) ;
#54525=ORIENTED_EDGE('',*,*,#41993,.T.) ;
#54526=ORIENTED_EDGE('',*,*,#41691,.F.) ;
#54527=ORIENTED_EDGE('',*,*,#41994,.T.) ;
#54528=ORIENTED_EDGE('',*,*,#41679,.T.) ;
#54529=ORIENTED_EDGE('',*,*,#41995,.T.) ;
#54530=ORIENTED_EDGE('',*,*,#41681,.T.) ;
#54531=ORIENTED_EDGE('',*,*,#41996,.T.) ;
#54532=ORIENTED_EDGE('',*,*,#41689,.T.) ;
#54533=ORIENTED_EDGE('',*,*,#41997,.T.) ;
#54534=ORIENTED_EDGE('',*,*,#41998,.T.) ;
#54535=ORIENTED_EDGE('',*,*,#41999,.T.) ;
#54536=ORIENTED_EDGE('',*,*,#42000,.T.) ;
#54537=ORIENTED_EDGE('',*,*,#42001,.T.) ;
#54538=ORIENTED_EDGE('',*,*,#42002,.T.) ;
#54539=ORIENTED_EDGE('',*,*,#42003,.T.) ;
#54540=ORIENTED_EDGE('',*,*,#42004,.T.) ;
#54541=ORIENTED_EDGE('',*,*,#42005,.T.) ;
#54542=ORIENTED_EDGE('',*,*,#42006,.T.) ;
#54543=ORIENTED_EDGE('',*,*,#42007,.T.) ;
#54544=ORIENTED_EDGE('',*,*,#42008,.T.) ;
#54545=ORIENTED_EDGE('',*,*,#42009,.T.) ;
#54546=ORIENTED_EDGE('',*,*,#42010,.T.) ;
#54547=ORIENTED_EDGE('',*,*,#42011,.T.) ;
#54548=ORIENTED_EDGE('',*,*,#42012,.T.) ;
#54549=ORIENTED_EDGE('',*,*,#42013,.T.) ;
#54550=ORIENTED_EDGE('',*,*,#42014,.T.) ;
#54551=ORIENTED_EDGE('',*,*,#42015,.T.) ;
#54552=ORIENTED_EDGE('',*,*,#42016,.T.) ;
#54553=ORIENTED_EDGE('',*,*,#42017,.T.) ;
#54554=ORIENTED_EDGE('',*,*,#42018,.F.) ;
#54555=ORIENTED_EDGE('',*,*,#42019,.F.) ;
#54556=ORIENTED_EDGE('',*,*,#42020,.F.) ;
#54557=ORIENTED_EDGE('',*,*,#42021,.F.) ;
#54558=ORIENTED_EDGE('',*,*,#42022,.F.) ;
#54559=ORIENTED_EDGE('',*,*,#42023,.F.) ;
#54560=ORIENTED_EDGE('',*,*,#42024,.F.) ;
#54561=ORIENTED_EDGE('',*,*,#42025,.F.) ;
#54562=ORIENTED_EDGE('',*,*,#42026,.T.) ;
#54563=ORIENTED_EDGE('',*,*,#42027,.T.) ;
#54564=ORIENTED_EDGE('',*,*,#42028,.F.) ;
#54565=ORIENTED_EDGE('',*,*,#42025,.T.) ;
#54566=ORIENTED_EDGE('',*,*,#42028,.T.) ;
#54567=ORIENTED_EDGE('',*,*,#42029,.T.) ;
#54568=ORIENTED_EDGE('',*,*,#42030,.F.) ;
#54569=ORIENTED_EDGE('',*,*,#42018,.T.) ;
#54570=ORIENTED_EDGE('',*,*,#42030,.T.) ;
#54571=ORIENTED_EDGE('',*,*,#42031,.T.) ;
#54572=ORIENTED_EDGE('',*,*,#42032,.F.) ;
#54573=ORIENTED_EDGE('',*,*,#42019,.T.) ;
#54574=ORIENTED_EDGE('',*,*,#42032,.T.) ;
#54575=ORIENTED_EDGE('',*,*,#42033,.T.) ;
#54576=ORIENTED_EDGE('',*,*,#42034,.F.) ;
#54577=ORIENTED_EDGE('',*,*,#42020,.T.) ;
#54578=ORIENTED_EDGE('',*,*,#42034,.T.) ;
#54579=ORIENTED_EDGE('',*,*,#42035,.T.) ;
#54580=ORIENTED_EDGE('',*,*,#42036,.F.) ;
#54581=ORIENTED_EDGE('',*,*,#42021,.T.) ;
#54582=ORIENTED_EDGE('',*,*,#42036,.T.) ;
#54583=ORIENTED_EDGE('',*,*,#42037,.T.) ;
#54584=ORIENTED_EDGE('',*,*,#42038,.F.) ;
#54585=ORIENTED_EDGE('',*,*,#42022,.T.) ;
#54586=ORIENTED_EDGE('',*,*,#42038,.T.) ;
#54587=ORIENTED_EDGE('',*,*,#42039,.T.) ;
#54588=ORIENTED_EDGE('',*,*,#42040,.F.) ;
#54589=ORIENTED_EDGE('',*,*,#42023,.T.) ;
#54590=ORIENTED_EDGE('',*,*,#42040,.T.) ;
#54591=ORIENTED_EDGE('',*,*,#42041,.T.) ;
#54592=ORIENTED_EDGE('',*,*,#42026,.F.) ;
#54593=ORIENTED_EDGE('',*,*,#42024,.T.) ;
#54594=ORIENTED_EDGE('',*,*,#42042,.T.) ;
#54595=ORIENTED_EDGE('',*,*,#42043,.T.) ;
#54596=ORIENTED_EDGE('',*,*,#42044,.T.) ;
#54597=ORIENTED_EDGE('',*,*,#42045,.T.) ;
#54598=ORIENTED_EDGE('',*,*,#42046,.T.) ;
#54599=ORIENTED_EDGE('',*,*,#42047,.T.) ;
#54600=ORIENTED_EDGE('',*,*,#42048,.T.) ;
#54601=ORIENTED_EDGE('',*,*,#42049,.T.) ;
#54602=ORIENTED_EDGE('',*,*,#42050,.T.) ;
#54603=ORIENTED_EDGE('',*,*,#41668,.T.) ;
#54604=ORIENTED_EDGE('',*,*,#42051,.T.) ;
#54605=ORIENTED_EDGE('',*,*,#42052,.T.) ;
#54606=ORIENTED_EDGE('',*,*,#41670,.T.) ;
#54607=ORIENTED_EDGE('',*,*,#42053,.T.) ;
#54608=ORIENTED_EDGE('',*,*,#42054,.T.) ;
#54609=ORIENTED_EDGE('',*,*,#42055,.T.) ;
#54610=ORIENTED_EDGE('',*,*,#42056,.T.) ;
#54611=ORIENTED_EDGE('',*,*,#42057,.T.) ;
#54612=ORIENTED_EDGE('',*,*,#42058,.T.) ;
#54613=ORIENTED_EDGE('',*,*,#42059,.T.) ;
#54614=ORIENTED_EDGE('',*,*,#42060,.T.) ;
#54615=ORIENTED_EDGE('',*,*,#41642,.T.) ;
#54616=ORIENTED_EDGE('',*,*,#41674,.T.) ;
#54617=ORIENTED_EDGE('',*,*,#42061,.T.) ;
#54618=ORIENTED_EDGE('',*,*,#42062,.T.) ;
#54619=ORIENTED_EDGE('',*,*,#42063,.T.) ;
#54620=ORIENTED_EDGE('',*,*,#42064,.T.) ;
#54621=ORIENTED_EDGE('',*,*,#42065,.T.) ;
#54622=ORIENTED_EDGE('',*,*,#42066,.T.) ;
#54623=ORIENTED_EDGE('',*,*,#42067,.F.) ;
#54624=ORIENTED_EDGE('',*,*,#42068,.F.) ;
#54625=ORIENTED_EDGE('',*,*,#42069,.F.) ;
#54626=ORIENTED_EDGE('',*,*,#41832,.F.) ;
#54627=ORIENTED_EDGE('',*,*,#41919,.F.) ;
#54628=ORIENTED_EDGE('',*,*,#41908,.F.) ;
#54629=ORIENTED_EDGE('',*,*,#42070,.F.) ;
#54630=ORIENTED_EDGE('',*,*,#41929,.F.) ;
#54631=ORIENTED_EDGE('',*,*,#42070,.T.) ;
#54632=ORIENTED_EDGE('',*,*,#41907,.T.) ;
#54633=ORIENTED_EDGE('',*,*,#42071,.F.) ;
#54634=ORIENTED_EDGE('',*,*,#42072,.F.) ;
#54635=ORIENTED_EDGE('',*,*,#42071,.T.) ;
#54636=ORIENTED_EDGE('',*,*,#41914,.F.) ;
#54637=ORIENTED_EDGE('',*,*,#42073,.F.) ;
#54638=ORIENTED_EDGE('',*,*,#41945,.F.) ;
#54639=ORIENTED_EDGE('',*,*,#42068,.T.) ;
#54640=ORIENTED_EDGE('',*,*,#41946,.F.) ;
#54641=ORIENTED_EDGE('',*,*,#42074,.F.) ;
#54642=ORIENTED_EDGE('',*,*,#41905,.F.) ;
#54643=ORIENTED_EDGE('',*,*,#42069,.T.) ;
#54644=ORIENTED_EDGE('',*,*,#41904,.F.) ;
#54645=ORIENTED_EDGE('',*,*,#42075,.F.) ;
#54646=ORIENTED_EDGE('',*,*,#41833,.F.) ;
#54647=ORIENTED_EDGE('',*,*,#42067,.T.) ;
#54648=ORIENTED_EDGE('',*,*,#41831,.F.) ;
#54649=ORIENTED_EDGE('',*,*,#42076,.F.) ;
#54650=ORIENTED_EDGE('',*,*,#41941,.F.) ;
#54651=ORIENTED_EDGE('',*,*,#42072,.T.) ;
#54652=ORIENTED_EDGE('',*,*,#41944,.F.) ;
#54653=ORIENTED_EDGE('',*,*,#42077,.F.) ;
#54654=ORIENTED_EDGE('',*,*,#41930,.F.) ;
#54655=ORIENTED_EDGE('',*,*,#41921,.F.) ;
#54656=ORIENTED_EDGE('',*,*,#41931,.F.) ;
#54657=ORIENTED_EDGE('',*,*,#42078,.F.) ;
#54658=ORIENTED_EDGE('',*,*,#41924,.F.) ;
#54659=ORIENTED_EDGE('',*,*,#42074,.T.) ;
#54660=ORIENTED_EDGE('',*,*,#42073,.T.) ;
#54661=ORIENTED_EDGE('',*,*,#42079,.F.) ;
#54662=ORIENTED_EDGE('',*,*,#41834,.T.) ;
#54663=ORIENTED_EDGE('',*,*,#42075,.T.) ;
#54664=ORIENTED_EDGE('',*,*,#42080,.F.) ;
#54665=ORIENTED_EDGE('',*,*,#42081,.F.) ;
#54666=ORIENTED_EDGE('',*,*,#42076,.T.) ;
#54667=ORIENTED_EDGE('',*,*,#41838,.F.) ;
#54668=ORIENTED_EDGE('',*,*,#42082,.F.) ;
#54669=ORIENTED_EDGE('',*,*,#42083,.F.) ;
#54670=ORIENTED_EDGE('',*,*,#42078,.T.) ;
#54671=ORIENTED_EDGE('',*,*,#42077,.T.) ;
#54672=ORIENTED_EDGE('',*,*,#42084,.F.) ;
#54673=ORIENTED_EDGE('',*,*,#41925,.T.) ;
#54674=ORIENTED_EDGE('',*,*,#42079,.T.) ;
#54675=ORIENTED_EDGE('',*,*,#41913,.F.) ;
#54676=ORIENTED_EDGE('',*,*,#42085,.F.) ;
#54677=ORIENTED_EDGE('',*,*,#41906,.F.) ;
#54678=ORIENTED_EDGE('',*,*,#42080,.T.) ;
#54679=ORIENTED_EDGE('',*,*,#41903,.F.) ;
#54680=ORIENTED_EDGE('',*,*,#42086,.F.) ;
#54681=ORIENTED_EDGE('',*,*,#41939,.F.) ;
#54682=ORIENTED_EDGE('',*,*,#42081,.T.) ;
#54683=ORIENTED_EDGE('',*,*,#41938,.F.) ;
#54684=ORIENTED_EDGE('',*,*,#42087,.F.) ;
#54685=ORIENTED_EDGE('',*,*,#41835,.F.) ;
#54686=ORIENTED_EDGE('',*,*,#42082,.T.) ;
#54687=ORIENTED_EDGE('',*,*,#41837,.F.) ;
#54688=ORIENTED_EDGE('',*,*,#42088,.F.) ;
#54689=ORIENTED_EDGE('',*,*,#41900,.F.) ;
#54690=ORIENTED_EDGE('',*,*,#42083,.T.) ;
#54691=ORIENTED_EDGE('',*,*,#41899,.F.) ;
#54692=ORIENTED_EDGE('',*,*,#42089,.F.) ;
#54693=ORIENTED_EDGE('',*,*,#41942,.F.) ;
#54694=ORIENTED_EDGE('',*,*,#42084,.T.) ;
#54695=ORIENTED_EDGE('',*,*,#41943,.F.) ;
#54696=ORIENTED_EDGE('',*,*,#42090,.F.) ;
#54697=ORIENTED_EDGE('',*,*,#41926,.F.) ;
#54698=ORIENTED_EDGE('',*,*,#42086,.T.) ;
#54699=ORIENTED_EDGE('',*,*,#42085,.T.) ;
#54700=ORIENTED_EDGE('',*,*,#42091,.F.) ;
#54701=ORIENTED_EDGE('',*,*,#41836,.T.) ;
#54702=ORIENTED_EDGE('',*,*,#42087,.T.) ;
#54703=ORIENTED_EDGE('',*,*,#42092,.F.) ;
#54704=ORIENTED_EDGE('',*,*,#42088,.T.) ;
#54705=ORIENTED_EDGE('',*,*,#42090,.T.) ;
#54706=ORIENTED_EDGE('',*,*,#42089,.T.) ;
#54707=ORIENTED_EDGE('',*,*,#42093,.F.) ;
#54708=ORIENTED_EDGE('',*,*,#41918,.F.) ;
#54709=ORIENTED_EDGE('',*,*,#41934,.F.) ;
#54710=ORIENTED_EDGE('',*,*,#42094,.F.) ;
#54711=ORIENTED_EDGE('',*,*,#41910,.F.) ;
#54712=ORIENTED_EDGE('',*,*,#42091,.T.) ;
#54713=ORIENTED_EDGE('',*,*,#41912,.F.) ;
#54714=ORIENTED_EDGE('',*,*,#42095,.F.) ;
#54715=ORIENTED_EDGE('',*,*,#41940,.F.) ;
#54716=ORIENTED_EDGE('',*,*,#42092,.T.) ;
#54717=ORIENTED_EDGE('',*,*,#41937,.F.) ;
#54718=ORIENTED_EDGE('',*,*,#42096,.F.) ;
#54719=ORIENTED_EDGE('',*,*,#41901,.F.) ;
#54720=ORIENTED_EDGE('',*,*,#42093,.T.) ;
#54721=ORIENTED_EDGE('',*,*,#41902,.F.) ;
#54722=ORIENTED_EDGE('',*,*,#42097,.F.) ;
#54723=ORIENTED_EDGE('',*,*,#41927,.F.) ;
#54724=ORIENTED_EDGE('',*,*,#41911,.T.) ;
#54725=ORIENTED_EDGE('',*,*,#42094,.T.) ;
#54726=ORIENTED_EDGE('',*,*,#42098,.F.) ;
#54727=ORIENTED_EDGE('',*,*,#42095,.T.) ;
#54728=ORIENTED_EDGE('',*,*,#42097,.T.) ;
#54729=ORIENTED_EDGE('',*,*,#42096,.T.) ;
#54730=ORIENTED_EDGE('',*,*,#42099,.F.) ;
#54731=ORIENTED_EDGE('',*,*,#42098,.T.) ;
#54732=ORIENTED_EDGE('',*,*,#41933,.F.) ;
#54733=ORIENTED_EDGE('',*,*,#42100,.F.) ;
#54734=ORIENTED_EDGE('',*,*,#41935,.F.) ;
#54735=ORIENTED_EDGE('',*,*,#42099,.T.) ;
#54736=ORIENTED_EDGE('',*,*,#41936,.F.) ;
#54737=ORIENTED_EDGE('',*,*,#42101,.F.) ;
#54738=ORIENTED_EDGE('',*,*,#41928,.F.) ;
#54739=ORIENTED_EDGE('',*,*,#42101,.T.) ;
#54740=ORIENTED_EDGE('',*,*,#42100,.T.) ;
#54741=ORIENTED_EDGE('',*,*,#42102,.F.) ;
#54742=ORIENTED_EDGE('',*,*,#41922,.T.) ;
#54743=ORIENTED_EDGE('',*,*,#41916,.F.) ;
#54744=ORIENTED_EDGE('',*,*,#41923,.F.) ;
#54745=ORIENTED_EDGE('',*,*,#42102,.T.) ;
#54746=ORIENTED_EDGE('',*,*,#41932,.F.) ;
#54747=ORIENTED_EDGE('',*,*,#41672,.F.) ;
#54748=ORIENTED_EDGE('',*,*,#41762,.F.) ;
#54749=ORIENTED_EDGE('',*,*,#41613,.F.) ;
#54750=ORIENTED_EDGE('',*,*,#41739,.F.) ;
#54751=ORIENTED_EDGE('',*,*,#41742,.F.) ;
#54752=ORIENTED_EDGE('',*,*,#42103,.T.) ;
#54753=ORIENTED_EDGE('',*,*,#42104,.T.) ;
#54754=ORIENTED_EDGE('',*,*,#41644,.T.) ;
#54755=ORIENTED_EDGE('',*,*,#42046,.F.) ;
#54756=ORIENTED_EDGE('',*,*,#41673,.T.) ;
#54757=ORIENTED_EDGE('',*,*,#42048,.F.) ;
#54758=ORIENTED_EDGE('',*,*,#42105,.T.) ;
#54759=ORIENTED_EDGE('',*,*,#42052,.F.) ;
#54760=ORIENTED_EDGE('',*,*,#42106,.F.) ;
#54761=ORIENTED_EDGE('',*,*,#41671,.T.) ;
#54762=ORIENTED_EDGE('',*,*,#42049,.F.) ;
#54763=ORIENTED_EDGE('',*,*,#42107,.F.) ;
#54764=ORIENTED_EDGE('',*,*,#41763,.F.) ;
#54765=ORIENTED_EDGE('',*,*,#41773,.F.) ;
#54766=ORIENTED_EDGE('',*,*,#42108,.T.) ;
#54767=ORIENTED_EDGE('',*,*,#42056,.F.) ;
#54768=ORIENTED_EDGE('',*,*,#42109,.T.) ;
#54769=ORIENTED_EDGE('',*,*,#42059,.F.) ;
#54770=ORIENTED_EDGE('',*,*,#42110,.T.) ;
#54771=ORIENTED_EDGE('',*,*,#42050,.F.) ;
#54772=ORIENTED_EDGE('',*,*,#42111,.T.) ;
#54773=ORIENTED_EDGE('',*,*,#42107,.T.) ;
#54774=ORIENTED_EDGE('',*,*,#42106,.T.) ;
#54775=ORIENTED_EDGE('',*,*,#42112,.F.) ;
#54776=ORIENTED_EDGE('',*,*,#41764,.T.) ;
#54777=ORIENTED_EDGE('',*,*,#41895,.F.) ;
#54778=ORIENTED_EDGE('',*,*,#41745,.F.) ;
#54779=ORIENTED_EDGE('',*,*,#41666,.F.) ;
#54780=ORIENTED_EDGE('',*,*,#41769,.F.) ;
#54781=ORIENTED_EDGE('',*,*,#42113,.T.) ;
#54782=ORIENTED_EDGE('',*,*,#42114,.T.) ;
#54783=ORIENTED_EDGE('',*,*,#41766,.F.) ;
#54784=ORIENTED_EDGE('',*,*,#41665,.F.) ;
#54785=ORIENTED_EDGE('',*,*,#42054,.F.) ;
#54786=ORIENTED_EDGE('',*,*,#42115,.T.) ;
#54787=ORIENTED_EDGE('',*,*,#42112,.T.) ;
#54788=ORIENTED_EDGE('',*,*,#42051,.F.) ;
#54789=ORIENTED_EDGE('',*,*,#41664,.F.) ;
#54790=ORIENTED_EDGE('',*,*,#41765,.F.) ;
#54791=ORIENTED_EDGE('',*,*,#41667,.T.) ;
#54792=ORIENTED_EDGE('',*,*,#41744,.F.) ;
#54793=ORIENTED_EDGE('',*,*,#41662,.T.) ;
#54794=ORIENTED_EDGE('',*,*,#42055,.F.) ;
#54795=ORIENTED_EDGE('',*,*,#42116,.F.) ;
#54796=ORIENTED_EDGE('',*,*,#42031,.F.) ;
#54797=ORIENTED_EDGE('',*,*,#42117,.F.) ;
#54798=ORIENTED_EDGE('',*,*,#42117,.T.) ;
#54799=ORIENTED_EDGE('',*,*,#42029,.F.) ;
#54800=ORIENTED_EDGE('',*,*,#42118,.F.) ;
#54801=ORIENTED_EDGE('',*,*,#42042,.F.) ;
#54802=ORIENTED_EDGE('',*,*,#42116,.T.) ;
#54803=ORIENTED_EDGE('',*,*,#42045,.F.) ;
#54804=ORIENTED_EDGE('',*,*,#42119,.F.) ;
#54805=ORIENTED_EDGE('',*,*,#42033,.F.) ;
#54806=ORIENTED_EDGE('',*,*,#42118,.T.) ;
#54807=ORIENTED_EDGE('',*,*,#42027,.F.) ;
#54808=ORIENTED_EDGE('',*,*,#42120,.F.) ;
#54809=ORIENTED_EDGE('',*,*,#42035,.F.) ;
#54810=ORIENTED_EDGE('',*,*,#42119,.T.) ;
#54811=ORIENTED_EDGE('',*,*,#42121,.F.) ;
#54812=ORIENTED_EDGE('',*,*,#42120,.T.) ;
#54813=ORIENTED_EDGE('',*,*,#42041,.F.) ;
#54814=ORIENTED_EDGE('',*,*,#42122,.F.) ;
#54815=ORIENTED_EDGE('',*,*,#42043,.F.) ;
#54816=ORIENTED_EDGE('',*,*,#42121,.T.) ;
#54817=ORIENTED_EDGE('',*,*,#42044,.F.) ;
#54818=ORIENTED_EDGE('',*,*,#42123,.F.) ;
#54819=ORIENTED_EDGE('',*,*,#42037,.F.) ;
#54820=ORIENTED_EDGE('',*,*,#42122,.T.) ;
#54821=ORIENTED_EDGE('',*,*,#42039,.F.) ;
#54822=ORIENTED_EDGE('',*,*,#42123,.T.) ;
#54823=ORIENTED_EDGE('',*,*,#42124,.F.) ;
#54824=ORIENTED_EDGE('',*,*,#41856,.F.) ;
#54825=ORIENTED_EDGE('',*,*,#42125,.F.) ;
#54826=ORIENTED_EDGE('',*,*,#41950,.F.) ;
#54827=ORIENTED_EDGE('',*,*,#42125,.T.) ;
#54828=ORIENTED_EDGE('',*,*,#41855,.T.) ;
#54829=ORIENTED_EDGE('',*,*,#42126,.F.) ;
#54830=ORIENTED_EDGE('',*,*,#42127,.F.) ;
#54831=ORIENTED_EDGE('',*,*,#41857,.T.) ;
#54832=ORIENTED_EDGE('',*,*,#42124,.T.) ;
#54833=ORIENTED_EDGE('',*,*,#42128,.F.) ;
#54834=ORIENTED_EDGE('',*,*,#42129,.F.) ;
#54835=ORIENTED_EDGE('',*,*,#42126,.T.) ;
#54836=ORIENTED_EDGE('',*,*,#41854,.F.) ;
#54837=ORIENTED_EDGE('',*,*,#42130,.F.) ;
#54838=ORIENTED_EDGE('',*,*,#41962,.F.) ;
#54839=ORIENTED_EDGE('',*,*,#42127,.T.) ;
#54840=ORIENTED_EDGE('',*,*,#41961,.F.) ;
#54841=ORIENTED_EDGE('',*,*,#42131,.F.) ;
#54842=ORIENTED_EDGE('',*,*,#41947,.F.) ;
#54843=ORIENTED_EDGE('',*,*,#42132,.F.) ;
#54844=ORIENTED_EDGE('',*,*,#41948,.F.) ;
#54845=ORIENTED_EDGE('',*,*,#42133,.F.) ;
#54846=ORIENTED_EDGE('',*,*,#41966,.F.) ;
#54847=ORIENTED_EDGE('',*,*,#42128,.T.) ;
#54848=ORIENTED_EDGE('',*,*,#41949,.F.) ;
#54849=ORIENTED_EDGE('',*,*,#42134,.F.) ;
#54850=ORIENTED_EDGE('',*,*,#41954,.F.) ;
#54851=ORIENTED_EDGE('',*,*,#42129,.T.) ;
#54852=ORIENTED_EDGE('',*,*,#41953,.F.) ;
#54853=ORIENTED_EDGE('',*,*,#42135,.F.) ;
#54854=ORIENTED_EDGE('',*,*,#41858,.F.) ;
#54855=ORIENTED_EDGE('',*,*,#42136,.F.) ;
#54856=ORIENTED_EDGE('',*,*,#41852,.F.) ;
#54857=ORIENTED_EDGE('',*,*,#42137,.F.) ;
#54858=ORIENTED_EDGE('',*,*,#41957,.F.) ;
#54859=ORIENTED_EDGE('',*,*,#41853,.T.) ;
#54860=ORIENTED_EDGE('',*,*,#42136,.T.) ;
#54861=ORIENTED_EDGE('',*,*,#42138,.F.) ;
#54862=ORIENTED_EDGE('',*,*,#42130,.T.) ;
#54863=ORIENTED_EDGE('',*,*,#42133,.T.) ;
#54864=ORIENTED_EDGE('',*,*,#42131,.T.) ;
#54865=ORIENTED_EDGE('',*,*,#42139,.F.) ;
#54866=ORIENTED_EDGE('',*,*,#42134,.T.) ;
#54867=ORIENTED_EDGE('',*,*,#42132,.T.) ;
#54868=ORIENTED_EDGE('',*,*,#42140,.F.) ;
#54869=ORIENTED_EDGE('',*,*,#41851,.T.) ;
#54870=ORIENTED_EDGE('',*,*,#42135,.T.) ;
#54871=ORIENTED_EDGE('',*,*,#42141,.F.) ;
#54872=ORIENTED_EDGE('',*,*,#42137,.T.) ;
#54873=ORIENTED_EDGE('',*,*,#42138,.T.) ;
#54874=ORIENTED_EDGE('',*,*,#41956,.F.) ;
#54875=ORIENTED_EDGE('',*,*,#42142,.F.) ;
#54876=ORIENTED_EDGE('',*,*,#41959,.F.) ;
#54877=ORIENTED_EDGE('',*,*,#42139,.T.) ;
#54878=ORIENTED_EDGE('',*,*,#41960,.F.) ;
#54879=ORIENTED_EDGE('',*,*,#42143,.F.) ;
#54880=ORIENTED_EDGE('',*,*,#41963,.F.) ;
#54881=ORIENTED_EDGE('',*,*,#42140,.T.) ;
#54882=ORIENTED_EDGE('',*,*,#41965,.F.) ;
#54883=ORIENTED_EDGE('',*,*,#42144,.F.) ;
#54884=ORIENTED_EDGE('',*,*,#41951,.F.) ;
#54885=ORIENTED_EDGE('',*,*,#42141,.T.) ;
#54886=ORIENTED_EDGE('',*,*,#41952,.F.) ;
#54887=ORIENTED_EDGE('',*,*,#42145,.F.) ;
#54888=ORIENTED_EDGE('',*,*,#41958,.F.) ;
#54889=ORIENTED_EDGE('',*,*,#42143,.T.) ;
#54890=ORIENTED_EDGE('',*,*,#42142,.T.) ;
#54891=ORIENTED_EDGE('',*,*,#42146,.F.) ;
#54892=ORIENTED_EDGE('',*,*,#42145,.T.) ;
#54893=ORIENTED_EDGE('',*,*,#42144,.T.) ;
#54894=ORIENTED_EDGE('',*,*,#42147,.F.) ;
#54895=ORIENTED_EDGE('',*,*,#42146,.T.) ;
#54896=ORIENTED_EDGE('',*,*,#41955,.F.) ;
#54897=ORIENTED_EDGE('',*,*,#42147,.T.) ;
#54898=ORIENTED_EDGE('',*,*,#41964,.F.) ;
#54899=ORIENTED_EDGE('',*,*,#42148,.F.) ;
#54900=ORIENTED_EDGE('',*,*,#41806,.F.) ;
#54901=ORIENTED_EDGE('',*,*,#42149,.F.) ;
#54902=ORIENTED_EDGE('',*,*,#42009,.F.) ;
#54903=ORIENTED_EDGE('',*,*,#42149,.T.) ;
#54904=ORIENTED_EDGE('',*,*,#41805,.T.) ;
#54905=ORIENTED_EDGE('',*,*,#42150,.F.) ;
#54906=ORIENTED_EDGE('',*,*,#42151,.F.) ;
#54907=ORIENTED_EDGE('',*,*,#41807,.T.) ;
#54908=ORIENTED_EDGE('',*,*,#42148,.T.) ;
#54909=ORIENTED_EDGE('',*,*,#42152,.F.) ;
#54910=ORIENTED_EDGE('',*,*,#42153,.F.) ;
#54911=ORIENTED_EDGE('',*,*,#42150,.T.) ;
#54912=ORIENTED_EDGE('',*,*,#41804,.F.) ;
#54913=ORIENTED_EDGE('',*,*,#42154,.F.) ;
#54914=ORIENTED_EDGE('',*,*,#42005,.F.) ;
#54915=ORIENTED_EDGE('',*,*,#42151,.T.) ;
#54916=ORIENTED_EDGE('',*,*,#42004,.F.) ;
#54917=ORIENTED_EDGE('',*,*,#42155,.F.) ;
#54918=ORIENTED_EDGE('',*,*,#42006,.F.) ;
#54919=ORIENTED_EDGE('',*,*,#42156,.F.) ;
#54920=ORIENTED_EDGE('',*,*,#42007,.F.) ;
#54921=ORIENTED_EDGE('',*,*,#42157,.F.) ;
#54922=ORIENTED_EDGE('',*,*,#42017,.F.) ;
#54923=ORIENTED_EDGE('',*,*,#42152,.T.) ;
#54924=ORIENTED_EDGE('',*,*,#42008,.F.) ;
#54925=ORIENTED_EDGE('',*,*,#42158,.F.) ;
#54926=ORIENTED_EDGE('',*,*,#42013,.F.) ;
#54927=ORIENTED_EDGE('',*,*,#42153,.T.) ;
#54928=ORIENTED_EDGE('',*,*,#42012,.F.) ;
#54929=ORIENTED_EDGE('',*,*,#42159,.F.) ;
#54930=ORIENTED_EDGE('',*,*,#41808,.F.) ;
#54931=ORIENTED_EDGE('',*,*,#42160,.F.) ;
#54932=ORIENTED_EDGE('',*,*,#41802,.F.) ;
#54933=ORIENTED_EDGE('',*,*,#42161,.F.) ;
#54934=ORIENTED_EDGE('',*,*,#42000,.F.) ;
#54935=ORIENTED_EDGE('',*,*,#41803,.T.) ;
#54936=ORIENTED_EDGE('',*,*,#42160,.T.) ;
#54937=ORIENTED_EDGE('',*,*,#42162,.F.) ;
#54938=ORIENTED_EDGE('',*,*,#42154,.T.) ;
#54939=ORIENTED_EDGE('',*,*,#42157,.T.) ;
#54940=ORIENTED_EDGE('',*,*,#42155,.T.) ;
#54941=ORIENTED_EDGE('',*,*,#42163,.F.) ;
#54942=ORIENTED_EDGE('',*,*,#42158,.T.) ;
#54943=ORIENTED_EDGE('',*,*,#42156,.T.) ;
#54944=ORIENTED_EDGE('',*,*,#42164,.F.) ;
#54945=ORIENTED_EDGE('',*,*,#41801,.T.) ;
#54946=ORIENTED_EDGE('',*,*,#42159,.T.) ;
#54947=ORIENTED_EDGE('',*,*,#42165,.F.) ;
#54948=ORIENTED_EDGE('',*,*,#42161,.T.) ;
#54949=ORIENTED_EDGE('',*,*,#42162,.T.) ;
#54950=ORIENTED_EDGE('',*,*,#41999,.F.) ;
#54951=ORIENTED_EDGE('',*,*,#42166,.F.) ;
#54952=ORIENTED_EDGE('',*,*,#42002,.F.) ;
#54953=ORIENTED_EDGE('',*,*,#42163,.T.) ;
#54954=ORIENTED_EDGE('',*,*,#42003,.F.) ;
#54955=ORIENTED_EDGE('',*,*,#42167,.F.) ;
#54956=ORIENTED_EDGE('',*,*,#42014,.F.) ;
#54957=ORIENTED_EDGE('',*,*,#42164,.T.) ;
#54958=ORIENTED_EDGE('',*,*,#42016,.F.) ;
#54959=ORIENTED_EDGE('',*,*,#42168,.F.) ;
#54960=ORIENTED_EDGE('',*,*,#42010,.F.) ;
#54961=ORIENTED_EDGE('',*,*,#42165,.T.) ;
#54962=ORIENTED_EDGE('',*,*,#42011,.F.) ;
#54963=ORIENTED_EDGE('',*,*,#42169,.F.) ;
#54964=ORIENTED_EDGE('',*,*,#42001,.F.) ;
#54965=ORIENTED_EDGE('',*,*,#42167,.T.) ;
#54966=ORIENTED_EDGE('',*,*,#42166,.T.) ;
#54967=ORIENTED_EDGE('',*,*,#42170,.F.) ;
#54968=ORIENTED_EDGE('',*,*,#42169,.T.) ;
#54969=ORIENTED_EDGE('',*,*,#42168,.T.) ;
#54970=ORIENTED_EDGE('',*,*,#42171,.F.) ;
#54971=ORIENTED_EDGE('',*,*,#42170,.T.) ;
#54972=ORIENTED_EDGE('',*,*,#41998,.F.) ;
#54973=ORIENTED_EDGE('',*,*,#42171,.T.) ;
#54974=ORIENTED_EDGE('',*,*,#42015,.F.) ;
#54975=ORIENTED_EDGE('',*,*,#41879,.F.) ;
#54976=ORIENTED_EDGE('',*,*,#42172,.T.) ;
#54977=ORIENTED_EDGE('',*,*,#42061,.F.) ;
#54978=ORIENTED_EDGE('',*,*,#42173,.F.) ;
#54979=ORIENTED_EDGE('',*,*,#41893,.F.) ;
#54980=ORIENTED_EDGE('',*,*,#41880,.F.) ;
#54981=ORIENTED_EDGE('',*,*,#42174,.F.) ;
#54982=ORIENTED_EDGE('',*,*,#41736,.F.) ;
#54983=ORIENTED_EDGE('',*,*,#42174,.T.) ;
#54984=ORIENTED_EDGE('',*,*,#42173,.T.) ;
#54985=ORIENTED_EDGE('',*,*,#42175,.F.) ;
#54986=ORIENTED_EDGE('',*,*,#42175,.T.) ;
#54987=ORIENTED_EDGE('',*,*,#42066,.F.) ;
#54988=ORIENTED_EDGE('',*,*,#42176,.F.) ;
#54989=ORIENTED_EDGE('',*,*,#41737,.F.) ;
#54990=ORIENTED_EDGE('',*,*,#41894,.F.) ;
#54991=ORIENTED_EDGE('',*,*,#41738,.F.) ;
#54992=ORIENTED_EDGE('',*,*,#42177,.F.) ;
#54993=ORIENTED_EDGE('',*,*,#41747,.F.) ;
#54994=ORIENTED_EDGE('',*,*,#42177,.T.) ;
#54995=ORIENTED_EDGE('',*,*,#42176,.T.) ;
#54996=ORIENTED_EDGE('',*,*,#42178,.F.) ;
#54997=ORIENTED_EDGE('',*,*,#41748,.T.) ;
#54998=ORIENTED_EDGE('',*,*,#42178,.T.) ;
#54999=ORIENTED_EDGE('',*,*,#42065,.F.) ;
#55000=ORIENTED_EDGE('',*,*,#42179,.F.) ;
#55001=ORIENTED_EDGE('',*,*,#41749,.F.) ;
#55002=ORIENTED_EDGE('',*,*,#41884,.F.) ;
#55003=ORIENTED_EDGE('',*,*,#42180,.F.) ;
#55004=ORIENTED_EDGE('',*,*,#41751,.F.) ;
#55005=ORIENTED_EDGE('',*,*,#42181,.F.) ;
#55006=ORIENTED_EDGE('',*,*,#41750,.T.) ;
#55007=ORIENTED_EDGE('',*,*,#42179,.T.) ;
#55008=ORIENTED_EDGE('',*,*,#42182,.F.) ;
#55009=ORIENTED_EDGE('',*,*,#42181,.T.) ;
#55010=ORIENTED_EDGE('',*,*,#42182,.T.) ;
#55011=ORIENTED_EDGE('',*,*,#42064,.F.) ;
#55012=ORIENTED_EDGE('',*,*,#42183,.F.) ;
#55013=ORIENTED_EDGE('',*,*,#41881,.F.) ;
#55014=ORIENTED_EDGE('',*,*,#41734,.F.) ;
#55015=ORIENTED_EDGE('',*,*,#42184,.F.) ;
#55016=ORIENTED_EDGE('',*,*,#41882,.F.) ;
#55017=ORIENTED_EDGE('',*,*,#42185,.F.) ;
#55018=ORIENTED_EDGE('',*,*,#42185,.T.) ;
#55019=ORIENTED_EDGE('',*,*,#42183,.T.) ;
#55020=ORIENTED_EDGE('',*,*,#42186,.F.) ;
#55021=ORIENTED_EDGE('',*,*,#42063,.F.) ;
#55022=ORIENTED_EDGE('',*,*,#42187,.T.) ;
#55023=ORIENTED_EDGE('',*,*,#41731,.F.) ;
#55024=ORIENTED_EDGE('',*,*,#42186,.T.) ;
#55025=ORIENTED_EDGE('',*,*,#41891,.F.) ;
#55026=ORIENTED_EDGE('',*,*,#41861,.F.) ;
#55027=ORIENTED_EDGE('',*,*,#42188,.F.) ;
#55028=ORIENTED_EDGE('',*,*,#41869,.F.) ;
#55029=ORIENTED_EDGE('',*,*,#41890,.F.) ;
#55030=ORIENTED_EDGE('',*,*,#41841,.F.) ;
#55031=ORIENTED_EDGE('',*,*,#42189,.F.) ;
#55032=ORIENTED_EDGE('',*,*,#41859,.F.) ;
#55033=ORIENTED_EDGE('',*,*,#41889,.F.) ;
#55034=ORIENTED_EDGE('',*,*,#41821,.F.) ;
#55035=ORIENTED_EDGE('',*,*,#42190,.F.) ;
#55036=ORIENTED_EDGE('',*,*,#41839,.F.) ;
#55037=ORIENTED_EDGE('',*,*,#41888,.F.) ;
#55038=ORIENTED_EDGE('',*,*,#41817,.F.) ;
#55039=ORIENTED_EDGE('',*,*,#42191,.F.) ;
#55040=ORIENTED_EDGE('',*,*,#41819,.F.) ;
#55041=ORIENTED_EDGE('',*,*,#41887,.F.) ;
#55042=ORIENTED_EDGE('',*,*,#41811,.F.) ;
#55043=ORIENTED_EDGE('',*,*,#42192,.F.) ;
#55044=ORIENTED_EDGE('',*,*,#41813,.F.) ;
#55045=ORIENTED_EDGE('',*,*,#41886,.F.) ;
#55046=ORIENTED_EDGE('',*,*,#41791,.F.) ;
#55047=ORIENTED_EDGE('',*,*,#42193,.F.) ;
#55048=ORIENTED_EDGE('',*,*,#41809,.F.) ;
#55049=ORIENTED_EDGE('',*,*,#41680,.F.) ;
#55050=ORIENTED_EDGE('',*,*,#41994,.F.) ;
#55051=ORIENTED_EDGE('',*,*,#41690,.F.) ;
#55052=ORIENTED_EDGE('',*,*,#41996,.F.) ;
#55053=ORIENTED_EDGE('',*,*,#41688,.F.) ;
#55054=ORIENTED_EDGE('',*,*,#41992,.F.) ;
#55055=ORIENTED_EDGE('',*,*,#41682,.F.) ;
#55056=ORIENTED_EDGE('',*,*,#41997,.F.) ;
#55057=ORIENTED_EDGE('',*,*,#41678,.F.) ;
#55058=ORIENTED_EDGE('',*,*,#41743,.F.) ;
#55059=ORIENTED_EDGE('',*,*,#41692,.F.) ;
#55060=ORIENTED_EDGE('',*,*,#41995,.F.) ;
#55061=ORIENTED_EDGE('',*,*,#41686,.F.) ;
#55062=ORIENTED_EDGE('',*,*,#41991,.F.) ;
#55063=ORIENTED_EDGE('',*,*,#41684,.F.) ;
#55064=ORIENTED_EDGE('',*,*,#41993,.F.) ;
#55065=ORIENTED_EDGE('',*,*,#41885,.F.) ;
#55066=ORIENTED_EDGE('',*,*,#41786,.F.) ;
#55067=ORIENTED_EDGE('',*,*,#42194,.F.) ;
#55068=ORIENTED_EDGE('',*,*,#41789,.F.) ;
#55069=ORIENTED_EDGE('',*,*,#41898,.F.) ;
#55070=ORIENTED_EDGE('',*,*,#41696,.F.) ;
#55071=ORIENTED_EDGE('',*,*,#42195,.F.) ;
#55072=ORIENTED_EDGE('',*,*,#41782,.F.) ;
#55073=ORIENTED_EDGE('',*,*,#41897,.F.) ;
#55074=ORIENTED_EDGE('',*,*,#41781,.F.) ;
#55075=ORIENTED_EDGE('',*,*,#42196,.F.) ;
#55076=ORIENTED_EDGE('',*,*,#41698,.F.) ;
#55077=ORIENTED_EDGE('',*,*,#42197,.F.) ;
#55078=ORIENTED_EDGE('',*,*,#41669,.F.) ;
#55079=ORIENTED_EDGE('',*,*,#42110,.F.) ;
#55080=ORIENTED_EDGE('',*,*,#42197,.T.) ;
#55081=ORIENTED_EDGE('',*,*,#42058,.F.) ;
#55082=ORIENTED_EDGE('',*,*,#42198,.F.) ;
#55083=ORIENTED_EDGE('',*,*,#42053,.F.) ;
#55084=ORIENTED_EDGE('',*,*,#42198,.T.) ;
#55085=ORIENTED_EDGE('',*,*,#42057,.F.) ;
#55086=ORIENTED_EDGE('',*,*,#42199,.F.) ;
#55087=ORIENTED_EDGE('',*,*,#42115,.F.) ;
#55088=ORIENTED_EDGE('',*,*,#42199,.T.) ;
#55089=ORIENTED_EDGE('',*,*,#42108,.F.) ;
#55090=ORIENTED_EDGE('',*,*,#42200,.F.) ;
#55091=ORIENTED_EDGE('',*,*,#42113,.F.) ;
#55092=ORIENTED_EDGE('',*,*,#42200,.T.) ;
#55093=ORIENTED_EDGE('',*,*,#41772,.F.) ;
#55094=ORIENTED_EDGE('',*,*,#42201,.F.) ;
#55095=ORIENTED_EDGE('',*,*,#42114,.F.) ;
#55096=ORIENTED_EDGE('',*,*,#42201,.T.) ;
#55097=ORIENTED_EDGE('',*,*,#41771,.F.) ;
#55098=ORIENTED_EDGE('',*,*,#41896,.F.) ;
#55099=ORIENTED_EDGE('',*,*,#41767,.F.) ;
#55100=ORIENTED_EDGE('',*,*,#41741,.F.) ;
#55101=ORIENTED_EDGE('',*,*,#42202,.T.) ;
#55102=ORIENTED_EDGE('',*,*,#41775,.F.) ;
#55103=ORIENTED_EDGE('',*,*,#42203,.F.) ;
#55104=ORIENTED_EDGE('',*,*,#42203,.T.) ;
#55105=ORIENTED_EDGE('',*,*,#41774,.F.) ;
#55106=ORIENTED_EDGE('',*,*,#42204,.F.) ;
#55107=ORIENTED_EDGE('',*,*,#42103,.F.) ;
#55108=ORIENTED_EDGE('',*,*,#42204,.T.) ;
#55109=ORIENTED_EDGE('',*,*,#42109,.F.) ;
#55110=ORIENTED_EDGE('',*,*,#41645,.F.) ;
#55111=ORIENTED_EDGE('',*,*,#42104,.F.) ;
#55112=ORIENTED_EDGE('',*,*,#42205,.F.) ;
#55113=ORIENTED_EDGE('',*,*,#42047,.F.) ;
#55114=ORIENTED_EDGE('',*,*,#41643,.T.) ;
#55115=ORIENTED_EDGE('',*,*,#42060,.F.) ;
#55116=ORIENTED_EDGE('',*,*,#42111,.F.) ;
#55117=ORIENTED_EDGE('',*,*,#42105,.F.) ;
#55118=ORIENTED_EDGE('',*,*,#42205,.T.) ;
#55119=ORIENTED_EDGE('',*,*,#42206,.T.) ;
#55120=ORIENTED_EDGE('',*,*,#42207,.T.) ;
#55121=ORIENTED_EDGE('',*,*,#42062,.F.) ;
#55122=ORIENTED_EDGE('',*,*,#42208,.T.) ;
#55123=ORIENTED_EDGE('',*,*,#42209,.T.) ;
#55124=ORIENTED_EDGE('',*,*,#41892,.F.) ;
#55125=ORIENTED_EDGE('',*,*,#41867,.F.) ;
#55126=ORIENTED_EDGE('',*,*,#42210,.F.) ;
#55127=ORIENTED_EDGE('',*,*,#41878,.F.) ;
#55128=ORIENTED_EDGE('',*,*,#41866,.F.) ;
#55129=ORIENTED_EDGE('',*,*,#42211,.T.) ;
#55130=ORIENTED_EDGE('',*,*,#42172,.F.) ;
#55131=ORIENTED_EDGE('',*,*,#42210,.T.) ;
#55132=ORIENTED_EDGE('',*,*,#41876,.F.) ;
#55133=ORIENTED_EDGE('',*,*,#42212,.F.) ;
#55134=ORIENTED_EDGE('',*,*,#41732,.F.) ;
#55135=ORIENTED_EDGE('',*,*,#42213,.F.) ;
#55136=ORIENTED_EDGE('',*,*,#42187,.F.) ;
#55137=ORIENTED_EDGE('',*,*,#42214,.T.) ;
#55138=ORIENTED_EDGE('',*,*,#41863,.F.) ;
#55139=ORIENTED_EDGE('',*,*,#42213,.T.) ;
#55140=ORIENTED_EDGE('',*,*,#42208,.F.) ;
#55141=ORIENTED_EDGE('',*,*,#42211,.F.) ;
#55142=ORIENTED_EDGE('',*,*,#42215,.F.) ;
#55143=ORIENTED_EDGE('',*,*,#42216,.F.) ;
#55144=ORIENTED_EDGE('',*,*,#42209,.F.) ;
#55145=ORIENTED_EDGE('',*,*,#42215,.T.) ;
#55146=ORIENTED_EDGE('',*,*,#41865,.F.) ;
#55147=ORIENTED_EDGE('',*,*,#42216,.T.) ;
#55148=ORIENTED_EDGE('',*,*,#41864,.F.) ;
#55149=ORIENTED_EDGE('',*,*,#42217,.F.) ;
#55150=ORIENTED_EDGE('',*,*,#42206,.F.) ;
#55151=ORIENTED_EDGE('',*,*,#42217,.T.) ;
#55152=ORIENTED_EDGE('',*,*,#42214,.F.) ;
#55153=ORIENTED_EDGE('',*,*,#42207,.F.) ;
#55154=ORIENTED_EDGE('',*,*,#41720,.F.) ;
#55155=ORIENTED_EDGE('',*,*,#41788,.T.) ;
#55156=ORIENTED_EDGE('',*,*,#41726,.F.) ;
#55157=ORIENTED_EDGE('',*,*,#41707,.T.) ;
#55158=ORIENTED_EDGE('',*,*,#41724,.T.) ;
#55159=ORIENTED_EDGE('',*,*,#41711,.T.) ;
#55160=ORIENTED_EDGE('',*,*,#41722,.T.) ;
#55161=ORIENTED_EDGE('',*,*,#41715,.T.) ;
#55162=ORIENTED_EDGE('',*,*,#42218,.T.) ;
#55163=ORIENTED_EDGE('',*,*,#42219,.T.) ;
#55164=ORIENTED_EDGE('',*,*,#42220,.F.) ;
#55165=ORIENTED_EDGE('',*,*,#42221,.T.) ;
#55166=ORIENTED_EDGE('',*,*,#42220,.T.) ;
#55167=ORIENTED_EDGE('',*,*,#42222,.T.) ;
#55168=ORIENTED_EDGE('',*,*,#42223,.F.) ;
#55169=ORIENTED_EDGE('',*,*,#42224,.T.) ;
#55170=ORIENTED_EDGE('',*,*,#42223,.T.) ;
#55171=ORIENTED_EDGE('',*,*,#42225,.T.) ;
#55172=ORIENTED_EDGE('',*,*,#42226,.F.) ;
#55173=ORIENTED_EDGE('',*,*,#42227,.T.) ;
#55174=ORIENTED_EDGE('',*,*,#42226,.T.) ;
#55175=ORIENTED_EDGE('',*,*,#42228,.T.) ;
#55176=ORIENTED_EDGE('',*,*,#42229,.F.) ;
#55177=ORIENTED_EDGE('',*,*,#42230,.T.) ;
#55178=ORIENTED_EDGE('',*,*,#42229,.T.) ;
#55179=ORIENTED_EDGE('',*,*,#42231,.T.) ;
#55180=ORIENTED_EDGE('',*,*,#42232,.F.) ;
#55181=ORIENTED_EDGE('',*,*,#42233,.T.) ;
#55182=ORIENTED_EDGE('',*,*,#42232,.T.) ;
#55183=ORIENTED_EDGE('',*,*,#42234,.T.) ;
#55184=ORIENTED_EDGE('',*,*,#42235,.F.) ;
#55185=ORIENTED_EDGE('',*,*,#42236,.T.) ;
#55186=ORIENTED_EDGE('',*,*,#42235,.T.) ;
#55187=ORIENTED_EDGE('',*,*,#42237,.T.) ;
#55188=ORIENTED_EDGE('',*,*,#42238,.F.) ;
#55189=ORIENTED_EDGE('',*,*,#42239,.T.) ;
#55190=ORIENTED_EDGE('',*,*,#42238,.T.) ;
#55191=ORIENTED_EDGE('',*,*,#42240,.T.) ;
#55192=ORIENTED_EDGE('',*,*,#42241,.F.) ;
#55193=ORIENTED_EDGE('',*,*,#42242,.T.) ;
#55194=ORIENTED_EDGE('',*,*,#42241,.T.) ;
#55195=ORIENTED_EDGE('',*,*,#42243,.T.) ;
#55196=ORIENTED_EDGE('',*,*,#42244,.T.) ;
#55197=ORIENTED_EDGE('',*,*,#42245,.T.) ;
#55198=ORIENTED_EDGE('',*,*,#42246,.T.) ;
#55199=ORIENTED_EDGE('',*,*,#42247,.T.) ;
#55200=ORIENTED_EDGE('',*,*,#42248,.T.) ;
#55201=ORIENTED_EDGE('',*,*,#42249,.T.) ;
#55202=ORIENTED_EDGE('',*,*,#42250,.T.) ;
#55203=ORIENTED_EDGE('',*,*,#42251,.T.) ;
#55204=ORIENTED_EDGE('',*,*,#42252,.T.) ;
#55205=ORIENTED_EDGE('',*,*,#42253,.T.) ;
#55206=ORIENTED_EDGE('',*,*,#42254,.T.) ;
#55207=ORIENTED_EDGE('',*,*,#42255,.T.) ;
#55208=ORIENTED_EDGE('',*,*,#42256,.T.) ;
#55209=ORIENTED_EDGE('',*,*,#42257,.T.) ;
#55210=ORIENTED_EDGE('',*,*,#42258,.T.) ;
#55211=ORIENTED_EDGE('',*,*,#42259,.T.) ;
#55212=ORIENTED_EDGE('',*,*,#42260,.T.) ;
#55213=ORIENTED_EDGE('',*,*,#42261,.T.) ;
#55214=ORIENTED_EDGE('',*,*,#42262,.T.) ;
#55215=ORIENTED_EDGE('',*,*,#42263,.T.) ;
#55216=ORIENTED_EDGE('',*,*,#42264,.T.) ;
#55217=ORIENTED_EDGE('',*,*,#42265,.T.) ;
#55218=ORIENTED_EDGE('',*,*,#42266,.T.) ;
#55219=ORIENTED_EDGE('',*,*,#42267,.T.) ;
#55220=ORIENTED_EDGE('',*,*,#41624,.T.) ;
#55221=ORIENTED_EDGE('',*,*,#41640,.T.) ;
#55222=ORIENTED_EDGE('',*,*,#42268,.T.) ;
#55223=ORIENTED_EDGE('',*,*,#42269,.T.) ;
#55224=ORIENTED_EDGE('',*,*,#42270,.T.) ;
#55225=ORIENTED_EDGE('',*,*,#42271,.T.) ;
#55226=ORIENTED_EDGE('',*,*,#42272,.T.) ;
#55227=ORIENTED_EDGE('',*,*,#42262,.F.) ;
#55228=ORIENTED_EDGE('',*,*,#42273,.T.) ;
#55229=ORIENTED_EDGE('',*,*,#41870,.F.) ;
#55230=ORIENTED_EDGE('',*,*,#42188,.T.) ;
#55231=ORIENTED_EDGE('',*,*,#41860,.F.) ;
#55232=ORIENTED_EDGE('',*,*,#42189,.T.) ;
#55233=ORIENTED_EDGE('',*,*,#41840,.F.) ;
#55234=ORIENTED_EDGE('',*,*,#42190,.T.) ;
#55235=ORIENTED_EDGE('',*,*,#41820,.F.) ;
#55236=ORIENTED_EDGE('',*,*,#42191,.T.) ;
#55237=ORIENTED_EDGE('',*,*,#41816,.F.) ;
#55238=ORIENTED_EDGE('',*,*,#41646,.T.) ;
#55239=ORIENTED_EDGE('',*,*,#41814,.F.) ;
#55240=ORIENTED_EDGE('',*,*,#42192,.T.) ;
#55241=ORIENTED_EDGE('',*,*,#41810,.F.) ;
#55242=ORIENTED_EDGE('',*,*,#42193,.T.) ;
#55243=ORIENTED_EDGE('',*,*,#41790,.F.) ;
#55244=ORIENTED_EDGE('',*,*,#42194,.T.) ;
#55245=ORIENTED_EDGE('',*,*,#41785,.F.) ;
#55246=ORIENTED_EDGE('',*,*,#41721,.T.) ;
#55247=ORIENTED_EDGE('',*,*,#41717,.F.) ;
#55248=ORIENTED_EDGE('',*,*,#41723,.T.) ;
#55249=ORIENTED_EDGE('',*,*,#41713,.F.) ;
#55250=ORIENTED_EDGE('',*,*,#41725,.T.) ;
#55251=ORIENTED_EDGE('',*,*,#41709,.F.) ;
#55252=ORIENTED_EDGE('',*,*,#41730,.T.) ;
#55253=ORIENTED_EDGE('',*,*,#41783,.F.) ;
#55254=ORIENTED_EDGE('',*,*,#42195,.T.) ;
#55255=ORIENTED_EDGE('',*,*,#41695,.F.) ;
#55256=ORIENTED_EDGE('',*,*,#42196,.T.) ;
#55257=ORIENTED_EDGE('',*,*,#41780,.F.) ;
#55258=ORIENTED_EDGE('',*,*,#42274,.T.) ;
#55259=ORIENTED_EDGE('',*,*,#42264,.F.) ;
#55260=ORIENTED_EDGE('',*,*,#42275,.T.) ;
#55261=ORIENTED_EDGE('',*,*,#41756,.F.) ;
#55262=ORIENTED_EDGE('',*,*,#42276,.T.) ;
#55263=ORIENTED_EDGE('',*,*,#42271,.F.) ;
#55264=ORIENTED_EDGE('',*,*,#42277,.T.) ;
#55265=ORIENTED_EDGE('',*,*,#42278,.T.) ;
#55266=ORIENTED_EDGE('',*,*,#42279,.T.) ;
#55267=ORIENTED_EDGE('',*,*,#42280,.T.) ;
#55268=ORIENTED_EDGE('',*,*,#42281,.T.) ;
#55269=ORIENTED_EDGE('',*,*,#42282,.T.) ;
#55270=ORIENTED_EDGE('',*,*,#42283,.T.) ;
#55271=ORIENTED_EDGE('',*,*,#42284,.T.) ;
#55272=ORIENTED_EDGE('',*,*,#42285,.T.) ;
#55273=ORIENTED_EDGE('',*,*,#42286,.F.) ;
#55274=ORIENTED_EDGE('',*,*,#42287,.T.) ;
#55275=ORIENTED_EDGE('',*,*,#42288,.T.) ;
#55276=ORIENTED_EDGE('',*,*,#42289,.T.) ;
#55277=ORIENTED_EDGE('',*,*,#42290,.F.) ;
#55278=ORIENTED_EDGE('',*,*,#42291,.T.) ;
#55279=ORIENTED_EDGE('',*,*,#42292,.T.) ;
#55280=ORIENTED_EDGE('',*,*,#42293,.T.) ;
#55281=ORIENTED_EDGE('',*,*,#42294,.T.) ;
#55282=ORIENTED_EDGE('',*,*,#42295,.T.) ;
#55283=ORIENTED_EDGE('',*,*,#42296,.F.) ;
#55284=ORIENTED_EDGE('',*,*,#42297,.T.) ;
#55285=ORIENTED_EDGE('',*,*,#42288,.F.) ;
#55286=ORIENTED_EDGE('',*,*,#42298,.T.) ;
#55287=ORIENTED_EDGE('',*,*,#42299,.T.) ;
#55288=ORIENTED_EDGE('',*,*,#42300,.T.) ;
#55289=ORIENTED_EDGE('',*,*,#42301,.F.) ;
#55290=ORIENTED_EDGE('',*,*,#42302,.T.) ;
#55291=ORIENTED_EDGE('',*,*,#42294,.F.) ;
#55292=ORIENTED_EDGE('',*,*,#42303,.T.) ;
#55293=ORIENTED_EDGE('',*,*,#42304,.F.) ;
#55294=ORIENTED_EDGE('',*,*,#42305,.T.) ;
#55295=ORIENTED_EDGE('',*,*,#42306,.T.) ;
#55296=ORIENTED_EDGE('',*,*,#42307,.T.) ;
#55297=ORIENTED_EDGE('',*,*,#42299,.F.) ;
#55298=ORIENTED_EDGE('',*,*,#42308,.T.) ;
#55299=ORIENTED_EDGE('',*,*,#42309,.T.) ;
#55300=ORIENTED_EDGE('',*,*,#42310,.T.) ;
#55301=ORIENTED_EDGE('',*,*,#42296,.T.) ;
#55302=ORIENTED_EDGE('',*,*,#42311,.T.) ;
#55303=ORIENTED_EDGE('',*,*,#42312,.T.) ;
#55304=ORIENTED_EDGE('',*,*,#42313,.T.) ;
#55305=ORIENTED_EDGE('',*,*,#42314,.T.) ;
#55306=ORIENTED_EDGE('',*,*,#42315,.T.) ;
#55307=ORIENTED_EDGE('',*,*,#42316,.T.) ;
#55308=ORIENTED_EDGE('',*,*,#42317,.T.) ;
#55309=ORIENTED_EDGE('',*,*,#42318,.T.) ;
#55310=ORIENTED_EDGE('',*,*,#42319,.T.) ;
#55311=ORIENTED_EDGE('',*,*,#42320,.T.) ;
#55312=ORIENTED_EDGE('',*,*,#42321,.T.) ;
#55313=ORIENTED_EDGE('',*,*,#42322,.T.) ;
#55314=ORIENTED_EDGE('',*,*,#42323,.T.) ;
#55315=ORIENTED_EDGE('',*,*,#42324,.T.) ;
#55316=ORIENTED_EDGE('',*,*,#42325,.T.) ;
#55317=ORIENTED_EDGE('',*,*,#42326,.T.) ;
#55318=ORIENTED_EDGE('',*,*,#42327,.T.) ;
#55319=ORIENTED_EDGE('',*,*,#42328,.T.) ;
#55320=ORIENTED_EDGE('',*,*,#42329,.T.) ;
#55321=ORIENTED_EDGE('',*,*,#42330,.T.) ;
#55322=ORIENTED_EDGE('',*,*,#42331,.T.) ;
#55323=ORIENTED_EDGE('',*,*,#42332,.T.) ;
#55324=ORIENTED_EDGE('',*,*,#42333,.T.) ;
#55325=ORIENTED_EDGE('',*,*,#42334,.T.) ;
#55326=ORIENTED_EDGE('',*,*,#42335,.T.) ;
#55327=ORIENTED_EDGE('',*,*,#42336,.T.) ;
#55328=ORIENTED_EDGE('',*,*,#42337,.T.) ;
#55329=ORIENTED_EDGE('',*,*,#42338,.T.) ;
#55330=ORIENTED_EDGE('',*,*,#42339,.T.) ;
#55331=ORIENTED_EDGE('',*,*,#42340,.T.) ;
#55332=ORIENTED_EDGE('',*,*,#42341,.T.) ;
#55333=ORIENTED_EDGE('',*,*,#42342,.T.) ;
#55334=ORIENTED_EDGE('',*,*,#42343,.T.) ;
#55335=ORIENTED_EDGE('',*,*,#42344,.T.) ;
#55336=ORIENTED_EDGE('',*,*,#42345,.T.) ;
#55337=ORIENTED_EDGE('',*,*,#42346,.F.) ;
#55338=ORIENTED_EDGE('',*,*,#42347,.F.) ;
#55339=ORIENTED_EDGE('',*,*,#42348,.F.) ;
#55340=ORIENTED_EDGE('',*,*,#42349,.F.) ;
#55341=ORIENTED_EDGE('',*,*,#42350,.F.) ;
#55342=ORIENTED_EDGE('',*,*,#42351,.F.) ;
#55343=ORIENTED_EDGE('',*,*,#42352,.F.) ;
#55344=ORIENTED_EDGE('',*,*,#42353,.F.) ;
#55345=ORIENTED_EDGE('',*,*,#42354,.F.) ;
#55346=ORIENTED_EDGE('',*,*,#42355,.F.) ;
#55347=ORIENTED_EDGE('',*,*,#42353,.T.) ;
#55348=ORIENTED_EDGE('',*,*,#42356,.T.) ;
#55349=ORIENTED_EDGE('',*,*,#42357,.F.) ;
#55350=ORIENTED_EDGE('',*,*,#42358,.F.) ;
#55351=ORIENTED_EDGE('',*,*,#42346,.T.) ;
#55352=ORIENTED_EDGE('',*,*,#42355,.T.) ;
#55353=ORIENTED_EDGE('',*,*,#42359,.F.) ;
#55354=ORIENTED_EDGE('',*,*,#42360,.F.) ;
#55355=ORIENTED_EDGE('',*,*,#42347,.T.) ;
#55356=ORIENTED_EDGE('',*,*,#42358,.T.) ;
#55357=ORIENTED_EDGE('',*,*,#42361,.F.) ;
#55358=ORIENTED_EDGE('',*,*,#42362,.F.) ;
#55359=ORIENTED_EDGE('',*,*,#42348,.T.) ;
#55360=ORIENTED_EDGE('',*,*,#42360,.T.) ;
#55361=ORIENTED_EDGE('',*,*,#42363,.F.) ;
#55362=ORIENTED_EDGE('',*,*,#42364,.F.) ;
#55363=ORIENTED_EDGE('',*,*,#42349,.T.) ;
#55364=ORIENTED_EDGE('',*,*,#42362,.T.) ;
#55365=ORIENTED_EDGE('',*,*,#42365,.F.) ;
#55366=ORIENTED_EDGE('',*,*,#42366,.F.) ;
#55367=ORIENTED_EDGE('',*,*,#42350,.T.) ;
#55368=ORIENTED_EDGE('',*,*,#42364,.T.) ;
#55369=ORIENTED_EDGE('',*,*,#42367,.F.) ;
#55370=ORIENTED_EDGE('',*,*,#42368,.F.) ;
#55371=ORIENTED_EDGE('',*,*,#42351,.T.) ;
#55372=ORIENTED_EDGE('',*,*,#42366,.T.) ;
#55373=ORIENTED_EDGE('',*,*,#42369,.F.) ;
#55374=ORIENTED_EDGE('',*,*,#42356,.F.) ;
#55375=ORIENTED_EDGE('',*,*,#42352,.T.) ;
#55376=ORIENTED_EDGE('',*,*,#42368,.T.) ;
#55377=ORIENTED_EDGE('',*,*,#42357,.T.) ;
#55378=ORIENTED_EDGE('',*,*,#42354,.T.) ;
#55379=ORIENTED_EDGE('',*,*,#42369,.T.) ;
#55380=ORIENTED_EDGE('',*,*,#42367,.T.) ;
#55381=ORIENTED_EDGE('',*,*,#42365,.T.) ;
#55382=ORIENTED_EDGE('',*,*,#42363,.T.) ;
#55383=ORIENTED_EDGE('',*,*,#42361,.T.) ;
#55384=ORIENTED_EDGE('',*,*,#42359,.T.) ;
#55385=ORIENTED_EDGE('',*,*,#41632,.T.) ;
#55386=ORIENTED_EDGE('',*,*,#42370,.T.) ;
#55387=ORIENTED_EDGE('',*,*,#41630,.F.) ;
#55388=ORIENTED_EDGE('',*,*,#42371,.T.) ;
#55389=ORIENTED_EDGE('',*,*,#41634,.T.) ;
#55390=ORIENTED_EDGE('',*,*,#42372,.T.) ;
#55391=ORIENTED_EDGE('',*,*,#41638,.F.) ;
#55392=ORIENTED_EDGE('',*,*,#42373,.T.) ;
#55393=ORIENTED_EDGE('',*,*,#41626,.T.) ;
#55394=ORIENTED_EDGE('',*,*,#42374,.T.) ;
#55395=ORIENTED_EDGE('',*,*,#41628,.T.) ;
#55396=ORIENTED_EDGE('',*,*,#42375,.T.) ;
#55397=ORIENTED_EDGE('',*,*,#41636,.T.) ;
#55398=ORIENTED_EDGE('',*,*,#42376,.T.) ;
#55399=ORIENTED_EDGE('',*,*,#42377,.T.) ;
#55400=ORIENTED_EDGE('',*,*,#42378,.T.) ;
#55401=ORIENTED_EDGE('',*,*,#42379,.T.) ;
#55402=ORIENTED_EDGE('',*,*,#42380,.T.) ;
#55403=ORIENTED_EDGE('',*,*,#42381,.T.) ;
#55404=ORIENTED_EDGE('',*,*,#42382,.T.) ;
#55405=ORIENTED_EDGE('',*,*,#42383,.T.) ;
#55406=ORIENTED_EDGE('',*,*,#42384,.T.) ;
#55407=ORIENTED_EDGE('',*,*,#42385,.T.) ;
#55408=ORIENTED_EDGE('',*,*,#42386,.T.) ;
#55409=ORIENTED_EDGE('',*,*,#42387,.T.) ;
#55410=ORIENTED_EDGE('',*,*,#42388,.T.) ;
#55411=ORIENTED_EDGE('',*,*,#42389,.T.) ;
#55412=ORIENTED_EDGE('',*,*,#42390,.T.) ;
#55413=ORIENTED_EDGE('',*,*,#42391,.T.) ;
#55414=ORIENTED_EDGE('',*,*,#42392,.T.) ;
#55415=ORIENTED_EDGE('',*,*,#42393,.T.) ;
#55416=ORIENTED_EDGE('',*,*,#42394,.T.) ;
#55417=ORIENTED_EDGE('',*,*,#42395,.T.) ;
#55418=ORIENTED_EDGE('',*,*,#42396,.T.) ;
#55419=ORIENTED_EDGE('',*,*,#42397,.F.) ;
#55420=ORIENTED_EDGE('',*,*,#42398,.F.) ;
#55421=ORIENTED_EDGE('',*,*,#42399,.F.) ;
#55422=ORIENTED_EDGE('',*,*,#42400,.F.) ;
#55423=ORIENTED_EDGE('',*,*,#42401,.F.) ;
#55424=ORIENTED_EDGE('',*,*,#42402,.F.) ;
#55425=ORIENTED_EDGE('',*,*,#42403,.F.) ;
#55426=ORIENTED_EDGE('',*,*,#42404,.F.) ;
#55427=ORIENTED_EDGE('',*,*,#42405,.T.) ;
#55428=ORIENTED_EDGE('',*,*,#42406,.T.) ;
#55429=ORIENTED_EDGE('',*,*,#42407,.F.) ;
#55430=ORIENTED_EDGE('',*,*,#42404,.T.) ;
#55431=ORIENTED_EDGE('',*,*,#42407,.T.) ;
#55432=ORIENTED_EDGE('',*,*,#42408,.T.) ;
#55433=ORIENTED_EDGE('',*,*,#42409,.F.) ;
#55434=ORIENTED_EDGE('',*,*,#42397,.T.) ;
#55435=ORIENTED_EDGE('',*,*,#42409,.T.) ;
#55436=ORIENTED_EDGE('',*,*,#42410,.T.) ;
#55437=ORIENTED_EDGE('',*,*,#42411,.F.) ;
#55438=ORIENTED_EDGE('',*,*,#42398,.T.) ;
#55439=ORIENTED_EDGE('',*,*,#42411,.T.) ;
#55440=ORIENTED_EDGE('',*,*,#42412,.T.) ;
#55441=ORIENTED_EDGE('',*,*,#42413,.F.) ;
#55442=ORIENTED_EDGE('',*,*,#42399,.T.) ;
#55443=ORIENTED_EDGE('',*,*,#42413,.T.) ;
#55444=ORIENTED_EDGE('',*,*,#42414,.T.) ;
#55445=ORIENTED_EDGE('',*,*,#42415,.F.) ;
#55446=ORIENTED_EDGE('',*,*,#42400,.T.) ;
#55447=ORIENTED_EDGE('',*,*,#42415,.T.) ;
#55448=ORIENTED_EDGE('',*,*,#42416,.T.) ;
#55449=ORIENTED_EDGE('',*,*,#42417,.F.) ;
#55450=ORIENTED_EDGE('',*,*,#42401,.T.) ;
#55451=ORIENTED_EDGE('',*,*,#42417,.T.) ;
#55452=ORIENTED_EDGE('',*,*,#42418,.T.) ;
#55453=ORIENTED_EDGE('',*,*,#42419,.F.) ;
#55454=ORIENTED_EDGE('',*,*,#42402,.T.) ;
#55455=ORIENTED_EDGE('',*,*,#42419,.T.) ;
#55456=ORIENTED_EDGE('',*,*,#42420,.T.) ;
#55457=ORIENTED_EDGE('',*,*,#42405,.F.) ;
#55458=ORIENTED_EDGE('',*,*,#42403,.T.) ;
#55459=ORIENTED_EDGE('',*,*,#42421,.T.) ;
#55460=ORIENTED_EDGE('',*,*,#42422,.T.) ;
#55461=ORIENTED_EDGE('',*,*,#42423,.T.) ;
#55462=ORIENTED_EDGE('',*,*,#42424,.T.) ;
#55463=ORIENTED_EDGE('',*,*,#42425,.T.) ;
#55464=ORIENTED_EDGE('',*,*,#42426,.T.) ;
#55465=ORIENTED_EDGE('',*,*,#42427,.T.) ;
#55466=ORIENTED_EDGE('',*,*,#42428,.T.) ;
#55467=ORIENTED_EDGE('',*,*,#42429,.T.) ;
#55468=ORIENTED_EDGE('',*,*,#41615,.T.) ;
#55469=ORIENTED_EDGE('',*,*,#42430,.T.) ;
#55470=ORIENTED_EDGE('',*,*,#42431,.T.) ;
#55471=ORIENTED_EDGE('',*,*,#41617,.T.) ;
#55472=ORIENTED_EDGE('',*,*,#42432,.T.) ;
#55473=ORIENTED_EDGE('',*,*,#42433,.T.) ;
#55474=ORIENTED_EDGE('',*,*,#42434,.T.) ;
#55475=ORIENTED_EDGE('',*,*,#42435,.T.) ;
#55476=ORIENTED_EDGE('',*,*,#42436,.T.) ;
#55477=ORIENTED_EDGE('',*,*,#42437,.T.) ;
#55478=ORIENTED_EDGE('',*,*,#42438,.T.) ;
#55479=ORIENTED_EDGE('',*,*,#42439,.T.) ;
#55480=ORIENTED_EDGE('',*,*,#41593,.T.) ;
#55481=ORIENTED_EDGE('',*,*,#41621,.T.) ;
#55482=ORIENTED_EDGE('',*,*,#42440,.T.) ;
#55483=ORIENTED_EDGE('',*,*,#42441,.T.) ;
#55484=ORIENTED_EDGE('',*,*,#42442,.T.) ;
#55485=ORIENTED_EDGE('',*,*,#42443,.T.) ;
#55486=ORIENTED_EDGE('',*,*,#42444,.T.) ;
#55487=ORIENTED_EDGE('',*,*,#42445,.T.) ;
#55488=ORIENTED_EDGE('',*,*,#42446,.F.) ;
#55489=ORIENTED_EDGE('',*,*,#42447,.F.) ;
#55490=ORIENTED_EDGE('',*,*,#42448,.F.) ;
#55491=ORIENTED_EDGE('',*,*,#41824,.F.) ;
#55492=ORIENTED_EDGE('',*,*,#42298,.F.) ;
#55493=ORIENTED_EDGE('',*,*,#42287,.F.) ;
#55494=ORIENTED_EDGE('',*,*,#42449,.F.) ;
#55495=ORIENTED_EDGE('',*,*,#42308,.F.) ;
#55496=ORIENTED_EDGE('',*,*,#42449,.T.) ;
#55497=ORIENTED_EDGE('',*,*,#42286,.T.) ;
#55498=ORIENTED_EDGE('',*,*,#42450,.F.) ;
#55499=ORIENTED_EDGE('',*,*,#42451,.F.) ;
#55500=ORIENTED_EDGE('',*,*,#42450,.T.) ;
#55501=ORIENTED_EDGE('',*,*,#42293,.F.) ;
#55502=ORIENTED_EDGE('',*,*,#42452,.F.) ;
#55503=ORIENTED_EDGE('',*,*,#42324,.F.) ;
#55504=ORIENTED_EDGE('',*,*,#42447,.T.) ;
#55505=ORIENTED_EDGE('',*,*,#42325,.F.) ;
#55506=ORIENTED_EDGE('',*,*,#42453,.F.) ;
#55507=ORIENTED_EDGE('',*,*,#42284,.F.) ;
#55508=ORIENTED_EDGE('',*,*,#42448,.T.) ;
#55509=ORIENTED_EDGE('',*,*,#42283,.F.) ;
#55510=ORIENTED_EDGE('',*,*,#42454,.F.) ;
#55511=ORIENTED_EDGE('',*,*,#41825,.F.) ;
#55512=ORIENTED_EDGE('',*,*,#42446,.T.) ;
#55513=ORIENTED_EDGE('',*,*,#41823,.F.) ;
#55514=ORIENTED_EDGE('',*,*,#42455,.F.) ;
#55515=ORIENTED_EDGE('',*,*,#42320,.F.) ;
#55516=ORIENTED_EDGE('',*,*,#42451,.T.) ;
#55517=ORIENTED_EDGE('',*,*,#42323,.F.) ;
#55518=ORIENTED_EDGE('',*,*,#42456,.F.) ;
#55519=ORIENTED_EDGE('',*,*,#42309,.F.) ;
#55520=ORIENTED_EDGE('',*,*,#42300,.F.) ;
#55521=ORIENTED_EDGE('',*,*,#42310,.F.) ;
#55522=ORIENTED_EDGE('',*,*,#42457,.F.) ;
#55523=ORIENTED_EDGE('',*,*,#42303,.F.) ;
#55524=ORIENTED_EDGE('',*,*,#42453,.T.) ;
#55525=ORIENTED_EDGE('',*,*,#42452,.T.) ;
#55526=ORIENTED_EDGE('',*,*,#42458,.F.) ;
#55527=ORIENTED_EDGE('',*,*,#41826,.T.) ;
#55528=ORIENTED_EDGE('',*,*,#42454,.T.) ;
#55529=ORIENTED_EDGE('',*,*,#42459,.F.) ;
#55530=ORIENTED_EDGE('',*,*,#42460,.F.) ;
#55531=ORIENTED_EDGE('',*,*,#42455,.T.) ;
#55532=ORIENTED_EDGE('',*,*,#41830,.F.) ;
#55533=ORIENTED_EDGE('',*,*,#42461,.F.) ;
#55534=ORIENTED_EDGE('',*,*,#42462,.F.) ;
#55535=ORIENTED_EDGE('',*,*,#42457,.T.) ;
#55536=ORIENTED_EDGE('',*,*,#42456,.T.) ;
#55537=ORIENTED_EDGE('',*,*,#42463,.F.) ;
#55538=ORIENTED_EDGE('',*,*,#42304,.T.) ;
#55539=ORIENTED_EDGE('',*,*,#42458,.T.) ;
#55540=ORIENTED_EDGE('',*,*,#42292,.F.) ;
#55541=ORIENTED_EDGE('',*,*,#42464,.F.) ;
#55542=ORIENTED_EDGE('',*,*,#42285,.F.) ;
#55543=ORIENTED_EDGE('',*,*,#42459,.T.) ;
#55544=ORIENTED_EDGE('',*,*,#42282,.F.) ;
#55545=ORIENTED_EDGE('',*,*,#42465,.F.) ;
#55546=ORIENTED_EDGE('',*,*,#42318,.F.) ;
#55547=ORIENTED_EDGE('',*,*,#42460,.T.) ;
#55548=ORIENTED_EDGE('',*,*,#42317,.F.) ;
#55549=ORIENTED_EDGE('',*,*,#42466,.F.) ;
#55550=ORIENTED_EDGE('',*,*,#41827,.F.) ;
#55551=ORIENTED_EDGE('',*,*,#42461,.T.) ;
#55552=ORIENTED_EDGE('',*,*,#41829,.F.) ;
#55553=ORIENTED_EDGE('',*,*,#42467,.F.) ;
#55554=ORIENTED_EDGE('',*,*,#42279,.F.) ;
#55555=ORIENTED_EDGE('',*,*,#42462,.T.) ;
#55556=ORIENTED_EDGE('',*,*,#42278,.F.) ;
#55557=ORIENTED_EDGE('',*,*,#42468,.F.) ;
#55558=ORIENTED_EDGE('',*,*,#42321,.F.) ;
#55559=ORIENTED_EDGE('',*,*,#42463,.T.) ;
#55560=ORIENTED_EDGE('',*,*,#42322,.F.) ;
#55561=ORIENTED_EDGE('',*,*,#42469,.F.) ;
#55562=ORIENTED_EDGE('',*,*,#42305,.F.) ;
#55563=ORIENTED_EDGE('',*,*,#42465,.T.) ;
#55564=ORIENTED_EDGE('',*,*,#42464,.T.) ;
#55565=ORIENTED_EDGE('',*,*,#42470,.F.) ;
#55566=ORIENTED_EDGE('',*,*,#41828,.T.) ;
#55567=ORIENTED_EDGE('',*,*,#42466,.T.) ;
#55568=ORIENTED_EDGE('',*,*,#42471,.F.) ;
#55569=ORIENTED_EDGE('',*,*,#42467,.T.) ;
#55570=ORIENTED_EDGE('',*,*,#42469,.T.) ;
#55571=ORIENTED_EDGE('',*,*,#42468,.T.) ;
#55572=ORIENTED_EDGE('',*,*,#42472,.F.) ;
#55573=ORIENTED_EDGE('',*,*,#42297,.F.) ;
#55574=ORIENTED_EDGE('',*,*,#42313,.F.) ;
#55575=ORIENTED_EDGE('',*,*,#42473,.F.) ;
#55576=ORIENTED_EDGE('',*,*,#42289,.F.) ;
#55577=ORIENTED_EDGE('',*,*,#42470,.T.) ;
#55578=ORIENTED_EDGE('',*,*,#42291,.F.) ;
#55579=ORIENTED_EDGE('',*,*,#42474,.F.) ;
#55580=ORIENTED_EDGE('',*,*,#42319,.F.) ;
#55581=ORIENTED_EDGE('',*,*,#42471,.T.) ;
#55582=ORIENTED_EDGE('',*,*,#42316,.F.) ;
#55583=ORIENTED_EDGE('',*,*,#42475,.F.) ;
#55584=ORIENTED_EDGE('',*,*,#42280,.F.) ;
#55585=ORIENTED_EDGE('',*,*,#42472,.T.) ;
#55586=ORIENTED_EDGE('',*,*,#42281,.F.) ;
#55587=ORIENTED_EDGE('',*,*,#42476,.F.) ;
#55588=ORIENTED_EDGE('',*,*,#42306,.F.) ;
#55589=ORIENTED_EDGE('',*,*,#42290,.T.) ;
#55590=ORIENTED_EDGE('',*,*,#42473,.T.) ;
#55591=ORIENTED_EDGE('',*,*,#42477,.F.) ;
#55592=ORIENTED_EDGE('',*,*,#42474,.T.) ;
#55593=ORIENTED_EDGE('',*,*,#42476,.T.) ;
#55594=ORIENTED_EDGE('',*,*,#42475,.T.) ;
#55595=ORIENTED_EDGE('',*,*,#42478,.F.) ;
#55596=ORIENTED_EDGE('',*,*,#42477,.T.) ;
#55597=ORIENTED_EDGE('',*,*,#42312,.F.) ;
#55598=ORIENTED_EDGE('',*,*,#42479,.F.) ;
#55599=ORIENTED_EDGE('',*,*,#42314,.F.) ;
#55600=ORIENTED_EDGE('',*,*,#42478,.T.) ;
#55601=ORIENTED_EDGE('',*,*,#42315,.F.) ;
#55602=ORIENTED_EDGE('',*,*,#42480,.F.) ;
#55603=ORIENTED_EDGE('',*,*,#42307,.F.) ;
#55604=ORIENTED_EDGE('',*,*,#42480,.T.) ;
#55605=ORIENTED_EDGE('',*,*,#42479,.T.) ;
#55606=ORIENTED_EDGE('',*,*,#42481,.F.) ;
#55607=ORIENTED_EDGE('',*,*,#42301,.T.) ;
#55608=ORIENTED_EDGE('',*,*,#42295,.F.) ;
#55609=ORIENTED_EDGE('',*,*,#42302,.F.) ;
#55610=ORIENTED_EDGE('',*,*,#42481,.T.) ;
#55611=ORIENTED_EDGE('',*,*,#42311,.F.) ;
#55612=ORIENTED_EDGE('',*,*,#41619,.F.) ;
#55613=ORIENTED_EDGE('',*,*,#41757,.F.) ;
#55614=ORIENTED_EDGE('',*,*,#42275,.F.) ;
#55615=ORIENTED_EDGE('',*,*,#42267,.F.) ;
#55616=ORIENTED_EDGE('',*,*,#42266,.F.) ;
#55617=ORIENTED_EDGE('',*,*,#42482,.T.) ;
#55618=ORIENTED_EDGE('',*,*,#42483,.T.) ;
#55619=ORIENTED_EDGE('',*,*,#41595,.T.) ;
#55620=ORIENTED_EDGE('',*,*,#42425,.F.) ;
#55621=ORIENTED_EDGE('',*,*,#41620,.T.) ;
#55622=ORIENTED_EDGE('',*,*,#42427,.F.) ;
#55623=ORIENTED_EDGE('',*,*,#42484,.T.) ;
#55624=ORIENTED_EDGE('',*,*,#42431,.F.) ;
#55625=ORIENTED_EDGE('',*,*,#42485,.F.) ;
#55626=ORIENTED_EDGE('',*,*,#41618,.T.) ;
#55627=ORIENTED_EDGE('',*,*,#42428,.F.) ;
#55628=ORIENTED_EDGE('',*,*,#42486,.F.) ;
#55629=ORIENTED_EDGE('',*,*,#41758,.F.) ;
#55630=ORIENTED_EDGE('',*,*,#41777,.F.) ;
#55631=ORIENTED_EDGE('',*,*,#42487,.T.) ;
#55632=ORIENTED_EDGE('',*,*,#42435,.F.) ;
#55633=ORIENTED_EDGE('',*,*,#42488,.T.) ;
#55634=ORIENTED_EDGE('',*,*,#42438,.F.) ;
#55635=ORIENTED_EDGE('',*,*,#42489,.T.) ;
#55636=ORIENTED_EDGE('',*,*,#42429,.F.) ;
#55637=ORIENTED_EDGE('',*,*,#42490,.T.) ;
#55638=ORIENTED_EDGE('',*,*,#42486,.T.) ;
#55639=ORIENTED_EDGE('',*,*,#42485,.T.) ;
#55640=ORIENTED_EDGE('',*,*,#42491,.F.) ;
#55641=ORIENTED_EDGE('',*,*,#41759,.T.) ;
#55642=ORIENTED_EDGE('',*,*,#42492,.T.) ;
#55643=ORIENTED_EDGE('',*,*,#42493,.T.) ;
#55644=ORIENTED_EDGE('',*,*,#41740,.F.) ;
#55645=ORIENTED_EDGE('',*,*,#41612,.F.) ;
#55646=ORIENTED_EDGE('',*,*,#42433,.F.) ;
#55647=ORIENTED_EDGE('',*,*,#42494,.T.) ;
#55648=ORIENTED_EDGE('',*,*,#42491,.T.) ;
#55649=ORIENTED_EDGE('',*,*,#42430,.F.) ;
#55650=ORIENTED_EDGE('',*,*,#41611,.F.) ;
#55651=ORIENTED_EDGE('',*,*,#41760,.F.) ;
#55652=ORIENTED_EDGE('',*,*,#41614,.T.) ;
#55653=ORIENTED_EDGE('',*,*,#41761,.F.) ;
#55654=ORIENTED_EDGE('',*,*,#41609,.T.) ;
#55655=ORIENTED_EDGE('',*,*,#42434,.F.) ;
#55656=ORIENTED_EDGE('',*,*,#42495,.F.) ;
#55657=ORIENTED_EDGE('',*,*,#42410,.F.) ;
#55658=ORIENTED_EDGE('',*,*,#42496,.F.) ;
#55659=ORIENTED_EDGE('',*,*,#42496,.T.) ;
#55660=ORIENTED_EDGE('',*,*,#42408,.F.) ;
#55661=ORIENTED_EDGE('',*,*,#42497,.F.) ;
#55662=ORIENTED_EDGE('',*,*,#42421,.F.) ;
#55663=ORIENTED_EDGE('',*,*,#42495,.T.) ;
#55664=ORIENTED_EDGE('',*,*,#42424,.F.) ;
#55665=ORIENTED_EDGE('',*,*,#42498,.F.) ;
#55666=ORIENTED_EDGE('',*,*,#42412,.F.) ;
#55667=ORIENTED_EDGE('',*,*,#42497,.T.) ;
#55668=ORIENTED_EDGE('',*,*,#42406,.F.) ;
#55669=ORIENTED_EDGE('',*,*,#42499,.F.) ;
#55670=ORIENTED_EDGE('',*,*,#42414,.F.) ;
#55671=ORIENTED_EDGE('',*,*,#42498,.T.) ;
#55672=ORIENTED_EDGE('',*,*,#42500,.F.) ;
#55673=ORIENTED_EDGE('',*,*,#42499,.T.) ;
#55674=ORIENTED_EDGE('',*,*,#42420,.F.) ;
#55675=ORIENTED_EDGE('',*,*,#42501,.F.) ;
#55676=ORIENTED_EDGE('',*,*,#42422,.F.) ;
#55677=ORIENTED_EDGE('',*,*,#42500,.T.) ;
#55678=ORIENTED_EDGE('',*,*,#42423,.F.) ;
#55679=ORIENTED_EDGE('',*,*,#42502,.F.) ;
#55680=ORIENTED_EDGE('',*,*,#42416,.F.) ;
#55681=ORIENTED_EDGE('',*,*,#42501,.T.) ;
#55682=ORIENTED_EDGE('',*,*,#42418,.F.) ;
#55683=ORIENTED_EDGE('',*,*,#42502,.T.) ;
#55684=ORIENTED_EDGE('',*,*,#42503,.F.) ;
#55685=ORIENTED_EDGE('',*,*,#41848,.F.) ;
#55686=ORIENTED_EDGE('',*,*,#42504,.F.) ;
#55687=ORIENTED_EDGE('',*,*,#42329,.F.) ;
#55688=ORIENTED_EDGE('',*,*,#42504,.T.) ;
#55689=ORIENTED_EDGE('',*,*,#41847,.T.) ;
#55690=ORIENTED_EDGE('',*,*,#42505,.F.) ;
#55691=ORIENTED_EDGE('',*,*,#42506,.F.) ;
#55692=ORIENTED_EDGE('',*,*,#41849,.T.) ;
#55693=ORIENTED_EDGE('',*,*,#42503,.T.) ;
#55694=ORIENTED_EDGE('',*,*,#42507,.F.) ;
#55695=ORIENTED_EDGE('',*,*,#42508,.F.) ;
#55696=ORIENTED_EDGE('',*,*,#42505,.T.) ;
#55697=ORIENTED_EDGE('',*,*,#41846,.F.) ;
#55698=ORIENTED_EDGE('',*,*,#42509,.F.) ;
#55699=ORIENTED_EDGE('',*,*,#42341,.F.) ;
#55700=ORIENTED_EDGE('',*,*,#42506,.T.) ;
#55701=ORIENTED_EDGE('',*,*,#42340,.F.) ;
#55702=ORIENTED_EDGE('',*,*,#42510,.F.) ;
#55703=ORIENTED_EDGE('',*,*,#42326,.F.) ;
#55704=ORIENTED_EDGE('',*,*,#42511,.F.) ;
#55705=ORIENTED_EDGE('',*,*,#42327,.F.) ;
#55706=ORIENTED_EDGE('',*,*,#42512,.F.) ;
#55707=ORIENTED_EDGE('',*,*,#42345,.F.) ;
#55708=ORIENTED_EDGE('',*,*,#42507,.T.) ;
#55709=ORIENTED_EDGE('',*,*,#42328,.F.) ;
#55710=ORIENTED_EDGE('',*,*,#42513,.F.) ;
#55711=ORIENTED_EDGE('',*,*,#42333,.F.) ;
#55712=ORIENTED_EDGE('',*,*,#42508,.T.) ;
#55713=ORIENTED_EDGE('',*,*,#42332,.F.) ;
#55714=ORIENTED_EDGE('',*,*,#42514,.F.) ;
#55715=ORIENTED_EDGE('',*,*,#41850,.F.) ;
#55716=ORIENTED_EDGE('',*,*,#42515,.F.) ;
#55717=ORIENTED_EDGE('',*,*,#41844,.F.) ;
#55718=ORIENTED_EDGE('',*,*,#42516,.F.) ;
#55719=ORIENTED_EDGE('',*,*,#42336,.F.) ;
#55720=ORIENTED_EDGE('',*,*,#41845,.T.) ;
#55721=ORIENTED_EDGE('',*,*,#42515,.T.) ;
#55722=ORIENTED_EDGE('',*,*,#42517,.F.) ;
#55723=ORIENTED_EDGE('',*,*,#42509,.T.) ;
#55724=ORIENTED_EDGE('',*,*,#42512,.T.) ;
#55725=ORIENTED_EDGE('',*,*,#42510,.T.) ;
#55726=ORIENTED_EDGE('',*,*,#42518,.F.) ;
#55727=ORIENTED_EDGE('',*,*,#42513,.T.) ;
#55728=ORIENTED_EDGE('',*,*,#42511,.T.) ;
#55729=ORIENTED_EDGE('',*,*,#42519,.F.) ;
#55730=ORIENTED_EDGE('',*,*,#41843,.T.) ;
#55731=ORIENTED_EDGE('',*,*,#42514,.T.) ;
#55732=ORIENTED_EDGE('',*,*,#42520,.F.) ;
#55733=ORIENTED_EDGE('',*,*,#42516,.T.) ;
#55734=ORIENTED_EDGE('',*,*,#42517,.T.) ;
#55735=ORIENTED_EDGE('',*,*,#42335,.F.) ;
#55736=ORIENTED_EDGE('',*,*,#42521,.F.) ;
#55737=ORIENTED_EDGE('',*,*,#42338,.F.) ;
#55738=ORIENTED_EDGE('',*,*,#42518,.T.) ;
#55739=ORIENTED_EDGE('',*,*,#42339,.F.) ;
#55740=ORIENTED_EDGE('',*,*,#42522,.F.) ;
#55741=ORIENTED_EDGE('',*,*,#42342,.F.) ;
#55742=ORIENTED_EDGE('',*,*,#42519,.T.) ;
#55743=ORIENTED_EDGE('',*,*,#42344,.F.) ;
#55744=ORIENTED_EDGE('',*,*,#42523,.F.) ;
#55745=ORIENTED_EDGE('',*,*,#42330,.F.) ;
#55746=ORIENTED_EDGE('',*,*,#42520,.T.) ;
#55747=ORIENTED_EDGE('',*,*,#42331,.F.) ;
#55748=ORIENTED_EDGE('',*,*,#42524,.F.) ;
#55749=ORIENTED_EDGE('',*,*,#42337,.F.) ;
#55750=ORIENTED_EDGE('',*,*,#42522,.T.) ;
#55751=ORIENTED_EDGE('',*,*,#42521,.T.) ;
#55752=ORIENTED_EDGE('',*,*,#42525,.F.) ;
#55753=ORIENTED_EDGE('',*,*,#42524,.T.) ;
#55754=ORIENTED_EDGE('',*,*,#42523,.T.) ;
#55755=ORIENTED_EDGE('',*,*,#42526,.F.) ;
#55756=ORIENTED_EDGE('',*,*,#42525,.T.) ;
#55757=ORIENTED_EDGE('',*,*,#42334,.F.) ;
#55758=ORIENTED_EDGE('',*,*,#42526,.T.) ;
#55759=ORIENTED_EDGE('',*,*,#42343,.F.) ;
#55760=ORIENTED_EDGE('',*,*,#42527,.F.) ;
#55761=ORIENTED_EDGE('',*,*,#41798,.F.) ;
#55762=ORIENTED_EDGE('',*,*,#42528,.F.) ;
#55763=ORIENTED_EDGE('',*,*,#42388,.F.) ;
#55764=ORIENTED_EDGE('',*,*,#42528,.T.) ;
#55765=ORIENTED_EDGE('',*,*,#41797,.T.) ;
#55766=ORIENTED_EDGE('',*,*,#42529,.F.) ;
#55767=ORIENTED_EDGE('',*,*,#42530,.F.) ;
#55768=ORIENTED_EDGE('',*,*,#41799,.T.) ;
#55769=ORIENTED_EDGE('',*,*,#42527,.T.) ;
#55770=ORIENTED_EDGE('',*,*,#42531,.F.) ;
#55771=ORIENTED_EDGE('',*,*,#42532,.F.) ;
#55772=ORIENTED_EDGE('',*,*,#42529,.T.) ;
#55773=ORIENTED_EDGE('',*,*,#41796,.F.) ;
#55774=ORIENTED_EDGE('',*,*,#42533,.F.) ;
#55775=ORIENTED_EDGE('',*,*,#42384,.F.) ;
#55776=ORIENTED_EDGE('',*,*,#42530,.T.) ;
#55777=ORIENTED_EDGE('',*,*,#42383,.F.) ;
#55778=ORIENTED_EDGE('',*,*,#42534,.F.) ;
#55779=ORIENTED_EDGE('',*,*,#42385,.F.) ;
#55780=ORIENTED_EDGE('',*,*,#42535,.F.) ;
#55781=ORIENTED_EDGE('',*,*,#42386,.F.) ;
#55782=ORIENTED_EDGE('',*,*,#42536,.F.) ;
#55783=ORIENTED_EDGE('',*,*,#42396,.F.) ;
#55784=ORIENTED_EDGE('',*,*,#42531,.T.) ;
#55785=ORIENTED_EDGE('',*,*,#42387,.F.) ;
#55786=ORIENTED_EDGE('',*,*,#42537,.F.) ;
#55787=ORIENTED_EDGE('',*,*,#42392,.F.) ;
#55788=ORIENTED_EDGE('',*,*,#42532,.T.) ;
#55789=ORIENTED_EDGE('',*,*,#42391,.F.) ;
#55790=ORIENTED_EDGE('',*,*,#42538,.F.) ;
#55791=ORIENTED_EDGE('',*,*,#41800,.F.) ;
#55792=ORIENTED_EDGE('',*,*,#42539,.F.) ;
#55793=ORIENTED_EDGE('',*,*,#41794,.F.) ;
#55794=ORIENTED_EDGE('',*,*,#42540,.F.) ;
#55795=ORIENTED_EDGE('',*,*,#42379,.F.) ;
#55796=ORIENTED_EDGE('',*,*,#41795,.T.) ;
#55797=ORIENTED_EDGE('',*,*,#42539,.T.) ;
#55798=ORIENTED_EDGE('',*,*,#42541,.F.) ;
#55799=ORIENTED_EDGE('',*,*,#42533,.T.) ;
#55800=ORIENTED_EDGE('',*,*,#42536,.T.) ;
#55801=ORIENTED_EDGE('',*,*,#42534,.T.) ;
#55802=ORIENTED_EDGE('',*,*,#42542,.F.) ;
#55803=ORIENTED_EDGE('',*,*,#42537,.T.) ;
#55804=ORIENTED_EDGE('',*,*,#42535,.T.) ;
#55805=ORIENTED_EDGE('',*,*,#42543,.F.) ;
#55806=ORIENTED_EDGE('',*,*,#41793,.T.) ;
#55807=ORIENTED_EDGE('',*,*,#42538,.T.) ;
#55808=ORIENTED_EDGE('',*,*,#42544,.F.) ;
#55809=ORIENTED_EDGE('',*,*,#42540,.T.) ;
#55810=ORIENTED_EDGE('',*,*,#42541,.T.) ;
#55811=ORIENTED_EDGE('',*,*,#42378,.F.) ;
#55812=ORIENTED_EDGE('',*,*,#42545,.F.) ;
#55813=ORIENTED_EDGE('',*,*,#42381,.F.) ;
#55814=ORIENTED_EDGE('',*,*,#42542,.T.) ;
#55815=ORIENTED_EDGE('',*,*,#42382,.F.) ;
#55816=ORIENTED_EDGE('',*,*,#42546,.F.) ;
#55817=ORIENTED_EDGE('',*,*,#42393,.F.) ;
#55818=ORIENTED_EDGE('',*,*,#42543,.T.) ;
#55819=ORIENTED_EDGE('',*,*,#42395,.F.) ;
#55820=ORIENTED_EDGE('',*,*,#42547,.F.) ;
#55821=ORIENTED_EDGE('',*,*,#42389,.F.) ;
#55822=ORIENTED_EDGE('',*,*,#42544,.T.) ;
#55823=ORIENTED_EDGE('',*,*,#42390,.F.) ;
#55824=ORIENTED_EDGE('',*,*,#42548,.F.) ;
#55825=ORIENTED_EDGE('',*,*,#42380,.F.) ;
#55826=ORIENTED_EDGE('',*,*,#42546,.T.) ;
#55827=ORIENTED_EDGE('',*,*,#42545,.T.) ;
#55828=ORIENTED_EDGE('',*,*,#42549,.F.) ;
#55829=ORIENTED_EDGE('',*,*,#42548,.T.) ;
#55830=ORIENTED_EDGE('',*,*,#42547,.T.) ;
#55831=ORIENTED_EDGE('',*,*,#42550,.F.) ;
#55832=ORIENTED_EDGE('',*,*,#42549,.T.) ;
#55833=ORIENTED_EDGE('',*,*,#42377,.F.) ;
#55834=ORIENTED_EDGE('',*,*,#42550,.T.) ;
#55835=ORIENTED_EDGE('',*,*,#42394,.F.) ;
#55836=ORIENTED_EDGE('',*,*,#41733,.F.) ;
#55837=ORIENTED_EDGE('',*,*,#42551,.T.) ;
#55838=ORIENTED_EDGE('',*,*,#42440,.F.) ;
#55839=ORIENTED_EDGE('',*,*,#42552,.F.) ;
#55840=ORIENTED_EDGE('',*,*,#42184,.T.) ;
#55841=ORIENTED_EDGE('',*,*,#42552,.T.) ;
#55842=ORIENTED_EDGE('',*,*,#42553,.F.) ;
#55843=ORIENTED_EDGE('',*,*,#42553,.T.) ;
#55844=ORIENTED_EDGE('',*,*,#42445,.F.) ;
#55845=ORIENTED_EDGE('',*,*,#42554,.F.) ;
#55846=ORIENTED_EDGE('',*,*,#41883,.F.) ;
#55847=ORIENTED_EDGE('',*,*,#42180,.T.) ;
#55848=ORIENTED_EDGE('',*,*,#42554,.T.) ;
#55849=ORIENTED_EDGE('',*,*,#42555,.F.) ;
#55850=ORIENTED_EDGE('',*,*,#41752,.T.) ;
#55851=ORIENTED_EDGE('',*,*,#42555,.T.) ;
#55852=ORIENTED_EDGE('',*,*,#42444,.F.) ;
#55853=ORIENTED_EDGE('',*,*,#42556,.F.) ;
#55854=ORIENTED_EDGE('',*,*,#41753,.F.) ;
#55855=ORIENTED_EDGE('',*,*,#42276,.F.) ;
#55856=ORIENTED_EDGE('',*,*,#41755,.F.) ;
#55857=ORIENTED_EDGE('',*,*,#42557,.F.) ;
#55858=ORIENTED_EDGE('',*,*,#42272,.F.) ;
#55859=ORIENTED_EDGE('',*,*,#41754,.T.) ;
#55860=ORIENTED_EDGE('',*,*,#42556,.T.) ;
#55861=ORIENTED_EDGE('',*,*,#42558,.F.) ;
#55862=ORIENTED_EDGE('',*,*,#42557,.T.) ;
#55863=ORIENTED_EDGE('',*,*,#42558,.T.) ;
#55864=ORIENTED_EDGE('',*,*,#42443,.F.) ;
#55865=ORIENTED_EDGE('',*,*,#42559,.F.) ;
#55866=ORIENTED_EDGE('',*,*,#42269,.F.) ;
#55867=ORIENTED_EDGE('',*,*,#42277,.F.) ;
#55868=ORIENTED_EDGE('',*,*,#42270,.F.) ;
#55869=ORIENTED_EDGE('',*,*,#42560,.F.) ;
#55870=ORIENTED_EDGE('',*,*,#42263,.F.) ;
#55871=ORIENTED_EDGE('',*,*,#42560,.T.) ;
#55872=ORIENTED_EDGE('',*,*,#42559,.T.) ;
#55873=ORIENTED_EDGE('',*,*,#42561,.F.) ;
#55874=ORIENTED_EDGE('',*,*,#42442,.F.) ;
#55875=ORIENTED_EDGE('',*,*,#42562,.T.) ;
#55876=ORIENTED_EDGE('',*,*,#42260,.F.) ;
#55877=ORIENTED_EDGE('',*,*,#42561,.T.) ;
#55878=ORIENTED_EDGE('',*,*,#41627,.F.) ;
#55879=ORIENTED_EDGE('',*,*,#42373,.F.) ;
#55880=ORIENTED_EDGE('',*,*,#41637,.F.) ;
#55881=ORIENTED_EDGE('',*,*,#42375,.F.) ;
#55882=ORIENTED_EDGE('',*,*,#41635,.F.) ;
#55883=ORIENTED_EDGE('',*,*,#42371,.F.) ;
#55884=ORIENTED_EDGE('',*,*,#41629,.F.) ;
#55885=ORIENTED_EDGE('',*,*,#42376,.F.) ;
#55886=ORIENTED_EDGE('',*,*,#41625,.F.) ;
#55887=ORIENTED_EDGE('',*,*,#42268,.F.) ;
#55888=ORIENTED_EDGE('',*,*,#41639,.F.) ;
#55889=ORIENTED_EDGE('',*,*,#42374,.F.) ;
#55890=ORIENTED_EDGE('',*,*,#41633,.F.) ;
#55891=ORIENTED_EDGE('',*,*,#42370,.F.) ;
#55892=ORIENTED_EDGE('',*,*,#41631,.F.) ;
#55893=ORIENTED_EDGE('',*,*,#42372,.F.) ;
#55894=ORIENTED_EDGE('',*,*,#42563,.F.) ;
#55895=ORIENTED_EDGE('',*,*,#41616,.F.) ;
#55896=ORIENTED_EDGE('',*,*,#42489,.F.) ;
#55897=ORIENTED_EDGE('',*,*,#42563,.T.) ;
#55898=ORIENTED_EDGE('',*,*,#42437,.F.) ;
#55899=ORIENTED_EDGE('',*,*,#42564,.F.) ;
#55900=ORIENTED_EDGE('',*,*,#42432,.F.) ;
#55901=ORIENTED_EDGE('',*,*,#42564,.T.) ;
#55902=ORIENTED_EDGE('',*,*,#42436,.F.) ;
#55903=ORIENTED_EDGE('',*,*,#42565,.F.) ;
#55904=ORIENTED_EDGE('',*,*,#42494,.F.) ;
#55905=ORIENTED_EDGE('',*,*,#42565,.T.) ;
#55906=ORIENTED_EDGE('',*,*,#42487,.F.) ;
#55907=ORIENTED_EDGE('',*,*,#42566,.F.) ;
#55908=ORIENTED_EDGE('',*,*,#42492,.F.) ;
#55909=ORIENTED_EDGE('',*,*,#42566,.T.) ;
#55910=ORIENTED_EDGE('',*,*,#41776,.F.) ;
#55911=ORIENTED_EDGE('',*,*,#42202,.F.) ;
#55912=ORIENTED_EDGE('',*,*,#42493,.F.) ;
#55913=ORIENTED_EDGE('',*,*,#42274,.F.) ;
#55914=ORIENTED_EDGE('',*,*,#41779,.F.) ;
#55915=ORIENTED_EDGE('',*,*,#42567,.F.) ;
#55916=ORIENTED_EDGE('',*,*,#42265,.F.) ;
#55917=ORIENTED_EDGE('',*,*,#42567,.T.) ;
#55918=ORIENTED_EDGE('',*,*,#41778,.F.) ;
#55919=ORIENTED_EDGE('',*,*,#42568,.F.) ;
#55920=ORIENTED_EDGE('',*,*,#42482,.F.) ;
#55921=ORIENTED_EDGE('',*,*,#42568,.T.) ;
#55922=ORIENTED_EDGE('',*,*,#42488,.F.) ;
#55923=ORIENTED_EDGE('',*,*,#41596,.F.) ;
#55924=ORIENTED_EDGE('',*,*,#42483,.F.) ;
#55925=ORIENTED_EDGE('',*,*,#42569,.F.) ;
#55926=ORIENTED_EDGE('',*,*,#42426,.F.) ;
#55927=ORIENTED_EDGE('',*,*,#41594,.T.) ;
#55928=ORIENTED_EDGE('',*,*,#42439,.F.) ;
#55929=ORIENTED_EDGE('',*,*,#42490,.F.) ;
#55930=ORIENTED_EDGE('',*,*,#42484,.F.) ;
#55931=ORIENTED_EDGE('',*,*,#42569,.T.) ;
#55932=ORIENTED_EDGE('',*,*,#42570,.T.) ;
#55933=ORIENTED_EDGE('',*,*,#42571,.T.) ;
#55934=ORIENTED_EDGE('',*,*,#42441,.F.) ;
#55935=ORIENTED_EDGE('',*,*,#42572,.T.) ;
#55936=ORIENTED_EDGE('',*,*,#42573,.T.) ;
#55937=ORIENTED_EDGE('',*,*,#41875,.F.) ;
#55938=ORIENTED_EDGE('',*,*,#42574,.T.) ;
#55939=ORIENTED_EDGE('',*,*,#42551,.F.) ;
#55940=ORIENTED_EDGE('',*,*,#42212,.T.) ;
#55941=ORIENTED_EDGE('',*,*,#42273,.F.) ;
#55942=ORIENTED_EDGE('',*,*,#42261,.F.) ;
#55943=ORIENTED_EDGE('',*,*,#42575,.F.) ;
#55944=ORIENTED_EDGE('',*,*,#41871,.F.) ;
#55945=ORIENTED_EDGE('',*,*,#42562,.F.) ;
#55946=ORIENTED_EDGE('',*,*,#42576,.T.) ;
#55947=ORIENTED_EDGE('',*,*,#41872,.F.) ;
#55948=ORIENTED_EDGE('',*,*,#42575,.T.) ;
#55949=ORIENTED_EDGE('',*,*,#42572,.F.) ;
#55950=ORIENTED_EDGE('',*,*,#42574,.F.) ;
#55951=ORIENTED_EDGE('',*,*,#42577,.F.) ;
#55952=ORIENTED_EDGE('',*,*,#42578,.F.) ;
#55953=ORIENTED_EDGE('',*,*,#42573,.F.) ;
#55954=ORIENTED_EDGE('',*,*,#42577,.T.) ;
#55955=ORIENTED_EDGE('',*,*,#41874,.F.) ;
#55956=ORIENTED_EDGE('',*,*,#42578,.T.) ;
#55957=ORIENTED_EDGE('',*,*,#41873,.F.) ;
#55958=ORIENTED_EDGE('',*,*,#42579,.F.) ;
#55959=ORIENTED_EDGE('',*,*,#42570,.F.) ;
#55960=ORIENTED_EDGE('',*,*,#42579,.T.) ;
#55961=ORIENTED_EDGE('',*,*,#42576,.F.) ;
#55962=ORIENTED_EDGE('',*,*,#42571,.F.) ;
#55963=ORIENTED_EDGE('',*,*,#42580,.F.) ;
#55964=ORIENTED_EDGE('',*,*,#42230,.F.) ;
#55965=ORIENTED_EDGE('',*,*,#42581,.F.) ;
#55966=ORIENTED_EDGE('',*,*,#42582,.F.) ;
#55967=ORIENTED_EDGE('',*,*,#42228,.F.) ;
#55968=ORIENTED_EDGE('',*,*,#42583,.F.) ;
#55969=ORIENTED_EDGE('',*,*,#42581,.T.) ;
#55970=ORIENTED_EDGE('',*,*,#42233,.F.) ;
#55971=ORIENTED_EDGE('',*,*,#42584,.F.) ;
#55972=ORIENTED_EDGE('',*,*,#42251,.F.) ;
#55973=ORIENTED_EDGE('',*,*,#42580,.T.) ;
#55974=ORIENTED_EDGE('',*,*,#42250,.F.) ;
#55975=ORIENTED_EDGE('',*,*,#42585,.F.) ;
#55976=ORIENTED_EDGE('',*,*,#42227,.F.) ;
#55977=ORIENTED_EDGE('',*,*,#42583,.T.) ;
#55978=ORIENTED_EDGE('',*,*,#42225,.F.) ;
#55979=ORIENTED_EDGE('',*,*,#42586,.F.) ;
#55980=ORIENTED_EDGE('',*,*,#42253,.F.) ;
#55981=ORIENTED_EDGE('',*,*,#42582,.T.) ;
#55982=ORIENTED_EDGE('',*,*,#42259,.F.) ;
#55983=ORIENTED_EDGE('',*,*,#42587,.F.) ;
#55984=ORIENTED_EDGE('',*,*,#42231,.F.) ;
#55985=ORIENTED_EDGE('',*,*,#42584,.T.) ;
#55986=ORIENTED_EDGE('',*,*,#42236,.F.) ;
#55987=ORIENTED_EDGE('',*,*,#42588,.F.) ;
#55988=ORIENTED_EDGE('',*,*,#42224,.F.) ;
#55989=ORIENTED_EDGE('',*,*,#42585,.T.) ;
#55990=ORIENTED_EDGE('',*,*,#42589,.F.) ;
#55991=ORIENTED_EDGE('',*,*,#42586,.T.) ;
#55992=ORIENTED_EDGE('',*,*,#42222,.F.) ;
#55993=ORIENTED_EDGE('',*,*,#42590,.F.) ;
#55994=ORIENTED_EDGE('',*,*,#42234,.F.) ;
#55995=ORIENTED_EDGE('',*,*,#42587,.T.) ;
#55996=ORIENTED_EDGE('',*,*,#42591,.F.) ;
#55997=ORIENTED_EDGE('',*,*,#42588,.T.) ;
#55998=ORIENTED_EDGE('',*,*,#42239,.F.) ;
#55999=ORIENTED_EDGE('',*,*,#42592,.F.) ;
#56000=ORIENTED_EDGE('',*,*,#42252,.F.) ;
#56001=ORIENTED_EDGE('',*,*,#42589,.T.) ;
#56002=ORIENTED_EDGE('',*,*,#42249,.F.) ;
#56003=ORIENTED_EDGE('',*,*,#42593,.F.) ;
#56004=ORIENTED_EDGE('',*,*,#42221,.F.) ;
#56005=ORIENTED_EDGE('',*,*,#42594,.F.) ;
#56006=ORIENTED_EDGE('',*,*,#42218,.F.) ;
#56007=ORIENTED_EDGE('',*,*,#42595,.F.) ;
#56008=ORIENTED_EDGE('',*,*,#41702,.F.) ;
#56009=ORIENTED_EDGE('',*,*,#42590,.T.) ;
#56010=ORIENTED_EDGE('',*,*,#42219,.F.) ;
#56011=ORIENTED_EDGE('',*,*,#42596,.F.) ;
#56012=ORIENTED_EDGE('',*,*,#42254,.F.) ;
#56013=ORIENTED_EDGE('',*,*,#42591,.T.) ;
#56014=ORIENTED_EDGE('',*,*,#42258,.F.) ;
#56015=ORIENTED_EDGE('',*,*,#42597,.F.) ;
#56016=ORIENTED_EDGE('',*,*,#42237,.F.) ;
#56017=ORIENTED_EDGE('',*,*,#42592,.T.) ;
#56018=ORIENTED_EDGE('',*,*,#42242,.F.) ;
#56019=ORIENTED_EDGE('',*,*,#42598,.F.) ;
#56020=ORIENTED_EDGE('',*,*,#42246,.F.) ;
#56021=ORIENTED_EDGE('',*,*,#42595,.T.) ;
#56022=ORIENTED_EDGE('',*,*,#42593,.T.) ;
#56023=ORIENTED_EDGE('',*,*,#42599,.F.) ;
#56024=ORIENTED_EDGE('',*,*,#41703,.T.) ;
#56025=ORIENTED_EDGE('',*,*,#42594,.T.) ;
#56026=ORIENTED_EDGE('',*,*,#41701,.T.) ;
#56027=ORIENTED_EDGE('',*,*,#42600,.F.) ;
#56028=ORIENTED_EDGE('',*,*,#42596,.T.) ;
#56029=ORIENTED_EDGE('',*,*,#42597,.T.) ;
#56030=ORIENTED_EDGE('',*,*,#42257,.F.) ;
#56031=ORIENTED_EDGE('',*,*,#42601,.F.) ;
#56032=ORIENTED_EDGE('',*,*,#42240,.F.) ;
#56033=ORIENTED_EDGE('',*,*,#42598,.T.) ;
#56034=ORIENTED_EDGE('',*,*,#42245,.F.) ;
#56035=ORIENTED_EDGE('',*,*,#42602,.F.) ;
#56036=ORIENTED_EDGE('',*,*,#42247,.F.) ;
#56037=ORIENTED_EDGE('',*,*,#42599,.T.) ;
#56038=ORIENTED_EDGE('',*,*,#42248,.F.) ;
#56039=ORIENTED_EDGE('',*,*,#42603,.F.) ;
#56040=ORIENTED_EDGE('',*,*,#41704,.F.) ;
#56041=ORIENTED_EDGE('',*,*,#42600,.T.) ;
#56042=ORIENTED_EDGE('',*,*,#41700,.F.) ;
#56043=ORIENTED_EDGE('',*,*,#42604,.F.) ;
#56044=ORIENTED_EDGE('',*,*,#42255,.F.) ;
#56045=ORIENTED_EDGE('',*,*,#42601,.T.) ;
#56046=ORIENTED_EDGE('',*,*,#42256,.F.) ;
#56047=ORIENTED_EDGE('',*,*,#42605,.F.) ;
#56048=ORIENTED_EDGE('',*,*,#42243,.F.) ;
#56049=ORIENTED_EDGE('',*,*,#42603,.T.) ;
#56050=ORIENTED_EDGE('',*,*,#42602,.T.) ;
#56051=ORIENTED_EDGE('',*,*,#42606,.F.) ;
#56052=ORIENTED_EDGE('',*,*,#41705,.T.) ;
#56053=ORIENTED_EDGE('',*,*,#42604,.T.) ;
#56054=ORIENTED_EDGE('',*,*,#41699,.T.) ;
#56055=ORIENTED_EDGE('',*,*,#42607,.F.) ;
#56056=ORIENTED_EDGE('',*,*,#42605,.T.) ;
#56057=ORIENTED_EDGE('',*,*,#42606,.T.) ;
#56058=ORIENTED_EDGE('',*,*,#42244,.F.) ;
#56059=ORIENTED_EDGE('',*,*,#42607,.T.) ;
#56060=ORIENTED_EDGE('',*,*,#41706,.F.) ;
#56061=ORIENTED_EDGE('',*,*,#42608,.F.) ;
#56062=ORIENTED_EDGE('',*,*,#42609,.F.) ;
#56063=ORIENTED_EDGE('',*,*,#42610,.F.) ;
#56064=ORIENTED_EDGE('',*,*,#42611,.T.) ;
#56065=ORIENTED_EDGE('',*,*,#42612,.F.) ;
#56066=ORIENTED_EDGE('',*,*,#42613,.T.) ;
#56067=ORIENTED_EDGE('',*,*,#42614,.F.) ;
#56068=ORIENTED_EDGE('',*,*,#42615,.F.) ;
#56069=ORIENTED_EDGE('',*,*,#42613,.F.) ;
#56070=ORIENTED_EDGE('',*,*,#42616,.F.) ;
#56071=ORIENTED_EDGE('',*,*,#42617,.T.) ;
#56072=ORIENTED_EDGE('',*,*,#42618,.F.) ;
#56073=ORIENTED_EDGE('',*,*,#42617,.F.) ;
#56074=ORIENTED_EDGE('',*,*,#42619,.F.) ;
#56075=ORIENTED_EDGE('',*,*,#42620,.T.) ;
#56076=ORIENTED_EDGE('',*,*,#42621,.F.) ;
#56077=ORIENTED_EDGE('',*,*,#42622,.F.) ;
#56078=ORIENTED_EDGE('',*,*,#42620,.F.) ;
#56079=ORIENTED_EDGE('',*,*,#42623,.T.) ;
#56080=ORIENTED_EDGE('',*,*,#42624,.F.) ;
#56081=ORIENTED_EDGE('',*,*,#42625,.T.) ;
#56082=ORIENTED_EDGE('',*,*,#42626,.T.) ;
#56083=ORIENTED_EDGE('',*,*,#42627,.T.) ;
#56084=ORIENTED_EDGE('',*,*,#42628,.T.) ;
#56085=ORIENTED_EDGE('',*,*,#42629,.F.) ;
#56086=ORIENTED_EDGE('',*,*,#42623,.F.) ;
#56087=ORIENTED_EDGE('',*,*,#42630,.F.) ;
#56088=ORIENTED_EDGE('',*,*,#42631,.T.) ;
#56089=ORIENTED_EDGE('',*,*,#42632,.F.) ;
#56090=ORIENTED_EDGE('',*,*,#42633,.F.) ;
#56091=ORIENTED_EDGE('',*,*,#42634,.T.) ;
#56092=ORIENTED_EDGE('',*,*,#42635,.F.) ;
#56093=ORIENTED_EDGE('',*,*,#42636,.F.) ;
#56094=ORIENTED_EDGE('',*,*,#42637,.T.) ;
#56095=ORIENTED_EDGE('',*,*,#42616,.T.) ;
#56096=ORIENTED_EDGE('',*,*,#42637,.F.) ;
#56097=ORIENTED_EDGE('',*,*,#42618,.T.) ;
#56098=ORIENTED_EDGE('',*,*,#42638,.T.) ;
#56099=ORIENTED_EDGE('',*,*,#42621,.T.) ;
#56100=ORIENTED_EDGE('',*,*,#42622,.T.) ;
#56101=ORIENTED_EDGE('',*,*,#42638,.F.) ;
#56102=ORIENTED_EDGE('',*,*,#42639,.F.) ;
#56103=ORIENTED_EDGE('',*,*,#42640,.T.) ;
#56104=ORIENTED_EDGE('',*,*,#42641,.F.) ;
#56105=ORIENTED_EDGE('',*,*,#42642,.T.) ;
#56106=ORIENTED_EDGE('',*,*,#42643,.F.) ;
#56107=ORIENTED_EDGE('',*,*,#42644,.T.) ;
#56108=ORIENTED_EDGE('',*,*,#42645,.T.) ;
#56109=ORIENTED_EDGE('',*,*,#42646,.T.) ;
#56110=ORIENTED_EDGE('',*,*,#42647,.F.) ;
#56111=ORIENTED_EDGE('',*,*,#42648,.T.) ;
#56112=ORIENTED_EDGE('',*,*,#42649,.F.) ;
#56113=ORIENTED_EDGE('',*,*,#42650,.T.) ;
#56114=ORIENTED_EDGE('',*,*,#42651,.F.) ;
#56115=ORIENTED_EDGE('',*,*,#42652,.T.) ;
#56116=ORIENTED_EDGE('',*,*,#42653,.T.) ;
#56117=ORIENTED_EDGE('',*,*,#42654,.T.) ;
#56118=ORIENTED_EDGE('',*,*,#42655,.F.) ;
#56119=ORIENTED_EDGE('',*,*,#42656,.T.) ;
#56120=ORIENTED_EDGE('',*,*,#42614,.T.) ;
#56121=ORIENTED_EDGE('',*,*,#42615,.T.) ;
#56122=ORIENTED_EDGE('',*,*,#42656,.F.) ;
#56123=ORIENTED_EDGE('',*,*,#42657,.F.) ;
#56124=ORIENTED_EDGE('',*,*,#42658,.F.) ;
#56125=ORIENTED_EDGE('',*,*,#42659,.F.) ;
#56126=ORIENTED_EDGE('',*,*,#42660,.T.) ;
#56127=ORIENTED_EDGE('',*,*,#42661,.F.) ;
#56128=ORIENTED_EDGE('',*,*,#42662,.F.) ;
#56129=ORIENTED_EDGE('',*,*,#42663,.F.) ;
#56130=ORIENTED_EDGE('',*,*,#42664,.F.) ;
#56131=ORIENTED_EDGE('',*,*,#42665,.F.) ;
#56132=ORIENTED_EDGE('',*,*,#42666,.T.) ;
#56133=ORIENTED_EDGE('',*,*,#42667,.F.) ;
#56134=ORIENTED_EDGE('',*,*,#42668,.F.) ;
#56135=ORIENTED_EDGE('',*,*,#42666,.F.) ;
#56136=ORIENTED_EDGE('',*,*,#42669,.F.) ;
#56137=ORIENTED_EDGE('',*,*,#42670,.T.) ;
#56138=ORIENTED_EDGE('',*,*,#42671,.F.) ;
#56139=ORIENTED_EDGE('',*,*,#42670,.F.) ;
#56140=ORIENTED_EDGE('',*,*,#42672,.F.) ;
#56141=ORIENTED_EDGE('',*,*,#42673,.T.) ;
#56142=ORIENTED_EDGE('',*,*,#42674,.F.) ;
#56143=ORIENTED_EDGE('',*,*,#42675,.F.) ;
#56144=ORIENTED_EDGE('',*,*,#42673,.F.) ;
#56145=ORIENTED_EDGE('',*,*,#42676,.T.) ;
#56146=ORIENTED_EDGE('',*,*,#42677,.F.) ;
#56147=ORIENTED_EDGE('',*,*,#42678,.T.) ;
#56148=ORIENTED_EDGE('',*,*,#42679,.T.) ;
#56149=ORIENTED_EDGE('',*,*,#42680,.T.) ;
#56150=ORIENTED_EDGE('',*,*,#42681,.T.) ;
#56151=ORIENTED_EDGE('',*,*,#42682,.F.) ;
#56152=ORIENTED_EDGE('',*,*,#42676,.F.) ;
#56153=ORIENTED_EDGE('',*,*,#42683,.F.) ;
#56154=ORIENTED_EDGE('',*,*,#42684,.T.) ;
#56155=ORIENTED_EDGE('',*,*,#42685,.F.) ;
#56156=ORIENTED_EDGE('',*,*,#42686,.F.) ;
#56157=ORIENTED_EDGE('',*,*,#42687,.T.) ;
#56158=ORIENTED_EDGE('',*,*,#42688,.F.) ;
#56159=ORIENTED_EDGE('',*,*,#42689,.F.) ;
#56160=ORIENTED_EDGE('',*,*,#42690,.T.) ;
#56161=ORIENTED_EDGE('',*,*,#42669,.T.) ;
#56162=ORIENTED_EDGE('',*,*,#42690,.F.) ;
#56163=ORIENTED_EDGE('',*,*,#42671,.T.) ;
#56164=ORIENTED_EDGE('',*,*,#42691,.T.) ;
#56165=ORIENTED_EDGE('',*,*,#42674,.T.) ;
#56166=ORIENTED_EDGE('',*,*,#42675,.T.) ;
#56167=ORIENTED_EDGE('',*,*,#42691,.F.) ;
#56168=ORIENTED_EDGE('',*,*,#42692,.F.) ;
#56169=ORIENTED_EDGE('',*,*,#42693,.T.) ;
#56170=ORIENTED_EDGE('',*,*,#42694,.F.) ;
#56171=ORIENTED_EDGE('',*,*,#42695,.T.) ;
#56172=ORIENTED_EDGE('',*,*,#42696,.F.) ;
#56173=ORIENTED_EDGE('',*,*,#42697,.T.) ;
#56174=ORIENTED_EDGE('',*,*,#42698,.T.) ;
#56175=ORIENTED_EDGE('',*,*,#42699,.T.) ;
#56176=ORIENTED_EDGE('',*,*,#42700,.F.) ;
#56177=ORIENTED_EDGE('',*,*,#42701,.T.) ;
#56178=ORIENTED_EDGE('',*,*,#42702,.F.) ;
#56179=ORIENTED_EDGE('',*,*,#42703,.T.) ;
#56180=ORIENTED_EDGE('',*,*,#42704,.F.) ;
#56181=ORIENTED_EDGE('',*,*,#42705,.T.) ;
#56182=ORIENTED_EDGE('',*,*,#42706,.T.) ;
#56183=ORIENTED_EDGE('',*,*,#42707,.T.) ;
#56184=ORIENTED_EDGE('',*,*,#42708,.F.) ;
#56185=ORIENTED_EDGE('',*,*,#42709,.T.) ;
#56186=ORIENTED_EDGE('',*,*,#42667,.T.) ;
#56187=ORIENTED_EDGE('',*,*,#42668,.T.) ;
#56188=ORIENTED_EDGE('',*,*,#42709,.F.) ;
#56189=ORIENTED_EDGE('',*,*,#42710,.T.) ;
#56190=ORIENTED_EDGE('',*,*,#42711,.F.) ;
#56191=ORIENTED_EDGE('',*,*,#42712,.T.) ;
#56192=ORIENTED_EDGE('',*,*,#42713,.T.) ;
#56193=ORIENTED_EDGE('',*,*,#42714,.F.) ;
#56194=ORIENTED_EDGE('',*,*,#42715,.T.) ;
#56195=ORIENTED_EDGE('',*,*,#42716,.F.) ;
#56196=ORIENTED_EDGE('',*,*,#42717,.T.) ;
#56197=ORIENTED_EDGE('',*,*,#42718,.F.) ;
#56198=ORIENTED_EDGE('',*,*,#42719,.T.) ;
#56199=ORIENTED_EDGE('',*,*,#42720,.F.) ;
#56200=ORIENTED_EDGE('',*,*,#42721,.T.) ;
#56201=ORIENTED_EDGE('',*,*,#42722,.F.) ;
#56202=ORIENTED_EDGE('',*,*,#42723,.T.) ;
#56203=ORIENTED_EDGE('',*,*,#42724,.F.) ;
#56204=ORIENTED_EDGE('',*,*,#42725,.T.) ;
#56205=ORIENTED_EDGE('',*,*,#42726,.F.) ;
#56206=ORIENTED_EDGE('',*,*,#42727,.T.) ;
#56207=ORIENTED_EDGE('',*,*,#42728,.F.) ;
#56208=ORIENTED_EDGE('',*,*,#42729,.T.) ;
#56209=ORIENTED_EDGE('',*,*,#42730,.F.) ;
#56210=ORIENTED_EDGE('',*,*,#42731,.T.) ;
#56211=ORIENTED_EDGE('',*,*,#42732,.F.) ;
#56212=ORIENTED_EDGE('',*,*,#42733,.T.) ;
#56213=ORIENTED_EDGE('',*,*,#42731,.F.) ;
#56214=ORIENTED_EDGE('',*,*,#42734,.T.) ;
#56215=ORIENTED_EDGE('',*,*,#42735,.F.) ;
#56216=ORIENTED_EDGE('',*,*,#42736,.F.) ;
#56217=ORIENTED_EDGE('',*,*,#42737,.F.) ;
#56218=ORIENTED_EDGE('',*,*,#42733,.F.) ;
#56219=ORIENTED_EDGE('',*,*,#42738,.F.) ;
#56220=ORIENTED_EDGE('',*,*,#42727,.F.) ;
#56221=ORIENTED_EDGE('',*,*,#42739,.F.) ;
#56222=ORIENTED_EDGE('',*,*,#42729,.F.) ;
#56223=ORIENTED_EDGE('',*,*,#42740,.F.) ;
#56224=ORIENTED_EDGE('',*,*,#42723,.F.) ;
#56225=ORIENTED_EDGE('',*,*,#42741,.F.) ;
#56226=ORIENTED_EDGE('',*,*,#42742,.T.) ;
#56227=ORIENTED_EDGE('',*,*,#42743,.T.) ;
#56228=ORIENTED_EDGE('',*,*,#42725,.F.) ;
#56229=ORIENTED_EDGE('',*,*,#42744,.F.) ;
#56230=ORIENTED_EDGE('',*,*,#42745,.F.) ;
#56231=ORIENTED_EDGE('',*,*,#42746,.T.) ;
#56232=ORIENTED_EDGE('',*,*,#42747,.T.) ;
#56233=ORIENTED_EDGE('',*,*,#42748,.T.) ;
#56234=ORIENTED_EDGE('',*,*,#42749,.T.) ;
#56235=ORIENTED_EDGE('',*,*,#42750,.T.) ;
#56236=ORIENTED_EDGE('',*,*,#42751,.T.) ;
#56237=ORIENTED_EDGE('',*,*,#42752,.T.) ;
#56238=ORIENTED_EDGE('',*,*,#42753,.T.) ;
#56239=ORIENTED_EDGE('',*,*,#42754,.T.) ;
#56240=ORIENTED_EDGE('',*,*,#42755,.T.) ;
#56241=ORIENTED_EDGE('',*,*,#42756,.T.) ;
#56242=ORIENTED_EDGE('',*,*,#42757,.T.) ;
#56243=ORIENTED_EDGE('',*,*,#42692,.T.) ;
#56244=ORIENTED_EDGE('',*,*,#42708,.T.) ;
#56245=ORIENTED_EDGE('',*,*,#42758,.T.) ;
#56246=ORIENTED_EDGE('',*,*,#42759,.T.) ;
#56247=ORIENTED_EDGE('',*,*,#42760,.T.) ;
#56248=ORIENTED_EDGE('',*,*,#42761,.T.) ;
#56249=ORIENTED_EDGE('',*,*,#42762,.F.) ;
#56250=ORIENTED_EDGE('',*,*,#42763,.T.) ;
#56251=ORIENTED_EDGE('',*,*,#42625,.F.) ;
#56252=ORIENTED_EDGE('',*,*,#42764,.T.) ;
#56253=ORIENTED_EDGE('',*,*,#42765,.T.) ;
#56254=ORIENTED_EDGE('',*,*,#42766,.F.) ;
#56255=ORIENTED_EDGE('',*,*,#42767,.T.) ;
#56256=ORIENTED_EDGE('',*,*,#42768,.F.) ;
#56257=ORIENTED_EDGE('',*,*,#42769,.T.) ;
#56258=ORIENTED_EDGE('',*,*,#42770,.F.) ;
#56259=ORIENTED_EDGE('',*,*,#42771,.T.) ;
#56260=ORIENTED_EDGE('',*,*,#42772,.F.) ;
#56261=ORIENTED_EDGE('',*,*,#42773,.T.) ;
#56262=ORIENTED_EDGE('',*,*,#42774,.F.) ;
#56263=ORIENTED_EDGE('',*,*,#42775,.T.) ;
#56264=ORIENTED_EDGE('',*,*,#42776,.T.) ;
#56265=ORIENTED_EDGE('',*,*,#42777,.T.) ;
#56266=ORIENTED_EDGE('',*,*,#42778,.T.) ;
#56267=ORIENTED_EDGE('',*,*,#42779,.F.) ;
#56268=ORIENTED_EDGE('',*,*,#42780,.T.) ;
#56269=ORIENTED_EDGE('',*,*,#42678,.F.) ;
#56270=ORIENTED_EDGE('',*,*,#42619,.T.) ;
#56271=ORIENTED_EDGE('',*,*,#42672,.T.) ;
#56272=ORIENTED_EDGE('',*,*,#42781,.T.) ;
#56273=ORIENTED_EDGE('',*,*,#42782,.T.) ;
#56274=ORIENTED_EDGE('',*,*,#42783,.T.) ;
#56275=ORIENTED_EDGE('',*,*,#42784,.T.) ;
#56276=ORIENTED_EDGE('',*,*,#42785,.T.) ;
#56277=ORIENTED_EDGE('',*,*,#42786,.F.) ;
#56278=ORIENTED_EDGE('',*,*,#42787,.T.) ;
#56279=ORIENTED_EDGE('',*,*,#42788,.T.) ;
#56280=ORIENTED_EDGE('',*,*,#42789,.T.) ;
#56281=ORIENTED_EDGE('',*,*,#42790,.T.) ;
#56282=ORIENTED_EDGE('',*,*,#42791,.T.) ;
#56283=ORIENTED_EDGE('',*,*,#42792,.T.) ;
#56284=ORIENTED_EDGE('',*,*,#42793,.T.) ;
#56285=ORIENTED_EDGE('',*,*,#42794,.T.) ;
#56286=ORIENTED_EDGE('',*,*,#42795,.T.) ;
#56287=ORIENTED_EDGE('',*,*,#42796,.T.) ;
#56288=ORIENTED_EDGE('',*,*,#42797,.T.) ;
#56289=ORIENTED_EDGE('',*,*,#42745,.T.) ;
#56290=ORIENTED_EDGE('',*,*,#42798,.F.) ;
#56291=ORIENTED_EDGE('',*,*,#42799,.T.) ;
#56292=ORIENTED_EDGE('',*,*,#42800,.T.) ;
#56293=ORIENTED_EDGE('',*,*,#42801,.T.) ;
#56294=ORIENTED_EDGE('',*,*,#42802,.F.) ;
#56295=ORIENTED_EDGE('',*,*,#42735,.T.) ;
#56296=ORIENTED_EDGE('',*,*,#42803,.F.) ;
#56297=ORIENTED_EDGE('',*,*,#42742,.F.) ;
#56298=ORIENTED_EDGE('',*,*,#42804,.T.) ;
#56299=ORIENTED_EDGE('',*,*,#42805,.T.) ;
#56300=ORIENTED_EDGE('',*,*,#42806,.F.) ;
#56301=ORIENTED_EDGE('',*,*,#42807,.T.) ;
#56302=ORIENTED_EDGE('',*,*,#42808,.F.) ;
#56303=ORIENTED_EDGE('',*,*,#42809,.T.) ;
#56304=ORIENTED_EDGE('',*,*,#42810,.F.) ;
#56305=ORIENTED_EDGE('',*,*,#42811,.T.) ;
#56306=ORIENTED_EDGE('',*,*,#42812,.F.) ;
#56307=ORIENTED_EDGE('',*,*,#42813,.T.) ;
#56308=ORIENTED_EDGE('',*,*,#42814,.F.) ;
#56309=ORIENTED_EDGE('',*,*,#42815,.T.) ;
#56310=ORIENTED_EDGE('',*,*,#42612,.T.) ;
#56311=ORIENTED_EDGE('',*,*,#42816,.F.) ;
#56312=ORIENTED_EDGE('',*,*,#42817,.T.) ;
#56313=ORIENTED_EDGE('',*,*,#42818,.F.) ;
#56314=ORIENTED_EDGE('',*,*,#42819,.T.) ;
#56315=ORIENTED_EDGE('',*,*,#42820,.F.) ;
#56316=ORIENTED_EDGE('',*,*,#42821,.T.) ;
#56317=ORIENTED_EDGE('',*,*,#42822,.F.) ;
#56318=ORIENTED_EDGE('',*,*,#42823,.T.) ;
#56319=ORIENTED_EDGE('',*,*,#42665,.T.) ;
#56320=ORIENTED_EDGE('',*,*,#42824,.T.) ;
#56321=ORIENTED_EDGE('',*,*,#42825,.T.) ;
#56322=ORIENTED_EDGE('',*,*,#42826,.F.) ;
#56323=ORIENTED_EDGE('',*,*,#42827,.T.) ;
#56324=ORIENTED_EDGE('',*,*,#42828,.T.) ;
#56325=ORIENTED_EDGE('',*,*,#42664,.T.) ;
#56326=ORIENTED_EDGE('',*,*,#42829,.F.) ;
#56327=ORIENTED_EDGE('',*,*,#42830,.T.) ;
#56328=ORIENTED_EDGE('',*,*,#42831,.T.) ;
#56329=ORIENTED_EDGE('',*,*,#42832,.T.) ;
#56330=ORIENTED_EDGE('',*,*,#42833,.F.) ;
#56331=ORIENTED_EDGE('',*,*,#42662,.T.) ;
#56332=ORIENTED_EDGE('',*,*,#42834,.T.) ;
#56333=ORIENTED_EDGE('',*,*,#42835,.T.) ;
#56334=ORIENTED_EDGE('',*,*,#42836,.F.) ;
#56335=ORIENTED_EDGE('',*,*,#42837,.T.) ;
#56336=ORIENTED_EDGE('',*,*,#42838,.T.) ;
#56337=ORIENTED_EDGE('',*,*,#42839,.T.) ;
#56338=ORIENTED_EDGE('',*,*,#42840,.T.) ;
#56339=ORIENTED_EDGE('',*,*,#42841,.F.) ;
#56340=ORIENTED_EDGE('',*,*,#42842,.T.) ;
#56341=ORIENTED_EDGE('',*,*,#42843,.F.) ;
#56342=ORIENTED_EDGE('',*,*,#42844,.T.) ;
#56343=ORIENTED_EDGE('',*,*,#42845,.T.) ;
#56344=ORIENTED_EDGE('',*,*,#42846,.T.) ;
#56345=ORIENTED_EDGE('',*,*,#42847,.T.) ;
#56346=ORIENTED_EDGE('',*,*,#42848,.T.) ;
#56347=ORIENTED_EDGE('',*,*,#42849,.F.) ;
#56348=ORIENTED_EDGE('',*,*,#42850,.T.) ;
#56349=ORIENTED_EDGE('',*,*,#42851,.F.) ;
#56350=ORIENTED_EDGE('',*,*,#42852,.T.) ;
#56351=ORIENTED_EDGE('',*,*,#42853,.T.) ;
#56352=ORIENTED_EDGE('',*,*,#42854,.T.) ;
#56353=ORIENTED_EDGE('',*,*,#42855,.T.) ;
#56354=ORIENTED_EDGE('',*,*,#42856,.F.) ;
#56355=ORIENTED_EDGE('',*,*,#42857,.T.) ;
#56356=ORIENTED_EDGE('',*,*,#42858,.F.) ;
#56357=ORIENTED_EDGE('',*,*,#42859,.T.) ;
#56358=ORIENTED_EDGE('',*,*,#42860,.F.) ;
#56359=ORIENTED_EDGE('',*,*,#42861,.T.) ;
#56360=ORIENTED_EDGE('',*,*,#42862,.F.) ;
#56361=ORIENTED_EDGE('',*,*,#42863,.T.) ;
#56362=ORIENTED_EDGE('',*,*,#42864,.F.) ;
#56363=ORIENTED_EDGE('',*,*,#42865,.T.) ;
#56364=ORIENTED_EDGE('',*,*,#42866,.F.) ;
#56365=ORIENTED_EDGE('',*,*,#42867,.T.) ;
#56366=ORIENTED_EDGE('',*,*,#42868,.F.) ;
#56367=ORIENTED_EDGE('',*,*,#42869,.T.) ;
#56368=ORIENTED_EDGE('',*,*,#42870,.F.) ;
#56369=ORIENTED_EDGE('',*,*,#42871,.T.) ;
#56370=ORIENTED_EDGE('',*,*,#42872,.F.) ;
#56371=ORIENTED_EDGE('',*,*,#42873,.T.) ;
#56372=ORIENTED_EDGE('',*,*,#42874,.T.) ;
#56373=ORIENTED_EDGE('',*,*,#42875,.T.) ;
#56374=ORIENTED_EDGE('',*,*,#42876,.F.) ;
#56375=ORIENTED_EDGE('',*,*,#42877,.T.) ;
#56376=ORIENTED_EDGE('',*,*,#42878,.T.) ;
#56377=ORIENTED_EDGE('',*,*,#42879,.T.) ;
#56378=ORIENTED_EDGE('',*,*,#42880,.T.) ;
#56379=ORIENTED_EDGE('',*,*,#42881,.T.) ;
#56380=ORIENTED_EDGE('',*,*,#42882,.T.) ;
#56381=ORIENTED_EDGE('',*,*,#42883,.T.) ;
#56382=ORIENTED_EDGE('',*,*,#42884,.T.) ;
#56383=ORIENTED_EDGE('',*,*,#42885,.T.) ;
#56384=ORIENTED_EDGE('',*,*,#42886,.T.) ;
#56385=ORIENTED_EDGE('',*,*,#42887,.T.) ;
#56386=ORIENTED_EDGE('',*,*,#42888,.F.) ;
#56387=ORIENTED_EDGE('',*,*,#42889,.T.) ;
#56388=ORIENTED_EDGE('',*,*,#42890,.T.) ;
#56389=ORIENTED_EDGE('',*,*,#42891,.T.) ;
#56390=ORIENTED_EDGE('',*,*,#42892,.T.) ;
#56391=ORIENTED_EDGE('',*,*,#42893,.T.) ;
#56392=ORIENTED_EDGE('',*,*,#42894,.T.) ;
#56393=ORIENTED_EDGE('',*,*,#42895,.T.) ;
#56394=ORIENTED_EDGE('',*,*,#42896,.T.) ;
#56395=ORIENTED_EDGE('',*,*,#42897,.T.) ;
#56396=ORIENTED_EDGE('',*,*,#42898,.T.) ;
#56397=ORIENTED_EDGE('',*,*,#42899,.T.) ;
#56398=ORIENTED_EDGE('',*,*,#42900,.T.) ;
#56399=ORIENTED_EDGE('',*,*,#42800,.F.) ;
#56400=ORIENTED_EDGE('',*,*,#42741,.T.) ;
#56401=ORIENTED_EDGE('',*,*,#42797,.F.) ;
#56402=ORIENTED_EDGE('',*,*,#42901,.T.) ;
#56403=ORIENTED_EDGE('',*,*,#42713,.F.) ;
#56404=ORIENTED_EDGE('',*,*,#42902,.T.) ;
#56405=ORIENTED_EDGE('',*,*,#42796,.F.) ;
#56406=ORIENTED_EDGE('',*,*,#42903,.T.) ;
#56407=ORIENTED_EDGE('',*,*,#42754,.F.) ;
#56408=ORIENTED_EDGE('',*,*,#42904,.T.) ;
#56409=ORIENTED_EDGE('',*,*,#42776,.F.) ;
#56410=ORIENTED_EDGE('',*,*,#42905,.T.) ;
#56411=ORIENTED_EDGE('',*,*,#42898,.F.) ;
#56412=ORIENTED_EDGE('',*,*,#42906,.T.) ;
#56413=ORIENTED_EDGE('',*,*,#42748,.F.) ;
#56414=ORIENTED_EDGE('',*,*,#42907,.T.) ;
#56415=ORIENTED_EDGE('',*,*,#42890,.F.) ;
#56416=ORIENTED_EDGE('',*,*,#42908,.T.) ;
#56417=ORIENTED_EDGE('',*,*,#42874,.F.) ;
#56418=ORIENTED_EDGE('',*,*,#42909,.T.) ;
#56419=ORIENTED_EDGE('',*,*,#42854,.F.) ;
#56420=ORIENTED_EDGE('',*,*,#42910,.T.) ;
#56421=ORIENTED_EDGE('',*,*,#42834,.F.) ;
#56422=ORIENTED_EDGE('',*,*,#42911,.T.) ;
#56423=ORIENTED_EDGE('',*,*,#42831,.F.) ;
#56424=ORIENTED_EDGE('',*,*,#42661,.T.) ;
#56425=ORIENTED_EDGE('',*,*,#42828,.F.) ;
#56426=ORIENTED_EDGE('',*,*,#42912,.T.) ;
#56427=ORIENTED_EDGE('',*,*,#42824,.F.) ;
#56428=ORIENTED_EDGE('',*,*,#42913,.T.) ;
#56429=ORIENTED_EDGE('',*,*,#42804,.F.) ;
#56430=ORIENTED_EDGE('',*,*,#42914,.T.) ;
#56431=ORIENTED_EDGE('',*,*,#42915,.T.) ;
#56432=ORIENTED_EDGE('',*,*,#42916,.T.) ;
#56433=ORIENTED_EDGE('',*,*,#42917,.T.) ;
#56434=ORIENTED_EDGE('',*,*,#42918,.T.) ;
#56435=ORIENTED_EDGE('',*,*,#42919,.T.) ;
#56436=ORIENTED_EDGE('',*,*,#42920,.T.) ;
#56437=ORIENTED_EDGE('',*,*,#42921,.T.) ;
#56438=ORIENTED_EDGE('',*,*,#42922,.F.) ;
#56439=ORIENTED_EDGE('',*,*,#42923,.T.) ;
#56440=ORIENTED_EDGE('',*,*,#42924,.T.) ;
#56441=ORIENTED_EDGE('',*,*,#42925,.T.) ;
#56442=ORIENTED_EDGE('',*,*,#42926,.F.) ;
#56443=ORIENTED_EDGE('',*,*,#42927,.T.) ;
#56444=ORIENTED_EDGE('',*,*,#42928,.T.) ;
#56445=ORIENTED_EDGE('',*,*,#42929,.T.) ;
#56446=ORIENTED_EDGE('',*,*,#42930,.T.) ;
#56447=ORIENTED_EDGE('',*,*,#42931,.T.) ;
#56448=ORIENTED_EDGE('',*,*,#42932,.F.) ;
#56449=ORIENTED_EDGE('',*,*,#42933,.T.) ;
#56450=ORIENTED_EDGE('',*,*,#42924,.F.) ;
#56451=ORIENTED_EDGE('',*,*,#42934,.T.) ;
#56452=ORIENTED_EDGE('',*,*,#42935,.T.) ;
#56453=ORIENTED_EDGE('',*,*,#42936,.T.) ;
#56454=ORIENTED_EDGE('',*,*,#42937,.F.) ;
#56455=ORIENTED_EDGE('',*,*,#42938,.T.) ;
#56456=ORIENTED_EDGE('',*,*,#42930,.F.) ;
#56457=ORIENTED_EDGE('',*,*,#42939,.T.) ;
#56458=ORIENTED_EDGE('',*,*,#42940,.F.) ;
#56459=ORIENTED_EDGE('',*,*,#42941,.T.) ;
#56460=ORIENTED_EDGE('',*,*,#42942,.T.) ;
#56461=ORIENTED_EDGE('',*,*,#42943,.T.) ;
#56462=ORIENTED_EDGE('',*,*,#42935,.F.) ;
#56463=ORIENTED_EDGE('',*,*,#42944,.T.) ;
#56464=ORIENTED_EDGE('',*,*,#42945,.T.) ;
#56465=ORIENTED_EDGE('',*,*,#42946,.T.) ;
#56466=ORIENTED_EDGE('',*,*,#42932,.T.) ;
#56467=ORIENTED_EDGE('',*,*,#42947,.T.) ;
#56468=ORIENTED_EDGE('',*,*,#42948,.T.) ;
#56469=ORIENTED_EDGE('',*,*,#42949,.T.) ;
#56470=ORIENTED_EDGE('',*,*,#42950,.T.) ;
#56471=ORIENTED_EDGE('',*,*,#42951,.T.) ;
#56472=ORIENTED_EDGE('',*,*,#42952,.T.) ;
#56473=ORIENTED_EDGE('',*,*,#42953,.T.) ;
#56474=ORIENTED_EDGE('',*,*,#42954,.T.) ;
#56475=ORIENTED_EDGE('',*,*,#42955,.T.) ;
#56476=ORIENTED_EDGE('',*,*,#42956,.T.) ;
#56477=ORIENTED_EDGE('',*,*,#42957,.T.) ;
#56478=ORIENTED_EDGE('',*,*,#42958,.T.) ;
#56479=ORIENTED_EDGE('',*,*,#42959,.T.) ;
#56480=ORIENTED_EDGE('',*,*,#42960,.T.) ;
#56481=ORIENTED_EDGE('',*,*,#42961,.T.) ;
#56482=ORIENTED_EDGE('',*,*,#42962,.T.) ;
#56483=ORIENTED_EDGE('',*,*,#42963,.T.) ;
#56484=ORIENTED_EDGE('',*,*,#42964,.T.) ;
#56485=ORIENTED_EDGE('',*,*,#42965,.T.) ;
#56486=ORIENTED_EDGE('',*,*,#42966,.T.) ;
#56487=ORIENTED_EDGE('',*,*,#42967,.T.) ;
#56488=ORIENTED_EDGE('',*,*,#42968,.T.) ;
#56489=ORIENTED_EDGE('',*,*,#42969,.T.) ;
#56490=ORIENTED_EDGE('',*,*,#42970,.T.) ;
#56491=ORIENTED_EDGE('',*,*,#42971,.T.) ;
#56492=ORIENTED_EDGE('',*,*,#42972,.T.) ;
#56493=ORIENTED_EDGE('',*,*,#42973,.T.) ;
#56494=ORIENTED_EDGE('',*,*,#42974,.T.) ;
#56495=ORIENTED_EDGE('',*,*,#42975,.T.) ;
#56496=ORIENTED_EDGE('',*,*,#42976,.T.) ;
#56497=ORIENTED_EDGE('',*,*,#42977,.T.) ;
#56498=ORIENTED_EDGE('',*,*,#42978,.T.) ;
#56499=ORIENTED_EDGE('',*,*,#42979,.T.) ;
#56500=ORIENTED_EDGE('',*,*,#42980,.T.) ;
#56501=ORIENTED_EDGE('',*,*,#42981,.T.) ;
#56502=ORIENTED_EDGE('',*,*,#42982,.F.) ;
#56503=ORIENTED_EDGE('',*,*,#42983,.F.) ;
#56504=ORIENTED_EDGE('',*,*,#42984,.F.) ;
#56505=ORIENTED_EDGE('',*,*,#42985,.F.) ;
#56506=ORIENTED_EDGE('',*,*,#42986,.F.) ;
#56507=ORIENTED_EDGE('',*,*,#42987,.F.) ;
#56508=ORIENTED_EDGE('',*,*,#42988,.F.) ;
#56509=ORIENTED_EDGE('',*,*,#42989,.F.) ;
#56510=ORIENTED_EDGE('',*,*,#42990,.F.) ;
#56511=ORIENTED_EDGE('',*,*,#42991,.F.) ;
#56512=ORIENTED_EDGE('',*,*,#42989,.T.) ;
#56513=ORIENTED_EDGE('',*,*,#42992,.T.) ;
#56514=ORIENTED_EDGE('',*,*,#42993,.F.) ;
#56515=ORIENTED_EDGE('',*,*,#42994,.F.) ;
#56516=ORIENTED_EDGE('',*,*,#42982,.T.) ;
#56517=ORIENTED_EDGE('',*,*,#42991,.T.) ;
#56518=ORIENTED_EDGE('',*,*,#42995,.F.) ;
#56519=ORIENTED_EDGE('',*,*,#42996,.F.) ;
#56520=ORIENTED_EDGE('',*,*,#42983,.T.) ;
#56521=ORIENTED_EDGE('',*,*,#42994,.T.) ;
#56522=ORIENTED_EDGE('',*,*,#42997,.F.) ;
#56523=ORIENTED_EDGE('',*,*,#42998,.F.) ;
#56524=ORIENTED_EDGE('',*,*,#42984,.T.) ;
#56525=ORIENTED_EDGE('',*,*,#42996,.T.) ;
#56526=ORIENTED_EDGE('',*,*,#42999,.F.) ;
#56527=ORIENTED_EDGE('',*,*,#43000,.F.) ;
#56528=ORIENTED_EDGE('',*,*,#42985,.T.) ;
#56529=ORIENTED_EDGE('',*,*,#42998,.T.) ;
#56530=ORIENTED_EDGE('',*,*,#43001,.F.) ;
#56531=ORIENTED_EDGE('',*,*,#43002,.F.) ;
#56532=ORIENTED_EDGE('',*,*,#42986,.T.) ;
#56533=ORIENTED_EDGE('',*,*,#43000,.T.) ;
#56534=ORIENTED_EDGE('',*,*,#43003,.F.) ;
#56535=ORIENTED_EDGE('',*,*,#43004,.F.) ;
#56536=ORIENTED_EDGE('',*,*,#42987,.T.) ;
#56537=ORIENTED_EDGE('',*,*,#43002,.T.) ;
#56538=ORIENTED_EDGE('',*,*,#43005,.F.) ;
#56539=ORIENTED_EDGE('',*,*,#42992,.F.) ;
#56540=ORIENTED_EDGE('',*,*,#42988,.T.) ;
#56541=ORIENTED_EDGE('',*,*,#43004,.T.) ;
#56542=ORIENTED_EDGE('',*,*,#42993,.T.) ;
#56543=ORIENTED_EDGE('',*,*,#42990,.T.) ;
#56544=ORIENTED_EDGE('',*,*,#43005,.T.) ;
#56545=ORIENTED_EDGE('',*,*,#43003,.T.) ;
#56546=ORIENTED_EDGE('',*,*,#43001,.T.) ;
#56547=ORIENTED_EDGE('',*,*,#42999,.T.) ;
#56548=ORIENTED_EDGE('',*,*,#42997,.T.) ;
#56549=ORIENTED_EDGE('',*,*,#42995,.T.) ;
#56550=ORIENTED_EDGE('',*,*,#42700,.T.) ;
#56551=ORIENTED_EDGE('',*,*,#43006,.T.) ;
#56552=ORIENTED_EDGE('',*,*,#42698,.F.) ;
#56553=ORIENTED_EDGE('',*,*,#43007,.T.) ;
#56554=ORIENTED_EDGE('',*,*,#42702,.T.) ;
#56555=ORIENTED_EDGE('',*,*,#43008,.T.) ;
#56556=ORIENTED_EDGE('',*,*,#42706,.F.) ;
#56557=ORIENTED_EDGE('',*,*,#43009,.T.) ;
#56558=ORIENTED_EDGE('',*,*,#42694,.T.) ;
#56559=ORIENTED_EDGE('',*,*,#43010,.T.) ;
#56560=ORIENTED_EDGE('',*,*,#42696,.T.) ;
#56561=ORIENTED_EDGE('',*,*,#43011,.T.) ;
#56562=ORIENTED_EDGE('',*,*,#42704,.T.) ;
#56563=ORIENTED_EDGE('',*,*,#43012,.T.) ;
#56564=ORIENTED_EDGE('',*,*,#43013,.T.) ;
#56565=ORIENTED_EDGE('',*,*,#43014,.T.) ;
#56566=ORIENTED_EDGE('',*,*,#43015,.T.) ;
#56567=ORIENTED_EDGE('',*,*,#43016,.T.) ;
#56568=ORIENTED_EDGE('',*,*,#43017,.T.) ;
#56569=ORIENTED_EDGE('',*,*,#43018,.T.) ;
#56570=ORIENTED_EDGE('',*,*,#43019,.T.) ;
#56571=ORIENTED_EDGE('',*,*,#43020,.T.) ;
#56572=ORIENTED_EDGE('',*,*,#43021,.T.) ;
#56573=ORIENTED_EDGE('',*,*,#43022,.T.) ;
#56574=ORIENTED_EDGE('',*,*,#43023,.T.) ;
#56575=ORIENTED_EDGE('',*,*,#43024,.T.) ;
#56576=ORIENTED_EDGE('',*,*,#43025,.T.) ;
#56577=ORIENTED_EDGE('',*,*,#43026,.T.) ;
#56578=ORIENTED_EDGE('',*,*,#43027,.T.) ;
#56579=ORIENTED_EDGE('',*,*,#43028,.T.) ;
#56580=ORIENTED_EDGE('',*,*,#43029,.T.) ;
#56581=ORIENTED_EDGE('',*,*,#43030,.T.) ;
#56582=ORIENTED_EDGE('',*,*,#43031,.T.) ;
#56583=ORIENTED_EDGE('',*,*,#43032,.T.) ;
#56584=ORIENTED_EDGE('',*,*,#43033,.F.) ;
#56585=ORIENTED_EDGE('',*,*,#43034,.F.) ;
#56586=ORIENTED_EDGE('',*,*,#43035,.F.) ;
#56587=ORIENTED_EDGE('',*,*,#43036,.F.) ;
#56588=ORIENTED_EDGE('',*,*,#43037,.F.) ;
#56589=ORIENTED_EDGE('',*,*,#43038,.F.) ;
#56590=ORIENTED_EDGE('',*,*,#43039,.F.) ;
#56591=ORIENTED_EDGE('',*,*,#43040,.F.) ;
#56592=ORIENTED_EDGE('',*,*,#43041,.T.) ;
#56593=ORIENTED_EDGE('',*,*,#43042,.T.) ;
#56594=ORIENTED_EDGE('',*,*,#43043,.F.) ;
#56595=ORIENTED_EDGE('',*,*,#43040,.T.) ;
#56596=ORIENTED_EDGE('',*,*,#43043,.T.) ;
#56597=ORIENTED_EDGE('',*,*,#43044,.T.) ;
#56598=ORIENTED_EDGE('',*,*,#43045,.F.) ;
#56599=ORIENTED_EDGE('',*,*,#43033,.T.) ;
#56600=ORIENTED_EDGE('',*,*,#43045,.T.) ;
#56601=ORIENTED_EDGE('',*,*,#43046,.T.) ;
#56602=ORIENTED_EDGE('',*,*,#43047,.F.) ;
#56603=ORIENTED_EDGE('',*,*,#43034,.T.) ;
#56604=ORIENTED_EDGE('',*,*,#43047,.T.) ;
#56605=ORIENTED_EDGE('',*,*,#43048,.T.) ;
#56606=ORIENTED_EDGE('',*,*,#43049,.F.) ;
#56607=ORIENTED_EDGE('',*,*,#43035,.T.) ;
#56608=ORIENTED_EDGE('',*,*,#43049,.T.) ;
#56609=ORIENTED_EDGE('',*,*,#43050,.T.) ;
#56610=ORIENTED_EDGE('',*,*,#43051,.F.) ;
#56611=ORIENTED_EDGE('',*,*,#43036,.T.) ;
#56612=ORIENTED_EDGE('',*,*,#43051,.T.) ;
#56613=ORIENTED_EDGE('',*,*,#43052,.T.) ;
#56614=ORIENTED_EDGE('',*,*,#43053,.F.) ;
#56615=ORIENTED_EDGE('',*,*,#43037,.T.) ;
#56616=ORIENTED_EDGE('',*,*,#43053,.T.) ;
#56617=ORIENTED_EDGE('',*,*,#43054,.T.) ;
#56618=ORIENTED_EDGE('',*,*,#43055,.F.) ;
#56619=ORIENTED_EDGE('',*,*,#43038,.T.) ;
#56620=ORIENTED_EDGE('',*,*,#43055,.T.) ;
#56621=ORIENTED_EDGE('',*,*,#43056,.T.) ;
#56622=ORIENTED_EDGE('',*,*,#43041,.F.) ;
#56623=ORIENTED_EDGE('',*,*,#43039,.T.) ;
#56624=ORIENTED_EDGE('',*,*,#43057,.T.) ;
#56625=ORIENTED_EDGE('',*,*,#43058,.T.) ;
#56626=ORIENTED_EDGE('',*,*,#43059,.T.) ;
#56627=ORIENTED_EDGE('',*,*,#43060,.T.) ;
#56628=ORIENTED_EDGE('',*,*,#43061,.T.) ;
#56629=ORIENTED_EDGE('',*,*,#43062,.T.) ;
#56630=ORIENTED_EDGE('',*,*,#43063,.T.) ;
#56631=ORIENTED_EDGE('',*,*,#43064,.T.) ;
#56632=ORIENTED_EDGE('',*,*,#43065,.T.) ;
#56633=ORIENTED_EDGE('',*,*,#42683,.T.) ;
#56634=ORIENTED_EDGE('',*,*,#43066,.T.) ;
#56635=ORIENTED_EDGE('',*,*,#43067,.T.) ;
#56636=ORIENTED_EDGE('',*,*,#42685,.T.) ;
#56637=ORIENTED_EDGE('',*,*,#43068,.T.) ;
#56638=ORIENTED_EDGE('',*,*,#43069,.T.) ;
#56639=ORIENTED_EDGE('',*,*,#43070,.T.) ;
#56640=ORIENTED_EDGE('',*,*,#43071,.T.) ;
#56641=ORIENTED_EDGE('',*,*,#43072,.T.) ;
#56642=ORIENTED_EDGE('',*,*,#43073,.T.) ;
#56643=ORIENTED_EDGE('',*,*,#43074,.T.) ;
#56644=ORIENTED_EDGE('',*,*,#43075,.T.) ;
#56645=ORIENTED_EDGE('',*,*,#42657,.T.) ;
#56646=ORIENTED_EDGE('',*,*,#42689,.T.) ;
#56647=ORIENTED_EDGE('',*,*,#43076,.T.) ;
#56648=ORIENTED_EDGE('',*,*,#43077,.T.) ;
#56649=ORIENTED_EDGE('',*,*,#43078,.T.) ;
#56650=ORIENTED_EDGE('',*,*,#43079,.T.) ;
#56651=ORIENTED_EDGE('',*,*,#43080,.T.) ;
#56652=ORIENTED_EDGE('',*,*,#43081,.T.) ;
#56653=ORIENTED_EDGE('',*,*,#43082,.F.) ;
#56654=ORIENTED_EDGE('',*,*,#43083,.F.) ;
#56655=ORIENTED_EDGE('',*,*,#43084,.F.) ;
#56656=ORIENTED_EDGE('',*,*,#42847,.F.) ;
#56657=ORIENTED_EDGE('',*,*,#42934,.F.) ;
#56658=ORIENTED_EDGE('',*,*,#42923,.F.) ;
#56659=ORIENTED_EDGE('',*,*,#43085,.F.) ;
#56660=ORIENTED_EDGE('',*,*,#42944,.F.) ;
#56661=ORIENTED_EDGE('',*,*,#43085,.T.) ;
#56662=ORIENTED_EDGE('',*,*,#42922,.T.) ;
#56663=ORIENTED_EDGE('',*,*,#43086,.F.) ;
#56664=ORIENTED_EDGE('',*,*,#43087,.F.) ;
#56665=ORIENTED_EDGE('',*,*,#43086,.T.) ;
#56666=ORIENTED_EDGE('',*,*,#42929,.F.) ;
#56667=ORIENTED_EDGE('',*,*,#43088,.F.) ;
#56668=ORIENTED_EDGE('',*,*,#42960,.F.) ;
#56669=ORIENTED_EDGE('',*,*,#43083,.T.) ;
#56670=ORIENTED_EDGE('',*,*,#42961,.F.) ;
#56671=ORIENTED_EDGE('',*,*,#43089,.F.) ;
#56672=ORIENTED_EDGE('',*,*,#42920,.F.) ;
#56673=ORIENTED_EDGE('',*,*,#43084,.T.) ;
#56674=ORIENTED_EDGE('',*,*,#42919,.F.) ;
#56675=ORIENTED_EDGE('',*,*,#43090,.F.) ;
#56676=ORIENTED_EDGE('',*,*,#42848,.F.) ;
#56677=ORIENTED_EDGE('',*,*,#43082,.T.) ;
#56678=ORIENTED_EDGE('',*,*,#42846,.F.) ;
#56679=ORIENTED_EDGE('',*,*,#43091,.F.) ;
#56680=ORIENTED_EDGE('',*,*,#42956,.F.) ;
#56681=ORIENTED_EDGE('',*,*,#43087,.T.) ;
#56682=ORIENTED_EDGE('',*,*,#42959,.F.) ;
#56683=ORIENTED_EDGE('',*,*,#43092,.F.) ;
#56684=ORIENTED_EDGE('',*,*,#42945,.F.) ;
#56685=ORIENTED_EDGE('',*,*,#42936,.F.) ;
#56686=ORIENTED_EDGE('',*,*,#42946,.F.) ;
#56687=ORIENTED_EDGE('',*,*,#43093,.F.) ;
#56688=ORIENTED_EDGE('',*,*,#42939,.F.) ;
#56689=ORIENTED_EDGE('',*,*,#43089,.T.) ;
#56690=ORIENTED_EDGE('',*,*,#43088,.T.) ;
#56691=ORIENTED_EDGE('',*,*,#43094,.F.) ;
#56692=ORIENTED_EDGE('',*,*,#42849,.T.) ;
#56693=ORIENTED_EDGE('',*,*,#43090,.T.) ;
#56694=ORIENTED_EDGE('',*,*,#43095,.F.) ;
#56695=ORIENTED_EDGE('',*,*,#43096,.F.) ;
#56696=ORIENTED_EDGE('',*,*,#43091,.T.) ;
#56697=ORIENTED_EDGE('',*,*,#42853,.F.) ;
#56698=ORIENTED_EDGE('',*,*,#43097,.F.) ;
#56699=ORIENTED_EDGE('',*,*,#43098,.F.) ;
#56700=ORIENTED_EDGE('',*,*,#43093,.T.) ;
#56701=ORIENTED_EDGE('',*,*,#43092,.T.) ;
#56702=ORIENTED_EDGE('',*,*,#43099,.F.) ;
#56703=ORIENTED_EDGE('',*,*,#42940,.T.) ;
#56704=ORIENTED_EDGE('',*,*,#43094,.T.) ;
#56705=ORIENTED_EDGE('',*,*,#42928,.F.) ;
#56706=ORIENTED_EDGE('',*,*,#43100,.F.) ;
#56707=ORIENTED_EDGE('',*,*,#42921,.F.) ;
#56708=ORIENTED_EDGE('',*,*,#43095,.T.) ;
#56709=ORIENTED_EDGE('',*,*,#42918,.F.) ;
#56710=ORIENTED_EDGE('',*,*,#43101,.F.) ;
#56711=ORIENTED_EDGE('',*,*,#42954,.F.) ;
#56712=ORIENTED_EDGE('',*,*,#43096,.T.) ;
#56713=ORIENTED_EDGE('',*,*,#42953,.F.) ;
#56714=ORIENTED_EDGE('',*,*,#43102,.F.) ;
#56715=ORIENTED_EDGE('',*,*,#42850,.F.) ;
#56716=ORIENTED_EDGE('',*,*,#43097,.T.) ;
#56717=ORIENTED_EDGE('',*,*,#42852,.F.) ;
#56718=ORIENTED_EDGE('',*,*,#43103,.F.) ;
#56719=ORIENTED_EDGE('',*,*,#42915,.F.) ;
#56720=ORIENTED_EDGE('',*,*,#43098,.T.) ;
#56721=ORIENTED_EDGE('',*,*,#42914,.F.) ;
#56722=ORIENTED_EDGE('',*,*,#43104,.F.) ;
#56723=ORIENTED_EDGE('',*,*,#42957,.F.) ;
#56724=ORIENTED_EDGE('',*,*,#43099,.T.) ;
#56725=ORIENTED_EDGE('',*,*,#42958,.F.) ;
#56726=ORIENTED_EDGE('',*,*,#43105,.F.) ;
#56727=ORIENTED_EDGE('',*,*,#42941,.F.) ;
#56728=ORIENTED_EDGE('',*,*,#43101,.T.) ;
#56729=ORIENTED_EDGE('',*,*,#43100,.T.) ;
#56730=ORIENTED_EDGE('',*,*,#43106,.F.) ;
#56731=ORIENTED_EDGE('',*,*,#42851,.T.) ;
#56732=ORIENTED_EDGE('',*,*,#43102,.T.) ;
#56733=ORIENTED_EDGE('',*,*,#43107,.F.) ;
#56734=ORIENTED_EDGE('',*,*,#43103,.T.) ;
#56735=ORIENTED_EDGE('',*,*,#43105,.T.) ;
#56736=ORIENTED_EDGE('',*,*,#43104,.T.) ;
#56737=ORIENTED_EDGE('',*,*,#43108,.F.) ;
#56738=ORIENTED_EDGE('',*,*,#42933,.F.) ;
#56739=ORIENTED_EDGE('',*,*,#42949,.F.) ;
#56740=ORIENTED_EDGE('',*,*,#43109,.F.) ;
#56741=ORIENTED_EDGE('',*,*,#42925,.F.) ;
#56742=ORIENTED_EDGE('',*,*,#43106,.T.) ;
#56743=ORIENTED_EDGE('',*,*,#42927,.F.) ;
#56744=ORIENTED_EDGE('',*,*,#43110,.F.) ;
#56745=ORIENTED_EDGE('',*,*,#42955,.F.) ;
#56746=ORIENTED_EDGE('',*,*,#43107,.T.) ;
#56747=ORIENTED_EDGE('',*,*,#42952,.F.) ;
#56748=ORIENTED_EDGE('',*,*,#43111,.F.) ;
#56749=ORIENTED_EDGE('',*,*,#42916,.F.) ;
#56750=ORIENTED_EDGE('',*,*,#43108,.T.) ;
#56751=ORIENTED_EDGE('',*,*,#42917,.F.) ;
#56752=ORIENTED_EDGE('',*,*,#43112,.F.) ;
#56753=ORIENTED_EDGE('',*,*,#42942,.F.) ;
#56754=ORIENTED_EDGE('',*,*,#42926,.T.) ;
#56755=ORIENTED_EDGE('',*,*,#43109,.T.) ;
#56756=ORIENTED_EDGE('',*,*,#43113,.F.) ;
#56757=ORIENTED_EDGE('',*,*,#43110,.T.) ;
#56758=ORIENTED_EDGE('',*,*,#43112,.T.) ;
#56759=ORIENTED_EDGE('',*,*,#43111,.T.) ;
#56760=ORIENTED_EDGE('',*,*,#43114,.F.) ;
#56761=ORIENTED_EDGE('',*,*,#43113,.T.) ;
#56762=ORIENTED_EDGE('',*,*,#42948,.F.) ;
#56763=ORIENTED_EDGE('',*,*,#43115,.F.) ;
#56764=ORIENTED_EDGE('',*,*,#42950,.F.) ;
#56765=ORIENTED_EDGE('',*,*,#43114,.T.) ;
#56766=ORIENTED_EDGE('',*,*,#42951,.F.) ;
#56767=ORIENTED_EDGE('',*,*,#43116,.F.) ;
#56768=ORIENTED_EDGE('',*,*,#42943,.F.) ;
#56769=ORIENTED_EDGE('',*,*,#43116,.T.) ;
#56770=ORIENTED_EDGE('',*,*,#43115,.T.) ;
#56771=ORIENTED_EDGE('',*,*,#43117,.F.) ;
#56772=ORIENTED_EDGE('',*,*,#42937,.T.) ;
#56773=ORIENTED_EDGE('',*,*,#42931,.F.) ;
#56774=ORIENTED_EDGE('',*,*,#42938,.F.) ;
#56775=ORIENTED_EDGE('',*,*,#43117,.T.) ;
#56776=ORIENTED_EDGE('',*,*,#42947,.F.) ;
#56777=ORIENTED_EDGE('',*,*,#42687,.F.) ;
#56778=ORIENTED_EDGE('',*,*,#42777,.F.) ;
#56779=ORIENTED_EDGE('',*,*,#42904,.F.) ;
#56780=ORIENTED_EDGE('',*,*,#42757,.F.) ;
#56781=ORIENTED_EDGE('',*,*,#42756,.F.) ;
#56782=ORIENTED_EDGE('',*,*,#43118,.T.) ;
#56783=ORIENTED_EDGE('',*,*,#43119,.T.) ;
#56784=ORIENTED_EDGE('',*,*,#42659,.T.) ;
#56785=ORIENTED_EDGE('',*,*,#43061,.F.) ;
#56786=ORIENTED_EDGE('',*,*,#42688,.T.) ;
#56787=ORIENTED_EDGE('',*,*,#43063,.F.) ;
#56788=ORIENTED_EDGE('',*,*,#43120,.T.) ;
#56789=ORIENTED_EDGE('',*,*,#43067,.F.) ;
#56790=ORIENTED_EDGE('',*,*,#43121,.F.) ;
#56791=ORIENTED_EDGE('',*,*,#42686,.T.) ;
#56792=ORIENTED_EDGE('',*,*,#43064,.F.) ;
#56793=ORIENTED_EDGE('',*,*,#43122,.F.) ;
#56794=ORIENTED_EDGE('',*,*,#42778,.F.) ;
#56795=ORIENTED_EDGE('',*,*,#42793,.F.) ;
#56796=ORIENTED_EDGE('',*,*,#43123,.T.) ;
#56797=ORIENTED_EDGE('',*,*,#43071,.F.) ;
#56798=ORIENTED_EDGE('',*,*,#43124,.T.) ;
#56799=ORIENTED_EDGE('',*,*,#43074,.F.) ;
#56800=ORIENTED_EDGE('',*,*,#43125,.T.) ;
#56801=ORIENTED_EDGE('',*,*,#43065,.F.) ;
#56802=ORIENTED_EDGE('',*,*,#43126,.T.) ;
#56803=ORIENTED_EDGE('',*,*,#43122,.T.) ;
#56804=ORIENTED_EDGE('',*,*,#43121,.T.) ;
#56805=ORIENTED_EDGE('',*,*,#43127,.F.) ;
#56806=ORIENTED_EDGE('',*,*,#42779,.T.) ;
#56807=ORIENTED_EDGE('',*,*,#42784,.F.) ;
#56808=ORIENTED_EDGE('',*,*,#42634,.F.) ;
#56809=ORIENTED_EDGE('',*,*,#42760,.F.) ;
#56810=ORIENTED_EDGE('',*,*,#42681,.F.) ;
#56811=ORIENTED_EDGE('',*,*,#43128,.T.) ;
#56812=ORIENTED_EDGE('',*,*,#43129,.T.) ;
#56813=ORIENTED_EDGE('',*,*,#42781,.F.) ;
#56814=ORIENTED_EDGE('',*,*,#42680,.F.) ;
#56815=ORIENTED_EDGE('',*,*,#43069,.F.) ;
#56816=ORIENTED_EDGE('',*,*,#43130,.T.) ;
#56817=ORIENTED_EDGE('',*,*,#43127,.T.) ;
#56818=ORIENTED_EDGE('',*,*,#43066,.F.) ;
#56819=ORIENTED_EDGE('',*,*,#42679,.F.) ;
#56820=ORIENTED_EDGE('',*,*,#42780,.F.) ;
#56821=ORIENTED_EDGE('',*,*,#42682,.T.) ;
#56822=ORIENTED_EDGE('',*,*,#42759,.F.) ;
#56823=ORIENTED_EDGE('',*,*,#42677,.T.) ;
#56824=ORIENTED_EDGE('',*,*,#43070,.F.) ;
#56825=ORIENTED_EDGE('',*,*,#43131,.F.) ;
#56826=ORIENTED_EDGE('',*,*,#43046,.F.) ;
#56827=ORIENTED_EDGE('',*,*,#43132,.F.) ;
#56828=ORIENTED_EDGE('',*,*,#43132,.T.) ;
#56829=ORIENTED_EDGE('',*,*,#43044,.F.) ;
#56830=ORIENTED_EDGE('',*,*,#43133,.F.) ;
#56831=ORIENTED_EDGE('',*,*,#43057,.F.) ;
#56832=ORIENTED_EDGE('',*,*,#43131,.T.) ;
#56833=ORIENTED_EDGE('',*,*,#43060,.F.) ;
#56834=ORIENTED_EDGE('',*,*,#43134,.F.) ;
#56835=ORIENTED_EDGE('',*,*,#43048,.F.) ;
#56836=ORIENTED_EDGE('',*,*,#43133,.T.) ;
#56837=ORIENTED_EDGE('',*,*,#43042,.F.) ;
#56838=ORIENTED_EDGE('',*,*,#43135,.F.) ;
#56839=ORIENTED_EDGE('',*,*,#43050,.F.) ;
#56840=ORIENTED_EDGE('',*,*,#43134,.T.) ;
#56841=ORIENTED_EDGE('',*,*,#43136,.F.) ;
#56842=ORIENTED_EDGE('',*,*,#43135,.T.) ;
#56843=ORIENTED_EDGE('',*,*,#43056,.F.) ;
#56844=ORIENTED_EDGE('',*,*,#43137,.F.) ;
#56845=ORIENTED_EDGE('',*,*,#43058,.F.) ;
#56846=ORIENTED_EDGE('',*,*,#43136,.T.) ;
#56847=ORIENTED_EDGE('',*,*,#43059,.F.) ;
#56848=ORIENTED_EDGE('',*,*,#43138,.F.) ;
#56849=ORIENTED_EDGE('',*,*,#43052,.F.) ;
#56850=ORIENTED_EDGE('',*,*,#43137,.T.) ;
#56851=ORIENTED_EDGE('',*,*,#43054,.F.) ;
#56852=ORIENTED_EDGE('',*,*,#43138,.T.) ;
#56853=ORIENTED_EDGE('',*,*,#43139,.F.) ;
#56854=ORIENTED_EDGE('',*,*,#42871,.F.) ;
#56855=ORIENTED_EDGE('',*,*,#43140,.F.) ;
#56856=ORIENTED_EDGE('',*,*,#42965,.F.) ;
#56857=ORIENTED_EDGE('',*,*,#43140,.T.) ;
#56858=ORIENTED_EDGE('',*,*,#42870,.T.) ;
#56859=ORIENTED_EDGE('',*,*,#43141,.F.) ;
#56860=ORIENTED_EDGE('',*,*,#43142,.F.) ;
#56861=ORIENTED_EDGE('',*,*,#42872,.T.) ;
#56862=ORIENTED_EDGE('',*,*,#43139,.T.) ;
#56863=ORIENTED_EDGE('',*,*,#43143,.F.) ;
#56864=ORIENTED_EDGE('',*,*,#43144,.F.) ;
#56865=ORIENTED_EDGE('',*,*,#43141,.T.) ;
#56866=ORIENTED_EDGE('',*,*,#42869,.F.) ;
#56867=ORIENTED_EDGE('',*,*,#43145,.F.) ;
#56868=ORIENTED_EDGE('',*,*,#42977,.F.) ;
#56869=ORIENTED_EDGE('',*,*,#43142,.T.) ;
#56870=ORIENTED_EDGE('',*,*,#42976,.F.) ;
#56871=ORIENTED_EDGE('',*,*,#43146,.F.) ;
#56872=ORIENTED_EDGE('',*,*,#42962,.F.) ;
#56873=ORIENTED_EDGE('',*,*,#43147,.F.) ;
#56874=ORIENTED_EDGE('',*,*,#42963,.F.) ;
#56875=ORIENTED_EDGE('',*,*,#43148,.F.) ;
#56876=ORIENTED_EDGE('',*,*,#42981,.F.) ;
#56877=ORIENTED_EDGE('',*,*,#43143,.T.) ;
#56878=ORIENTED_EDGE('',*,*,#42964,.F.) ;
#56879=ORIENTED_EDGE('',*,*,#43149,.F.) ;
#56880=ORIENTED_EDGE('',*,*,#42969,.F.) ;
#56881=ORIENTED_EDGE('',*,*,#43144,.T.) ;
#56882=ORIENTED_EDGE('',*,*,#42968,.F.) ;
#56883=ORIENTED_EDGE('',*,*,#43150,.F.) ;
#56884=ORIENTED_EDGE('',*,*,#42873,.F.) ;
#56885=ORIENTED_EDGE('',*,*,#43151,.F.) ;
#56886=ORIENTED_EDGE('',*,*,#42867,.F.) ;
#56887=ORIENTED_EDGE('',*,*,#43152,.F.) ;
#56888=ORIENTED_EDGE('',*,*,#42972,.F.) ;
#56889=ORIENTED_EDGE('',*,*,#42868,.T.) ;
#56890=ORIENTED_EDGE('',*,*,#43151,.T.) ;
#56891=ORIENTED_EDGE('',*,*,#43153,.F.) ;
#56892=ORIENTED_EDGE('',*,*,#43145,.T.) ;
#56893=ORIENTED_EDGE('',*,*,#43148,.T.) ;
#56894=ORIENTED_EDGE('',*,*,#43146,.T.) ;
#56895=ORIENTED_EDGE('',*,*,#43154,.F.) ;
#56896=ORIENTED_EDGE('',*,*,#43149,.T.) ;
#56897=ORIENTED_EDGE('',*,*,#43147,.T.) ;
#56898=ORIENTED_EDGE('',*,*,#43155,.F.) ;
#56899=ORIENTED_EDGE('',*,*,#42866,.T.) ;
#56900=ORIENTED_EDGE('',*,*,#43150,.T.) ;
#56901=ORIENTED_EDGE('',*,*,#43156,.F.) ;
#56902=ORIENTED_EDGE('',*,*,#43152,.T.) ;
#56903=ORIENTED_EDGE('',*,*,#43153,.T.) ;
#56904=ORIENTED_EDGE('',*,*,#42971,.F.) ;
#56905=ORIENTED_EDGE('',*,*,#43157,.F.) ;
#56906=ORIENTED_EDGE('',*,*,#42974,.F.) ;
#56907=ORIENTED_EDGE('',*,*,#43154,.T.) ;
#56908=ORIENTED_EDGE('',*,*,#42975,.F.) ;
#56909=ORIENTED_EDGE('',*,*,#43158,.F.) ;
#56910=ORIENTED_EDGE('',*,*,#42978,.F.) ;
#56911=ORIENTED_EDGE('',*,*,#43155,.T.) ;
#56912=ORIENTED_EDGE('',*,*,#42980,.F.) ;
#56913=ORIENTED_EDGE('',*,*,#43159,.F.) ;
#56914=ORIENTED_EDGE('',*,*,#42966,.F.) ;
#56915=ORIENTED_EDGE('',*,*,#43156,.T.) ;
#56916=ORIENTED_EDGE('',*,*,#42967,.F.) ;
#56917=ORIENTED_EDGE('',*,*,#43160,.F.) ;
#56918=ORIENTED_EDGE('',*,*,#42973,.F.) ;
#56919=ORIENTED_EDGE('',*,*,#43158,.T.) ;
#56920=ORIENTED_EDGE('',*,*,#43157,.T.) ;
#56921=ORIENTED_EDGE('',*,*,#43161,.F.) ;
#56922=ORIENTED_EDGE('',*,*,#43160,.T.) ;
#56923=ORIENTED_EDGE('',*,*,#43159,.T.) ;
#56924=ORIENTED_EDGE('',*,*,#43162,.F.) ;
#56925=ORIENTED_EDGE('',*,*,#43161,.T.) ;
#56926=ORIENTED_EDGE('',*,*,#42970,.F.) ;
#56927=ORIENTED_EDGE('',*,*,#43162,.T.) ;
#56928=ORIENTED_EDGE('',*,*,#42979,.F.) ;
#56929=ORIENTED_EDGE('',*,*,#43163,.F.) ;
#56930=ORIENTED_EDGE('',*,*,#42821,.F.) ;
#56931=ORIENTED_EDGE('',*,*,#43164,.F.) ;
#56932=ORIENTED_EDGE('',*,*,#43024,.F.) ;
#56933=ORIENTED_EDGE('',*,*,#43164,.T.) ;
#56934=ORIENTED_EDGE('',*,*,#42820,.T.) ;
#56935=ORIENTED_EDGE('',*,*,#43165,.F.) ;
#56936=ORIENTED_EDGE('',*,*,#43166,.F.) ;
#56937=ORIENTED_EDGE('',*,*,#42822,.T.) ;
#56938=ORIENTED_EDGE('',*,*,#43163,.T.) ;
#56939=ORIENTED_EDGE('',*,*,#43167,.F.) ;
#56940=ORIENTED_EDGE('',*,*,#43168,.F.) ;
#56941=ORIENTED_EDGE('',*,*,#43165,.T.) ;
#56942=ORIENTED_EDGE('',*,*,#42819,.F.) ;
#56943=ORIENTED_EDGE('',*,*,#43169,.F.) ;
#56944=ORIENTED_EDGE('',*,*,#43020,.F.) ;
#56945=ORIENTED_EDGE('',*,*,#43166,.T.) ;
#56946=ORIENTED_EDGE('',*,*,#43019,.F.) ;
#56947=ORIENTED_EDGE('',*,*,#43170,.F.) ;
#56948=ORIENTED_EDGE('',*,*,#43021,.F.) ;
#56949=ORIENTED_EDGE('',*,*,#43171,.F.) ;
#56950=ORIENTED_EDGE('',*,*,#43022,.F.) ;
#56951=ORIENTED_EDGE('',*,*,#43172,.F.) ;
#56952=ORIENTED_EDGE('',*,*,#43032,.F.) ;
#56953=ORIENTED_EDGE('',*,*,#43167,.T.) ;
#56954=ORIENTED_EDGE('',*,*,#43023,.F.) ;
#56955=ORIENTED_EDGE('',*,*,#43173,.F.) ;
#56956=ORIENTED_EDGE('',*,*,#43028,.F.) ;
#56957=ORIENTED_EDGE('',*,*,#43168,.T.) ;
#56958=ORIENTED_EDGE('',*,*,#43027,.F.) ;
#56959=ORIENTED_EDGE('',*,*,#43174,.F.) ;
#56960=ORIENTED_EDGE('',*,*,#42823,.F.) ;
#56961=ORIENTED_EDGE('',*,*,#43175,.F.) ;
#56962=ORIENTED_EDGE('',*,*,#42817,.F.) ;
#56963=ORIENTED_EDGE('',*,*,#43176,.F.) ;
#56964=ORIENTED_EDGE('',*,*,#43015,.F.) ;
#56965=ORIENTED_EDGE('',*,*,#42818,.T.) ;
#56966=ORIENTED_EDGE('',*,*,#43175,.T.) ;
#56967=ORIENTED_EDGE('',*,*,#43177,.F.) ;
#56968=ORIENTED_EDGE('',*,*,#43169,.T.) ;
#56969=ORIENTED_EDGE('',*,*,#43172,.T.) ;
#56970=ORIENTED_EDGE('',*,*,#43170,.T.) ;
#56971=ORIENTED_EDGE('',*,*,#43178,.F.) ;
#56972=ORIENTED_EDGE('',*,*,#43173,.T.) ;
#56973=ORIENTED_EDGE('',*,*,#43171,.T.) ;
#56974=ORIENTED_EDGE('',*,*,#43179,.F.) ;
#56975=ORIENTED_EDGE('',*,*,#42816,.T.) ;
#56976=ORIENTED_EDGE('',*,*,#43174,.T.) ;
#56977=ORIENTED_EDGE('',*,*,#43180,.F.) ;
#56978=ORIENTED_EDGE('',*,*,#43176,.T.) ;
#56979=ORIENTED_EDGE('',*,*,#43177,.T.) ;
#56980=ORIENTED_EDGE('',*,*,#43014,.F.) ;
#56981=ORIENTED_EDGE('',*,*,#43181,.F.) ;
#56982=ORIENTED_EDGE('',*,*,#43017,.F.) ;
#56983=ORIENTED_EDGE('',*,*,#43178,.T.) ;
#56984=ORIENTED_EDGE('',*,*,#43018,.F.) ;
#56985=ORIENTED_EDGE('',*,*,#43182,.F.) ;
#56986=ORIENTED_EDGE('',*,*,#43029,.F.) ;
#56987=ORIENTED_EDGE('',*,*,#43179,.T.) ;
#56988=ORIENTED_EDGE('',*,*,#43031,.F.) ;
#56989=ORIENTED_EDGE('',*,*,#43183,.F.) ;
#56990=ORIENTED_EDGE('',*,*,#43025,.F.) ;
#56991=ORIENTED_EDGE('',*,*,#43180,.T.) ;
#56992=ORIENTED_EDGE('',*,*,#43026,.F.) ;
#56993=ORIENTED_EDGE('',*,*,#43184,.F.) ;
#56994=ORIENTED_EDGE('',*,*,#43016,.F.) ;
#56995=ORIENTED_EDGE('',*,*,#43182,.T.) ;
#56996=ORIENTED_EDGE('',*,*,#43181,.T.) ;
#56997=ORIENTED_EDGE('',*,*,#43185,.F.) ;
#56998=ORIENTED_EDGE('',*,*,#43184,.T.) ;
#56999=ORIENTED_EDGE('',*,*,#43183,.T.) ;
#57000=ORIENTED_EDGE('',*,*,#43186,.F.) ;
#57001=ORIENTED_EDGE('',*,*,#43185,.T.) ;
#57002=ORIENTED_EDGE('',*,*,#43013,.F.) ;
#57003=ORIENTED_EDGE('',*,*,#43186,.T.) ;
#57004=ORIENTED_EDGE('',*,*,#43030,.F.) ;
#57005=ORIENTED_EDGE('',*,*,#42895,.F.) ;
#57006=ORIENTED_EDGE('',*,*,#43187,.T.) ;
#57007=ORIENTED_EDGE('',*,*,#43076,.F.) ;
#57008=ORIENTED_EDGE('',*,*,#43188,.F.) ;
#57009=ORIENTED_EDGE('',*,*,#42752,.F.) ;
#57010=ORIENTED_EDGE('',*,*,#43189,.F.) ;
#57011=ORIENTED_EDGE('',*,*,#42892,.F.) ;
#57012=ORIENTED_EDGE('',*,*,#43190,.F.) ;
#57013=ORIENTED_EDGE('',*,*,#43190,.T.) ;
#57014=ORIENTED_EDGE('',*,*,#43188,.T.) ;
#57015=ORIENTED_EDGE('',*,*,#43191,.F.) ;
#57016=ORIENTED_EDGE('',*,*,#43191,.T.) ;
#57017=ORIENTED_EDGE('',*,*,#43081,.F.) ;
#57018=ORIENTED_EDGE('',*,*,#43192,.F.) ;
#57019=ORIENTED_EDGE('',*,*,#42753,.F.) ;
#57020=ORIENTED_EDGE('',*,*,#42771,.F.) ;
#57021=ORIENTED_EDGE('',*,*,#43193,.F.) ;
#57022=ORIENTED_EDGE('',*,*,#42750,.F.) ;
#57023=ORIENTED_EDGE('',*,*,#43194,.F.) ;
#57024=ORIENTED_EDGE('',*,*,#43194,.T.) ;
#57025=ORIENTED_EDGE('',*,*,#43192,.T.) ;
#57026=ORIENTED_EDGE('',*,*,#43195,.F.) ;
#57027=ORIENTED_EDGE('',*,*,#42772,.T.) ;
#57028=ORIENTED_EDGE('',*,*,#43195,.T.) ;
#57029=ORIENTED_EDGE('',*,*,#43080,.F.) ;
#57030=ORIENTED_EDGE('',*,*,#43196,.F.) ;
#57031=ORIENTED_EDGE('',*,*,#42773,.F.) ;
#57032=ORIENTED_EDGE('',*,*,#42905,.F.) ;
#57033=ORIENTED_EDGE('',*,*,#42775,.F.) ;
#57034=ORIENTED_EDGE('',*,*,#43197,.F.) ;
#57035=ORIENTED_EDGE('',*,*,#42899,.F.) ;
#57036=ORIENTED_EDGE('',*,*,#42774,.T.) ;
#57037=ORIENTED_EDGE('',*,*,#43196,.T.) ;
#57038=ORIENTED_EDGE('',*,*,#43198,.F.) ;
#57039=ORIENTED_EDGE('',*,*,#43197,.T.) ;
#57040=ORIENTED_EDGE('',*,*,#43198,.T.) ;
#57041=ORIENTED_EDGE('',*,*,#43079,.F.) ;
#57042=ORIENTED_EDGE('',*,*,#43199,.F.) ;
#57043=ORIENTED_EDGE('',*,*,#42896,.F.) ;
#57044=ORIENTED_EDGE('',*,*,#42906,.F.) ;
#57045=ORIENTED_EDGE('',*,*,#42897,.F.) ;
#57046=ORIENTED_EDGE('',*,*,#43200,.F.) ;
#57047=ORIENTED_EDGE('',*,*,#42749,.F.) ;
#57048=ORIENTED_EDGE('',*,*,#43200,.T.) ;
#57049=ORIENTED_EDGE('',*,*,#43199,.T.) ;
#57050=ORIENTED_EDGE('',*,*,#43201,.F.) ;
#57051=ORIENTED_EDGE('',*,*,#43078,.F.) ;
#57052=ORIENTED_EDGE('',*,*,#43202,.T.) ;
#57053=ORIENTED_EDGE('',*,*,#42746,.F.) ;
#57054=ORIENTED_EDGE('',*,*,#43201,.T.) ;
#57055=ORIENTED_EDGE('',*,*,#42889,.F.) ;
#57056=ORIENTED_EDGE('',*,*,#43203,.F.) ;
#57057=ORIENTED_EDGE('',*,*,#42875,.F.) ;
#57058=ORIENTED_EDGE('',*,*,#42908,.F.) ;
#57059=ORIENTED_EDGE('',*,*,#42877,.F.) ;
#57060=ORIENTED_EDGE('',*,*,#43204,.F.) ;
#57061=ORIENTED_EDGE('',*,*,#42855,.F.) ;
#57062=ORIENTED_EDGE('',*,*,#42909,.F.) ;
#57063=ORIENTED_EDGE('',*,*,#42857,.F.) ;
#57064=ORIENTED_EDGE('',*,*,#43205,.F.) ;
#57065=ORIENTED_EDGE('',*,*,#42835,.F.) ;
#57066=ORIENTED_EDGE('',*,*,#42910,.F.) ;
#57067=ORIENTED_EDGE('',*,*,#42837,.F.) ;
#57068=ORIENTED_EDGE('',*,*,#43206,.F.) ;
#57069=ORIENTED_EDGE('',*,*,#42832,.F.) ;
#57070=ORIENTED_EDGE('',*,*,#42911,.F.) ;
#57071=ORIENTED_EDGE('',*,*,#42830,.F.) ;
#57072=ORIENTED_EDGE('',*,*,#43207,.F.) ;
#57073=ORIENTED_EDGE('',*,*,#42825,.F.) ;
#57074=ORIENTED_EDGE('',*,*,#42912,.F.) ;
#57075=ORIENTED_EDGE('',*,*,#42827,.F.) ;
#57076=ORIENTED_EDGE('',*,*,#43208,.F.) ;
#57077=ORIENTED_EDGE('',*,*,#42805,.F.) ;
#57078=ORIENTED_EDGE('',*,*,#42913,.F.) ;
#57079=ORIENTED_EDGE('',*,*,#42695,.F.) ;
#57080=ORIENTED_EDGE('',*,*,#43009,.F.) ;
#57081=ORIENTED_EDGE('',*,*,#42705,.F.) ;
#57082=ORIENTED_EDGE('',*,*,#43011,.F.) ;
#57083=ORIENTED_EDGE('',*,*,#42703,.F.) ;
#57084=ORIENTED_EDGE('',*,*,#43007,.F.) ;
#57085=ORIENTED_EDGE('',*,*,#42697,.F.) ;
#57086=ORIENTED_EDGE('',*,*,#43012,.F.) ;
#57087=ORIENTED_EDGE('',*,*,#42693,.F.) ;
#57088=ORIENTED_EDGE('',*,*,#42758,.F.) ;
#57089=ORIENTED_EDGE('',*,*,#42707,.F.) ;
#57090=ORIENTED_EDGE('',*,*,#43010,.F.) ;
#57091=ORIENTED_EDGE('',*,*,#42701,.F.) ;
#57092=ORIENTED_EDGE('',*,*,#43006,.F.) ;
#57093=ORIENTED_EDGE('',*,*,#42699,.F.) ;
#57094=ORIENTED_EDGE('',*,*,#43008,.F.) ;
#57095=ORIENTED_EDGE('',*,*,#42807,.F.) ;
#57096=ORIENTED_EDGE('',*,*,#43209,.F.) ;
#57097=ORIENTED_EDGE('',*,*,#42801,.F.) ;
#57098=ORIENTED_EDGE('',*,*,#42900,.F.) ;
#57099=ORIENTED_EDGE('',*,*,#42799,.F.) ;
#57100=ORIENTED_EDGE('',*,*,#43210,.F.) ;
#57101=ORIENTED_EDGE('',*,*,#42710,.F.) ;
#57102=ORIENTED_EDGE('',*,*,#42901,.F.) ;
#57103=ORIENTED_EDGE('',*,*,#42712,.F.) ;
#57104=ORIENTED_EDGE('',*,*,#43211,.F.) ;
#57105=ORIENTED_EDGE('',*,*,#42785,.F.) ;
#57106=ORIENTED_EDGE('',*,*,#42902,.F.) ;
#57107=ORIENTED_EDGE('',*,*,#43212,.F.) ;
#57108=ORIENTED_EDGE('',*,*,#42684,.F.) ;
#57109=ORIENTED_EDGE('',*,*,#43125,.F.) ;
#57110=ORIENTED_EDGE('',*,*,#43212,.T.) ;
#57111=ORIENTED_EDGE('',*,*,#43073,.F.) ;
#57112=ORIENTED_EDGE('',*,*,#43213,.F.) ;
#57113=ORIENTED_EDGE('',*,*,#43068,.F.) ;
#57114=ORIENTED_EDGE('',*,*,#43213,.T.) ;
#57115=ORIENTED_EDGE('',*,*,#43072,.F.) ;
#57116=ORIENTED_EDGE('',*,*,#43214,.F.) ;
#57117=ORIENTED_EDGE('',*,*,#43130,.F.) ;
#57118=ORIENTED_EDGE('',*,*,#43214,.T.) ;
#57119=ORIENTED_EDGE('',*,*,#43123,.F.) ;
#57120=ORIENTED_EDGE('',*,*,#43215,.F.) ;
#57121=ORIENTED_EDGE('',*,*,#43128,.F.) ;
#57122=ORIENTED_EDGE('',*,*,#43215,.T.) ;
#57123=ORIENTED_EDGE('',*,*,#42792,.F.) ;
#57124=ORIENTED_EDGE('',*,*,#43216,.F.) ;
#57125=ORIENTED_EDGE('',*,*,#43129,.F.) ;
#57126=ORIENTED_EDGE('',*,*,#43216,.T.) ;
#57127=ORIENTED_EDGE('',*,*,#42791,.F.) ;
#57128=ORIENTED_EDGE('',*,*,#43217,.F.) ;
#57129=ORIENTED_EDGE('',*,*,#42782,.F.) ;
#57130=ORIENTED_EDGE('',*,*,#42903,.F.) ;
#57131=ORIENTED_EDGE('',*,*,#42795,.F.) ;
#57132=ORIENTED_EDGE('',*,*,#43218,.F.) ;
#57133=ORIENTED_EDGE('',*,*,#42755,.F.) ;
#57134=ORIENTED_EDGE('',*,*,#43218,.T.) ;
#57135=ORIENTED_EDGE('',*,*,#42794,.F.) ;
#57136=ORIENTED_EDGE('',*,*,#43219,.F.) ;
#57137=ORIENTED_EDGE('',*,*,#43118,.F.) ;
#57138=ORIENTED_EDGE('',*,*,#43219,.T.) ;
#57139=ORIENTED_EDGE('',*,*,#43124,.F.) ;
#57140=ORIENTED_EDGE('',*,*,#42660,.F.) ;
#57141=ORIENTED_EDGE('',*,*,#43119,.F.) ;
#57142=ORIENTED_EDGE('',*,*,#43220,.F.) ;
#57143=ORIENTED_EDGE('',*,*,#43062,.F.) ;
#57144=ORIENTED_EDGE('',*,*,#42658,.T.) ;
#57145=ORIENTED_EDGE('',*,*,#43075,.F.) ;
#57146=ORIENTED_EDGE('',*,*,#43126,.F.) ;
#57147=ORIENTED_EDGE('',*,*,#43120,.F.) ;
#57148=ORIENTED_EDGE('',*,*,#43220,.T.) ;
#57149=ORIENTED_EDGE('',*,*,#43221,.T.) ;
#57150=ORIENTED_EDGE('',*,*,#43222,.T.) ;
#57151=ORIENTED_EDGE('',*,*,#43077,.F.) ;
#57152=ORIENTED_EDGE('',*,*,#43223,.T.) ;
#57153=ORIENTED_EDGE('',*,*,#43224,.T.) ;
#57154=ORIENTED_EDGE('',*,*,#42894,.F.) ;
#57155=ORIENTED_EDGE('',*,*,#43225,.F.) ;
#57156=ORIENTED_EDGE('',*,*,#42882,.F.) ;
#57157=ORIENTED_EDGE('',*,*,#43226,.F.) ;
#57158=ORIENTED_EDGE('',*,*,#42881,.F.) ;
#57159=ORIENTED_EDGE('',*,*,#43227,.T.) ;
#57160=ORIENTED_EDGE('',*,*,#43187,.F.) ;
#57161=ORIENTED_EDGE('',*,*,#43226,.T.) ;
#57162=ORIENTED_EDGE('',*,*,#42907,.F.) ;
#57163=ORIENTED_EDGE('',*,*,#42747,.F.) ;
#57164=ORIENTED_EDGE('',*,*,#43228,.F.) ;
#57165=ORIENTED_EDGE('',*,*,#42891,.F.) ;
#57166=ORIENTED_EDGE('',*,*,#43202,.F.) ;
#57167=ORIENTED_EDGE('',*,*,#43229,.T.) ;
#57168=ORIENTED_EDGE('',*,*,#42878,.F.) ;
#57169=ORIENTED_EDGE('',*,*,#43228,.T.) ;
#57170=ORIENTED_EDGE('',*,*,#43223,.F.) ;
#57171=ORIENTED_EDGE('',*,*,#43227,.F.) ;
#57172=ORIENTED_EDGE('',*,*,#43230,.F.) ;
#57173=ORIENTED_EDGE('',*,*,#43231,.F.) ;
#57174=ORIENTED_EDGE('',*,*,#43224,.F.) ;
#57175=ORIENTED_EDGE('',*,*,#43230,.T.) ;
#57176=ORIENTED_EDGE('',*,*,#42880,.F.) ;
#57177=ORIENTED_EDGE('',*,*,#43231,.T.) ;
#57178=ORIENTED_EDGE('',*,*,#42879,.F.) ;
#57179=ORIENTED_EDGE('',*,*,#43232,.F.) ;
#57180=ORIENTED_EDGE('',*,*,#43221,.F.) ;
#57181=ORIENTED_EDGE('',*,*,#43232,.T.) ;
#57182=ORIENTED_EDGE('',*,*,#43229,.F.) ;
#57183=ORIENTED_EDGE('',*,*,#43222,.F.) ;
#57184=ORIENTED_EDGE('',*,*,#42734,.F.) ;
#57185=ORIENTED_EDGE('',*,*,#42730,.T.) ;
#57186=ORIENTED_EDGE('',*,*,#42737,.T.) ;
#57187=ORIENTED_EDGE('',*,*,#42726,.T.) ;
#57188=ORIENTED_EDGE('',*,*,#42739,.T.) ;
#57189=ORIENTED_EDGE('',*,*,#42722,.T.) ;
#57190=ORIENTED_EDGE('',*,*,#42743,.F.) ;
#57191=ORIENTED_EDGE('',*,*,#42803,.T.) ;
#57192=ORIENTED_EDGE('',*,*,#43233,.T.) ;
#57193=ORIENTED_EDGE('',*,*,#43234,.T.) ;
#57194=ORIENTED_EDGE('',*,*,#43235,.F.) ;
#57195=ORIENTED_EDGE('',*,*,#43236,.T.) ;
#57196=ORIENTED_EDGE('',*,*,#43235,.T.) ;
#57197=ORIENTED_EDGE('',*,*,#43237,.T.) ;
#57198=ORIENTED_EDGE('',*,*,#43238,.F.) ;
#57199=ORIENTED_EDGE('',*,*,#43239,.T.) ;
#57200=ORIENTED_EDGE('',*,*,#43238,.T.) ;
#57201=ORIENTED_EDGE('',*,*,#43240,.T.) ;
#57202=ORIENTED_EDGE('',*,*,#43241,.F.) ;
#57203=ORIENTED_EDGE('',*,*,#43242,.T.) ;
#57204=ORIENTED_EDGE('',*,*,#43241,.T.) ;
#57205=ORIENTED_EDGE('',*,*,#43243,.T.) ;
#57206=ORIENTED_EDGE('',*,*,#43244,.F.) ;
#57207=ORIENTED_EDGE('',*,*,#43245,.T.) ;
#57208=ORIENTED_EDGE('',*,*,#43244,.T.) ;
#57209=ORIENTED_EDGE('',*,*,#43246,.T.) ;
#57210=ORIENTED_EDGE('',*,*,#43247,.F.) ;
#57211=ORIENTED_EDGE('',*,*,#43248,.T.) ;
#57212=ORIENTED_EDGE('',*,*,#43247,.T.) ;
#57213=ORIENTED_EDGE('',*,*,#43249,.T.) ;
#57214=ORIENTED_EDGE('',*,*,#43250,.F.) ;
#57215=ORIENTED_EDGE('',*,*,#43251,.T.) ;
#57216=ORIENTED_EDGE('',*,*,#43250,.T.) ;
#57217=ORIENTED_EDGE('',*,*,#43252,.T.) ;
#57218=ORIENTED_EDGE('',*,*,#43253,.F.) ;
#57219=ORIENTED_EDGE('',*,*,#43254,.T.) ;
#57220=ORIENTED_EDGE('',*,*,#43253,.T.) ;
#57221=ORIENTED_EDGE('',*,*,#43255,.T.) ;
#57222=ORIENTED_EDGE('',*,*,#43256,.F.) ;
#57223=ORIENTED_EDGE('',*,*,#43257,.T.) ;
#57224=ORIENTED_EDGE('',*,*,#43256,.T.) ;
#57225=ORIENTED_EDGE('',*,*,#43258,.T.) ;
#57226=ORIENTED_EDGE('',*,*,#43259,.T.) ;
#57227=ORIENTED_EDGE('',*,*,#43260,.T.) ;
#57228=ORIENTED_EDGE('',*,*,#43261,.T.) ;
#57229=ORIENTED_EDGE('',*,*,#43262,.T.) ;
#57230=ORIENTED_EDGE('',*,*,#43263,.T.) ;
#57231=ORIENTED_EDGE('',*,*,#43264,.T.) ;
#57232=ORIENTED_EDGE('',*,*,#43265,.T.) ;
#57233=ORIENTED_EDGE('',*,*,#43266,.T.) ;
#57234=ORIENTED_EDGE('',*,*,#43267,.T.) ;
#57235=ORIENTED_EDGE('',*,*,#43268,.T.) ;
#57236=ORIENTED_EDGE('',*,*,#43269,.T.) ;
#57237=ORIENTED_EDGE('',*,*,#43270,.T.) ;
#57238=ORIENTED_EDGE('',*,*,#43271,.T.) ;
#57239=ORIENTED_EDGE('',*,*,#43272,.T.) ;
#57240=ORIENTED_EDGE('',*,*,#43273,.T.) ;
#57241=ORIENTED_EDGE('',*,*,#43274,.T.) ;
#57242=ORIENTED_EDGE('',*,*,#43275,.F.) ;
#57243=ORIENTED_EDGE('',*,*,#43276,.T.) ;
#57244=ORIENTED_EDGE('',*,*,#43277,.T.) ;
#57245=ORIENTED_EDGE('',*,*,#43278,.T.) ;
#57246=ORIENTED_EDGE('',*,*,#42639,.T.) ;
#57247=ORIENTED_EDGE('',*,*,#42655,.T.) ;
#57248=ORIENTED_EDGE('',*,*,#43279,.T.) ;
#57249=ORIENTED_EDGE('',*,*,#43280,.T.) ;
#57250=ORIENTED_EDGE('',*,*,#43281,.T.) ;
#57251=ORIENTED_EDGE('',*,*,#43282,.F.) ;
#57252=ORIENTED_EDGE('',*,*,#43283,.T.) ;
#57253=ORIENTED_EDGE('',*,*,#43284,.F.) ;
#57254=ORIENTED_EDGE('',*,*,#43285,.T.) ;
#57255=ORIENTED_EDGE('',*,*,#43286,.T.) ;
#57256=ORIENTED_EDGE('',*,*,#43287,.T.) ;
#57257=ORIENTED_EDGE('',*,*,#42888,.T.) ;
#57258=ORIENTED_EDGE('',*,*,#43288,.T.) ;
#57259=ORIENTED_EDGE('',*,*,#43284,.T.) ;
#57260=ORIENTED_EDGE('',*,*,#43289,.T.) ;
#57261=ORIENTED_EDGE('',*,*,#43275,.T.) ;
#57262=ORIENTED_EDGE('',*,*,#43290,.T.) ;
#57263=ORIENTED_EDGE('',*,*,#42766,.T.) ;
#57264=ORIENTED_EDGE('',*,*,#43291,.T.) ;
#57265=ORIENTED_EDGE('',*,*,#43282,.T.) ;
#57266=ORIENTED_EDGE('',*,*,#43292,.T.) ;
#57267=ORIENTED_EDGE('',*,*,#42786,.T.) ;
#57268=ORIENTED_EDGE('',*,*,#43211,.T.) ;
#57269=ORIENTED_EDGE('',*,*,#42711,.T.) ;
#57270=ORIENTED_EDGE('',*,*,#43210,.T.) ;
#57271=ORIENTED_EDGE('',*,*,#42798,.T.) ;
#57272=ORIENTED_EDGE('',*,*,#42744,.T.) ;
#57273=ORIENTED_EDGE('',*,*,#42724,.T.) ;
#57274=ORIENTED_EDGE('',*,*,#42740,.T.) ;
#57275=ORIENTED_EDGE('',*,*,#42728,.T.) ;
#57276=ORIENTED_EDGE('',*,*,#42738,.T.) ;
#57277=ORIENTED_EDGE('',*,*,#42732,.T.) ;
#57278=ORIENTED_EDGE('',*,*,#42736,.T.) ;
#57279=ORIENTED_EDGE('',*,*,#42802,.T.) ;
#57280=ORIENTED_EDGE('',*,*,#43209,.T.) ;
#57281=ORIENTED_EDGE('',*,*,#42806,.T.) ;
#57282=ORIENTED_EDGE('',*,*,#43208,.T.) ;
#57283=ORIENTED_EDGE('',*,*,#42826,.T.) ;
#57284=ORIENTED_EDGE('',*,*,#43207,.T.) ;
#57285=ORIENTED_EDGE('',*,*,#42829,.T.) ;
#57286=ORIENTED_EDGE('',*,*,#42663,.T.) ;
#57287=ORIENTED_EDGE('',*,*,#42833,.T.) ;
#57288=ORIENTED_EDGE('',*,*,#43206,.T.) ;
#57289=ORIENTED_EDGE('',*,*,#42836,.T.) ;
#57290=ORIENTED_EDGE('',*,*,#43205,.T.) ;
#57291=ORIENTED_EDGE('',*,*,#42856,.T.) ;
#57292=ORIENTED_EDGE('',*,*,#43204,.T.) ;
#57293=ORIENTED_EDGE('',*,*,#42876,.T.) ;
#57294=ORIENTED_EDGE('',*,*,#43203,.T.) ;
#57295=ORIENTED_EDGE('',*,*,#43293,.T.) ;
#57296=ORIENTED_EDGE('',*,*,#43294,.T.) ;
#57297=ORIENTED_EDGE('',*,*,#43295,.T.) ;
#57298=ORIENTED_EDGE('',*,*,#43296,.T.) ;
#57299=ORIENTED_EDGE('',*,*,#43297,.T.) ;
#57300=ORIENTED_EDGE('',*,*,#43298,.T.) ;
#57301=ORIENTED_EDGE('',*,*,#43299,.T.) ;
#57302=ORIENTED_EDGE('',*,*,#43300,.T.) ;
#57303=ORIENTED_EDGE('',*,*,#43301,.F.) ;
#57304=ORIENTED_EDGE('',*,*,#43302,.T.) ;
#57305=ORIENTED_EDGE('',*,*,#43303,.T.) ;
#57306=ORIENTED_EDGE('',*,*,#43304,.T.) ;
#57307=ORIENTED_EDGE('',*,*,#43305,.F.) ;
#57308=ORIENTED_EDGE('',*,*,#43306,.T.) ;
#57309=ORIENTED_EDGE('',*,*,#43307,.T.) ;
#57310=ORIENTED_EDGE('',*,*,#43308,.T.) ;
#57311=ORIENTED_EDGE('',*,*,#43309,.T.) ;
#57312=ORIENTED_EDGE('',*,*,#43310,.T.) ;
#57313=ORIENTED_EDGE('',*,*,#43311,.F.) ;
#57314=ORIENTED_EDGE('',*,*,#43312,.T.) ;
#57315=ORIENTED_EDGE('',*,*,#43303,.F.) ;
#57316=ORIENTED_EDGE('',*,*,#43313,.T.) ;
#57317=ORIENTED_EDGE('',*,*,#43314,.T.) ;
#57318=ORIENTED_EDGE('',*,*,#43315,.T.) ;
#57319=ORIENTED_EDGE('',*,*,#43316,.F.) ;
#57320=ORIENTED_EDGE('',*,*,#43317,.T.) ;
#57321=ORIENTED_EDGE('',*,*,#43309,.F.) ;
#57322=ORIENTED_EDGE('',*,*,#43318,.T.) ;
#57323=ORIENTED_EDGE('',*,*,#43319,.F.) ;
#57324=ORIENTED_EDGE('',*,*,#43320,.T.) ;
#57325=ORIENTED_EDGE('',*,*,#43321,.T.) ;
#57326=ORIENTED_EDGE('',*,*,#43322,.T.) ;
#57327=ORIENTED_EDGE('',*,*,#43314,.F.) ;
#57328=ORIENTED_EDGE('',*,*,#43323,.T.) ;
#57329=ORIENTED_EDGE('',*,*,#43324,.T.) ;
#57330=ORIENTED_EDGE('',*,*,#43325,.T.) ;
#57331=ORIENTED_EDGE('',*,*,#43311,.T.) ;
#57332=ORIENTED_EDGE('',*,*,#43326,.T.) ;
#57333=ORIENTED_EDGE('',*,*,#43327,.T.) ;
#57334=ORIENTED_EDGE('',*,*,#43328,.T.) ;
#57335=ORIENTED_EDGE('',*,*,#43329,.T.) ;
#57336=ORIENTED_EDGE('',*,*,#43330,.T.) ;
#57337=ORIENTED_EDGE('',*,*,#43331,.T.) ;
#57338=ORIENTED_EDGE('',*,*,#43332,.T.) ;
#57339=ORIENTED_EDGE('',*,*,#43333,.T.) ;
#57340=ORIENTED_EDGE('',*,*,#43334,.T.) ;
#57341=ORIENTED_EDGE('',*,*,#43335,.T.) ;
#57342=ORIENTED_EDGE('',*,*,#43336,.T.) ;
#57343=ORIENTED_EDGE('',*,*,#43337,.T.) ;
#57344=ORIENTED_EDGE('',*,*,#43338,.T.) ;
#57345=ORIENTED_EDGE('',*,*,#43339,.T.) ;
#57346=ORIENTED_EDGE('',*,*,#43340,.T.) ;
#57347=ORIENTED_EDGE('',*,*,#43341,.T.) ;
#57348=ORIENTED_EDGE('',*,*,#43342,.T.) ;
#57349=ORIENTED_EDGE('',*,*,#43343,.T.) ;
#57350=ORIENTED_EDGE('',*,*,#43344,.T.) ;
#57351=ORIENTED_EDGE('',*,*,#43345,.T.) ;
#57352=ORIENTED_EDGE('',*,*,#43346,.T.) ;
#57353=ORIENTED_EDGE('',*,*,#43347,.T.) ;
#57354=ORIENTED_EDGE('',*,*,#43348,.T.) ;
#57355=ORIENTED_EDGE('',*,*,#43349,.T.) ;
#57356=ORIENTED_EDGE('',*,*,#43350,.T.) ;
#57357=ORIENTED_EDGE('',*,*,#43351,.T.) ;
#57358=ORIENTED_EDGE('',*,*,#43352,.T.) ;
#57359=ORIENTED_EDGE('',*,*,#43353,.T.) ;
#57360=ORIENTED_EDGE('',*,*,#43354,.T.) ;
#57361=ORIENTED_EDGE('',*,*,#43355,.T.) ;
#57362=ORIENTED_EDGE('',*,*,#43356,.T.) ;
#57363=ORIENTED_EDGE('',*,*,#43357,.T.) ;
#57364=ORIENTED_EDGE('',*,*,#43358,.T.) ;
#57365=ORIENTED_EDGE('',*,*,#43359,.T.) ;
#57366=ORIENTED_EDGE('',*,*,#43360,.T.) ;
#57367=ORIENTED_EDGE('',*,*,#43361,.F.) ;
#57368=ORIENTED_EDGE('',*,*,#43362,.F.) ;
#57369=ORIENTED_EDGE('',*,*,#43363,.F.) ;
#57370=ORIENTED_EDGE('',*,*,#43364,.F.) ;
#57371=ORIENTED_EDGE('',*,*,#43365,.F.) ;
#57372=ORIENTED_EDGE('',*,*,#43366,.F.) ;
#57373=ORIENTED_EDGE('',*,*,#43367,.F.) ;
#57374=ORIENTED_EDGE('',*,*,#43368,.F.) ;
#57375=ORIENTED_EDGE('',*,*,#43369,.F.) ;
#57376=ORIENTED_EDGE('',*,*,#43370,.F.) ;
#57377=ORIENTED_EDGE('',*,*,#43368,.T.) ;
#57378=ORIENTED_EDGE('',*,*,#43371,.T.) ;
#57379=ORIENTED_EDGE('',*,*,#43372,.F.) ;
#57380=ORIENTED_EDGE('',*,*,#43373,.F.) ;
#57381=ORIENTED_EDGE('',*,*,#43361,.T.) ;
#57382=ORIENTED_EDGE('',*,*,#43370,.T.) ;
#57383=ORIENTED_EDGE('',*,*,#43374,.F.) ;
#57384=ORIENTED_EDGE('',*,*,#43375,.F.) ;
#57385=ORIENTED_EDGE('',*,*,#43362,.T.) ;
#57386=ORIENTED_EDGE('',*,*,#43373,.T.) ;
#57387=ORIENTED_EDGE('',*,*,#43376,.F.) ;
#57388=ORIENTED_EDGE('',*,*,#43377,.F.) ;
#57389=ORIENTED_EDGE('',*,*,#43363,.T.) ;
#57390=ORIENTED_EDGE('',*,*,#43375,.T.) ;
#57391=ORIENTED_EDGE('',*,*,#43378,.F.) ;
#57392=ORIENTED_EDGE('',*,*,#43379,.F.) ;
#57393=ORIENTED_EDGE('',*,*,#43364,.T.) ;
#57394=ORIENTED_EDGE('',*,*,#43377,.T.) ;
#57395=ORIENTED_EDGE('',*,*,#43380,.F.) ;
#57396=ORIENTED_EDGE('',*,*,#43381,.F.) ;
#57397=ORIENTED_EDGE('',*,*,#43365,.T.) ;
#57398=ORIENTED_EDGE('',*,*,#43379,.T.) ;
#57399=ORIENTED_EDGE('',*,*,#43382,.F.) ;
#57400=ORIENTED_EDGE('',*,*,#43383,.F.) ;
#57401=ORIENTED_EDGE('',*,*,#43366,.T.) ;
#57402=ORIENTED_EDGE('',*,*,#43381,.T.) ;
#57403=ORIENTED_EDGE('',*,*,#43384,.F.) ;
#57404=ORIENTED_EDGE('',*,*,#43371,.F.) ;
#57405=ORIENTED_EDGE('',*,*,#43367,.T.) ;
#57406=ORIENTED_EDGE('',*,*,#43383,.T.) ;
#57407=ORIENTED_EDGE('',*,*,#43372,.T.) ;
#57408=ORIENTED_EDGE('',*,*,#43369,.T.) ;
#57409=ORIENTED_EDGE('',*,*,#43384,.T.) ;
#57410=ORIENTED_EDGE('',*,*,#43382,.T.) ;
#57411=ORIENTED_EDGE('',*,*,#43380,.T.) ;
#57412=ORIENTED_EDGE('',*,*,#43378,.T.) ;
#57413=ORIENTED_EDGE('',*,*,#43376,.T.) ;
#57414=ORIENTED_EDGE('',*,*,#43374,.T.) ;
#57415=ORIENTED_EDGE('',*,*,#42647,.T.) ;
#57416=ORIENTED_EDGE('',*,*,#43385,.T.) ;
#57417=ORIENTED_EDGE('',*,*,#42645,.F.) ;
#57418=ORIENTED_EDGE('',*,*,#43386,.T.) ;
#57419=ORIENTED_EDGE('',*,*,#42649,.T.) ;
#57420=ORIENTED_EDGE('',*,*,#43387,.T.) ;
#57421=ORIENTED_EDGE('',*,*,#42653,.F.) ;
#57422=ORIENTED_EDGE('',*,*,#43388,.T.) ;
#57423=ORIENTED_EDGE('',*,*,#42641,.T.) ;
#57424=ORIENTED_EDGE('',*,*,#43389,.T.) ;
#57425=ORIENTED_EDGE('',*,*,#42643,.T.) ;
#57426=ORIENTED_EDGE('',*,*,#43390,.T.) ;
#57427=ORIENTED_EDGE('',*,*,#42651,.T.) ;
#57428=ORIENTED_EDGE('',*,*,#43391,.T.) ;
#57429=ORIENTED_EDGE('',*,*,#43392,.T.) ;
#57430=ORIENTED_EDGE('',*,*,#43393,.T.) ;
#57431=ORIENTED_EDGE('',*,*,#43394,.T.) ;
#57432=ORIENTED_EDGE('',*,*,#43395,.T.) ;
#57433=ORIENTED_EDGE('',*,*,#43396,.T.) ;
#57434=ORIENTED_EDGE('',*,*,#43397,.T.) ;
#57435=ORIENTED_EDGE('',*,*,#43398,.T.) ;
#57436=ORIENTED_EDGE('',*,*,#43399,.T.) ;
#57437=ORIENTED_EDGE('',*,*,#43400,.T.) ;
#57438=ORIENTED_EDGE('',*,*,#43401,.T.) ;
#57439=ORIENTED_EDGE('',*,*,#43402,.T.) ;
#57440=ORIENTED_EDGE('',*,*,#43403,.T.) ;
#57441=ORIENTED_EDGE('',*,*,#43404,.T.) ;
#57442=ORIENTED_EDGE('',*,*,#43405,.T.) ;
#57443=ORIENTED_EDGE('',*,*,#43406,.T.) ;
#57444=ORIENTED_EDGE('',*,*,#43407,.T.) ;
#57445=ORIENTED_EDGE('',*,*,#43408,.T.) ;
#57446=ORIENTED_EDGE('',*,*,#43409,.T.) ;
#57447=ORIENTED_EDGE('',*,*,#43410,.T.) ;
#57448=ORIENTED_EDGE('',*,*,#43411,.T.) ;
#57449=ORIENTED_EDGE('',*,*,#43412,.F.) ;
#57450=ORIENTED_EDGE('',*,*,#43413,.F.) ;
#57451=ORIENTED_EDGE('',*,*,#43414,.F.) ;
#57452=ORIENTED_EDGE('',*,*,#43415,.F.) ;
#57453=ORIENTED_EDGE('',*,*,#43416,.F.) ;
#57454=ORIENTED_EDGE('',*,*,#43417,.F.) ;
#57455=ORIENTED_EDGE('',*,*,#43418,.F.) ;
#57456=ORIENTED_EDGE('',*,*,#43419,.F.) ;
#57457=ORIENTED_EDGE('',*,*,#43420,.T.) ;
#57458=ORIENTED_EDGE('',*,*,#43421,.T.) ;
#57459=ORIENTED_EDGE('',*,*,#43422,.F.) ;
#57460=ORIENTED_EDGE('',*,*,#43419,.T.) ;
#57461=ORIENTED_EDGE('',*,*,#43422,.T.) ;
#57462=ORIENTED_EDGE('',*,*,#43423,.T.) ;
#57463=ORIENTED_EDGE('',*,*,#43424,.F.) ;
#57464=ORIENTED_EDGE('',*,*,#43412,.T.) ;
#57465=ORIENTED_EDGE('',*,*,#43424,.T.) ;
#57466=ORIENTED_EDGE('',*,*,#43425,.T.) ;
#57467=ORIENTED_EDGE('',*,*,#43426,.F.) ;
#57468=ORIENTED_EDGE('',*,*,#43413,.T.) ;
#57469=ORIENTED_EDGE('',*,*,#43426,.T.) ;
#57470=ORIENTED_EDGE('',*,*,#43427,.T.) ;
#57471=ORIENTED_EDGE('',*,*,#43428,.F.) ;
#57472=ORIENTED_EDGE('',*,*,#43414,.T.) ;
#57473=ORIENTED_EDGE('',*,*,#43428,.T.) ;
#57474=ORIENTED_EDGE('',*,*,#43429,.T.) ;
#57475=ORIENTED_EDGE('',*,*,#43430,.F.) ;
#57476=ORIENTED_EDGE('',*,*,#43415,.T.) ;
#57477=ORIENTED_EDGE('',*,*,#43430,.T.) ;
#57478=ORIENTED_EDGE('',*,*,#43431,.T.) ;
#57479=ORIENTED_EDGE('',*,*,#43432,.F.) ;
#57480=ORIENTED_EDGE('',*,*,#43416,.T.) ;
#57481=ORIENTED_EDGE('',*,*,#43432,.T.) ;
#57482=ORIENTED_EDGE('',*,*,#43433,.T.) ;
#57483=ORIENTED_EDGE('',*,*,#43434,.F.) ;
#57484=ORIENTED_EDGE('',*,*,#43417,.T.) ;
#57485=ORIENTED_EDGE('',*,*,#43434,.T.) ;
#57486=ORIENTED_EDGE('',*,*,#43435,.T.) ;
#57487=ORIENTED_EDGE('',*,*,#43420,.F.) ;
#57488=ORIENTED_EDGE('',*,*,#43418,.T.) ;
#57489=ORIENTED_EDGE('',*,*,#43436,.T.) ;
#57490=ORIENTED_EDGE('',*,*,#43437,.T.) ;
#57491=ORIENTED_EDGE('',*,*,#43438,.T.) ;
#57492=ORIENTED_EDGE('',*,*,#43439,.T.) ;
#57493=ORIENTED_EDGE('',*,*,#43440,.T.) ;
#57494=ORIENTED_EDGE('',*,*,#43441,.T.) ;
#57495=ORIENTED_EDGE('',*,*,#43442,.T.) ;
#57496=ORIENTED_EDGE('',*,*,#43443,.T.) ;
#57497=ORIENTED_EDGE('',*,*,#43444,.T.) ;
#57498=ORIENTED_EDGE('',*,*,#42630,.T.) ;
#57499=ORIENTED_EDGE('',*,*,#43445,.T.) ;
#57500=ORIENTED_EDGE('',*,*,#43446,.T.) ;
#57501=ORIENTED_EDGE('',*,*,#42632,.T.) ;
#57502=ORIENTED_EDGE('',*,*,#43447,.T.) ;
#57503=ORIENTED_EDGE('',*,*,#43448,.T.) ;
#57504=ORIENTED_EDGE('',*,*,#43449,.T.) ;
#57505=ORIENTED_EDGE('',*,*,#43450,.T.) ;
#57506=ORIENTED_EDGE('',*,*,#43451,.T.) ;
#57507=ORIENTED_EDGE('',*,*,#43452,.T.) ;
#57508=ORIENTED_EDGE('',*,*,#43453,.T.) ;
#57509=ORIENTED_EDGE('',*,*,#43454,.T.) ;
#57510=ORIENTED_EDGE('',*,*,#42608,.T.) ;
#57511=ORIENTED_EDGE('',*,*,#42636,.T.) ;
#57512=ORIENTED_EDGE('',*,*,#43455,.T.) ;
#57513=ORIENTED_EDGE('',*,*,#43456,.T.) ;
#57514=ORIENTED_EDGE('',*,*,#43457,.T.) ;
#57515=ORIENTED_EDGE('',*,*,#43458,.T.) ;
#57516=ORIENTED_EDGE('',*,*,#43459,.T.) ;
#57517=ORIENTED_EDGE('',*,*,#43460,.T.) ;
#57518=ORIENTED_EDGE('',*,*,#43461,.F.) ;
#57519=ORIENTED_EDGE('',*,*,#43462,.F.) ;
#57520=ORIENTED_EDGE('',*,*,#43463,.F.) ;
#57521=ORIENTED_EDGE('',*,*,#42839,.F.) ;
#57522=ORIENTED_EDGE('',*,*,#43313,.F.) ;
#57523=ORIENTED_EDGE('',*,*,#43302,.F.) ;
#57524=ORIENTED_EDGE('',*,*,#43464,.F.) ;
#57525=ORIENTED_EDGE('',*,*,#43323,.F.) ;
#57526=ORIENTED_EDGE('',*,*,#43464,.T.) ;
#57527=ORIENTED_EDGE('',*,*,#43301,.T.) ;
#57528=ORIENTED_EDGE('',*,*,#43465,.F.) ;
#57529=ORIENTED_EDGE('',*,*,#43466,.F.) ;
#57530=ORIENTED_EDGE('',*,*,#43465,.T.) ;
#57531=ORIENTED_EDGE('',*,*,#43308,.F.) ;
#57532=ORIENTED_EDGE('',*,*,#43467,.F.) ;
#57533=ORIENTED_EDGE('',*,*,#43339,.F.) ;
#57534=ORIENTED_EDGE('',*,*,#43462,.T.) ;
#57535=ORIENTED_EDGE('',*,*,#43340,.F.) ;
#57536=ORIENTED_EDGE('',*,*,#43468,.F.) ;
#57537=ORIENTED_EDGE('',*,*,#43299,.F.) ;
#57538=ORIENTED_EDGE('',*,*,#43463,.T.) ;
#57539=ORIENTED_EDGE('',*,*,#43298,.F.) ;
#57540=ORIENTED_EDGE('',*,*,#43469,.F.) ;
#57541=ORIENTED_EDGE('',*,*,#42840,.F.) ;
#57542=ORIENTED_EDGE('',*,*,#43461,.T.) ;
#57543=ORIENTED_EDGE('',*,*,#42838,.F.) ;
#57544=ORIENTED_EDGE('',*,*,#43470,.F.) ;
#57545=ORIENTED_EDGE('',*,*,#43335,.F.) ;
#57546=ORIENTED_EDGE('',*,*,#43466,.T.) ;
#57547=ORIENTED_EDGE('',*,*,#43338,.F.) ;
#57548=ORIENTED_EDGE('',*,*,#43471,.F.) ;
#57549=ORIENTED_EDGE('',*,*,#43324,.F.) ;
#57550=ORIENTED_EDGE('',*,*,#43315,.F.) ;
#57551=ORIENTED_EDGE('',*,*,#43325,.F.) ;
#57552=ORIENTED_EDGE('',*,*,#43472,.F.) ;
#57553=ORIENTED_EDGE('',*,*,#43318,.F.) ;
#57554=ORIENTED_EDGE('',*,*,#43468,.T.) ;
#57555=ORIENTED_EDGE('',*,*,#43467,.T.) ;
#57556=ORIENTED_EDGE('',*,*,#43473,.F.) ;
#57557=ORIENTED_EDGE('',*,*,#42841,.T.) ;
#57558=ORIENTED_EDGE('',*,*,#43469,.T.) ;
#57559=ORIENTED_EDGE('',*,*,#43474,.F.) ;
#57560=ORIENTED_EDGE('',*,*,#43475,.F.) ;
#57561=ORIENTED_EDGE('',*,*,#43470,.T.) ;
#57562=ORIENTED_EDGE('',*,*,#42845,.F.) ;
#57563=ORIENTED_EDGE('',*,*,#43476,.F.) ;
#57564=ORIENTED_EDGE('',*,*,#43477,.F.) ;
#57565=ORIENTED_EDGE('',*,*,#43472,.T.) ;
#57566=ORIENTED_EDGE('',*,*,#43471,.T.) ;
#57567=ORIENTED_EDGE('',*,*,#43478,.F.) ;
#57568=ORIENTED_EDGE('',*,*,#43319,.T.) ;
#57569=ORIENTED_EDGE('',*,*,#43473,.T.) ;
#57570=ORIENTED_EDGE('',*,*,#43307,.F.) ;
#57571=ORIENTED_EDGE('',*,*,#43479,.F.) ;
#57572=ORIENTED_EDGE('',*,*,#43300,.F.) ;
#57573=ORIENTED_EDGE('',*,*,#43474,.T.) ;
#57574=ORIENTED_EDGE('',*,*,#43297,.F.) ;
#57575=ORIENTED_EDGE('',*,*,#43480,.F.) ;
#57576=ORIENTED_EDGE('',*,*,#43333,.F.) ;
#57577=ORIENTED_EDGE('',*,*,#43475,.T.) ;
#57578=ORIENTED_EDGE('',*,*,#43332,.F.) ;
#57579=ORIENTED_EDGE('',*,*,#43481,.F.) ;
#57580=ORIENTED_EDGE('',*,*,#42842,.F.) ;
#57581=ORIENTED_EDGE('',*,*,#43476,.T.) ;
#57582=ORIENTED_EDGE('',*,*,#42844,.F.) ;
#57583=ORIENTED_EDGE('',*,*,#43482,.F.) ;
#57584=ORIENTED_EDGE('',*,*,#43294,.F.) ;
#57585=ORIENTED_EDGE('',*,*,#43477,.T.) ;
#57586=ORIENTED_EDGE('',*,*,#43293,.F.) ;
#57587=ORIENTED_EDGE('',*,*,#43483,.F.) ;
#57588=ORIENTED_EDGE('',*,*,#43336,.F.) ;
#57589=ORIENTED_EDGE('',*,*,#43478,.T.) ;
#57590=ORIENTED_EDGE('',*,*,#43337,.F.) ;
#57591=ORIENTED_EDGE('',*,*,#43484,.F.) ;
#57592=ORIENTED_EDGE('',*,*,#43320,.F.) ;
#57593=ORIENTED_EDGE('',*,*,#43480,.T.) ;
#57594=ORIENTED_EDGE('',*,*,#43479,.T.) ;
#57595=ORIENTED_EDGE('',*,*,#43485,.F.) ;
#57596=ORIENTED_EDGE('',*,*,#42843,.T.) ;
#57597=ORIENTED_EDGE('',*,*,#43481,.T.) ;
#57598=ORIENTED_EDGE('',*,*,#43486,.F.) ;
#57599=ORIENTED_EDGE('',*,*,#43482,.T.) ;
#57600=ORIENTED_EDGE('',*,*,#43484,.T.) ;
#57601=ORIENTED_EDGE('',*,*,#43483,.T.) ;
#57602=ORIENTED_EDGE('',*,*,#43487,.F.) ;
#57603=ORIENTED_EDGE('',*,*,#43312,.F.) ;
#57604=ORIENTED_EDGE('',*,*,#43328,.F.) ;
#57605=ORIENTED_EDGE('',*,*,#43488,.F.) ;
#57606=ORIENTED_EDGE('',*,*,#43304,.F.) ;
#57607=ORIENTED_EDGE('',*,*,#43485,.T.) ;
#57608=ORIENTED_EDGE('',*,*,#43306,.F.) ;
#57609=ORIENTED_EDGE('',*,*,#43489,.F.) ;
#57610=ORIENTED_EDGE('',*,*,#43334,.F.) ;
#57611=ORIENTED_EDGE('',*,*,#43486,.T.) ;
#57612=ORIENTED_EDGE('',*,*,#43331,.F.) ;
#57613=ORIENTED_EDGE('',*,*,#43490,.F.) ;
#57614=ORIENTED_EDGE('',*,*,#43295,.F.) ;
#57615=ORIENTED_EDGE('',*,*,#43487,.T.) ;
#57616=ORIENTED_EDGE('',*,*,#43296,.F.) ;
#57617=ORIENTED_EDGE('',*,*,#43491,.F.) ;
#57618=ORIENTED_EDGE('',*,*,#43321,.F.) ;
#57619=ORIENTED_EDGE('',*,*,#43305,.T.) ;
#57620=ORIENTED_EDGE('',*,*,#43488,.T.) ;
#57621=ORIENTED_EDGE('',*,*,#43492,.F.) ;
#57622=ORIENTED_EDGE('',*,*,#43489,.T.) ;
#57623=ORIENTED_EDGE('',*,*,#43491,.T.) ;
#57624=ORIENTED_EDGE('',*,*,#43490,.T.) ;
#57625=ORIENTED_EDGE('',*,*,#43493,.F.) ;
#57626=ORIENTED_EDGE('',*,*,#43492,.T.) ;
#57627=ORIENTED_EDGE('',*,*,#43327,.F.) ;
#57628=ORIENTED_EDGE('',*,*,#43494,.F.) ;
#57629=ORIENTED_EDGE('',*,*,#43329,.F.) ;
#57630=ORIENTED_EDGE('',*,*,#43493,.T.) ;
#57631=ORIENTED_EDGE('',*,*,#43330,.F.) ;
#57632=ORIENTED_EDGE('',*,*,#43495,.F.) ;
#57633=ORIENTED_EDGE('',*,*,#43322,.F.) ;
#57634=ORIENTED_EDGE('',*,*,#43495,.T.) ;
#57635=ORIENTED_EDGE('',*,*,#43494,.T.) ;
#57636=ORIENTED_EDGE('',*,*,#43496,.F.) ;
#57637=ORIENTED_EDGE('',*,*,#43316,.T.) ;
#57638=ORIENTED_EDGE('',*,*,#43310,.F.) ;
#57639=ORIENTED_EDGE('',*,*,#43317,.F.) ;
#57640=ORIENTED_EDGE('',*,*,#43496,.T.) ;
#57641=ORIENTED_EDGE('',*,*,#43326,.F.) ;
#57642=ORIENTED_EDGE('',*,*,#42783,.F.) ;
#57643=ORIENTED_EDGE('',*,*,#43497,.T.) ;
#57644=ORIENTED_EDGE('',*,*,#43498,.T.) ;
#57645=ORIENTED_EDGE('',*,*,#42610,.T.) ;
#57646=ORIENTED_EDGE('',*,*,#43440,.F.) ;
#57647=ORIENTED_EDGE('',*,*,#42635,.T.) ;
#57648=ORIENTED_EDGE('',*,*,#43442,.F.) ;
#57649=ORIENTED_EDGE('',*,*,#43499,.T.) ;
#57650=ORIENTED_EDGE('',*,*,#43446,.F.) ;
#57651=ORIENTED_EDGE('',*,*,#43500,.F.) ;
#57652=ORIENTED_EDGE('',*,*,#42633,.T.) ;
#57653=ORIENTED_EDGE('',*,*,#43443,.F.) ;
#57654=ORIENTED_EDGE('',*,*,#43501,.F.) ;
#57655=ORIENTED_EDGE('',*,*,#42761,.F.) ;
#57656=ORIENTED_EDGE('',*,*,#42789,.F.) ;
#57657=ORIENTED_EDGE('',*,*,#43502,.T.) ;
#57658=ORIENTED_EDGE('',*,*,#43450,.F.) ;
#57659=ORIENTED_EDGE('',*,*,#43503,.T.) ;
#57660=ORIENTED_EDGE('',*,*,#43453,.F.) ;
#57661=ORIENTED_EDGE('',*,*,#43504,.T.) ;
#57662=ORIENTED_EDGE('',*,*,#43444,.F.) ;
#57663=ORIENTED_EDGE('',*,*,#43505,.T.) ;
#57664=ORIENTED_EDGE('',*,*,#43501,.T.) ;
#57665=ORIENTED_EDGE('',*,*,#43500,.T.) ;
#57666=ORIENTED_EDGE('',*,*,#43506,.F.) ;
#57667=ORIENTED_EDGE('',*,*,#42762,.T.) ;
#57668=ORIENTED_EDGE('',*,*,#43291,.F.) ;
#57669=ORIENTED_EDGE('',*,*,#42765,.F.) ;
#57670=ORIENTED_EDGE('',*,*,#42628,.F.) ;
#57671=ORIENTED_EDGE('',*,*,#43283,.F.) ;
#57672=ORIENTED_EDGE('',*,*,#43507,.T.) ;
#57673=ORIENTED_EDGE('',*,*,#43508,.T.) ;
#57674=ORIENTED_EDGE('',*,*,#43280,.F.) ;
#57675=ORIENTED_EDGE('',*,*,#42627,.F.) ;
#57676=ORIENTED_EDGE('',*,*,#43448,.F.) ;
#57677=ORIENTED_EDGE('',*,*,#43509,.T.) ;
#57678=ORIENTED_EDGE('',*,*,#43506,.T.) ;
#57679=ORIENTED_EDGE('',*,*,#43445,.F.) ;
#57680=ORIENTED_EDGE('',*,*,#42626,.F.) ;
#57681=ORIENTED_EDGE('',*,*,#42763,.F.) ;
#57682=ORIENTED_EDGE('',*,*,#42629,.T.) ;
#57683=ORIENTED_EDGE('',*,*,#42764,.F.) ;
#57684=ORIENTED_EDGE('',*,*,#42624,.T.) ;
#57685=ORIENTED_EDGE('',*,*,#43449,.F.) ;
#57686=ORIENTED_EDGE('',*,*,#43510,.F.) ;
#57687=ORIENTED_EDGE('',*,*,#43425,.F.) ;
#57688=ORIENTED_EDGE('',*,*,#43511,.F.) ;
#57689=ORIENTED_EDGE('',*,*,#43511,.T.) ;
#57690=ORIENTED_EDGE('',*,*,#43423,.F.) ;
#57691=ORIENTED_EDGE('',*,*,#43512,.F.) ;
#57692=ORIENTED_EDGE('',*,*,#43436,.F.) ;
#57693=ORIENTED_EDGE('',*,*,#43510,.T.) ;
#57694=ORIENTED_EDGE('',*,*,#43439,.F.) ;
#57695=ORIENTED_EDGE('',*,*,#43513,.F.) ;
#57696=ORIENTED_EDGE('',*,*,#43427,.F.) ;
#57697=ORIENTED_EDGE('',*,*,#43512,.T.) ;
#57698=ORIENTED_EDGE('',*,*,#43421,.F.) ;
#57699=ORIENTED_EDGE('',*,*,#43514,.F.) ;
#57700=ORIENTED_EDGE('',*,*,#43429,.F.) ;
#57701=ORIENTED_EDGE('',*,*,#43513,.T.) ;
#57702=ORIENTED_EDGE('',*,*,#43515,.F.) ;
#57703=ORIENTED_EDGE('',*,*,#43514,.T.) ;
#57704=ORIENTED_EDGE('',*,*,#43435,.F.) ;
#57705=ORIENTED_EDGE('',*,*,#43516,.F.) ;
#57706=ORIENTED_EDGE('',*,*,#43437,.F.) ;
#57707=ORIENTED_EDGE('',*,*,#43515,.T.) ;
#57708=ORIENTED_EDGE('',*,*,#43438,.F.) ;
#57709=ORIENTED_EDGE('',*,*,#43517,.F.) ;
#57710=ORIENTED_EDGE('',*,*,#43431,.F.) ;
#57711=ORIENTED_EDGE('',*,*,#43516,.T.) ;
#57712=ORIENTED_EDGE('',*,*,#43433,.F.) ;
#57713=ORIENTED_EDGE('',*,*,#43517,.T.) ;
#57714=ORIENTED_EDGE('',*,*,#43518,.F.) ;
#57715=ORIENTED_EDGE('',*,*,#42863,.F.) ;
#57716=ORIENTED_EDGE('',*,*,#43519,.F.) ;
#57717=ORIENTED_EDGE('',*,*,#43344,.F.) ;
#57718=ORIENTED_EDGE('',*,*,#43519,.T.) ;
#57719=ORIENTED_EDGE('',*,*,#42862,.T.) ;
#57720=ORIENTED_EDGE('',*,*,#43520,.F.) ;
#57721=ORIENTED_EDGE('',*,*,#43521,.F.) ;
#57722=ORIENTED_EDGE('',*,*,#42864,.T.) ;
#57723=ORIENTED_EDGE('',*,*,#43518,.T.) ;
#57724=ORIENTED_EDGE('',*,*,#43522,.F.) ;
#57725=ORIENTED_EDGE('',*,*,#43523,.F.) ;
#57726=ORIENTED_EDGE('',*,*,#43520,.T.) ;
#57727=ORIENTED_EDGE('',*,*,#42861,.F.) ;
#57728=ORIENTED_EDGE('',*,*,#43524,.F.) ;
#57729=ORIENTED_EDGE('',*,*,#43356,.F.) ;
#57730=ORIENTED_EDGE('',*,*,#43521,.T.) ;
#57731=ORIENTED_EDGE('',*,*,#43355,.F.) ;
#57732=ORIENTED_EDGE('',*,*,#43525,.F.) ;
#57733=ORIENTED_EDGE('',*,*,#43341,.F.) ;
#57734=ORIENTED_EDGE('',*,*,#43526,.F.) ;
#57735=ORIENTED_EDGE('',*,*,#43342,.F.) ;
#57736=ORIENTED_EDGE('',*,*,#43527,.F.) ;
#57737=ORIENTED_EDGE('',*,*,#43360,.F.) ;
#57738=ORIENTED_EDGE('',*,*,#43522,.T.) ;
#57739=ORIENTED_EDGE('',*,*,#43343,.F.) ;
#57740=ORIENTED_EDGE('',*,*,#43528,.F.) ;
#57741=ORIENTED_EDGE('',*,*,#43348,.F.) ;
#57742=ORIENTED_EDGE('',*,*,#43523,.T.) ;
#57743=ORIENTED_EDGE('',*,*,#43347,.F.) ;
#57744=ORIENTED_EDGE('',*,*,#43529,.F.) ;
#57745=ORIENTED_EDGE('',*,*,#42865,.F.) ;
#57746=ORIENTED_EDGE('',*,*,#43530,.F.) ;
#57747=ORIENTED_EDGE('',*,*,#42859,.F.) ;
#57748=ORIENTED_EDGE('',*,*,#43531,.F.) ;
#57749=ORIENTED_EDGE('',*,*,#43351,.F.) ;
#57750=ORIENTED_EDGE('',*,*,#42860,.T.) ;
#57751=ORIENTED_EDGE('',*,*,#43530,.T.) ;
#57752=ORIENTED_EDGE('',*,*,#43532,.F.) ;
#57753=ORIENTED_EDGE('',*,*,#43524,.T.) ;
#57754=ORIENTED_EDGE('',*,*,#43527,.T.) ;
#57755=ORIENTED_EDGE('',*,*,#43525,.T.) ;
#57756=ORIENTED_EDGE('',*,*,#43533,.F.) ;
#57757=ORIENTED_EDGE('',*,*,#43528,.T.) ;
#57758=ORIENTED_EDGE('',*,*,#43526,.T.) ;
#57759=ORIENTED_EDGE('',*,*,#43534,.F.) ;
#57760=ORIENTED_EDGE('',*,*,#42858,.T.) ;
#57761=ORIENTED_EDGE('',*,*,#43529,.T.) ;
#57762=ORIENTED_EDGE('',*,*,#43535,.F.) ;
#57763=ORIENTED_EDGE('',*,*,#43531,.T.) ;
#57764=ORIENTED_EDGE('',*,*,#43532,.T.) ;
#57765=ORIENTED_EDGE('',*,*,#43350,.F.) ;
#57766=ORIENTED_EDGE('',*,*,#43536,.F.) ;
#57767=ORIENTED_EDGE('',*,*,#43353,.F.) ;
#57768=ORIENTED_EDGE('',*,*,#43533,.T.) ;
#57769=ORIENTED_EDGE('',*,*,#43354,.F.) ;
#57770=ORIENTED_EDGE('',*,*,#43537,.F.) ;
#57771=ORIENTED_EDGE('',*,*,#43357,.F.) ;
#57772=ORIENTED_EDGE('',*,*,#43534,.T.) ;
#57773=ORIENTED_EDGE('',*,*,#43359,.F.) ;
#57774=ORIENTED_EDGE('',*,*,#43538,.F.) ;
#57775=ORIENTED_EDGE('',*,*,#43345,.F.) ;
#57776=ORIENTED_EDGE('',*,*,#43535,.T.) ;
#57777=ORIENTED_EDGE('',*,*,#43346,.F.) ;
#57778=ORIENTED_EDGE('',*,*,#43539,.F.) ;
#57779=ORIENTED_EDGE('',*,*,#43352,.F.) ;
#57780=ORIENTED_EDGE('',*,*,#43537,.T.) ;
#57781=ORIENTED_EDGE('',*,*,#43536,.T.) ;
#57782=ORIENTED_EDGE('',*,*,#43540,.F.) ;
#57783=ORIENTED_EDGE('',*,*,#43539,.T.) ;
#57784=ORIENTED_EDGE('',*,*,#43538,.T.) ;
#57785=ORIENTED_EDGE('',*,*,#43541,.F.) ;
#57786=ORIENTED_EDGE('',*,*,#43540,.T.) ;
#57787=ORIENTED_EDGE('',*,*,#43349,.F.) ;
#57788=ORIENTED_EDGE('',*,*,#43541,.T.) ;
#57789=ORIENTED_EDGE('',*,*,#43358,.F.) ;
#57790=ORIENTED_EDGE('',*,*,#43542,.F.) ;
#57791=ORIENTED_EDGE('',*,*,#42813,.F.) ;
#57792=ORIENTED_EDGE('',*,*,#43543,.F.) ;
#57793=ORIENTED_EDGE('',*,*,#43403,.F.) ;
#57794=ORIENTED_EDGE('',*,*,#43543,.T.) ;
#57795=ORIENTED_EDGE('',*,*,#42812,.T.) ;
#57796=ORIENTED_EDGE('',*,*,#43544,.F.) ;
#57797=ORIENTED_EDGE('',*,*,#43545,.F.) ;
#57798=ORIENTED_EDGE('',*,*,#42814,.T.) ;
#57799=ORIENTED_EDGE('',*,*,#43542,.T.) ;
#57800=ORIENTED_EDGE('',*,*,#43546,.F.) ;
#57801=ORIENTED_EDGE('',*,*,#43547,.F.) ;
#57802=ORIENTED_EDGE('',*,*,#43544,.T.) ;
#57803=ORIENTED_EDGE('',*,*,#42811,.F.) ;
#57804=ORIENTED_EDGE('',*,*,#43548,.F.) ;
#57805=ORIENTED_EDGE('',*,*,#43399,.F.) ;
#57806=ORIENTED_EDGE('',*,*,#43545,.T.) ;
#57807=ORIENTED_EDGE('',*,*,#43398,.F.) ;
#57808=ORIENTED_EDGE('',*,*,#43549,.F.) ;
#57809=ORIENTED_EDGE('',*,*,#43400,.F.) ;
#57810=ORIENTED_EDGE('',*,*,#43550,.F.) ;
#57811=ORIENTED_EDGE('',*,*,#43401,.F.) ;
#57812=ORIENTED_EDGE('',*,*,#43551,.F.) ;
#57813=ORIENTED_EDGE('',*,*,#43411,.F.) ;
#57814=ORIENTED_EDGE('',*,*,#43546,.T.) ;
#57815=ORIENTED_EDGE('',*,*,#43402,.F.) ;
#57816=ORIENTED_EDGE('',*,*,#43552,.F.) ;
#57817=ORIENTED_EDGE('',*,*,#43407,.F.) ;
#57818=ORIENTED_EDGE('',*,*,#43547,.T.) ;
#57819=ORIENTED_EDGE('',*,*,#43406,.F.) ;
#57820=ORIENTED_EDGE('',*,*,#43553,.F.) ;
#57821=ORIENTED_EDGE('',*,*,#42815,.F.) ;
#57822=ORIENTED_EDGE('',*,*,#43554,.F.) ;
#57823=ORIENTED_EDGE('',*,*,#42809,.F.) ;
#57824=ORIENTED_EDGE('',*,*,#43555,.F.) ;
#57825=ORIENTED_EDGE('',*,*,#43394,.F.) ;
#57826=ORIENTED_EDGE('',*,*,#42810,.T.) ;
#57827=ORIENTED_EDGE('',*,*,#43554,.T.) ;
#57828=ORIENTED_EDGE('',*,*,#43556,.F.) ;
#57829=ORIENTED_EDGE('',*,*,#43548,.T.) ;
#57830=ORIENTED_EDGE('',*,*,#43551,.T.) ;
#57831=ORIENTED_EDGE('',*,*,#43549,.T.) ;
#57832=ORIENTED_EDGE('',*,*,#43557,.F.) ;
#57833=ORIENTED_EDGE('',*,*,#43552,.T.) ;
#57834=ORIENTED_EDGE('',*,*,#43550,.T.) ;
#57835=ORIENTED_EDGE('',*,*,#43558,.F.) ;
#57836=ORIENTED_EDGE('',*,*,#42808,.T.) ;
#57837=ORIENTED_EDGE('',*,*,#43553,.T.) ;
#57838=ORIENTED_EDGE('',*,*,#43559,.F.) ;
#57839=ORIENTED_EDGE('',*,*,#43555,.T.) ;
#57840=ORIENTED_EDGE('',*,*,#43556,.T.) ;
#57841=ORIENTED_EDGE('',*,*,#43393,.F.) ;
#57842=ORIENTED_EDGE('',*,*,#43560,.F.) ;
#57843=ORIENTED_EDGE('',*,*,#43396,.F.) ;
#57844=ORIENTED_EDGE('',*,*,#43557,.T.) ;
#57845=ORIENTED_EDGE('',*,*,#43397,.F.) ;
#57846=ORIENTED_EDGE('',*,*,#43561,.F.) ;
#57847=ORIENTED_EDGE('',*,*,#43408,.F.) ;
#57848=ORIENTED_EDGE('',*,*,#43558,.T.) ;
#57849=ORIENTED_EDGE('',*,*,#43410,.F.) ;
#57850=ORIENTED_EDGE('',*,*,#43562,.F.) ;
#57851=ORIENTED_EDGE('',*,*,#43404,.F.) ;
#57852=ORIENTED_EDGE('',*,*,#43559,.T.) ;
#57853=ORIENTED_EDGE('',*,*,#43405,.F.) ;
#57854=ORIENTED_EDGE('',*,*,#43563,.F.) ;
#57855=ORIENTED_EDGE('',*,*,#43395,.F.) ;
#57856=ORIENTED_EDGE('',*,*,#43561,.T.) ;
#57857=ORIENTED_EDGE('',*,*,#43560,.T.) ;
#57858=ORIENTED_EDGE('',*,*,#43564,.F.) ;
#57859=ORIENTED_EDGE('',*,*,#43563,.T.) ;
#57860=ORIENTED_EDGE('',*,*,#43562,.T.) ;
#57861=ORIENTED_EDGE('',*,*,#43565,.F.) ;
#57862=ORIENTED_EDGE('',*,*,#43564,.T.) ;
#57863=ORIENTED_EDGE('',*,*,#43392,.F.) ;
#57864=ORIENTED_EDGE('',*,*,#43565,.T.) ;
#57865=ORIENTED_EDGE('',*,*,#43409,.F.) ;
#57866=ORIENTED_EDGE('',*,*,#43286,.F.) ;
#57867=ORIENTED_EDGE('',*,*,#43566,.T.) ;
#57868=ORIENTED_EDGE('',*,*,#43455,.F.) ;
#57869=ORIENTED_EDGE('',*,*,#43567,.F.) ;
#57870=ORIENTED_EDGE('',*,*,#43289,.F.) ;
#57871=ORIENTED_EDGE('',*,*,#43287,.F.) ;
#57872=ORIENTED_EDGE('',*,*,#43568,.F.) ;
#57873=ORIENTED_EDGE('',*,*,#43276,.F.) ;
#57874=ORIENTED_EDGE('',*,*,#43568,.T.) ;
#57875=ORIENTED_EDGE('',*,*,#43567,.T.) ;
#57876=ORIENTED_EDGE('',*,*,#43569,.F.) ;
#57877=ORIENTED_EDGE('',*,*,#43569,.T.) ;
#57878=ORIENTED_EDGE('',*,*,#43460,.F.) ;
#57879=ORIENTED_EDGE('',*,*,#43570,.F.) ;
#57880=ORIENTED_EDGE('',*,*,#43277,.F.) ;
#57881=ORIENTED_EDGE('',*,*,#43290,.F.) ;
#57882=ORIENTED_EDGE('',*,*,#43278,.F.) ;
#57883=ORIENTED_EDGE('',*,*,#43571,.F.) ;
#57884=ORIENTED_EDGE('',*,*,#42767,.F.) ;
#57885=ORIENTED_EDGE('',*,*,#43571,.T.) ;
#57886=ORIENTED_EDGE('',*,*,#43570,.T.) ;
#57887=ORIENTED_EDGE('',*,*,#43572,.F.) ;
#57888=ORIENTED_EDGE('',*,*,#42768,.T.) ;
#57889=ORIENTED_EDGE('',*,*,#43572,.T.) ;
#57890=ORIENTED_EDGE('',*,*,#43459,.F.) ;
#57891=ORIENTED_EDGE('',*,*,#43573,.F.) ;
#57892=ORIENTED_EDGE('',*,*,#42769,.F.) ;
#57893=ORIENTED_EDGE('',*,*,#42770,.T.) ;
#57894=ORIENTED_EDGE('',*,*,#43573,.T.) ;
#57895=ORIENTED_EDGE('',*,*,#43574,.F.) ;
#57896=ORIENTED_EDGE('',*,*,#43193,.T.) ;
#57897=ORIENTED_EDGE('',*,*,#43574,.T.) ;
#57898=ORIENTED_EDGE('',*,*,#43458,.F.) ;
#57899=ORIENTED_EDGE('',*,*,#43575,.F.) ;
#57900=ORIENTED_EDGE('',*,*,#42751,.F.) ;
#57901=ORIENTED_EDGE('',*,*,#43189,.T.) ;
#57902=ORIENTED_EDGE('',*,*,#43575,.T.) ;
#57903=ORIENTED_EDGE('',*,*,#43576,.F.) ;
#57904=ORIENTED_EDGE('',*,*,#43457,.F.) ;
#57905=ORIENTED_EDGE('',*,*,#43577,.T.) ;
#57906=ORIENTED_EDGE('',*,*,#42893,.F.) ;
#57907=ORIENTED_EDGE('',*,*,#43576,.T.) ;
#57908=ORIENTED_EDGE('',*,*,#42642,.F.) ;
#57909=ORIENTED_EDGE('',*,*,#43388,.F.) ;
#57910=ORIENTED_EDGE('',*,*,#42652,.F.) ;
#57911=ORIENTED_EDGE('',*,*,#43390,.F.) ;
#57912=ORIENTED_EDGE('',*,*,#42650,.F.) ;
#57913=ORIENTED_EDGE('',*,*,#43386,.F.) ;
#57914=ORIENTED_EDGE('',*,*,#42644,.F.) ;
#57915=ORIENTED_EDGE('',*,*,#43391,.F.) ;
#57916=ORIENTED_EDGE('',*,*,#42640,.F.) ;
#57917=ORIENTED_EDGE('',*,*,#43279,.F.) ;
#57918=ORIENTED_EDGE('',*,*,#42654,.F.) ;
#57919=ORIENTED_EDGE('',*,*,#43389,.F.) ;
#57920=ORIENTED_EDGE('',*,*,#42648,.F.) ;
#57921=ORIENTED_EDGE('',*,*,#43385,.F.) ;
#57922=ORIENTED_EDGE('',*,*,#42646,.F.) ;
#57923=ORIENTED_EDGE('',*,*,#43387,.F.) ;
#57924=ORIENTED_EDGE('',*,*,#43578,.F.) ;
#57925=ORIENTED_EDGE('',*,*,#42631,.F.) ;
#57926=ORIENTED_EDGE('',*,*,#43504,.F.) ;
#57927=ORIENTED_EDGE('',*,*,#43578,.T.) ;
#57928=ORIENTED_EDGE('',*,*,#43452,.F.) ;
#57929=ORIENTED_EDGE('',*,*,#43579,.F.) ;
#57930=ORIENTED_EDGE('',*,*,#43447,.F.) ;
#57931=ORIENTED_EDGE('',*,*,#43579,.T.) ;
#57932=ORIENTED_EDGE('',*,*,#43451,.F.) ;
#57933=ORIENTED_EDGE('',*,*,#43580,.F.) ;
#57934=ORIENTED_EDGE('',*,*,#43509,.F.) ;
#57935=ORIENTED_EDGE('',*,*,#43580,.T.) ;
#57936=ORIENTED_EDGE('',*,*,#43502,.F.) ;
#57937=ORIENTED_EDGE('',*,*,#43581,.F.) ;
#57938=ORIENTED_EDGE('',*,*,#43507,.F.) ;
#57939=ORIENTED_EDGE('',*,*,#43581,.T.) ;
#57940=ORIENTED_EDGE('',*,*,#42788,.F.) ;
#57941=ORIENTED_EDGE('',*,*,#43582,.F.) ;
#57942=ORIENTED_EDGE('',*,*,#43508,.F.) ;
#57943=ORIENTED_EDGE('',*,*,#43582,.T.) ;
#57944=ORIENTED_EDGE('',*,*,#42787,.F.) ;
#57945=ORIENTED_EDGE('',*,*,#43292,.F.) ;
#57946=ORIENTED_EDGE('',*,*,#43281,.F.) ;
#57947=ORIENTED_EDGE('',*,*,#43217,.T.) ;
#57948=ORIENTED_EDGE('',*,*,#42790,.F.) ;
#57949=ORIENTED_EDGE('',*,*,#43583,.F.) ;
#57950=ORIENTED_EDGE('',*,*,#43497,.F.) ;
#57951=ORIENTED_EDGE('',*,*,#43583,.T.) ;
#57952=ORIENTED_EDGE('',*,*,#43503,.F.) ;
#57953=ORIENTED_EDGE('',*,*,#42611,.F.) ;
#57954=ORIENTED_EDGE('',*,*,#43498,.F.) ;
#57955=ORIENTED_EDGE('',*,*,#43584,.F.) ;
#57956=ORIENTED_EDGE('',*,*,#43441,.F.) ;
#57957=ORIENTED_EDGE('',*,*,#42609,.T.) ;
#57958=ORIENTED_EDGE('',*,*,#43454,.F.) ;
#57959=ORIENTED_EDGE('',*,*,#43505,.F.) ;
#57960=ORIENTED_EDGE('',*,*,#43499,.F.) ;
#57961=ORIENTED_EDGE('',*,*,#43584,.T.) ;
#57962=ORIENTED_EDGE('',*,*,#43585,.T.) ;
#57963=ORIENTED_EDGE('',*,*,#43586,.T.) ;
#57964=ORIENTED_EDGE('',*,*,#43456,.F.) ;
#57965=ORIENTED_EDGE('',*,*,#43587,.T.) ;
#57966=ORIENTED_EDGE('',*,*,#43588,.T.) ;
#57967=ORIENTED_EDGE('',*,*,#43288,.F.) ;
#57968=ORIENTED_EDGE('',*,*,#42887,.F.) ;
#57969=ORIENTED_EDGE('',*,*,#43589,.F.) ;
#57970=ORIENTED_EDGE('',*,*,#43285,.F.) ;
#57971=ORIENTED_EDGE('',*,*,#42886,.F.) ;
#57972=ORIENTED_EDGE('',*,*,#43590,.T.) ;
#57973=ORIENTED_EDGE('',*,*,#43566,.F.) ;
#57974=ORIENTED_EDGE('',*,*,#43589,.T.) ;
#57975=ORIENTED_EDGE('',*,*,#43577,.F.) ;
#57976=ORIENTED_EDGE('',*,*,#43591,.T.) ;
#57977=ORIENTED_EDGE('',*,*,#42883,.F.) ;
#57978=ORIENTED_EDGE('',*,*,#43225,.T.) ;
#57979=ORIENTED_EDGE('',*,*,#43587,.F.) ;
#57980=ORIENTED_EDGE('',*,*,#43590,.F.) ;
#57981=ORIENTED_EDGE('',*,*,#43592,.F.) ;
#57982=ORIENTED_EDGE('',*,*,#43593,.F.) ;
#57983=ORIENTED_EDGE('',*,*,#43588,.F.) ;
#57984=ORIENTED_EDGE('',*,*,#43592,.T.) ;
#57985=ORIENTED_EDGE('',*,*,#42885,.F.) ;
#57986=ORIENTED_EDGE('',*,*,#43593,.T.) ;
#57987=ORIENTED_EDGE('',*,*,#42884,.F.) ;
#57988=ORIENTED_EDGE('',*,*,#43594,.F.) ;
#57989=ORIENTED_EDGE('',*,*,#43585,.F.) ;
#57990=ORIENTED_EDGE('',*,*,#43594,.T.) ;
#57991=ORIENTED_EDGE('',*,*,#43591,.F.) ;
#57992=ORIENTED_EDGE('',*,*,#43586,.F.) ;
#57993=ORIENTED_EDGE('',*,*,#43595,.F.) ;
#57994=ORIENTED_EDGE('',*,*,#43245,.F.) ;
#57995=ORIENTED_EDGE('',*,*,#43596,.F.) ;
#57996=ORIENTED_EDGE('',*,*,#43597,.F.) ;
#57997=ORIENTED_EDGE('',*,*,#43243,.F.) ;
#57998=ORIENTED_EDGE('',*,*,#43598,.F.) ;
#57999=ORIENTED_EDGE('',*,*,#43596,.T.) ;
#58000=ORIENTED_EDGE('',*,*,#43248,.F.) ;
#58001=ORIENTED_EDGE('',*,*,#43599,.F.) ;
#58002=ORIENTED_EDGE('',*,*,#43266,.F.) ;
#58003=ORIENTED_EDGE('',*,*,#43595,.T.) ;
#58004=ORIENTED_EDGE('',*,*,#43265,.F.) ;
#58005=ORIENTED_EDGE('',*,*,#43600,.F.) ;
#58006=ORIENTED_EDGE('',*,*,#43242,.F.) ;
#58007=ORIENTED_EDGE('',*,*,#43598,.T.) ;
#58008=ORIENTED_EDGE('',*,*,#43240,.F.) ;
#58009=ORIENTED_EDGE('',*,*,#43601,.F.) ;
#58010=ORIENTED_EDGE('',*,*,#43268,.F.) ;
#58011=ORIENTED_EDGE('',*,*,#43597,.T.) ;
#58012=ORIENTED_EDGE('',*,*,#43274,.F.) ;
#58013=ORIENTED_EDGE('',*,*,#43602,.F.) ;
#58014=ORIENTED_EDGE('',*,*,#43246,.F.) ;
#58015=ORIENTED_EDGE('',*,*,#43599,.T.) ;
#58016=ORIENTED_EDGE('',*,*,#43251,.F.) ;
#58017=ORIENTED_EDGE('',*,*,#43603,.F.) ;
#58018=ORIENTED_EDGE('',*,*,#43239,.F.) ;
#58019=ORIENTED_EDGE('',*,*,#43600,.T.) ;
#58020=ORIENTED_EDGE('',*,*,#43604,.F.) ;
#58021=ORIENTED_EDGE('',*,*,#43601,.T.) ;
#58022=ORIENTED_EDGE('',*,*,#43237,.F.) ;
#58023=ORIENTED_EDGE('',*,*,#43605,.F.) ;
#58024=ORIENTED_EDGE('',*,*,#43249,.F.) ;
#58025=ORIENTED_EDGE('',*,*,#43602,.T.) ;
#58026=ORIENTED_EDGE('',*,*,#43606,.F.) ;
#58027=ORIENTED_EDGE('',*,*,#43603,.T.) ;
#58028=ORIENTED_EDGE('',*,*,#43254,.F.) ;
#58029=ORIENTED_EDGE('',*,*,#43607,.F.) ;
#58030=ORIENTED_EDGE('',*,*,#43267,.F.) ;
#58031=ORIENTED_EDGE('',*,*,#43604,.T.) ;
#58032=ORIENTED_EDGE('',*,*,#43264,.F.) ;
#58033=ORIENTED_EDGE('',*,*,#43608,.F.) ;
#58034=ORIENTED_EDGE('',*,*,#43236,.F.) ;
#58035=ORIENTED_EDGE('',*,*,#43609,.F.) ;
#58036=ORIENTED_EDGE('',*,*,#43233,.F.) ;
#58037=ORIENTED_EDGE('',*,*,#43610,.F.) ;
#58038=ORIENTED_EDGE('',*,*,#42717,.F.) ;
#58039=ORIENTED_EDGE('',*,*,#43605,.T.) ;
#58040=ORIENTED_EDGE('',*,*,#43234,.F.) ;
#58041=ORIENTED_EDGE('',*,*,#43611,.F.) ;
#58042=ORIENTED_EDGE('',*,*,#43269,.F.) ;
#58043=ORIENTED_EDGE('',*,*,#43606,.T.) ;
#58044=ORIENTED_EDGE('',*,*,#43273,.F.) ;
#58045=ORIENTED_EDGE('',*,*,#43612,.F.) ;
#58046=ORIENTED_EDGE('',*,*,#43252,.F.) ;
#58047=ORIENTED_EDGE('',*,*,#43607,.T.) ;
#58048=ORIENTED_EDGE('',*,*,#43257,.F.) ;
#58049=ORIENTED_EDGE('',*,*,#43613,.F.) ;
#58050=ORIENTED_EDGE('',*,*,#43261,.F.) ;
#58051=ORIENTED_EDGE('',*,*,#43610,.T.) ;
#58052=ORIENTED_EDGE('',*,*,#43608,.T.) ;
#58053=ORIENTED_EDGE('',*,*,#43614,.F.) ;
#58054=ORIENTED_EDGE('',*,*,#42718,.T.) ;
#58055=ORIENTED_EDGE('',*,*,#43609,.T.) ;
#58056=ORIENTED_EDGE('',*,*,#42716,.T.) ;
#58057=ORIENTED_EDGE('',*,*,#43615,.F.) ;
#58058=ORIENTED_EDGE('',*,*,#43611,.T.) ;
#58059=ORIENTED_EDGE('',*,*,#43612,.T.) ;
#58060=ORIENTED_EDGE('',*,*,#43272,.F.) ;
#58061=ORIENTED_EDGE('',*,*,#43616,.F.) ;
#58062=ORIENTED_EDGE('',*,*,#43255,.F.) ;
#58063=ORIENTED_EDGE('',*,*,#43613,.T.) ;
#58064=ORIENTED_EDGE('',*,*,#43260,.F.) ;
#58065=ORIENTED_EDGE('',*,*,#43617,.F.) ;
#58066=ORIENTED_EDGE('',*,*,#43262,.F.) ;
#58067=ORIENTED_EDGE('',*,*,#43614,.T.) ;
#58068=ORIENTED_EDGE('',*,*,#43263,.F.) ;
#58069=ORIENTED_EDGE('',*,*,#43618,.F.) ;
#58070=ORIENTED_EDGE('',*,*,#42719,.F.) ;
#58071=ORIENTED_EDGE('',*,*,#43615,.T.) ;
#58072=ORIENTED_EDGE('',*,*,#42715,.F.) ;
#58073=ORIENTED_EDGE('',*,*,#43619,.F.) ;
#58074=ORIENTED_EDGE('',*,*,#43270,.F.) ;
#58075=ORIENTED_EDGE('',*,*,#43616,.T.) ;
#58076=ORIENTED_EDGE('',*,*,#43271,.F.) ;
#58077=ORIENTED_EDGE('',*,*,#43620,.F.) ;
#58078=ORIENTED_EDGE('',*,*,#43258,.F.) ;
#58079=ORIENTED_EDGE('',*,*,#43618,.T.) ;
#58080=ORIENTED_EDGE('',*,*,#43617,.T.) ;
#58081=ORIENTED_EDGE('',*,*,#43621,.F.) ;
#58082=ORIENTED_EDGE('',*,*,#42720,.T.) ;
#58083=ORIENTED_EDGE('',*,*,#43619,.T.) ;
#58084=ORIENTED_EDGE('',*,*,#42714,.T.) ;
#58085=ORIENTED_EDGE('',*,*,#43622,.F.) ;
#58086=ORIENTED_EDGE('',*,*,#43620,.T.) ;
#58087=ORIENTED_EDGE('',*,*,#43621,.T.) ;
#58088=ORIENTED_EDGE('',*,*,#43259,.F.) ;
#58089=ORIENTED_EDGE('',*,*,#43622,.T.) ;
#58090=ORIENTED_EDGE('',*,*,#42721,.F.) ;
#58091=ORIENTED_EDGE('',*,*,#43623,.F.) ;
#58092=ORIENTED_EDGE('',*,*,#43624,.F.) ;
#58093=ORIENTED_EDGE('',*,*,#43625,.F.) ;
#58094=ORIENTED_EDGE('',*,*,#43626,.T.) ;
#58095=ORIENTED_EDGE('',*,*,#43627,.F.) ;
#58096=ORIENTED_EDGE('',*,*,#43628,.F.) ;
#58097=ORIENTED_EDGE('',*,*,#43629,.F.) ;
#58098=ORIENTED_EDGE('',*,*,#43630,.F.) ;
#58099=ORIENTED_EDGE('',*,*,#43631,.F.) ;
#58100=ORIENTED_EDGE('',*,*,#43632,.T.) ;
#58101=ORIENTED_EDGE('',*,*,#43633,.F.) ;
#58102=ORIENTED_EDGE('',*,*,#43634,.F.) ;
#58103=ORIENTED_EDGE('',*,*,#43632,.F.) ;
#58104=ORIENTED_EDGE('',*,*,#43635,.F.) ;
#58105=ORIENTED_EDGE('',*,*,#43636,.T.) ;
#58106=ORIENTED_EDGE('',*,*,#43637,.F.) ;
#58107=ORIENTED_EDGE('',*,*,#43636,.F.) ;
#58108=ORIENTED_EDGE('',*,*,#43638,.F.) ;
#58109=ORIENTED_EDGE('',*,*,#43639,.T.) ;
#58110=ORIENTED_EDGE('',*,*,#43640,.F.) ;
#58111=ORIENTED_EDGE('',*,*,#43641,.F.) ;
#58112=ORIENTED_EDGE('',*,*,#43639,.F.) ;
#58113=ORIENTED_EDGE('',*,*,#43642,.T.) ;
#58114=ORIENTED_EDGE('',*,*,#43643,.F.) ;
#58115=ORIENTED_EDGE('',*,*,#43644,.T.) ;
#58116=ORIENTED_EDGE('',*,*,#43645,.T.) ;
#58117=ORIENTED_EDGE('',*,*,#43646,.T.) ;
#58118=ORIENTED_EDGE('',*,*,#43647,.T.) ;
#58119=ORIENTED_EDGE('',*,*,#43648,.F.) ;
#58120=ORIENTED_EDGE('',*,*,#43642,.F.) ;
#58121=ORIENTED_EDGE('',*,*,#43649,.F.) ;
#58122=ORIENTED_EDGE('',*,*,#43650,.T.) ;
#58123=ORIENTED_EDGE('',*,*,#43651,.F.) ;
#58124=ORIENTED_EDGE('',*,*,#43652,.F.) ;
#58125=ORIENTED_EDGE('',*,*,#43653,.T.) ;
#58126=ORIENTED_EDGE('',*,*,#43654,.F.) ;
#58127=ORIENTED_EDGE('',*,*,#43655,.F.) ;
#58128=ORIENTED_EDGE('',*,*,#43656,.T.) ;
#58129=ORIENTED_EDGE('',*,*,#43635,.T.) ;
#58130=ORIENTED_EDGE('',*,*,#43656,.F.) ;
#58131=ORIENTED_EDGE('',*,*,#43637,.T.) ;
#58132=ORIENTED_EDGE('',*,*,#43657,.T.) ;
#58133=ORIENTED_EDGE('',*,*,#43640,.T.) ;
#58134=ORIENTED_EDGE('',*,*,#43641,.T.) ;
#58135=ORIENTED_EDGE('',*,*,#43657,.F.) ;
#58136=ORIENTED_EDGE('',*,*,#43658,.F.) ;
#58137=ORIENTED_EDGE('',*,*,#43659,.T.) ;
#58138=ORIENTED_EDGE('',*,*,#43660,.F.) ;
#58139=ORIENTED_EDGE('',*,*,#43661,.T.) ;
#58140=ORIENTED_EDGE('',*,*,#43662,.F.) ;
#58141=ORIENTED_EDGE('',*,*,#43663,.T.) ;
#58142=ORIENTED_EDGE('',*,*,#43664,.T.) ;
#58143=ORIENTED_EDGE('',*,*,#43665,.T.) ;
#58144=ORIENTED_EDGE('',*,*,#43666,.F.) ;
#58145=ORIENTED_EDGE('',*,*,#43667,.T.) ;
#58146=ORIENTED_EDGE('',*,*,#43668,.F.) ;
#58147=ORIENTED_EDGE('',*,*,#43669,.T.) ;
#58148=ORIENTED_EDGE('',*,*,#43670,.F.) ;
#58149=ORIENTED_EDGE('',*,*,#43671,.T.) ;
#58150=ORIENTED_EDGE('',*,*,#43672,.T.) ;
#58151=ORIENTED_EDGE('',*,*,#43673,.T.) ;
#58152=ORIENTED_EDGE('',*,*,#43674,.F.) ;
#58153=ORIENTED_EDGE('',*,*,#43675,.T.) ;
#58154=ORIENTED_EDGE('',*,*,#43633,.T.) ;
#58155=ORIENTED_EDGE('',*,*,#43634,.T.) ;
#58156=ORIENTED_EDGE('',*,*,#43675,.F.) ;
#58157=ORIENTED_EDGE('',*,*,#43676,.T.) ;
#58158=ORIENTED_EDGE('',*,*,#43677,.T.) ;
#58159=ORIENTED_EDGE('',*,*,#43678,.T.) ;
#58160=ORIENTED_EDGE('',*,*,#43679,.T.) ;
#58161=ORIENTED_EDGE('',*,*,#43680,.F.) ;
#58162=ORIENTED_EDGE('',*,*,#43681,.T.) ;
#58163=ORIENTED_EDGE('',*,*,#43682,.T.) ;
#58164=ORIENTED_EDGE('',*,*,#43683,.T.) ;
#58165=ORIENTED_EDGE('',*,*,#43684,.T.) ;
#58166=ORIENTED_EDGE('',*,*,#43685,.T.) ;
#58167=ORIENTED_EDGE('',*,*,#43686,.T.) ;
#58168=ORIENTED_EDGE('',*,*,#43687,.T.) ;
#58169=ORIENTED_EDGE('',*,*,#43658,.T.) ;
#58170=ORIENTED_EDGE('',*,*,#43674,.T.) ;
#58171=ORIENTED_EDGE('',*,*,#43688,.T.) ;
#58172=ORIENTED_EDGE('',*,*,#43689,.T.) ;
#58173=ORIENTED_EDGE('',*,*,#43690,.T.) ;
#58174=ORIENTED_EDGE('',*,*,#43691,.F.) ;
#58175=ORIENTED_EDGE('',*,*,#43692,.T.) ;
#58176=ORIENTED_EDGE('',*,*,#43693,.F.) ;
#58177=ORIENTED_EDGE('',*,*,#43694,.T.) ;
#58178=ORIENTED_EDGE('',*,*,#43695,.F.) ;
#58179=ORIENTED_EDGE('',*,*,#43696,.T.) ;
#58180=ORIENTED_EDGE('',*,*,#43697,.T.) ;
#58181=ORIENTED_EDGE('',*,*,#43698,.T.) ;
#58182=ORIENTED_EDGE('',*,*,#43699,.T.) ;
#58183=ORIENTED_EDGE('',*,*,#43700,.F.) ;
#58184=ORIENTED_EDGE('',*,*,#43701,.T.) ;
#58185=ORIENTED_EDGE('',*,*,#43644,.F.) ;
#58186=ORIENTED_EDGE('',*,*,#43638,.T.) ;
#58187=ORIENTED_EDGE('',*,*,#43702,.T.) ;
#58188=ORIENTED_EDGE('',*,*,#43703,.T.) ;
#58189=ORIENTED_EDGE('',*,*,#43704,.F.) ;
#58190=ORIENTED_EDGE('',*,*,#43705,.T.) ;
#58191=ORIENTED_EDGE('',*,*,#43706,.F.) ;
#58192=ORIENTED_EDGE('',*,*,#43707,.T.) ;
#58193=ORIENTED_EDGE('',*,*,#43708,.T.) ;
#58194=ORIENTED_EDGE('',*,*,#43709,.T.) ;
#58195=ORIENTED_EDGE('',*,*,#43710,.T.) ;
#58196=ORIENTED_EDGE('',*,*,#43711,.T.) ;
#58197=ORIENTED_EDGE('',*,*,#43712,.T.) ;
#58198=ORIENTED_EDGE('',*,*,#43713,.T.) ;
#58199=ORIENTED_EDGE('',*,*,#43714,.T.) ;
#58200=ORIENTED_EDGE('',*,*,#43715,.T.) ;
#58201=ORIENTED_EDGE('',*,*,#43716,.F.) ;
#58202=ORIENTED_EDGE('',*,*,#43717,.T.) ;
#58203=ORIENTED_EDGE('',*,*,#43718,.T.) ;
#58204=ORIENTED_EDGE('',*,*,#43719,.T.) ;
#58205=ORIENTED_EDGE('',*,*,#43720,.F.) ;
#58206=ORIENTED_EDGE('',*,*,#43721,.T.) ;
#58207=ORIENTED_EDGE('',*,*,#43722,.T.) ;
#58208=ORIENTED_EDGE('',*,*,#43723,.T.) ;
#58209=ORIENTED_EDGE('',*,*,#43724,.F.) ;
#58210=ORIENTED_EDGE('',*,*,#43725,.T.) ;
#58211=ORIENTED_EDGE('',*,*,#43726,.T.) ;
#58212=ORIENTED_EDGE('',*,*,#43727,.T.) ;
#58213=ORIENTED_EDGE('',*,*,#43728,.F.) ;
#58214=ORIENTED_EDGE('',*,*,#43729,.T.) ;
#58215=ORIENTED_EDGE('',*,*,#43730,.T.) ;
#58216=ORIENTED_EDGE('',*,*,#43731,.T.) ;
#58217=ORIENTED_EDGE('',*,*,#43732,.F.) ;
#58218=ORIENTED_EDGE('',*,*,#43733,.T.) ;
#58219=ORIENTED_EDGE('',*,*,#43734,.T.) ;
#58220=ORIENTED_EDGE('',*,*,#43735,.T.) ;
#58221=ORIENTED_EDGE('',*,*,#43736,.F.) ;
#58222=ORIENTED_EDGE('',*,*,#43737,.T.) ;
#58223=ORIENTED_EDGE('',*,*,#43738,.T.) ;
#58224=ORIENTED_EDGE('',*,*,#43739,.T.) ;
#58225=ORIENTED_EDGE('',*,*,#43740,.F.) ;
#58226=ORIENTED_EDGE('',*,*,#43741,.T.) ;
#58227=ORIENTED_EDGE('',*,*,#43742,.F.) ;
#58228=ORIENTED_EDGE('',*,*,#43743,.T.) ;
#58229=ORIENTED_EDGE('',*,*,#43744,.F.) ;
#58230=ORIENTED_EDGE('',*,*,#43745,.T.) ;
#58231=ORIENTED_EDGE('',*,*,#43746,.F.) ;
#58232=ORIENTED_EDGE('',*,*,#43747,.T.) ;
#58233=ORIENTED_EDGE('',*,*,#43748,.F.) ;
#58234=ORIENTED_EDGE('',*,*,#43749,.T.) ;
#58235=ORIENTED_EDGE('',*,*,#43631,.T.) ;
#58236=ORIENTED_EDGE('',*,*,#43750,.T.) ;
#58237=ORIENTED_EDGE('',*,*,#43751,.T.) ;
#58238=ORIENTED_EDGE('',*,*,#43752,.F.) ;
#58239=ORIENTED_EDGE('',*,*,#43753,.T.) ;
#58240=ORIENTED_EDGE('',*,*,#43754,.T.) ;
#58241=ORIENTED_EDGE('',*,*,#43630,.T.) ;
#58242=ORIENTED_EDGE('',*,*,#43755,.F.) ;
#58243=ORIENTED_EDGE('',*,*,#43756,.T.) ;
#58244=ORIENTED_EDGE('',*,*,#43757,.T.) ;
#58245=ORIENTED_EDGE('',*,*,#43758,.T.) ;
#58246=ORIENTED_EDGE('',*,*,#43759,.F.) ;
#58247=ORIENTED_EDGE('',*,*,#43628,.T.) ;
#58248=ORIENTED_EDGE('',*,*,#43760,.T.) ;
#58249=ORIENTED_EDGE('',*,*,#43761,.T.) ;
#58250=ORIENTED_EDGE('',*,*,#43762,.F.) ;
#58251=ORIENTED_EDGE('',*,*,#43763,.T.) ;
#58252=ORIENTED_EDGE('',*,*,#43764,.T.) ;
#58253=ORIENTED_EDGE('',*,*,#43765,.T.) ;
#58254=ORIENTED_EDGE('',*,*,#43766,.T.) ;
#58255=ORIENTED_EDGE('',*,*,#43767,.F.) ;
#58256=ORIENTED_EDGE('',*,*,#43768,.T.) ;
#58257=ORIENTED_EDGE('',*,*,#43769,.F.) ;
#58258=ORIENTED_EDGE('',*,*,#43770,.T.) ;
#58259=ORIENTED_EDGE('',*,*,#43771,.T.) ;
#58260=ORIENTED_EDGE('',*,*,#43772,.T.) ;
#58261=ORIENTED_EDGE('',*,*,#43773,.T.) ;
#58262=ORIENTED_EDGE('',*,*,#43774,.F.) ;
#58263=ORIENTED_EDGE('',*,*,#43775,.T.) ;
#58264=ORIENTED_EDGE('',*,*,#43776,.F.) ;
#58265=ORIENTED_EDGE('',*,*,#43777,.T.) ;
#58266=ORIENTED_EDGE('',*,*,#43778,.F.) ;
#58267=ORIENTED_EDGE('',*,*,#43779,.T.) ;
#58268=ORIENTED_EDGE('',*,*,#43780,.F.) ;
#58269=ORIENTED_EDGE('',*,*,#43781,.T.) ;
#58270=ORIENTED_EDGE('',*,*,#43782,.F.) ;
#58271=ORIENTED_EDGE('',*,*,#43783,.T.) ;
#58272=ORIENTED_EDGE('',*,*,#43784,.T.) ;
#58273=ORIENTED_EDGE('',*,*,#43785,.T.) ;
#58274=ORIENTED_EDGE('',*,*,#43786,.F.) ;
#58275=ORIENTED_EDGE('',*,*,#43787,.T.) ;
#58276=ORIENTED_EDGE('',*,*,#43788,.T.) ;
#58277=ORIENTED_EDGE('',*,*,#43789,.T.) ;
#58278=ORIENTED_EDGE('',*,*,#43790,.T.) ;
#58279=ORIENTED_EDGE('',*,*,#43791,.T.) ;
#58280=ORIENTED_EDGE('',*,*,#43792,.T.) ;
#58281=ORIENTED_EDGE('',*,*,#43793,.F.) ;
#58282=ORIENTED_EDGE('',*,*,#43794,.T.) ;
#58283=ORIENTED_EDGE('',*,*,#43795,.T.) ;
#58284=ORIENTED_EDGE('',*,*,#43796,.T.) ;
#58285=ORIENTED_EDGE('',*,*,#43797,.F.) ;
#58286=ORIENTED_EDGE('',*,*,#43798,.T.) ;
#58287=ORIENTED_EDGE('',*,*,#43799,.T.) ;
#58288=ORIENTED_EDGE('',*,*,#43800,.T.) ;
#58289=ORIENTED_EDGE('',*,*,#43801,.T.) ;
#58290=ORIENTED_EDGE('',*,*,#43802,.T.) ;
#58291=ORIENTED_EDGE('',*,*,#43803,.T.) ;
#58292=ORIENTED_EDGE('',*,*,#43804,.T.) ;
#58293=ORIENTED_EDGE('',*,*,#43793,.T.) ;
#58294=ORIENTED_EDGE('',*,*,#43805,.T.) ;
#58295=ORIENTED_EDGE('',*,*,#43797,.T.) ;
#58296=ORIENTED_EDGE('',*,*,#43806,.T.) ;
#58297=ORIENTED_EDGE('',*,*,#43680,.T.) ;
#58298=ORIENTED_EDGE('',*,*,#43807,.T.) ;
#58299=ORIENTED_EDGE('',*,*,#43691,.T.) ;
#58300=ORIENTED_EDGE('',*,*,#43808,.T.) ;
#58301=ORIENTED_EDGE('',*,*,#43704,.T.) ;
#58302=ORIENTED_EDGE('',*,*,#43809,.T.) ;
#58303=ORIENTED_EDGE('',*,*,#43706,.T.) ;
#58304=ORIENTED_EDGE('',*,*,#43810,.T.) ;
#58305=ORIENTED_EDGE('',*,*,#43716,.T.) ;
#58306=ORIENTED_EDGE('',*,*,#43811,.T.) ;
#58307=ORIENTED_EDGE('',*,*,#43720,.T.) ;
#58308=ORIENTED_EDGE('',*,*,#43812,.T.) ;
#58309=ORIENTED_EDGE('',*,*,#43724,.T.) ;
#58310=ORIENTED_EDGE('',*,*,#43813,.T.) ;
#58311=ORIENTED_EDGE('',*,*,#43728,.T.) ;
#58312=ORIENTED_EDGE('',*,*,#43814,.T.) ;
#58313=ORIENTED_EDGE('',*,*,#43732,.T.) ;
#58314=ORIENTED_EDGE('',*,*,#43815,.T.) ;
#58315=ORIENTED_EDGE('',*,*,#43736,.T.) ;
#58316=ORIENTED_EDGE('',*,*,#43816,.T.) ;
#58317=ORIENTED_EDGE('',*,*,#43740,.T.) ;
#58318=ORIENTED_EDGE('',*,*,#43817,.T.) ;
#58319=ORIENTED_EDGE('',*,*,#43752,.T.) ;
#58320=ORIENTED_EDGE('',*,*,#43818,.T.) ;
#58321=ORIENTED_EDGE('',*,*,#43755,.T.) ;
#58322=ORIENTED_EDGE('',*,*,#43629,.T.) ;
#58323=ORIENTED_EDGE('',*,*,#43759,.T.) ;
#58324=ORIENTED_EDGE('',*,*,#43819,.T.) ;
#58325=ORIENTED_EDGE('',*,*,#43762,.T.) ;
#58326=ORIENTED_EDGE('',*,*,#43820,.T.) ;
#58327=ORIENTED_EDGE('',*,*,#43774,.T.) ;
#58328=ORIENTED_EDGE('',*,*,#43821,.T.) ;
#58329=ORIENTED_EDGE('',*,*,#43786,.T.) ;
#58330=ORIENTED_EDGE('',*,*,#43822,.T.) ;
#58331=ORIENTED_EDGE('',*,*,#43678,.F.) ;
#58332=ORIENTED_EDGE('',*,*,#43823,.T.) ;
#58333=ORIENTED_EDGE('',*,*,#43795,.F.) ;
#58334=ORIENTED_EDGE('',*,*,#43824,.T.) ;
#58335=ORIENTED_EDGE('',*,*,#43784,.F.) ;
#58336=ORIENTED_EDGE('',*,*,#43825,.T.) ;
#58337=ORIENTED_EDGE('',*,*,#43772,.F.) ;
#58338=ORIENTED_EDGE('',*,*,#43826,.T.) ;
#58339=ORIENTED_EDGE('',*,*,#43760,.F.) ;
#58340=ORIENTED_EDGE('',*,*,#43827,.T.) ;
#58341=ORIENTED_EDGE('',*,*,#43757,.F.) ;
#58342=ORIENTED_EDGE('',*,*,#43627,.T.) ;
#58343=ORIENTED_EDGE('',*,*,#43754,.F.) ;
#58344=ORIENTED_EDGE('',*,*,#43828,.T.) ;
#58345=ORIENTED_EDGE('',*,*,#43750,.F.) ;
#58346=ORIENTED_EDGE('',*,*,#43829,.T.) ;
#58347=ORIENTED_EDGE('',*,*,#43738,.F.) ;
#58348=ORIENTED_EDGE('',*,*,#43830,.T.) ;
#58349=ORIENTED_EDGE('',*,*,#43734,.F.) ;
#58350=ORIENTED_EDGE('',*,*,#43831,.T.) ;
#58351=ORIENTED_EDGE('',*,*,#43730,.F.) ;
#58352=ORIENTED_EDGE('',*,*,#43832,.T.) ;
#58353=ORIENTED_EDGE('',*,*,#43726,.F.) ;
#58354=ORIENTED_EDGE('',*,*,#43833,.T.) ;
#58355=ORIENTED_EDGE('',*,*,#43722,.F.) ;
#58356=ORIENTED_EDGE('',*,*,#43834,.T.) ;
#58357=ORIENTED_EDGE('',*,*,#43718,.F.) ;
#58358=ORIENTED_EDGE('',*,*,#43835,.T.) ;
#58359=ORIENTED_EDGE('',*,*,#43714,.F.) ;
#58360=ORIENTED_EDGE('',*,*,#43836,.T.) ;
#58361=ORIENTED_EDGE('',*,*,#43712,.F.) ;
#58362=ORIENTED_EDGE('',*,*,#43837,.T.) ;
#58363=ORIENTED_EDGE('',*,*,#43684,.F.) ;
#58364=ORIENTED_EDGE('',*,*,#43838,.T.) ;
#58365=ORIENTED_EDGE('',*,*,#43697,.F.) ;
#58366=ORIENTED_EDGE('',*,*,#43839,.T.) ;
#58367=ORIENTED_EDGE('',*,*,#43803,.F.) ;
#58368=ORIENTED_EDGE('',*,*,#43840,.T.) ;
#58369=ORIENTED_EDGE('',*,*,#43841,.T.) ;
#58370=ORIENTED_EDGE('',*,*,#43842,.T.) ;
#58371=ORIENTED_EDGE('',*,*,#43843,.T.) ;
#58372=ORIENTED_EDGE('',*,*,#43844,.T.) ;
#58373=ORIENTED_EDGE('',*,*,#43845,.T.) ;
#58374=ORIENTED_EDGE('',*,*,#43846,.T.) ;
#58375=ORIENTED_EDGE('',*,*,#43847,.T.) ;
#58376=ORIENTED_EDGE('',*,*,#43848,.T.) ;
#58377=ORIENTED_EDGE('',*,*,#43849,.F.) ;
#58378=ORIENTED_EDGE('',*,*,#43850,.T.) ;
#58379=ORIENTED_EDGE('',*,*,#43851,.T.) ;
#58380=ORIENTED_EDGE('',*,*,#43852,.T.) ;
#58381=ORIENTED_EDGE('',*,*,#43853,.F.) ;
#58382=ORIENTED_EDGE('',*,*,#43854,.T.) ;
#58383=ORIENTED_EDGE('',*,*,#43855,.T.) ;
#58384=ORIENTED_EDGE('',*,*,#43856,.T.) ;
#58385=ORIENTED_EDGE('',*,*,#43857,.T.) ;
#58386=ORIENTED_EDGE('',*,*,#43858,.T.) ;
#58387=ORIENTED_EDGE('',*,*,#43859,.F.) ;
#58388=ORIENTED_EDGE('',*,*,#43860,.T.) ;
#58389=ORIENTED_EDGE('',*,*,#43851,.F.) ;
#58390=ORIENTED_EDGE('',*,*,#43861,.T.) ;
#58391=ORIENTED_EDGE('',*,*,#43862,.T.) ;
#58392=ORIENTED_EDGE('',*,*,#43863,.T.) ;
#58393=ORIENTED_EDGE('',*,*,#43864,.F.) ;
#58394=ORIENTED_EDGE('',*,*,#43865,.T.) ;
#58395=ORIENTED_EDGE('',*,*,#43857,.F.) ;
#58396=ORIENTED_EDGE('',*,*,#43866,.T.) ;
#58397=ORIENTED_EDGE('',*,*,#43867,.F.) ;
#58398=ORIENTED_EDGE('',*,*,#43868,.T.) ;
#58399=ORIENTED_EDGE('',*,*,#43869,.T.) ;
#58400=ORIENTED_EDGE('',*,*,#43870,.T.) ;
#58401=ORIENTED_EDGE('',*,*,#43862,.F.) ;
#58402=ORIENTED_EDGE('',*,*,#43871,.T.) ;
#58403=ORIENTED_EDGE('',*,*,#43872,.T.) ;
#58404=ORIENTED_EDGE('',*,*,#43873,.T.) ;
#58405=ORIENTED_EDGE('',*,*,#43859,.T.) ;
#58406=ORIENTED_EDGE('',*,*,#43874,.T.) ;
#58407=ORIENTED_EDGE('',*,*,#43875,.T.) ;
#58408=ORIENTED_EDGE('',*,*,#43876,.T.) ;
#58409=ORIENTED_EDGE('',*,*,#43877,.T.) ;
#58410=ORIENTED_EDGE('',*,*,#43878,.T.) ;
#58411=ORIENTED_EDGE('',*,*,#43879,.T.) ;
#58412=ORIENTED_EDGE('',*,*,#43880,.T.) ;
#58413=ORIENTED_EDGE('',*,*,#43881,.T.) ;
#58414=ORIENTED_EDGE('',*,*,#43882,.T.) ;
#58415=ORIENTED_EDGE('',*,*,#43883,.T.) ;
#58416=ORIENTED_EDGE('',*,*,#43884,.T.) ;
#58417=ORIENTED_EDGE('',*,*,#43885,.T.) ;
#58418=ORIENTED_EDGE('',*,*,#43886,.T.) ;
#58419=ORIENTED_EDGE('',*,*,#43887,.T.) ;
#58420=ORIENTED_EDGE('',*,*,#43888,.T.) ;
#58421=ORIENTED_EDGE('',*,*,#43889,.T.) ;
#58422=ORIENTED_EDGE('',*,*,#43890,.T.) ;
#58423=ORIENTED_EDGE('',*,*,#43891,.T.) ;
#58424=ORIENTED_EDGE('',*,*,#43892,.T.) ;
#58425=ORIENTED_EDGE('',*,*,#43893,.T.) ;
#58426=ORIENTED_EDGE('',*,*,#43894,.T.) ;
#58427=ORIENTED_EDGE('',*,*,#43895,.T.) ;
#58428=ORIENTED_EDGE('',*,*,#43896,.T.) ;
#58429=ORIENTED_EDGE('',*,*,#43897,.T.) ;
#58430=ORIENTED_EDGE('',*,*,#43898,.T.) ;
#58431=ORIENTED_EDGE('',*,*,#43899,.T.) ;
#58432=ORIENTED_EDGE('',*,*,#43900,.T.) ;
#58433=ORIENTED_EDGE('',*,*,#43901,.T.) ;
#58434=ORIENTED_EDGE('',*,*,#43902,.T.) ;
#58435=ORIENTED_EDGE('',*,*,#43903,.T.) ;
#58436=ORIENTED_EDGE('',*,*,#43904,.T.) ;
#58437=ORIENTED_EDGE('',*,*,#43905,.T.) ;
#58438=ORIENTED_EDGE('',*,*,#43906,.T.) ;
#58439=ORIENTED_EDGE('',*,*,#43907,.T.) ;
#58440=ORIENTED_EDGE('',*,*,#43908,.T.) ;
#58441=ORIENTED_EDGE('',*,*,#43909,.F.) ;
#58442=ORIENTED_EDGE('',*,*,#43910,.F.) ;
#58443=ORIENTED_EDGE('',*,*,#43911,.F.) ;
#58444=ORIENTED_EDGE('',*,*,#43912,.F.) ;
#58445=ORIENTED_EDGE('',*,*,#43913,.F.) ;
#58446=ORIENTED_EDGE('',*,*,#43914,.F.) ;
#58447=ORIENTED_EDGE('',*,*,#43915,.F.) ;
#58448=ORIENTED_EDGE('',*,*,#43916,.F.) ;
#58449=ORIENTED_EDGE('',*,*,#43917,.F.) ;
#58450=ORIENTED_EDGE('',*,*,#43918,.F.) ;
#58451=ORIENTED_EDGE('',*,*,#43916,.T.) ;
#58452=ORIENTED_EDGE('',*,*,#43919,.T.) ;
#58453=ORIENTED_EDGE('',*,*,#43920,.F.) ;
#58454=ORIENTED_EDGE('',*,*,#43921,.F.) ;
#58455=ORIENTED_EDGE('',*,*,#43909,.T.) ;
#58456=ORIENTED_EDGE('',*,*,#43918,.T.) ;
#58457=ORIENTED_EDGE('',*,*,#43922,.F.) ;
#58458=ORIENTED_EDGE('',*,*,#43923,.F.) ;
#58459=ORIENTED_EDGE('',*,*,#43910,.T.) ;
#58460=ORIENTED_EDGE('',*,*,#43921,.T.) ;
#58461=ORIENTED_EDGE('',*,*,#43924,.F.) ;
#58462=ORIENTED_EDGE('',*,*,#43925,.F.) ;
#58463=ORIENTED_EDGE('',*,*,#43911,.T.) ;
#58464=ORIENTED_EDGE('',*,*,#43923,.T.) ;
#58465=ORIENTED_EDGE('',*,*,#43926,.F.) ;
#58466=ORIENTED_EDGE('',*,*,#43927,.F.) ;
#58467=ORIENTED_EDGE('',*,*,#43912,.T.) ;
#58468=ORIENTED_EDGE('',*,*,#43925,.T.) ;
#58469=ORIENTED_EDGE('',*,*,#43928,.F.) ;
#58470=ORIENTED_EDGE('',*,*,#43929,.F.) ;
#58471=ORIENTED_EDGE('',*,*,#43913,.T.) ;
#58472=ORIENTED_EDGE('',*,*,#43927,.T.) ;
#58473=ORIENTED_EDGE('',*,*,#43930,.F.) ;
#58474=ORIENTED_EDGE('',*,*,#43931,.F.) ;
#58475=ORIENTED_EDGE('',*,*,#43914,.T.) ;
#58476=ORIENTED_EDGE('',*,*,#43929,.T.) ;
#58477=ORIENTED_EDGE('',*,*,#43932,.F.) ;
#58478=ORIENTED_EDGE('',*,*,#43919,.F.) ;
#58479=ORIENTED_EDGE('',*,*,#43915,.T.) ;
#58480=ORIENTED_EDGE('',*,*,#43931,.T.) ;
#58481=ORIENTED_EDGE('',*,*,#43920,.T.) ;
#58482=ORIENTED_EDGE('',*,*,#43917,.T.) ;
#58483=ORIENTED_EDGE('',*,*,#43932,.T.) ;
#58484=ORIENTED_EDGE('',*,*,#43930,.T.) ;
#58485=ORIENTED_EDGE('',*,*,#43928,.T.) ;
#58486=ORIENTED_EDGE('',*,*,#43926,.T.) ;
#58487=ORIENTED_EDGE('',*,*,#43924,.T.) ;
#58488=ORIENTED_EDGE('',*,*,#43922,.T.) ;
#58489=ORIENTED_EDGE('',*,*,#43666,.T.) ;
#58490=ORIENTED_EDGE('',*,*,#43933,.T.) ;
#58491=ORIENTED_EDGE('',*,*,#43664,.F.) ;
#58492=ORIENTED_EDGE('',*,*,#43934,.T.) ;
#58493=ORIENTED_EDGE('',*,*,#43668,.T.) ;
#58494=ORIENTED_EDGE('',*,*,#43935,.T.) ;
#58495=ORIENTED_EDGE('',*,*,#43672,.F.) ;
#58496=ORIENTED_EDGE('',*,*,#43936,.T.) ;
#58497=ORIENTED_EDGE('',*,*,#43660,.T.) ;
#58498=ORIENTED_EDGE('',*,*,#43937,.T.) ;
#58499=ORIENTED_EDGE('',*,*,#43662,.T.) ;
#58500=ORIENTED_EDGE('',*,*,#43938,.T.) ;
#58501=ORIENTED_EDGE('',*,*,#43670,.T.) ;
#58502=ORIENTED_EDGE('',*,*,#43939,.T.) ;
#58503=ORIENTED_EDGE('',*,*,#43940,.T.) ;
#58504=ORIENTED_EDGE('',*,*,#43941,.T.) ;
#58505=ORIENTED_EDGE('',*,*,#43942,.T.) ;
#58506=ORIENTED_EDGE('',*,*,#43943,.T.) ;
#58507=ORIENTED_EDGE('',*,*,#43944,.T.) ;
#58508=ORIENTED_EDGE('',*,*,#43945,.T.) ;
#58509=ORIENTED_EDGE('',*,*,#43946,.T.) ;
#58510=ORIENTED_EDGE('',*,*,#43947,.T.) ;
#58511=ORIENTED_EDGE('',*,*,#43948,.T.) ;
#58512=ORIENTED_EDGE('',*,*,#43949,.T.) ;
#58513=ORIENTED_EDGE('',*,*,#43950,.T.) ;
#58514=ORIENTED_EDGE('',*,*,#43951,.T.) ;
#58515=ORIENTED_EDGE('',*,*,#43952,.T.) ;
#58516=ORIENTED_EDGE('',*,*,#43953,.T.) ;
#58517=ORIENTED_EDGE('',*,*,#43954,.T.) ;
#58518=ORIENTED_EDGE('',*,*,#43955,.T.) ;
#58519=ORIENTED_EDGE('',*,*,#43956,.T.) ;
#58520=ORIENTED_EDGE('',*,*,#43957,.T.) ;
#58521=ORIENTED_EDGE('',*,*,#43958,.T.) ;
#58522=ORIENTED_EDGE('',*,*,#43959,.T.) ;
#58523=ORIENTED_EDGE('',*,*,#43960,.F.) ;
#58524=ORIENTED_EDGE('',*,*,#43961,.F.) ;
#58525=ORIENTED_EDGE('',*,*,#43962,.F.) ;
#58526=ORIENTED_EDGE('',*,*,#43963,.F.) ;
#58527=ORIENTED_EDGE('',*,*,#43964,.F.) ;
#58528=ORIENTED_EDGE('',*,*,#43965,.F.) ;
#58529=ORIENTED_EDGE('',*,*,#43966,.F.) ;
#58530=ORIENTED_EDGE('',*,*,#43967,.F.) ;
#58531=ORIENTED_EDGE('',*,*,#43968,.T.) ;
#58532=ORIENTED_EDGE('',*,*,#43969,.T.) ;
#58533=ORIENTED_EDGE('',*,*,#43970,.F.) ;
#58534=ORIENTED_EDGE('',*,*,#43967,.T.) ;
#58535=ORIENTED_EDGE('',*,*,#43970,.T.) ;
#58536=ORIENTED_EDGE('',*,*,#43971,.T.) ;
#58537=ORIENTED_EDGE('',*,*,#43972,.F.) ;
#58538=ORIENTED_EDGE('',*,*,#43960,.T.) ;
#58539=ORIENTED_EDGE('',*,*,#43972,.T.) ;
#58540=ORIENTED_EDGE('',*,*,#43973,.T.) ;
#58541=ORIENTED_EDGE('',*,*,#43974,.F.) ;
#58542=ORIENTED_EDGE('',*,*,#43961,.T.) ;
#58543=ORIENTED_EDGE('',*,*,#43974,.T.) ;
#58544=ORIENTED_EDGE('',*,*,#43975,.T.) ;
#58545=ORIENTED_EDGE('',*,*,#43976,.F.) ;
#58546=ORIENTED_EDGE('',*,*,#43962,.T.) ;
#58547=ORIENTED_EDGE('',*,*,#43976,.T.) ;
#58548=ORIENTED_EDGE('',*,*,#43977,.T.) ;
#58549=ORIENTED_EDGE('',*,*,#43978,.F.) ;
#58550=ORIENTED_EDGE('',*,*,#43963,.T.) ;
#58551=ORIENTED_EDGE('',*,*,#43978,.T.) ;
#58552=ORIENTED_EDGE('',*,*,#43979,.T.) ;
#58553=ORIENTED_EDGE('',*,*,#43980,.F.) ;
#58554=ORIENTED_EDGE('',*,*,#43964,.T.) ;
#58555=ORIENTED_EDGE('',*,*,#43980,.T.) ;
#58556=ORIENTED_EDGE('',*,*,#43981,.T.) ;
#58557=ORIENTED_EDGE('',*,*,#43982,.F.) ;
#58558=ORIENTED_EDGE('',*,*,#43965,.T.) ;
#58559=ORIENTED_EDGE('',*,*,#43982,.T.) ;
#58560=ORIENTED_EDGE('',*,*,#43983,.T.) ;
#58561=ORIENTED_EDGE('',*,*,#43968,.F.) ;
#58562=ORIENTED_EDGE('',*,*,#43966,.T.) ;
#58563=ORIENTED_EDGE('',*,*,#43984,.T.) ;
#58564=ORIENTED_EDGE('',*,*,#43985,.T.) ;
#58565=ORIENTED_EDGE('',*,*,#43986,.T.) ;
#58566=ORIENTED_EDGE('',*,*,#43987,.T.) ;
#58567=ORIENTED_EDGE('',*,*,#43988,.T.) ;
#58568=ORIENTED_EDGE('',*,*,#43989,.T.) ;
#58569=ORIENTED_EDGE('',*,*,#43990,.T.) ;
#58570=ORIENTED_EDGE('',*,*,#43991,.T.) ;
#58571=ORIENTED_EDGE('',*,*,#43992,.T.) ;
#58572=ORIENTED_EDGE('',*,*,#43649,.T.) ;
#58573=ORIENTED_EDGE('',*,*,#43993,.T.) ;
#58574=ORIENTED_EDGE('',*,*,#43994,.T.) ;
#58575=ORIENTED_EDGE('',*,*,#43651,.T.) ;
#58576=ORIENTED_EDGE('',*,*,#43995,.T.) ;
#58577=ORIENTED_EDGE('',*,*,#43996,.T.) ;
#58578=ORIENTED_EDGE('',*,*,#43997,.T.) ;
#58579=ORIENTED_EDGE('',*,*,#43998,.T.) ;
#58580=ORIENTED_EDGE('',*,*,#43999,.T.) ;
#58581=ORIENTED_EDGE('',*,*,#44000,.T.) ;
#58582=ORIENTED_EDGE('',*,*,#44001,.T.) ;
#58583=ORIENTED_EDGE('',*,*,#44002,.T.) ;
#58584=ORIENTED_EDGE('',*,*,#43623,.T.) ;
#58585=ORIENTED_EDGE('',*,*,#43655,.T.) ;
#58586=ORIENTED_EDGE('',*,*,#44003,.T.) ;
#58587=ORIENTED_EDGE('',*,*,#44004,.T.) ;
#58588=ORIENTED_EDGE('',*,*,#44005,.T.) ;
#58589=ORIENTED_EDGE('',*,*,#44006,.T.) ;
#58590=ORIENTED_EDGE('',*,*,#44007,.T.) ;
#58591=ORIENTED_EDGE('',*,*,#44008,.T.) ;
#58592=ORIENTED_EDGE('',*,*,#44009,.F.) ;
#58593=ORIENTED_EDGE('',*,*,#44010,.F.) ;
#58594=ORIENTED_EDGE('',*,*,#44011,.F.) ;
#58595=ORIENTED_EDGE('',*,*,#43765,.F.) ;
#58596=ORIENTED_EDGE('',*,*,#43861,.F.) ;
#58597=ORIENTED_EDGE('',*,*,#43850,.F.) ;
#58598=ORIENTED_EDGE('',*,*,#44012,.F.) ;
#58599=ORIENTED_EDGE('',*,*,#43871,.F.) ;
#58600=ORIENTED_EDGE('',*,*,#44012,.T.) ;
#58601=ORIENTED_EDGE('',*,*,#43849,.T.) ;
#58602=ORIENTED_EDGE('',*,*,#44013,.F.) ;
#58603=ORIENTED_EDGE('',*,*,#44014,.F.) ;
#58604=ORIENTED_EDGE('',*,*,#44013,.T.) ;
#58605=ORIENTED_EDGE('',*,*,#43856,.F.) ;
#58606=ORIENTED_EDGE('',*,*,#44015,.F.) ;
#58607=ORIENTED_EDGE('',*,*,#43887,.F.) ;
#58608=ORIENTED_EDGE('',*,*,#44010,.T.) ;
#58609=ORIENTED_EDGE('',*,*,#43888,.F.) ;
#58610=ORIENTED_EDGE('',*,*,#44016,.F.) ;
#58611=ORIENTED_EDGE('',*,*,#43847,.F.) ;
#58612=ORIENTED_EDGE('',*,*,#44011,.T.) ;
#58613=ORIENTED_EDGE('',*,*,#43846,.F.) ;
#58614=ORIENTED_EDGE('',*,*,#44017,.F.) ;
#58615=ORIENTED_EDGE('',*,*,#43766,.F.) ;
#58616=ORIENTED_EDGE('',*,*,#44009,.T.) ;
#58617=ORIENTED_EDGE('',*,*,#43764,.F.) ;
#58618=ORIENTED_EDGE('',*,*,#44018,.F.) ;
#58619=ORIENTED_EDGE('',*,*,#43883,.F.) ;
#58620=ORIENTED_EDGE('',*,*,#44014,.T.) ;
#58621=ORIENTED_EDGE('',*,*,#43886,.F.) ;
#58622=ORIENTED_EDGE('',*,*,#44019,.F.) ;
#58623=ORIENTED_EDGE('',*,*,#43872,.F.) ;
#58624=ORIENTED_EDGE('',*,*,#43863,.F.) ;
#58625=ORIENTED_EDGE('',*,*,#43873,.F.) ;
#58626=ORIENTED_EDGE('',*,*,#44020,.F.) ;
#58627=ORIENTED_EDGE('',*,*,#43866,.F.) ;
#58628=ORIENTED_EDGE('',*,*,#44016,.T.) ;
#58629=ORIENTED_EDGE('',*,*,#44015,.T.) ;
#58630=ORIENTED_EDGE('',*,*,#44021,.F.) ;
#58631=ORIENTED_EDGE('',*,*,#43767,.T.) ;
#58632=ORIENTED_EDGE('',*,*,#44017,.T.) ;
#58633=ORIENTED_EDGE('',*,*,#44022,.F.) ;
#58634=ORIENTED_EDGE('',*,*,#44023,.F.) ;
#58635=ORIENTED_EDGE('',*,*,#44018,.T.) ;
#58636=ORIENTED_EDGE('',*,*,#43771,.F.) ;
#58637=ORIENTED_EDGE('',*,*,#44024,.F.) ;
#58638=ORIENTED_EDGE('',*,*,#44025,.F.) ;
#58639=ORIENTED_EDGE('',*,*,#44020,.T.) ;
#58640=ORIENTED_EDGE('',*,*,#44019,.T.) ;
#58641=ORIENTED_EDGE('',*,*,#44026,.F.) ;
#58642=ORIENTED_EDGE('',*,*,#43867,.T.) ;
#58643=ORIENTED_EDGE('',*,*,#44021,.T.) ;
#58644=ORIENTED_EDGE('',*,*,#43855,.F.) ;
#58645=ORIENTED_EDGE('',*,*,#44027,.F.) ;
#58646=ORIENTED_EDGE('',*,*,#43848,.F.) ;
#58647=ORIENTED_EDGE('',*,*,#44022,.T.) ;
#58648=ORIENTED_EDGE('',*,*,#43845,.F.) ;
#58649=ORIENTED_EDGE('',*,*,#44028,.F.) ;
#58650=ORIENTED_EDGE('',*,*,#43881,.F.) ;
#58651=ORIENTED_EDGE('',*,*,#44023,.T.) ;
#58652=ORIENTED_EDGE('',*,*,#43880,.F.) ;
#58653=ORIENTED_EDGE('',*,*,#44029,.F.) ;
#58654=ORIENTED_EDGE('',*,*,#43768,.F.) ;
#58655=ORIENTED_EDGE('',*,*,#44024,.T.) ;
#58656=ORIENTED_EDGE('',*,*,#43770,.F.) ;
#58657=ORIENTED_EDGE('',*,*,#44030,.F.) ;
#58658=ORIENTED_EDGE('',*,*,#43842,.F.) ;
#58659=ORIENTED_EDGE('',*,*,#44025,.T.) ;
#58660=ORIENTED_EDGE('',*,*,#43841,.F.) ;
#58661=ORIENTED_EDGE('',*,*,#44031,.F.) ;
#58662=ORIENTED_EDGE('',*,*,#43884,.F.) ;
#58663=ORIENTED_EDGE('',*,*,#44026,.T.) ;
#58664=ORIENTED_EDGE('',*,*,#43885,.F.) ;
#58665=ORIENTED_EDGE('',*,*,#44032,.F.) ;
#58666=ORIENTED_EDGE('',*,*,#43868,.F.) ;
#58667=ORIENTED_EDGE('',*,*,#44028,.T.) ;
#58668=ORIENTED_EDGE('',*,*,#44027,.T.) ;
#58669=ORIENTED_EDGE('',*,*,#44033,.F.) ;
#58670=ORIENTED_EDGE('',*,*,#43769,.T.) ;
#58671=ORIENTED_EDGE('',*,*,#44029,.T.) ;
#58672=ORIENTED_EDGE('',*,*,#44034,.F.) ;
#58673=ORIENTED_EDGE('',*,*,#44030,.T.) ;
#58674=ORIENTED_EDGE('',*,*,#44032,.T.) ;
#58675=ORIENTED_EDGE('',*,*,#44031,.T.) ;
#58676=ORIENTED_EDGE('',*,*,#44035,.F.) ;
#58677=ORIENTED_EDGE('',*,*,#43860,.F.) ;
#58678=ORIENTED_EDGE('',*,*,#43876,.F.) ;
#58679=ORIENTED_EDGE('',*,*,#44036,.F.) ;
#58680=ORIENTED_EDGE('',*,*,#43852,.F.) ;
#58681=ORIENTED_EDGE('',*,*,#44033,.T.) ;
#58682=ORIENTED_EDGE('',*,*,#43854,.F.) ;
#58683=ORIENTED_EDGE('',*,*,#44037,.F.) ;
#58684=ORIENTED_EDGE('',*,*,#43882,.F.) ;
#58685=ORIENTED_EDGE('',*,*,#44034,.T.) ;
#58686=ORIENTED_EDGE('',*,*,#43879,.F.) ;
#58687=ORIENTED_EDGE('',*,*,#44038,.F.) ;
#58688=ORIENTED_EDGE('',*,*,#43843,.F.) ;
#58689=ORIENTED_EDGE('',*,*,#44035,.T.) ;
#58690=ORIENTED_EDGE('',*,*,#43844,.F.) ;
#58691=ORIENTED_EDGE('',*,*,#44039,.F.) ;
#58692=ORIENTED_EDGE('',*,*,#43869,.F.) ;
#58693=ORIENTED_EDGE('',*,*,#43853,.T.) ;
#58694=ORIENTED_EDGE('',*,*,#44036,.T.) ;
#58695=ORIENTED_EDGE('',*,*,#44040,.F.) ;
#58696=ORIENTED_EDGE('',*,*,#44037,.T.) ;
#58697=ORIENTED_EDGE('',*,*,#44039,.T.) ;
#58698=ORIENTED_EDGE('',*,*,#44038,.T.) ;
#58699=ORIENTED_EDGE('',*,*,#44041,.F.) ;
#58700=ORIENTED_EDGE('',*,*,#44040,.T.) ;
#58701=ORIENTED_EDGE('',*,*,#43875,.F.) ;
#58702=ORIENTED_EDGE('',*,*,#44042,.F.) ;
#58703=ORIENTED_EDGE('',*,*,#43877,.F.) ;
#58704=ORIENTED_EDGE('',*,*,#44041,.T.) ;
#58705=ORIENTED_EDGE('',*,*,#43878,.F.) ;
#58706=ORIENTED_EDGE('',*,*,#44043,.F.) ;
#58707=ORIENTED_EDGE('',*,*,#43870,.F.) ;
#58708=ORIENTED_EDGE('',*,*,#44043,.T.) ;
#58709=ORIENTED_EDGE('',*,*,#44042,.T.) ;
#58710=ORIENTED_EDGE('',*,*,#44044,.F.) ;
#58711=ORIENTED_EDGE('',*,*,#43864,.T.) ;
#58712=ORIENTED_EDGE('',*,*,#43858,.F.) ;
#58713=ORIENTED_EDGE('',*,*,#43865,.F.) ;
#58714=ORIENTED_EDGE('',*,*,#44044,.T.) ;
#58715=ORIENTED_EDGE('',*,*,#43874,.F.) ;
#58716=ORIENTED_EDGE('',*,*,#43653,.F.) ;
#58717=ORIENTED_EDGE('',*,*,#43698,.F.) ;
#58718=ORIENTED_EDGE('',*,*,#43838,.F.) ;
#58719=ORIENTED_EDGE('',*,*,#43687,.F.) ;
#58720=ORIENTED_EDGE('',*,*,#43686,.F.) ;
#58721=ORIENTED_EDGE('',*,*,#44045,.T.) ;
#58722=ORIENTED_EDGE('',*,*,#44046,.T.) ;
#58723=ORIENTED_EDGE('',*,*,#43625,.T.) ;
#58724=ORIENTED_EDGE('',*,*,#43988,.F.) ;
#58725=ORIENTED_EDGE('',*,*,#43654,.T.) ;
#58726=ORIENTED_EDGE('',*,*,#43990,.F.) ;
#58727=ORIENTED_EDGE('',*,*,#44047,.T.) ;
#58728=ORIENTED_EDGE('',*,*,#43994,.F.) ;
#58729=ORIENTED_EDGE('',*,*,#44048,.F.) ;
#58730=ORIENTED_EDGE('',*,*,#43652,.T.) ;
#58731=ORIENTED_EDGE('',*,*,#43991,.F.) ;
#58732=ORIENTED_EDGE('',*,*,#44049,.F.) ;
#58733=ORIENTED_EDGE('',*,*,#43699,.F.) ;
#58734=ORIENTED_EDGE('',*,*,#43709,.F.) ;
#58735=ORIENTED_EDGE('',*,*,#44050,.T.) ;
#58736=ORIENTED_EDGE('',*,*,#43998,.F.) ;
#58737=ORIENTED_EDGE('',*,*,#44051,.T.) ;
#58738=ORIENTED_EDGE('',*,*,#44001,.F.) ;
#58739=ORIENTED_EDGE('',*,*,#44052,.T.) ;
#58740=ORIENTED_EDGE('',*,*,#43992,.F.) ;
#58741=ORIENTED_EDGE('',*,*,#44053,.T.) ;
#58742=ORIENTED_EDGE('',*,*,#44049,.T.) ;
#58743=ORIENTED_EDGE('',*,*,#44048,.T.) ;
#58744=ORIENTED_EDGE('',*,*,#44054,.F.) ;
#58745=ORIENTED_EDGE('',*,*,#43700,.T.) ;
#58746=ORIENTED_EDGE('',*,*,#43808,.F.) ;
#58747=ORIENTED_EDGE('',*,*,#43690,.F.) ;
#58748=ORIENTED_EDGE('',*,*,#43647,.F.) ;
#58749=ORIENTED_EDGE('',*,*,#43705,.F.) ;
#58750=ORIENTED_EDGE('',*,*,#44055,.T.) ;
#58751=ORIENTED_EDGE('',*,*,#44056,.T.) ;
#58752=ORIENTED_EDGE('',*,*,#43702,.F.) ;
#58753=ORIENTED_EDGE('',*,*,#43646,.F.) ;
#58754=ORIENTED_EDGE('',*,*,#43996,.F.) ;
#58755=ORIENTED_EDGE('',*,*,#44057,.T.) ;
#58756=ORIENTED_EDGE('',*,*,#44054,.T.) ;
#58757=ORIENTED_EDGE('',*,*,#43993,.F.) ;
#58758=ORIENTED_EDGE('',*,*,#43645,.F.) ;
#58759=ORIENTED_EDGE('',*,*,#43701,.F.) ;
#58760=ORIENTED_EDGE('',*,*,#43648,.T.) ;
#58761=ORIENTED_EDGE('',*,*,#43689,.F.) ;
#58762=ORIENTED_EDGE('',*,*,#43643,.T.) ;
#58763=ORIENTED_EDGE('',*,*,#43997,.F.) ;
#58764=ORIENTED_EDGE('',*,*,#44058,.F.) ;
#58765=ORIENTED_EDGE('',*,*,#43973,.F.) ;
#58766=ORIENTED_EDGE('',*,*,#44059,.F.) ;
#58767=ORIENTED_EDGE('',*,*,#44059,.T.) ;
#58768=ORIENTED_EDGE('',*,*,#43971,.F.) ;
#58769=ORIENTED_EDGE('',*,*,#44060,.F.) ;
#58770=ORIENTED_EDGE('',*,*,#43984,.F.) ;
#58771=ORIENTED_EDGE('',*,*,#44058,.T.) ;
#58772=ORIENTED_EDGE('',*,*,#43987,.F.) ;
#58773=ORIENTED_EDGE('',*,*,#44061,.F.) ;
#58774=ORIENTED_EDGE('',*,*,#43975,.F.) ;
#58775=ORIENTED_EDGE('',*,*,#44060,.T.) ;
#58776=ORIENTED_EDGE('',*,*,#43969,.F.) ;
#58777=ORIENTED_EDGE('',*,*,#44062,.F.) ;
#58778=ORIENTED_EDGE('',*,*,#43977,.F.) ;
#58779=ORIENTED_EDGE('',*,*,#44061,.T.) ;
#58780=ORIENTED_EDGE('',*,*,#44063,.F.) ;
#58781=ORIENTED_EDGE('',*,*,#44062,.T.) ;
#58782=ORIENTED_EDGE('',*,*,#43983,.F.) ;
#58783=ORIENTED_EDGE('',*,*,#44064,.F.) ;
#58784=ORIENTED_EDGE('',*,*,#43985,.F.) ;
#58785=ORIENTED_EDGE('',*,*,#44063,.T.) ;
#58786=ORIENTED_EDGE('',*,*,#43986,.F.) ;
#58787=ORIENTED_EDGE('',*,*,#44065,.F.) ;
#58788=ORIENTED_EDGE('',*,*,#43979,.F.) ;
#58789=ORIENTED_EDGE('',*,*,#44064,.T.) ;
#58790=ORIENTED_EDGE('',*,*,#43981,.F.) ;
#58791=ORIENTED_EDGE('',*,*,#44065,.T.) ;
#58792=ORIENTED_EDGE('',*,*,#44066,.F.) ;
#58793=ORIENTED_EDGE('',*,*,#43781,.F.) ;
#58794=ORIENTED_EDGE('',*,*,#44067,.F.) ;
#58795=ORIENTED_EDGE('',*,*,#43892,.F.) ;
#58796=ORIENTED_EDGE('',*,*,#44067,.T.) ;
#58797=ORIENTED_EDGE('',*,*,#43780,.T.) ;
#58798=ORIENTED_EDGE('',*,*,#44068,.F.) ;
#58799=ORIENTED_EDGE('',*,*,#44069,.F.) ;
#58800=ORIENTED_EDGE('',*,*,#43782,.T.) ;
#58801=ORIENTED_EDGE('',*,*,#44066,.T.) ;
#58802=ORIENTED_EDGE('',*,*,#44070,.F.) ;
#58803=ORIENTED_EDGE('',*,*,#44071,.F.) ;
#58804=ORIENTED_EDGE('',*,*,#44068,.T.) ;
#58805=ORIENTED_EDGE('',*,*,#43779,.F.) ;
#58806=ORIENTED_EDGE('',*,*,#44072,.F.) ;
#58807=ORIENTED_EDGE('',*,*,#43904,.F.) ;
#58808=ORIENTED_EDGE('',*,*,#44069,.T.) ;
#58809=ORIENTED_EDGE('',*,*,#43903,.F.) ;
#58810=ORIENTED_EDGE('',*,*,#44073,.F.) ;
#58811=ORIENTED_EDGE('',*,*,#43889,.F.) ;
#58812=ORIENTED_EDGE('',*,*,#44074,.F.) ;
#58813=ORIENTED_EDGE('',*,*,#43890,.F.) ;
#58814=ORIENTED_EDGE('',*,*,#44075,.F.) ;
#58815=ORIENTED_EDGE('',*,*,#43908,.F.) ;
#58816=ORIENTED_EDGE('',*,*,#44070,.T.) ;
#58817=ORIENTED_EDGE('',*,*,#43891,.F.) ;
#58818=ORIENTED_EDGE('',*,*,#44076,.F.) ;
#58819=ORIENTED_EDGE('',*,*,#43896,.F.) ;
#58820=ORIENTED_EDGE('',*,*,#44071,.T.) ;
#58821=ORIENTED_EDGE('',*,*,#43895,.F.) ;
#58822=ORIENTED_EDGE('',*,*,#44077,.F.) ;
#58823=ORIENTED_EDGE('',*,*,#43783,.F.) ;
#58824=ORIENTED_EDGE('',*,*,#44078,.F.) ;
#58825=ORIENTED_EDGE('',*,*,#43777,.F.) ;
#58826=ORIENTED_EDGE('',*,*,#44079,.F.) ;
#58827=ORIENTED_EDGE('',*,*,#43899,.F.) ;
#58828=ORIENTED_EDGE('',*,*,#43778,.T.) ;
#58829=ORIENTED_EDGE('',*,*,#44078,.T.) ;
#58830=ORIENTED_EDGE('',*,*,#44080,.F.) ;
#58831=ORIENTED_EDGE('',*,*,#44072,.T.) ;
#58832=ORIENTED_EDGE('',*,*,#44075,.T.) ;
#58833=ORIENTED_EDGE('',*,*,#44073,.T.) ;
#58834=ORIENTED_EDGE('',*,*,#44081,.F.) ;
#58835=ORIENTED_EDGE('',*,*,#44076,.T.) ;
#58836=ORIENTED_EDGE('',*,*,#44074,.T.) ;
#58837=ORIENTED_EDGE('',*,*,#44082,.F.) ;
#58838=ORIENTED_EDGE('',*,*,#43776,.T.) ;
#58839=ORIENTED_EDGE('',*,*,#44077,.T.) ;
#58840=ORIENTED_EDGE('',*,*,#44083,.F.) ;
#58841=ORIENTED_EDGE('',*,*,#44079,.T.) ;
#58842=ORIENTED_EDGE('',*,*,#44080,.T.) ;
#58843=ORIENTED_EDGE('',*,*,#43898,.F.) ;
#58844=ORIENTED_EDGE('',*,*,#44084,.F.) ;
#58845=ORIENTED_EDGE('',*,*,#43901,.F.) ;
#58846=ORIENTED_EDGE('',*,*,#44081,.T.) ;
#58847=ORIENTED_EDGE('',*,*,#43902,.F.) ;
#58848=ORIENTED_EDGE('',*,*,#44085,.F.) ;
#58849=ORIENTED_EDGE('',*,*,#43905,.F.) ;
#58850=ORIENTED_EDGE('',*,*,#44082,.T.) ;
#58851=ORIENTED_EDGE('',*,*,#43907,.F.) ;
#58852=ORIENTED_EDGE('',*,*,#44086,.F.) ;
#58853=ORIENTED_EDGE('',*,*,#43893,.F.) ;
#58854=ORIENTED_EDGE('',*,*,#44083,.T.) ;
#58855=ORIENTED_EDGE('',*,*,#43894,.F.) ;
#58856=ORIENTED_EDGE('',*,*,#44087,.F.) ;
#58857=ORIENTED_EDGE('',*,*,#43900,.F.) ;
#58858=ORIENTED_EDGE('',*,*,#44085,.T.) ;
#58859=ORIENTED_EDGE('',*,*,#44084,.T.) ;
#58860=ORIENTED_EDGE('',*,*,#44088,.F.) ;
#58861=ORIENTED_EDGE('',*,*,#44087,.T.) ;
#58862=ORIENTED_EDGE('',*,*,#44086,.T.) ;
#58863=ORIENTED_EDGE('',*,*,#44089,.F.) ;
#58864=ORIENTED_EDGE('',*,*,#44088,.T.) ;
#58865=ORIENTED_EDGE('',*,*,#43897,.F.) ;
#58866=ORIENTED_EDGE('',*,*,#44089,.T.) ;
#58867=ORIENTED_EDGE('',*,*,#43906,.F.) ;
#58868=ORIENTED_EDGE('',*,*,#44090,.F.) ;
#58869=ORIENTED_EDGE('',*,*,#43747,.F.) ;
#58870=ORIENTED_EDGE('',*,*,#44091,.F.) ;
#58871=ORIENTED_EDGE('',*,*,#43951,.F.) ;
#58872=ORIENTED_EDGE('',*,*,#44091,.T.) ;
#58873=ORIENTED_EDGE('',*,*,#43746,.T.) ;
#58874=ORIENTED_EDGE('',*,*,#44092,.F.) ;
#58875=ORIENTED_EDGE('',*,*,#44093,.F.) ;
#58876=ORIENTED_EDGE('',*,*,#43748,.T.) ;
#58877=ORIENTED_EDGE('',*,*,#44090,.T.) ;
#58878=ORIENTED_EDGE('',*,*,#44094,.F.) ;
#58879=ORIENTED_EDGE('',*,*,#44095,.F.) ;
#58880=ORIENTED_EDGE('',*,*,#44092,.T.) ;
#58881=ORIENTED_EDGE('',*,*,#43745,.F.) ;
#58882=ORIENTED_EDGE('',*,*,#44096,.F.) ;
#58883=ORIENTED_EDGE('',*,*,#43947,.F.) ;
#58884=ORIENTED_EDGE('',*,*,#44093,.T.) ;
#58885=ORIENTED_EDGE('',*,*,#43946,.F.) ;
#58886=ORIENTED_EDGE('',*,*,#44097,.F.) ;
#58887=ORIENTED_EDGE('',*,*,#43948,.F.) ;
#58888=ORIENTED_EDGE('',*,*,#44098,.F.) ;
#58889=ORIENTED_EDGE('',*,*,#43949,.F.) ;
#58890=ORIENTED_EDGE('',*,*,#44099,.F.) ;
#58891=ORIENTED_EDGE('',*,*,#43959,.F.) ;
#58892=ORIENTED_EDGE('',*,*,#44094,.T.) ;
#58893=ORIENTED_EDGE('',*,*,#43950,.F.) ;
#58894=ORIENTED_EDGE('',*,*,#44100,.F.) ;
#58895=ORIENTED_EDGE('',*,*,#43955,.F.) ;
#58896=ORIENTED_EDGE('',*,*,#44095,.T.) ;
#58897=ORIENTED_EDGE('',*,*,#43954,.F.) ;
#58898=ORIENTED_EDGE('',*,*,#44101,.F.) ;
#58899=ORIENTED_EDGE('',*,*,#43749,.F.) ;
#58900=ORIENTED_EDGE('',*,*,#44102,.F.) ;
#58901=ORIENTED_EDGE('',*,*,#43743,.F.) ;
#58902=ORIENTED_EDGE('',*,*,#44103,.F.) ;
#58903=ORIENTED_EDGE('',*,*,#43942,.F.) ;
#58904=ORIENTED_EDGE('',*,*,#43744,.T.) ;
#58905=ORIENTED_EDGE('',*,*,#44102,.T.) ;
#58906=ORIENTED_EDGE('',*,*,#44104,.F.) ;
#58907=ORIENTED_EDGE('',*,*,#44096,.T.) ;
#58908=ORIENTED_EDGE('',*,*,#44099,.T.) ;
#58909=ORIENTED_EDGE('',*,*,#44097,.T.) ;
#58910=ORIENTED_EDGE('',*,*,#44105,.F.) ;
#58911=ORIENTED_EDGE('',*,*,#44100,.T.) ;
#58912=ORIENTED_EDGE('',*,*,#44098,.T.) ;
#58913=ORIENTED_EDGE('',*,*,#44106,.F.) ;
#58914=ORIENTED_EDGE('',*,*,#43742,.T.) ;
#58915=ORIENTED_EDGE('',*,*,#44101,.T.) ;
#58916=ORIENTED_EDGE('',*,*,#44107,.F.) ;
#58917=ORIENTED_EDGE('',*,*,#44103,.T.) ;
#58918=ORIENTED_EDGE('',*,*,#44104,.T.) ;
#58919=ORIENTED_EDGE('',*,*,#43941,.F.) ;
#58920=ORIENTED_EDGE('',*,*,#44108,.F.) ;
#58921=ORIENTED_EDGE('',*,*,#43944,.F.) ;
#58922=ORIENTED_EDGE('',*,*,#44105,.T.) ;
#58923=ORIENTED_EDGE('',*,*,#43945,.F.) ;
#58924=ORIENTED_EDGE('',*,*,#44109,.F.) ;
#58925=ORIENTED_EDGE('',*,*,#43956,.F.) ;
#58926=ORIENTED_EDGE('',*,*,#44106,.T.) ;
#58927=ORIENTED_EDGE('',*,*,#43958,.F.) ;
#58928=ORIENTED_EDGE('',*,*,#44110,.F.) ;
#58929=ORIENTED_EDGE('',*,*,#43952,.F.) ;
#58930=ORIENTED_EDGE('',*,*,#44107,.T.) ;
#58931=ORIENTED_EDGE('',*,*,#43953,.F.) ;
#58932=ORIENTED_EDGE('',*,*,#44111,.F.) ;
#58933=ORIENTED_EDGE('',*,*,#43943,.F.) ;
#58934=ORIENTED_EDGE('',*,*,#44109,.T.) ;
#58935=ORIENTED_EDGE('',*,*,#44108,.T.) ;
#58936=ORIENTED_EDGE('',*,*,#44112,.F.) ;
#58937=ORIENTED_EDGE('',*,*,#44111,.T.) ;
#58938=ORIENTED_EDGE('',*,*,#44110,.T.) ;
#58939=ORIENTED_EDGE('',*,*,#44113,.F.) ;
#58940=ORIENTED_EDGE('',*,*,#44112,.T.) ;
#58941=ORIENTED_EDGE('',*,*,#43940,.F.) ;
#58942=ORIENTED_EDGE('',*,*,#44113,.T.) ;
#58943=ORIENTED_EDGE('',*,*,#43957,.F.) ;
#58944=ORIENTED_EDGE('',*,*,#43799,.F.) ;
#58945=ORIENTED_EDGE('',*,*,#44114,.T.) ;
#58946=ORIENTED_EDGE('',*,*,#44003,.F.) ;
#58947=ORIENTED_EDGE('',*,*,#44115,.F.) ;
#58948=ORIENTED_EDGE('',*,*,#43806,.F.) ;
#58949=ORIENTED_EDGE('',*,*,#43800,.F.) ;
#58950=ORIENTED_EDGE('',*,*,#44116,.F.) ;
#58951=ORIENTED_EDGE('',*,*,#43681,.F.) ;
#58952=ORIENTED_EDGE('',*,*,#44116,.T.) ;
#58953=ORIENTED_EDGE('',*,*,#44115,.T.) ;
#58954=ORIENTED_EDGE('',*,*,#44117,.F.) ;
#58955=ORIENTED_EDGE('',*,*,#44117,.T.) ;
#58956=ORIENTED_EDGE('',*,*,#44008,.F.) ;
#58957=ORIENTED_EDGE('',*,*,#44118,.F.) ;
#58958=ORIENTED_EDGE('',*,*,#43682,.F.) ;
#58959=ORIENTED_EDGE('',*,*,#43807,.F.) ;
#58960=ORIENTED_EDGE('',*,*,#43683,.F.) ;
#58961=ORIENTED_EDGE('',*,*,#44119,.F.) ;
#58962=ORIENTED_EDGE('',*,*,#43692,.F.) ;
#58963=ORIENTED_EDGE('',*,*,#44119,.T.) ;
#58964=ORIENTED_EDGE('',*,*,#44118,.T.) ;
#58965=ORIENTED_EDGE('',*,*,#44120,.F.) ;
#58966=ORIENTED_EDGE('',*,*,#43693,.T.) ;
#58967=ORIENTED_EDGE('',*,*,#44120,.T.) ;
#58968=ORIENTED_EDGE('',*,*,#44007,.F.) ;
#58969=ORIENTED_EDGE('',*,*,#44121,.F.) ;
#58970=ORIENTED_EDGE('',*,*,#43694,.F.) ;
#58971=ORIENTED_EDGE('',*,*,#43839,.F.) ;
#58972=ORIENTED_EDGE('',*,*,#43696,.F.) ;
#58973=ORIENTED_EDGE('',*,*,#44122,.F.) ;
#58974=ORIENTED_EDGE('',*,*,#43804,.F.) ;
#58975=ORIENTED_EDGE('',*,*,#43695,.T.) ;
#58976=ORIENTED_EDGE('',*,*,#44121,.T.) ;
#58977=ORIENTED_EDGE('',*,*,#44123,.F.) ;
#58978=ORIENTED_EDGE('',*,*,#44122,.T.) ;
#58979=ORIENTED_EDGE('',*,*,#44123,.T.) ;
#58980=ORIENTED_EDGE('',*,*,#44006,.F.) ;
#58981=ORIENTED_EDGE('',*,*,#44124,.F.) ;
#58982=ORIENTED_EDGE('',*,*,#43801,.F.) ;
#58983=ORIENTED_EDGE('',*,*,#43840,.F.) ;
#58984=ORIENTED_EDGE('',*,*,#43802,.F.) ;
#58985=ORIENTED_EDGE('',*,*,#44125,.F.) ;
#58986=ORIENTED_EDGE('',*,*,#43679,.F.) ;
#58987=ORIENTED_EDGE('',*,*,#44125,.T.) ;
#58988=ORIENTED_EDGE('',*,*,#44124,.T.) ;
#58989=ORIENTED_EDGE('',*,*,#44126,.F.) ;
#58990=ORIENTED_EDGE('',*,*,#44005,.F.) ;
#58991=ORIENTED_EDGE('',*,*,#44127,.T.) ;
#58992=ORIENTED_EDGE('',*,*,#43676,.F.) ;
#58993=ORIENTED_EDGE('',*,*,#44126,.T.) ;
#58994=ORIENTED_EDGE('',*,*,#43822,.F.) ;
#58995=ORIENTED_EDGE('',*,*,#43785,.F.) ;
#58996=ORIENTED_EDGE('',*,*,#43824,.F.) ;
#58997=ORIENTED_EDGE('',*,*,#43794,.F.) ;
#58998=ORIENTED_EDGE('',*,*,#43821,.F.) ;
#58999=ORIENTED_EDGE('',*,*,#43773,.F.) ;
#59000=ORIENTED_EDGE('',*,*,#43825,.F.) ;
#59001=ORIENTED_EDGE('',*,*,#43787,.F.) ;
#59002=ORIENTED_EDGE('',*,*,#43820,.F.) ;
#59003=ORIENTED_EDGE('',*,*,#43761,.F.) ;
#59004=ORIENTED_EDGE('',*,*,#43826,.F.) ;
#59005=ORIENTED_EDGE('',*,*,#43775,.F.) ;
#59006=ORIENTED_EDGE('',*,*,#43819,.F.) ;
#59007=ORIENTED_EDGE('',*,*,#43758,.F.) ;
#59008=ORIENTED_EDGE('',*,*,#43827,.F.) ;
#59009=ORIENTED_EDGE('',*,*,#43763,.F.) ;
#59010=ORIENTED_EDGE('',*,*,#43818,.F.) ;
#59011=ORIENTED_EDGE('',*,*,#43751,.F.) ;
#59012=ORIENTED_EDGE('',*,*,#43828,.F.) ;
#59013=ORIENTED_EDGE('',*,*,#43756,.F.) ;
#59014=ORIENTED_EDGE('',*,*,#43817,.F.) ;
#59015=ORIENTED_EDGE('',*,*,#43739,.F.) ;
#59016=ORIENTED_EDGE('',*,*,#43829,.F.) ;
#59017=ORIENTED_EDGE('',*,*,#43753,.F.) ;
#59018=ORIENTED_EDGE('',*,*,#43661,.F.) ;
#59019=ORIENTED_EDGE('',*,*,#43936,.F.) ;
#59020=ORIENTED_EDGE('',*,*,#43671,.F.) ;
#59021=ORIENTED_EDGE('',*,*,#43938,.F.) ;
#59022=ORIENTED_EDGE('',*,*,#43669,.F.) ;
#59023=ORIENTED_EDGE('',*,*,#43934,.F.) ;
#59024=ORIENTED_EDGE('',*,*,#43663,.F.) ;
#59025=ORIENTED_EDGE('',*,*,#43939,.F.) ;
#59026=ORIENTED_EDGE('',*,*,#43659,.F.) ;
#59027=ORIENTED_EDGE('',*,*,#43688,.F.) ;
#59028=ORIENTED_EDGE('',*,*,#43673,.F.) ;
#59029=ORIENTED_EDGE('',*,*,#43937,.F.) ;
#59030=ORIENTED_EDGE('',*,*,#43667,.F.) ;
#59031=ORIENTED_EDGE('',*,*,#43933,.F.) ;
#59032=ORIENTED_EDGE('',*,*,#43665,.F.) ;
#59033=ORIENTED_EDGE('',*,*,#43935,.F.) ;
#59034=ORIENTED_EDGE('',*,*,#43816,.F.) ;
#59035=ORIENTED_EDGE('',*,*,#43735,.F.) ;
#59036=ORIENTED_EDGE('',*,*,#43830,.F.) ;
#59037=ORIENTED_EDGE('',*,*,#43741,.F.) ;
#59038=ORIENTED_EDGE('',*,*,#43815,.F.) ;
#59039=ORIENTED_EDGE('',*,*,#43731,.F.) ;
#59040=ORIENTED_EDGE('',*,*,#43831,.F.) ;
#59041=ORIENTED_EDGE('',*,*,#43737,.F.) ;
#59042=ORIENTED_EDGE('',*,*,#43814,.F.) ;
#59043=ORIENTED_EDGE('',*,*,#43727,.F.) ;
#59044=ORIENTED_EDGE('',*,*,#43832,.F.) ;
#59045=ORIENTED_EDGE('',*,*,#43733,.F.) ;
#59046=ORIENTED_EDGE('',*,*,#43813,.F.) ;
#59047=ORIENTED_EDGE('',*,*,#43723,.F.) ;
#59048=ORIENTED_EDGE('',*,*,#43833,.F.) ;
#59049=ORIENTED_EDGE('',*,*,#43729,.F.) ;
#59050=ORIENTED_EDGE('',*,*,#43812,.F.) ;
#59051=ORIENTED_EDGE('',*,*,#43719,.F.) ;
#59052=ORIENTED_EDGE('',*,*,#43834,.F.) ;
#59053=ORIENTED_EDGE('',*,*,#43725,.F.) ;
#59054=ORIENTED_EDGE('',*,*,#43811,.F.) ;
#59055=ORIENTED_EDGE('',*,*,#43715,.F.) ;
#59056=ORIENTED_EDGE('',*,*,#43835,.F.) ;
#59057=ORIENTED_EDGE('',*,*,#43721,.F.) ;
#59058=ORIENTED_EDGE('',*,*,#43810,.F.) ;
#59059=ORIENTED_EDGE('',*,*,#43713,.F.) ;
#59060=ORIENTED_EDGE('',*,*,#43836,.F.) ;
#59061=ORIENTED_EDGE('',*,*,#43717,.F.) ;
#59062=ORIENTED_EDGE('',*,*,#44128,.F.) ;
#59063=ORIENTED_EDGE('',*,*,#43650,.F.) ;
#59064=ORIENTED_EDGE('',*,*,#44052,.F.) ;
#59065=ORIENTED_EDGE('',*,*,#44128,.T.) ;
#59066=ORIENTED_EDGE('',*,*,#44000,.F.) ;
#59067=ORIENTED_EDGE('',*,*,#44129,.F.) ;
#59068=ORIENTED_EDGE('',*,*,#43995,.F.) ;
#59069=ORIENTED_EDGE('',*,*,#44129,.T.) ;
#59070=ORIENTED_EDGE('',*,*,#43999,.F.) ;
#59071=ORIENTED_EDGE('',*,*,#44130,.F.) ;
#59072=ORIENTED_EDGE('',*,*,#44057,.F.) ;
#59073=ORIENTED_EDGE('',*,*,#44130,.T.) ;
#59074=ORIENTED_EDGE('',*,*,#44050,.F.) ;
#59075=ORIENTED_EDGE('',*,*,#44131,.F.) ;
#59076=ORIENTED_EDGE('',*,*,#44055,.F.) ;
#59077=ORIENTED_EDGE('',*,*,#44131,.T.) ;
#59078=ORIENTED_EDGE('',*,*,#43708,.F.) ;
#59079=ORIENTED_EDGE('',*,*,#44132,.F.) ;
#59080=ORIENTED_EDGE('',*,*,#44056,.F.) ;
#59081=ORIENTED_EDGE('',*,*,#44132,.T.) ;
#59082=ORIENTED_EDGE('',*,*,#43707,.F.) ;
#59083=ORIENTED_EDGE('',*,*,#43809,.F.) ;
#59084=ORIENTED_EDGE('',*,*,#43703,.F.) ;
#59085=ORIENTED_EDGE('',*,*,#43837,.F.) ;
#59086=ORIENTED_EDGE('',*,*,#43711,.F.) ;
#59087=ORIENTED_EDGE('',*,*,#44133,.F.) ;
#59088=ORIENTED_EDGE('',*,*,#43685,.F.) ;
#59089=ORIENTED_EDGE('',*,*,#44133,.T.) ;
#59090=ORIENTED_EDGE('',*,*,#43710,.F.) ;
#59091=ORIENTED_EDGE('',*,*,#44134,.F.) ;
#59092=ORIENTED_EDGE('',*,*,#44045,.F.) ;
#59093=ORIENTED_EDGE('',*,*,#44134,.T.) ;
#59094=ORIENTED_EDGE('',*,*,#44051,.F.) ;
#59095=ORIENTED_EDGE('',*,*,#43626,.F.) ;
#59096=ORIENTED_EDGE('',*,*,#44046,.F.) ;
#59097=ORIENTED_EDGE('',*,*,#44135,.F.) ;
#59098=ORIENTED_EDGE('',*,*,#43989,.F.) ;
#59099=ORIENTED_EDGE('',*,*,#43624,.T.) ;
#59100=ORIENTED_EDGE('',*,*,#44002,.F.) ;
#59101=ORIENTED_EDGE('',*,*,#44053,.F.) ;
#59102=ORIENTED_EDGE('',*,*,#44047,.F.) ;
#59103=ORIENTED_EDGE('',*,*,#44135,.T.) ;
#59104=ORIENTED_EDGE('',*,*,#44136,.T.) ;
#59105=ORIENTED_EDGE('',*,*,#44137,.T.) ;
#59106=ORIENTED_EDGE('',*,*,#44004,.F.) ;
#59107=ORIENTED_EDGE('',*,*,#44138,.T.) ;
#59108=ORIENTED_EDGE('',*,*,#44139,.T.) ;
#59109=ORIENTED_EDGE('',*,*,#43805,.F.) ;
#59110=ORIENTED_EDGE('',*,*,#43792,.F.) ;
#59111=ORIENTED_EDGE('',*,*,#44140,.F.) ;
#59112=ORIENTED_EDGE('',*,*,#43798,.F.) ;
#59113=ORIENTED_EDGE('',*,*,#43791,.F.) ;
#59114=ORIENTED_EDGE('',*,*,#44141,.T.) ;
#59115=ORIENTED_EDGE('',*,*,#44114,.F.) ;
#59116=ORIENTED_EDGE('',*,*,#44140,.T.) ;
#59117=ORIENTED_EDGE('',*,*,#43823,.F.) ;
#59118=ORIENTED_EDGE('',*,*,#43677,.F.) ;
#59119=ORIENTED_EDGE('',*,*,#44142,.F.) ;
#59120=ORIENTED_EDGE('',*,*,#43796,.F.) ;
#59121=ORIENTED_EDGE('',*,*,#44127,.F.) ;
#59122=ORIENTED_EDGE('',*,*,#44143,.T.) ;
#59123=ORIENTED_EDGE('',*,*,#43788,.F.) ;
#59124=ORIENTED_EDGE('',*,*,#44142,.T.) ;
#59125=ORIENTED_EDGE('',*,*,#44138,.F.) ;
#59126=ORIENTED_EDGE('',*,*,#44141,.F.) ;
#59127=ORIENTED_EDGE('',*,*,#44144,.F.) ;
#59128=ORIENTED_EDGE('',*,*,#44145,.F.) ;
#59129=ORIENTED_EDGE('',*,*,#44139,.F.) ;
#59130=ORIENTED_EDGE('',*,*,#44144,.T.) ;
#59131=ORIENTED_EDGE('',*,*,#43790,.F.) ;
#59132=ORIENTED_EDGE('',*,*,#44145,.T.) ;
#59133=ORIENTED_EDGE('',*,*,#43789,.F.) ;
#59134=ORIENTED_EDGE('',*,*,#44146,.F.) ;
#59135=ORIENTED_EDGE('',*,*,#44136,.F.) ;
#59136=ORIENTED_EDGE('',*,*,#44146,.T.) ;
#59137=ORIENTED_EDGE('',*,*,#44143,.F.) ;
#59138=ORIENTED_EDGE('',*,*,#44137,.F.) ;
#78907=TOROIDAL_SURFACE('',#91124,0.2,0.1) ;
#78908=TOROIDAL_SURFACE('',#91129,2.,0.1) ;
#78909=TOROIDAL_SURFACE('',#91134,1.4,0.1) ;
#78910=TOROIDAL_SURFACE('',#91138,1.6,0.1) ;
#78911=TOROIDAL_SURFACE('',#91143,0.2,0.1) ;
#78912=TOROIDAL_SURFACE('',#91167,0.2,0.1) ;
#78913=TOROIDAL_SURFACE('',#91175,2.,0.1) ;
#78914=TOROIDAL_SURFACE('',#91180,1.4,0.1) ;
#78915=TOROIDAL_SURFACE('',#91184,1.6,0.1) ;
#78916=TOROIDAL_SURFACE('',#91189,0.2,0.1) ;
#78917=TOROIDAL_SURFACE('',#91443,0.2,0.1) ;
#78918=TOROIDAL_SURFACE('',#91470,0.2,0.1) ;
#78919=TOROIDAL_SURFACE('',#91473,0.2,0.1) ;
#78920=TOROIDAL_SURFACE('',#91490,0.2,0.1) ;
#78921=TOROIDAL_SURFACE('',#91496,0.2,0.1) ;
#78922=TOROIDAL_SURFACE('',#91514,0.2,0.1) ;
#78923=TOROIDAL_SURFACE('',#91517,0.2,0.1) ;
#78924=TOROIDAL_SURFACE('',#91534,0.2,0.1) ;
#78925=TOROIDAL_SURFACE('',#91540,0.2,0.1) ;
#78926=TOROIDAL_SURFACE('',#91555,3.1,0.1) ;
#78927=TOROIDAL_SURFACE('',#91565,0.2,0.1) ;
#78928=TOROIDAL_SURFACE('',#91567,2.9,0.1) ;
#78929=TOROIDAL_SURFACE('',#91572,0.2,0.1) ;
#78930=TOROIDAL_SURFACE('',#91581,3.1,0.1) ;
#78931=TOROIDAL_SURFACE('',#91608,0.2,0.1) ;
#78932=TOROIDAL_SURFACE('',#91620,2.9,0.1) ;
#78933=TOROIDAL_SURFACE('',#91808,0.2,0.1) ;
#78934=TOROIDAL_SURFACE('',#91834,0.2,0.1) ;
#78935=TOROIDAL_SURFACE('',#91837,0.2,0.1) ;
#78936=TOROIDAL_SURFACE('',#91854,0.2,0.1) ;
#78937=TOROIDAL_SURFACE('',#91860,0.2,0.1) ;
#78938=TOROIDAL_SURFACE('',#91878,0.2,0.1) ;
#78939=TOROIDAL_SURFACE('',#91881,0.2,0.1) ;
#78940=TOROIDAL_SURFACE('',#91898,0.2,0.1) ;
#78941=TOROIDAL_SURFACE('',#91904,0.2,0.1) ;
#78942=TOROIDAL_SURFACE('',#91919,3.1,0.1) ;
#78943=TOROIDAL_SURFACE('',#91925,0.2,0.1) ;
#78944=TOROIDAL_SURFACE('',#91927,2.9,0.1) ;
#78945=TOROIDAL_SURFACE('',#91931,0.2,0.1) ;
#78946=TOROIDAL_SURFACE('',#91939,3.1,0.1) ;
#78947=TOROIDAL_SURFACE('',#91948,0.2,0.1) ;
#78948=TOROIDAL_SURFACE('',#91957,2.9,0.1) ;
#78949=TOROIDAL_SURFACE('',#91994,0.199999999999999,0.1) ;
#78950=TOROIDAL_SURFACE('',#91998,0.199999999999999,0.1) ;
#78951=TOROIDAL_SURFACE('',#92008,0.2,0.1) ;
#78952=TOROIDAL_SURFACE('',#92010,0.2,0.1) ;
#78953=TOROIDAL_SURFACE('',#92013,0.2,0.1) ;
#78954=TOROIDAL_SURFACE('',#92018,2.,0.1) ;
#78955=TOROIDAL_SURFACE('',#92023,1.4,0.1) ;
#78956=TOROIDAL_SURFACE('',#92027,1.6,0.1) ;
#78957=TOROIDAL_SURFACE('',#92032,0.2,0.1) ;
#78958=TOROIDAL_SURFACE('',#92056,0.2,0.1) ;
#78959=TOROIDAL_SURFACE('',#92064,2.,0.1) ;
#78960=TOROIDAL_SURFACE('',#92069,1.4,0.1) ;
#78961=TOROIDAL_SURFACE('',#92073,1.6,0.1) ;
#78962=TOROIDAL_SURFACE('',#92078,0.2,0.1) ;
#78963=TOROIDAL_SURFACE('',#92332,0.2,0.1) ;
#78964=TOROIDAL_SURFACE('',#92359,0.2,0.1) ;
#78965=TOROIDAL_SURFACE('',#92362,0.2,0.1) ;
#78966=TOROIDAL_SURFACE('',#92379,0.2,0.1) ;
#78967=TOROIDAL_SURFACE('',#92385,0.2,0.1) ;
#78968=TOROIDAL_SURFACE('',#92403,0.2,0.1) ;
#78969=TOROIDAL_SURFACE('',#92406,0.2,0.1) ;
#78970=TOROIDAL_SURFACE('',#92423,0.2,0.1) ;
#78971=TOROIDAL_SURFACE('',#92429,0.2,0.1) ;
#78972=TOROIDAL_SURFACE('',#92444,3.1,0.1) ;
#78973=TOROIDAL_SURFACE('',#92456,0.2,0.1) ;
#78974=TOROIDAL_SURFACE('',#92458,2.9,0.1) ;
#78975=TOROIDAL_SURFACE('',#92462,0.2,0.1) ;
#78976=TOROIDAL_SURFACE('',#92470,3.1,0.1) ;
#78977=TOROIDAL_SURFACE('',#92497,0.2,0.1) ;
#78978=TOROIDAL_SURFACE('',#92509,2.9,0.1) ;
#78979=TOROIDAL_SURFACE('',#92696,0.2,0.1) ;
#78980=TOROIDAL_SURFACE('',#92723,0.2,0.1) ;
#78981=TOROIDAL_SURFACE('',#92726,0.2,0.1) ;
#78982=TOROIDAL_SURFACE('',#92743,0.2,0.1) ;
#78983=TOROIDAL_SURFACE('',#92749,0.2,0.1) ;
#78984=TOROIDAL_SURFACE('',#92767,0.2,0.1) ;
#78985=TOROIDAL_SURFACE('',#92770,0.2,0.1) ;
#78986=TOROIDAL_SURFACE('',#92787,0.2,0.1) ;
#78987=TOROIDAL_SURFACE('',#92793,0.2,0.1) ;
#78988=TOROIDAL_SURFACE('',#92808,3.1,0.1) ;
#78989=TOROIDAL_SURFACE('',#92818,0.2,0.1) ;
#78990=TOROIDAL_SURFACE('',#92820,2.9,0.1) ;
#78991=TOROIDAL_SURFACE('',#92822,0.2,0.1) ;
#78992=TOROIDAL_SURFACE('',#92828,3.1,0.1) ;
#78993=TOROIDAL_SURFACE('',#92837,0.2,0.1) ;
#78994=TOROIDAL_SURFACE('',#92846,2.9,0.1) ;
#78995=TOROIDAL_SURFACE('',#92883,0.199999999999999,0.1) ;
#78996=TOROIDAL_SURFACE('',#92887,0.199999999999999,0.1) ;
#78997=TOROIDAL_SURFACE('',#92897,0.2,0.1) ;
#78998=TOROIDAL_SURFACE('',#92899,0.2,0.1) ;
#78999=TOROIDAL_SURFACE('',#92902,0.2,0.1) ;
#79000=TOROIDAL_SURFACE('',#92910,2.,0.1) ;
#79001=TOROIDAL_SURFACE('',#92915,1.4,0.1) ;
#79002=TOROIDAL_SURFACE('',#92919,1.6,0.1) ;
#79003=TOROIDAL_SURFACE('',#92924,0.2,0.1) ;
#79004=TOROIDAL_SURFACE('',#93171,0.2,0.1) ;
#79005=TOROIDAL_SURFACE('',#93198,0.2,0.1) ;
#79006=TOROIDAL_SURFACE('',#93201,0.2,0.1) ;
#79007=TOROIDAL_SURFACE('',#93218,0.2,0.1) ;
#79008=TOROIDAL_SURFACE('',#93224,0.2,0.1) ;
#79009=TOROIDAL_SURFACE('',#93242,0.2,0.1) ;
#79010=TOROIDAL_SURFACE('',#93245,0.2,0.1) ;
#79011=TOROIDAL_SURFACE('',#93262,0.2,0.1) ;
#79012=TOROIDAL_SURFACE('',#93268,0.2,0.1) ;
#79013=TOROIDAL_SURFACE('',#93283,3.1,0.1) ;
#79014=TOROIDAL_SURFACE('',#93293,0.2,0.1) ;
#79015=TOROIDAL_SURFACE('',#93295,2.9,0.1) ;
#79016=TOROIDAL_SURFACE('',#93299,0.2,0.1) ;
#79017=TOROIDAL_SURFACE('',#93307,3.1,0.1) ;
#79018=TOROIDAL_SURFACE('',#93329,0.2,0.1) ;
#79019=TOROIDAL_SURFACE('',#93340,2.9,0.1) ;
#79661=STYLED_ITEM('',(#170169),#85367) ;
#79662=STYLED_ITEM('',(#170169),#85368) ;
#79663=STYLED_ITEM('',(#170169),#85369) ;
#79664=STYLED_ITEM('',(#170169),#85370) ;
#79665=STYLED_ITEM('',(#170169),#85371) ;
#79666=STYLED_ITEM('',(#170169),#85372) ;
#79667=STYLED_ITEM('',(#170169),#85373) ;
#79668=STYLED_ITEM('',(#170169),#85374) ;
#79669=STYLED_ITEM('',(#170169),#85375) ;
#79670=STYLED_ITEM('',(#170169),#85376) ;
#79671=STYLED_ITEM('',(#170169),#85377) ;
#79672=STYLED_ITEM('',(#170169),#85378) ;
#79673=STYLED_ITEM('',(#170169),#85379) ;
#79674=STYLED_ITEM('',(#170169),#85380) ;
#79675=STYLED_ITEM('',(#170169),#85381) ;
#79676=STYLED_ITEM('',(#170169),#85382) ;
#79677=STYLED_ITEM('',(#170169),#85383) ;
#79678=STYLED_ITEM('',(#170169),#85384) ;
#79679=STYLED_ITEM('',(#170169),#85385) ;
#79680=STYLED_ITEM('',(#170169),#85386) ;
#79681=STYLED_ITEM('',(#170169),#85387) ;
#79682=STYLED_ITEM('',(#170169),#85388) ;
#79683=STYLED_ITEM('',(#170169),#85389) ;
#79684=STYLED_ITEM('',(#170169),#85390) ;
#79685=STYLED_ITEM('',(#170169),#85391) ;
#79686=STYLED_ITEM('',(#170169),#85392) ;
#79687=STYLED_ITEM('',(#170169),#85393) ;
#79688=STYLED_ITEM('',(#170169),#85394) ;
#79689=STYLED_ITEM('',(#170169),#85395) ;
#79690=STYLED_ITEM('',(#170169),#85396) ;
#79691=STYLED_ITEM('',(#170169),#85397) ;
#79692=STYLED_ITEM('',(#170169),#85398) ;
#79693=STYLED_ITEM('',(#170169),#85399) ;
#79694=STYLED_ITEM('',(#170169),#85400) ;
#79695=STYLED_ITEM('',(#170170),#85401) ;
#79696=STYLED_ITEM('',(#170169),#85402) ;
#79697=STYLED_ITEM('',(#170169),#85403) ;
#79698=STYLED_ITEM('',(#170169),#85404) ;
#79699=STYLED_ITEM('',(#170169),#85405) ;
#79700=STYLED_ITEM('',(#170169),#85406) ;
#79701=STYLED_ITEM('',(#170169),#85407) ;
#79702=STYLED_ITEM('',(#170169),#85408) ;
#79703=STYLED_ITEM('',(#170169),#85409) ;
#79704=STYLED_ITEM('',(#170169),#85410) ;
#79705=STYLED_ITEM('',(#170169),#85411) ;
#79706=STYLED_ITEM('',(#170169),#85412) ;
#79707=STYLED_ITEM('',(#170169),#85413) ;
#79708=STYLED_ITEM('',(#170169),#85414) ;
#79709=STYLED_ITEM('',(#170169),#85415) ;
#79710=STYLED_ITEM('',(#170169),#85416) ;
#79711=STYLED_ITEM('',(#170169),#85417) ;
#79712=STYLED_ITEM('',(#170169),#85418) ;
#79713=STYLED_ITEM('',(#170169),#85419) ;
#79714=STYLED_ITEM('',(#170169),#85420) ;
#79715=STYLED_ITEM('',(#170171),#85421) ;
#79716=STYLED_ITEM('',(#170169),#85422) ;
#79717=STYLED_ITEM('',(#170169),#85423) ;
#79718=STYLED_ITEM('',(#170169),#85424) ;
#79719=STYLED_ITEM('',(#170169),#85425) ;
#79720=STYLED_ITEM('',(#170169),#85426) ;
#79721=STYLED_ITEM('',(#170169),#85427) ;
#79722=STYLED_ITEM('',(#170169),#85428) ;
#79723=STYLED_ITEM('',(#170169),#85429) ;
#79724=STYLED_ITEM('',(#170169),#85430) ;
#79725=STYLED_ITEM('',(#170169),#85431) ;
#79726=STYLED_ITEM('',(#170169),#85432) ;
#79727=STYLED_ITEM('',(#170169),#85433) ;
#79728=STYLED_ITEM('',(#170169),#85434) ;
#79729=STYLED_ITEM('',(#170169),#85435) ;
#79730=STYLED_ITEM('',(#170169),#85436) ;
#79731=STYLED_ITEM('',(#170169),#85437) ;
#79732=STYLED_ITEM('',(#170169),#85438) ;
#79733=STYLED_ITEM('',(#170169),#85439) ;
#79734=STYLED_ITEM('',(#170169),#85440) ;
#79735=STYLED_ITEM('',(#170170),#85441) ;
#79736=STYLED_ITEM('',(#170170),#85442) ;
#79737=STYLED_ITEM('',(#170170),#85443) ;
#79738=STYLED_ITEM('',(#170170),#85444) ;
#79739=STYLED_ITEM('',(#170169),#85445) ;
#79740=STYLED_ITEM('',(#170169),#85446) ;
#79741=STYLED_ITEM('',(#170169),#85447) ;
#79742=STYLED_ITEM('',(#170169),#85448) ;
#79743=STYLED_ITEM('',(#170169),#85449) ;
#79744=STYLED_ITEM('',(#170169),#85450) ;
#79745=STYLED_ITEM('',(#170169),#85451) ;
#79746=STYLED_ITEM('',(#170169),#85452) ;
#79747=STYLED_ITEM('',(#170169),#85453) ;
#79748=STYLED_ITEM('',(#170169),#85454) ;
#79749=STYLED_ITEM('',(#170169),#85455) ;
#79750=STYLED_ITEM('',(#170169),#85456) ;
#79751=STYLED_ITEM('',(#170169),#85457) ;
#79752=STYLED_ITEM('',(#170169),#85458) ;
#79753=STYLED_ITEM('',(#170169),#85459) ;
#79754=STYLED_ITEM('',(#170169),#85460) ;
#79755=STYLED_ITEM('',(#170169),#85461) ;
#79756=STYLED_ITEM('',(#170169),#85462) ;
#79757=STYLED_ITEM('',(#170171),#85463) ;
#79758=STYLED_ITEM('',(#170169),#85464) ;
#79759=STYLED_ITEM('',(#170169),#85465) ;
#79760=STYLED_ITEM('',(#170169),#85466) ;
#79761=STYLED_ITEM('',(#170169),#85467) ;
#79762=STYLED_ITEM('',(#170169),#85468) ;
#79763=STYLED_ITEM('',(#170169),#85469) ;
#79764=STYLED_ITEM('',(#170169),#85470) ;
#79765=STYLED_ITEM('',(#170169),#85471) ;
#79766=STYLED_ITEM('',(#170169),#85472) ;
#79767=STYLED_ITEM('',(#170169),#85473) ;
#79768=STYLED_ITEM('',(#170169),#85474) ;
#79769=STYLED_ITEM('',(#170169),#85475) ;
#79770=STYLED_ITEM('',(#170169),#85476) ;
#79771=STYLED_ITEM('',(#170169),#85477) ;
#79772=STYLED_ITEM('',(#170169),#85478) ;
#79773=STYLED_ITEM('',(#170169),#85479) ;
#79774=STYLED_ITEM('',(#170169),#85480) ;
#79775=STYLED_ITEM('',(#170169),#85481) ;
#79776=STYLED_ITEM('',(#170169),#85482) ;
#79777=STYLED_ITEM('',(#170169),#85483) ;
#79778=STYLED_ITEM('',(#170169),#85485) ;
#79779=STYLED_ITEM('',(#170169),#85486) ;
#79780=STYLED_ITEM('',(#170169),#85487) ;
#79781=STYLED_ITEM('',(#170169),#85488) ;
#79782=STYLED_ITEM('',(#170169),#85489) ;
#79783=STYLED_ITEM('',(#170169),#85490) ;
#79784=STYLED_ITEM('',(#170169),#85491) ;
#79785=STYLED_ITEM('',(#170169),#85492) ;
#79786=STYLED_ITEM('',(#170169),#85493) ;
#79787=STYLED_ITEM('',(#170169),#85494) ;
#79788=STYLED_ITEM('',(#170169),#85495) ;
#79789=STYLED_ITEM('',(#170169),#85496) ;
#79790=STYLED_ITEM('',(#170169),#85497) ;
#79791=STYLED_ITEM('',(#170169),#85498) ;
#79792=STYLED_ITEM('',(#170169),#85499) ;
#79793=STYLED_ITEM('',(#170169),#85500) ;
#79794=STYLED_ITEM('',(#170169),#85501) ;
#79795=STYLED_ITEM('',(#170169),#85502) ;
#79796=STYLED_ITEM('',(#170169),#85503) ;
#79797=STYLED_ITEM('',(#170169),#85504) ;
#79798=STYLED_ITEM('',(#170169),#85505) ;
#79799=STYLED_ITEM('',(#170169),#85506) ;
#79800=STYLED_ITEM('',(#170169),#85507) ;
#79801=STYLED_ITEM('',(#170169),#85508) ;
#79802=STYLED_ITEM('',(#170169),#85509) ;
#79803=STYLED_ITEM('',(#170169),#85510) ;
#79804=STYLED_ITEM('',(#170169),#85511) ;
#79805=STYLED_ITEM('',(#170169),#85512) ;
#79806=STYLED_ITEM('',(#170169),#85513) ;
#79807=STYLED_ITEM('',(#170169),#85514) ;
#79808=STYLED_ITEM('',(#170169),#85515) ;
#79809=STYLED_ITEM('',(#170169),#85516) ;
#79810=STYLED_ITEM('',(#170169),#85517) ;
#79811=STYLED_ITEM('',(#170169),#85518) ;
#79812=STYLED_ITEM('',(#170169),#85519) ;
#79813=STYLED_ITEM('',(#170169),#85520) ;
#79814=STYLED_ITEM('',(#170169),#85521) ;
#79815=STYLED_ITEM('',(#170169),#85522) ;
#79816=STYLED_ITEM('',(#170169),#85523) ;
#79817=STYLED_ITEM('',(#170169),#85524) ;
#79818=STYLED_ITEM('',(#170169),#85525) ;
#79819=STYLED_ITEM('',(#170169),#85526) ;
#79820=STYLED_ITEM('',(#170169),#85527) ;
#79821=STYLED_ITEM('',(#170169),#85528) ;
#79822=STYLED_ITEM('',(#170169),#85529) ;
#79823=STYLED_ITEM('',(#170169),#85530) ;
#79824=STYLED_ITEM('',(#170169),#85531) ;
#79825=STYLED_ITEM('',(#170169),#85532) ;
#79826=STYLED_ITEM('',(#170169),#85533) ;
#79827=STYLED_ITEM('',(#170169),#85534) ;
#79828=STYLED_ITEM('',(#170169),#85535) ;
#79829=STYLED_ITEM('',(#170169),#85536) ;
#79830=STYLED_ITEM('',(#170169),#85537) ;
#79831=STYLED_ITEM('',(#170169),#85538) ;
#79832=STYLED_ITEM('',(#170169),#85539) ;
#79833=STYLED_ITEM('',(#170169),#85540) ;
#79834=STYLED_ITEM('',(#170169),#85541) ;
#79835=STYLED_ITEM('',(#170169),#85542) ;
#79836=STYLED_ITEM('',(#170169),#85543) ;
#79837=STYLED_ITEM('',(#170169),#85544) ;
#79838=STYLED_ITEM('',(#170169),#85545) ;
#79839=STYLED_ITEM('',(#170169),#85546) ;
#79840=STYLED_ITEM('',(#170169),#85547) ;
#79841=STYLED_ITEM('',(#170169),#85548) ;
#79842=STYLED_ITEM('',(#170169),#85549) ;
#79843=STYLED_ITEM('',(#170169),#85550) ;
#79844=STYLED_ITEM('',(#170169),#85551) ;
#79845=STYLED_ITEM('',(#170169),#85552) ;
#79846=STYLED_ITEM('',(#170169),#85553) ;
#79847=STYLED_ITEM('',(#170169),#85554) ;
#79848=STYLED_ITEM('',(#170169),#85555) ;
#79849=STYLED_ITEM('',(#170169),#85556) ;
#79850=STYLED_ITEM('',(#170169),#85557) ;
#79851=STYLED_ITEM('',(#170169),#85558) ;
#79852=STYLED_ITEM('',(#170169),#85559) ;
#79853=STYLED_ITEM('',(#170169),#85560) ;
#79854=STYLED_ITEM('',(#170169),#85561) ;
#79855=STYLED_ITEM('',(#170169),#85562) ;
#79856=STYLED_ITEM('',(#170169),#85563) ;
#79857=STYLED_ITEM('',(#170169),#85564) ;
#79858=STYLED_ITEM('',(#170169),#85565) ;
#79859=STYLED_ITEM('',(#170169),#85566) ;
#79860=STYLED_ITEM('',(#170169),#85567) ;
#79861=STYLED_ITEM('',(#170169),#85568) ;
#79862=STYLED_ITEM('',(#170169),#85569) ;
#79863=STYLED_ITEM('',(#170169),#85570) ;
#79864=STYLED_ITEM('',(#170169),#85571) ;
#79865=STYLED_ITEM('',(#170169),#85572) ;
#79866=STYLED_ITEM('',(#170169),#85573) ;
#79867=STYLED_ITEM('',(#170169),#85574) ;
#79868=STYLED_ITEM('',(#170170),#85575) ;
#79869=STYLED_ITEM('',(#170170),#85576) ;
#79870=STYLED_ITEM('',(#170170),#85577) ;
#79871=STYLED_ITEM('',(#170170),#85578) ;
#79872=STYLED_ITEM('',(#170169),#85579) ;
#79873=STYLED_ITEM('',(#170169),#85580) ;
#79874=STYLED_ITEM('',(#170169),#85581) ;
#79875=STYLED_ITEM('',(#170169),#85582) ;
#79876=STYLED_ITEM('',(#170169),#85583) ;
#79877=STYLED_ITEM('',(#170169),#85584) ;
#79878=STYLED_ITEM('',(#170169),#85585) ;
#79879=STYLED_ITEM('',(#170169),#85586) ;
#79880=STYLED_ITEM('',(#170169),#85587) ;
#79881=STYLED_ITEM('',(#170169),#85588) ;
#79882=STYLED_ITEM('',(#170169),#85589) ;
#79883=STYLED_ITEM('',(#170169),#85590) ;
#79884=STYLED_ITEM('',(#170169),#85591) ;
#79885=STYLED_ITEM('',(#170169),#85592) ;
#79886=STYLED_ITEM('',(#170169),#85593) ;
#79887=STYLED_ITEM('',(#170169),#85594) ;
#79888=STYLED_ITEM('',(#170169),#85595) ;
#79889=STYLED_ITEM('',(#170169),#85596) ;
#79890=STYLED_ITEM('',(#170169),#85597) ;
#79891=STYLED_ITEM('',(#170169),#85598) ;
#79892=STYLED_ITEM('',(#170169),#85599) ;
#79893=STYLED_ITEM('',(#170169),#85600) ;
#79894=STYLED_ITEM('',(#170169),#85601) ;
#79895=STYLED_ITEM('',(#170169),#85602) ;
#79896=STYLED_ITEM('',(#170169),#85603) ;
#79897=STYLED_ITEM('',(#170169),#85604) ;
#79898=STYLED_ITEM('',(#170169),#85605) ;
#79899=STYLED_ITEM('',(#170169),#85606) ;
#79900=STYLED_ITEM('',(#170169),#85607) ;
#79901=STYLED_ITEM('',(#170169),#85608) ;
#79902=STYLED_ITEM('',(#170169),#85609) ;
#79903=STYLED_ITEM('',(#170169),#85610) ;
#79904=STYLED_ITEM('',(#170169),#85611) ;
#79905=STYLED_ITEM('',(#170169),#85612) ;
#79906=STYLED_ITEM('',(#170169),#85613) ;
#79907=STYLED_ITEM('',(#170169),#85614) ;
#79908=STYLED_ITEM('',(#170169),#85615) ;
#79909=STYLED_ITEM('',(#170170),#85616) ;
#79910=STYLED_ITEM('',(#170169),#85617) ;
#79911=STYLED_ITEM('',(#170169),#85618) ;
#79912=STYLED_ITEM('',(#170169),#85619) ;
#79913=STYLED_ITEM('',(#170169),#85620) ;
#79914=STYLED_ITEM('',(#170169),#85621) ;
#79915=STYLED_ITEM('',(#170171),#85622) ;
#79916=STYLED_ITEM('',(#170169),#85623) ;
#79917=STYLED_ITEM('',(#170169),#85624) ;
#79918=STYLED_ITEM('',(#170169),#85625) ;
#79919=STYLED_ITEM('',(#170169),#85626) ;
#79920=STYLED_ITEM('',(#170169),#85627) ;
#79921=STYLED_ITEM('',(#170169),#85628) ;
#79922=STYLED_ITEM('',(#170169),#85629) ;
#79923=STYLED_ITEM('',(#170169),#85630) ;
#79924=STYLED_ITEM('',(#170169),#85631) ;
#79925=STYLED_ITEM('',(#170169),#85632) ;
#79926=STYLED_ITEM('',(#170169),#85633) ;
#79927=STYLED_ITEM('',(#170169),#85634) ;
#79928=STYLED_ITEM('',(#170169),#85635) ;
#79929=STYLED_ITEM('',(#170169),#85636) ;
#79930=STYLED_ITEM('',(#170169),#85637) ;
#79931=STYLED_ITEM('',(#170169),#85638) ;
#79932=STYLED_ITEM('',(#170169),#85639) ;
#79933=STYLED_ITEM('',(#170169),#85640) ;
#79934=STYLED_ITEM('',(#170169),#85641) ;
#79935=STYLED_ITEM('',(#170170),#85642) ;
#79936=STYLED_ITEM('',(#170170),#85643) ;
#79937=STYLED_ITEM('',(#170170),#85644) ;
#79938=STYLED_ITEM('',(#170170),#85645) ;
#79939=STYLED_ITEM('',(#170169),#85646) ;
#79940=STYLED_ITEM('',(#170169),#85647) ;
#79941=STYLED_ITEM('',(#170169),#85648) ;
#79942=STYLED_ITEM('',(#170169),#85649) ;
#79943=STYLED_ITEM('',(#170169),#85650) ;
#79944=STYLED_ITEM('',(#170169),#85651) ;
#79945=STYLED_ITEM('',(#170169),#85652) ;
#79946=STYLED_ITEM('',(#170169),#85653) ;
#79947=STYLED_ITEM('',(#170169),#85654) ;
#79948=STYLED_ITEM('',(#170169),#85655) ;
#79949=STYLED_ITEM('',(#170169),#85656) ;
#79950=STYLED_ITEM('',(#170169),#85657) ;
#79951=STYLED_ITEM('',(#170169),#85658) ;
#79952=STYLED_ITEM('',(#170169),#85659) ;
#79953=STYLED_ITEM('',(#170169),#85660) ;
#79954=STYLED_ITEM('',(#170169),#85661) ;
#79955=STYLED_ITEM('',(#170169),#85662) ;
#79956=STYLED_ITEM('',(#170169),#85663) ;
#79957=STYLED_ITEM('',(#170171),#85664) ;
#79958=STYLED_ITEM('',(#170169),#85665) ;
#79959=STYLED_ITEM('',(#170169),#85666) ;
#79960=STYLED_ITEM('',(#170169),#85667) ;
#79961=STYLED_ITEM('',(#170169),#85668) ;
#79962=STYLED_ITEM('',(#170169),#85669) ;
#79963=STYLED_ITEM('',(#170169),#85670) ;
#79964=STYLED_ITEM('',(#170169),#85671) ;
#79965=STYLED_ITEM('',(#170169),#85672) ;
#79966=STYLED_ITEM('',(#170169),#85673) ;
#79967=STYLED_ITEM('',(#170169),#85674) ;
#79968=STYLED_ITEM('',(#170169),#85675) ;
#79969=STYLED_ITEM('',(#170169),#85676) ;
#79970=STYLED_ITEM('',(#170169),#85677) ;
#79971=STYLED_ITEM('',(#170169),#85678) ;
#79972=STYLED_ITEM('',(#170169),#85679) ;
#79973=STYLED_ITEM('',(#170169),#85680) ;
#79974=STYLED_ITEM('',(#170169),#85681) ;
#79975=STYLED_ITEM('',(#170169),#85682) ;
#79976=STYLED_ITEM('',(#170169),#85683) ;
#79977=STYLED_ITEM('',(#170169),#85684) ;
#79978=STYLED_ITEM('',(#170169),#85685) ;
#79979=STYLED_ITEM('',(#170169),#85686) ;
#79980=STYLED_ITEM('',(#170169),#85687) ;
#79981=STYLED_ITEM('',(#170169),#85688) ;
#79982=STYLED_ITEM('',(#170169),#85689) ;
#79983=STYLED_ITEM('',(#170169),#85690) ;
#79984=STYLED_ITEM('',(#170169),#85691) ;
#79985=STYLED_ITEM('',(#170169),#85692) ;
#79986=STYLED_ITEM('',(#170169),#85693) ;
#79987=STYLED_ITEM('',(#170169),#85694) ;
#79988=STYLED_ITEM('',(#170169),#85695) ;
#79989=STYLED_ITEM('',(#170169),#85696) ;
#79990=STYLED_ITEM('',(#170169),#85697) ;
#79991=STYLED_ITEM('',(#170169),#85698) ;
#79992=STYLED_ITEM('',(#170169),#85699) ;
#79993=STYLED_ITEM('',(#170169),#85700) ;
#79994=STYLED_ITEM('',(#170169),#85701) ;
#79995=STYLED_ITEM('',(#170169),#85702) ;
#79996=STYLED_ITEM('',(#170169),#85703) ;
#79997=STYLED_ITEM('',(#170169),#85704) ;
#79998=STYLED_ITEM('',(#170169),#85705) ;
#79999=STYLED_ITEM('',(#170169),#85706) ;
#80000=STYLED_ITEM('',(#170169),#85707) ;
#80001=STYLED_ITEM('',(#170169),#85708) ;
#80002=STYLED_ITEM('',(#170169),#85709) ;
#80003=STYLED_ITEM('',(#170169),#85710) ;
#80004=STYLED_ITEM('',(#170169),#85711) ;
#80005=STYLED_ITEM('',(#170169),#85712) ;
#80006=STYLED_ITEM('',(#170169),#85713) ;
#80007=STYLED_ITEM('',(#170169),#85714) ;
#80008=STYLED_ITEM('',(#170169),#85715) ;
#80009=STYLED_ITEM('',(#170169),#85716) ;
#80010=STYLED_ITEM('',(#170169),#85717) ;
#80011=STYLED_ITEM('',(#170169),#85718) ;
#80012=STYLED_ITEM('',(#170169),#85719) ;
#80013=STYLED_ITEM('',(#170169),#85720) ;
#80014=STYLED_ITEM('',(#170169),#85721) ;
#80015=STYLED_ITEM('',(#170169),#85722) ;
#80016=STYLED_ITEM('',(#170169),#85723) ;
#80017=STYLED_ITEM('',(#170169),#85724) ;
#80018=STYLED_ITEM('',(#170169),#85725) ;
#80019=STYLED_ITEM('',(#170169),#85726) ;
#80020=STYLED_ITEM('',(#170169),#85727) ;
#80021=STYLED_ITEM('',(#170169),#85728) ;
#80022=STYLED_ITEM('',(#170169),#85729) ;
#80023=STYLED_ITEM('',(#170169),#85730) ;
#80024=STYLED_ITEM('',(#170169),#85731) ;
#80025=STYLED_ITEM('',(#170169),#85732) ;
#80026=STYLED_ITEM('',(#170169),#85733) ;
#80027=STYLED_ITEM('',(#170169),#85734) ;
#80028=STYLED_ITEM('',(#170169),#85735) ;
#80029=STYLED_ITEM('',(#170169),#85736) ;
#80030=STYLED_ITEM('',(#170169),#85737) ;
#80031=STYLED_ITEM('',(#170169),#85738) ;
#80032=STYLED_ITEM('',(#170169),#85739) ;
#80033=STYLED_ITEM('',(#170169),#85740) ;
#80034=STYLED_ITEM('',(#170169),#85741) ;
#80035=STYLED_ITEM('',(#170169),#85742) ;
#80036=STYLED_ITEM('',(#170169),#85743) ;
#80037=STYLED_ITEM('',(#170169),#85744) ;
#80038=STYLED_ITEM('',(#170169),#85745) ;
#80039=STYLED_ITEM('',(#170169),#85746) ;
#80040=STYLED_ITEM('',(#170169),#85747) ;
#80041=STYLED_ITEM('',(#170169),#85748) ;
#80042=STYLED_ITEM('',(#170169),#85749) ;
#80043=STYLED_ITEM('',(#170169),#85750) ;
#80044=STYLED_ITEM('',(#170169),#85751) ;
#80045=STYLED_ITEM('',(#170169),#85752) ;
#80046=STYLED_ITEM('',(#170169),#85753) ;
#80047=STYLED_ITEM('',(#170169),#85754) ;
#80048=STYLED_ITEM('',(#170169),#85755) ;
#80049=STYLED_ITEM('',(#170169),#85756) ;
#80050=STYLED_ITEM('',(#170169),#85757) ;
#80051=STYLED_ITEM('',(#170169),#85758) ;
#80052=STYLED_ITEM('',(#170169),#85759) ;
#80053=STYLED_ITEM('',(#170169),#85760) ;
#80054=STYLED_ITEM('',(#170169),#85761) ;
#80055=STYLED_ITEM('',(#170169),#85762) ;
#80056=STYLED_ITEM('',(#170169),#85763) ;
#80057=STYLED_ITEM('',(#170169),#85764) ;
#80058=STYLED_ITEM('',(#170169),#85765) ;
#80059=STYLED_ITEM('',(#170169),#85766) ;
#80060=STYLED_ITEM('',(#170170),#85767) ;
#80061=STYLED_ITEM('',(#170170),#85768) ;
#80062=STYLED_ITEM('',(#170170),#85769) ;
#80063=STYLED_ITEM('',(#170170),#85770) ;
#80064=STYLED_ITEM('',(#170169),#85771) ;
#80065=STYLED_ITEM('',(#170169),#85772) ;
#80066=STYLED_ITEM('',(#170169),#85773) ;
#80067=STYLED_ITEM('',(#170169),#85774) ;
#80068=STYLED_ITEM('',(#170169),#85775) ;
#80069=STYLED_ITEM('',(#170169),#85776) ;
#80070=STYLED_ITEM('',(#170169),#85777) ;
#80071=STYLED_ITEM('',(#170169),#85778) ;
#80072=STYLED_ITEM('',(#170169),#85779) ;
#80073=STYLED_ITEM('',(#170169),#85780) ;
#80074=STYLED_ITEM('',(#170169),#85781) ;
#80075=STYLED_ITEM('',(#170169),#85782) ;
#80076=STYLED_ITEM('',(#170169),#85783) ;
#80077=STYLED_ITEM('',(#170169),#85784) ;
#80078=STYLED_ITEM('',(#170169),#85785) ;
#80079=STYLED_ITEM('',(#170169),#85786) ;
#80080=STYLED_ITEM('',(#170169),#85787) ;
#80081=STYLED_ITEM('',(#170169),#85788) ;
#80082=STYLED_ITEM('',(#170169),#85789) ;
#80083=STYLED_ITEM('',(#170169),#85790) ;
#80084=STYLED_ITEM('',(#170169),#85791) ;
#80085=STYLED_ITEM('',(#170169),#85792) ;
#80086=STYLED_ITEM('',(#170169),#85793) ;
#80087=STYLED_ITEM('',(#170169),#85794) ;
#80088=STYLED_ITEM('',(#170169),#85795) ;
#80089=STYLED_ITEM('',(#170169),#85796) ;
#80090=STYLED_ITEM('',(#170169),#85797) ;
#80091=STYLED_ITEM('',(#170169),#85798) ;
#80092=STYLED_ITEM('',(#170169),#85799) ;
#80093=STYLED_ITEM('',(#170169),#85800) ;
#80094=STYLED_ITEM('',(#170169),#85801) ;
#80095=STYLED_ITEM('',(#170169),#85802) ;
#80096=STYLED_ITEM('',(#170169),#85803) ;
#80097=STYLED_ITEM('',(#170169),#85804) ;
#80098=STYLED_ITEM('',(#170169),#85805) ;
#80099=STYLED_ITEM('',(#170169),#85806) ;
#80100=STYLED_ITEM('',(#170169),#85807) ;
#80101=STYLED_ITEM('',(#170169),#85808) ;
#80102=STYLED_ITEM('',(#170169),#85809) ;
#80103=STYLED_ITEM('',(#170169),#85810) ;
#80104=STYLED_ITEM('',(#170169),#85811) ;
#80105=STYLED_ITEM('',(#170169),#85812) ;
#80106=STYLED_ITEM('',(#170169),#85813) ;
#80107=STYLED_ITEM('',(#170169),#85814) ;
#80108=STYLED_ITEM('',(#170168),#29) ;
#80109=STYLED_ITEM('',(#170169),#85815) ;
#80110=STYLED_ITEM('',(#170169),#85816) ;
#80111=STYLED_ITEM('',(#170169),#85817) ;
#80112=STYLED_ITEM('',(#170169),#85818) ;
#80113=STYLED_ITEM('',(#170169),#85819) ;
#80114=STYLED_ITEM('',(#170169),#85820) ;
#80115=STYLED_ITEM('',(#170169),#85821) ;
#80116=STYLED_ITEM('',(#170169),#85822) ;
#80117=STYLED_ITEM('',(#170169),#85823) ;
#80118=STYLED_ITEM('',(#170169),#85824) ;
#80119=STYLED_ITEM('',(#170169),#85825) ;
#80120=STYLED_ITEM('',(#170169),#85826) ;
#80121=STYLED_ITEM('',(#170169),#85827) ;
#80122=STYLED_ITEM('',(#170169),#85828) ;
#80123=STYLED_ITEM('',(#170169),#85829) ;
#80124=STYLED_ITEM('',(#170169),#85830) ;
#80125=STYLED_ITEM('',(#170169),#85831) ;
#80126=STYLED_ITEM('',(#170169),#85832) ;
#80127=STYLED_ITEM('',(#170169),#85833) ;
#80128=STYLED_ITEM('',(#170169),#85834) ;
#80129=STYLED_ITEM('',(#170169),#85835) ;
#80130=STYLED_ITEM('',(#170169),#85836) ;
#80131=STYLED_ITEM('',(#170169),#85837) ;
#80132=STYLED_ITEM('',(#170169),#85838) ;
#80133=STYLED_ITEM('',(#170169),#85839) ;
#80134=STYLED_ITEM('',(#170169),#85840) ;
#80135=STYLED_ITEM('',(#170169),#85841) ;
#80136=STYLED_ITEM('',(#170169),#85842) ;
#80137=STYLED_ITEM('',(#170169),#85843) ;
#80138=STYLED_ITEM('',(#170169),#85844) ;
#80139=STYLED_ITEM('',(#170169),#85845) ;
#80140=STYLED_ITEM('',(#170169),#85847) ;
#80141=STYLED_ITEM('',(#170170),#85849) ;
#80142=STYLED_ITEM('',(#170169),#85850) ;
#80143=STYLED_ITEM('',(#170169),#85851) ;
#80144=STYLED_ITEM('',(#170169),#85852) ;
#80145=STYLED_ITEM('',(#170169),#85853) ;
#80146=STYLED_ITEM('',(#170169),#85854) ;
#80147=STYLED_ITEM('',(#170169),#85855) ;
#80148=STYLED_ITEM('',(#170169),#85856) ;
#80149=STYLED_ITEM('',(#170169),#85857) ;
#80150=STYLED_ITEM('',(#170169),#85858) ;
#80151=STYLED_ITEM('',(#170169),#85859) ;
#80152=STYLED_ITEM('',(#170169),#85860) ;
#80153=STYLED_ITEM('',(#170169),#85861) ;
#80154=STYLED_ITEM('',(#170169),#85862) ;
#80155=STYLED_ITEM('',(#170169),#85863) ;
#80156=STYLED_ITEM('',(#170169),#85866) ;
#80157=STYLED_ITEM('',(#170169),#85867) ;
#80158=STYLED_ITEM('',(#170169),#85868) ;
#80159=STYLED_ITEM('',(#170171),#85869) ;
#80160=STYLED_ITEM('',(#170169),#85870) ;
#80161=STYLED_ITEM('',(#170169),#85871) ;
#80162=STYLED_ITEM('',(#170169),#85872) ;
#80163=STYLED_ITEM('',(#170169),#85873) ;
#80164=STYLED_ITEM('',(#170169),#85874) ;
#80165=STYLED_ITEM('',(#170169),#85875) ;
#80166=STYLED_ITEM('',(#170169),#85876) ;
#80167=STYLED_ITEM('',(#170169),#85877) ;
#80168=STYLED_ITEM('',(#170169),#85878) ;
#80169=STYLED_ITEM('',(#170169),#85879) ;
#80170=STYLED_ITEM('',(#170169),#85880) ;
#80171=STYLED_ITEM('',(#170169),#85881) ;
#80172=STYLED_ITEM('',(#170169),#85882) ;
#80173=STYLED_ITEM('',(#170169),#85883) ;
#80174=STYLED_ITEM('',(#170169),#85884) ;
#80175=STYLED_ITEM('',(#170169),#85885) ;
#80176=STYLED_ITEM('',(#170169),#85886) ;
#80177=STYLED_ITEM('',(#170169),#85887) ;
#80178=STYLED_ITEM('',(#170169),#85888) ;
#80179=STYLED_ITEM('',(#170170),#85889) ;
#80180=STYLED_ITEM('',(#170170),#85890) ;
#80181=STYLED_ITEM('',(#170170),#85891) ;
#80182=STYLED_ITEM('',(#170170),#85892) ;
#80183=STYLED_ITEM('',(#170169),#85893) ;
#80184=STYLED_ITEM('',(#170169),#85894) ;
#80185=STYLED_ITEM('',(#170169),#85895) ;
#80186=STYLED_ITEM('',(#170169),#85896) ;
#80187=STYLED_ITEM('',(#170169),#85897) ;
#80188=STYLED_ITEM('',(#170169),#85898) ;
#80189=STYLED_ITEM('',(#170169),#85899) ;
#80190=STYLED_ITEM('',(#170169),#85900) ;
#80191=STYLED_ITEM('',(#170169),#85901) ;
#80192=STYLED_ITEM('',(#170169),#85902) ;
#80193=STYLED_ITEM('',(#170169),#85903) ;
#80194=STYLED_ITEM('',(#170169),#85904) ;
#80195=STYLED_ITEM('',(#170169),#85905) ;
#80196=STYLED_ITEM('',(#170169),#85906) ;
#80197=STYLED_ITEM('',(#170169),#85907) ;
#80198=STYLED_ITEM('',(#170169),#85908) ;
#80199=STYLED_ITEM('',(#170169),#85909) ;
#80200=STYLED_ITEM('',(#170169),#85910) ;
#80201=STYLED_ITEM('',(#170171),#85911) ;
#80202=STYLED_ITEM('',(#170169),#85912) ;
#80203=STYLED_ITEM('',(#170169),#85913) ;
#80204=STYLED_ITEM('',(#170169),#85914) ;
#80205=STYLED_ITEM('',(#170169),#85915) ;
#80206=STYLED_ITEM('',(#170169),#85916) ;
#80207=STYLED_ITEM('',(#170169),#85917) ;
#80208=STYLED_ITEM('',(#170169),#85918) ;
#80209=STYLED_ITEM('',(#170169),#85919) ;
#80210=STYLED_ITEM('',(#170169),#85920) ;
#80211=STYLED_ITEM('',(#170169),#85921) ;
#80212=STYLED_ITEM('',(#170169),#85922) ;
#80213=STYLED_ITEM('',(#170169),#85923) ;
#80214=STYLED_ITEM('',(#170169),#85924) ;
#80215=STYLED_ITEM('',(#170169),#85925) ;
#80216=STYLED_ITEM('',(#170169),#85926) ;
#80217=STYLED_ITEM('',(#170169),#85927) ;
#80218=STYLED_ITEM('',(#170169),#85928) ;
#80219=STYLED_ITEM('',(#170169),#85929) ;
#80220=STYLED_ITEM('',(#170169),#85930) ;
#80221=STYLED_ITEM('',(#170169),#85931) ;
#80222=STYLED_ITEM('',(#170169),#85932) ;
#80223=STYLED_ITEM('',(#170169),#85933) ;
#80224=STYLED_ITEM('',(#170169),#85934) ;
#80225=STYLED_ITEM('',(#170169),#85935) ;
#80226=STYLED_ITEM('',(#170169),#85936) ;
#80227=STYLED_ITEM('',(#170169),#85937) ;
#80228=STYLED_ITEM('',(#170169),#85938) ;
#80229=STYLED_ITEM('',(#170169),#85939) ;
#80230=STYLED_ITEM('',(#170169),#85940) ;
#80231=STYLED_ITEM('',(#170169),#85941) ;
#80232=STYLED_ITEM('',(#170169),#85942) ;
#80233=STYLED_ITEM('',(#170169),#85943) ;
#80234=STYLED_ITEM('',(#170169),#85944) ;
#80235=STYLED_ITEM('',(#170169),#85945) ;
#80236=STYLED_ITEM('',(#170169),#85946) ;
#80237=STYLED_ITEM('',(#170169),#85947) ;
#80238=STYLED_ITEM('',(#170169),#85948) ;
#80239=STYLED_ITEM('',(#170169),#85949) ;
#80240=STYLED_ITEM('',(#170169),#85950) ;
#80241=STYLED_ITEM('',(#170169),#85951) ;
#80242=STYLED_ITEM('',(#170169),#85952) ;
#80243=STYLED_ITEM('',(#170169),#85953) ;
#80244=STYLED_ITEM('',(#170169),#85954) ;
#80245=STYLED_ITEM('',(#170169),#85955) ;
#80246=STYLED_ITEM('',(#170169),#85956) ;
#80247=STYLED_ITEM('',(#170169),#85957) ;
#80248=STYLED_ITEM('',(#170169),#85958) ;
#80249=STYLED_ITEM('',(#170169),#85959) ;
#80250=STYLED_ITEM('',(#170169),#85960) ;
#80251=STYLED_ITEM('',(#170169),#85961) ;
#80252=STYLED_ITEM('',(#170169),#85962) ;
#80253=STYLED_ITEM('',(#170169),#85963) ;
#80254=STYLED_ITEM('',(#170169),#85964) ;
#80255=STYLED_ITEM('',(#170169),#85965) ;
#80256=STYLED_ITEM('',(#170169),#85966) ;
#80257=STYLED_ITEM('',(#170169),#85967) ;
#80258=STYLED_ITEM('',(#170169),#85968) ;
#80259=STYLED_ITEM('',(#170169),#85969) ;
#80260=STYLED_ITEM('',(#170169),#85970) ;
#80261=STYLED_ITEM('',(#170169),#85971) ;
#80262=STYLED_ITEM('',(#170169),#85972) ;
#80263=STYLED_ITEM('',(#170169),#85973) ;
#80264=STYLED_ITEM('',(#170169),#85974) ;
#80265=STYLED_ITEM('',(#170169),#85975) ;
#80266=STYLED_ITEM('',(#170169),#85976) ;
#80267=STYLED_ITEM('',(#170169),#85977) ;
#80268=STYLED_ITEM('',(#170169),#85978) ;
#80269=STYLED_ITEM('',(#170169),#85979) ;
#80270=STYLED_ITEM('',(#170169),#85980) ;
#80271=STYLED_ITEM('',(#170169),#85981) ;
#80272=STYLED_ITEM('',(#170169),#85982) ;
#80273=STYLED_ITEM('',(#170169),#85983) ;
#80274=STYLED_ITEM('',(#170169),#85984) ;
#80275=STYLED_ITEM('',(#170169),#85985) ;
#80276=STYLED_ITEM('',(#170169),#85986) ;
#80277=STYLED_ITEM('',(#170169),#85987) ;
#80278=STYLED_ITEM('',(#170169),#85988) ;
#80279=STYLED_ITEM('',(#170169),#85989) ;
#80280=STYLED_ITEM('',(#170169),#85990) ;
#80281=STYLED_ITEM('',(#170169),#85991) ;
#80282=STYLED_ITEM('',(#170169),#85992) ;
#80283=STYLED_ITEM('',(#170169),#85993) ;
#80284=STYLED_ITEM('',(#170169),#85994) ;
#80285=STYLED_ITEM('',(#170169),#85995) ;
#80286=STYLED_ITEM('',(#170169),#85996) ;
#80287=STYLED_ITEM('',(#170169),#85997) ;
#80288=STYLED_ITEM('',(#170169),#85998) ;
#80289=STYLED_ITEM('',(#170169),#85999) ;
#80290=STYLED_ITEM('',(#170169),#86000) ;
#80291=STYLED_ITEM('',(#170169),#86001) ;
#80292=STYLED_ITEM('',(#170169),#86002) ;
#80293=STYLED_ITEM('',(#170169),#86003) ;
#80294=STYLED_ITEM('',(#170169),#86004) ;
#80295=STYLED_ITEM('',(#170169),#86005) ;
#80296=STYLED_ITEM('',(#170169),#86006) ;
#80297=STYLED_ITEM('',(#170169),#86007) ;
#80298=STYLED_ITEM('',(#170169),#86008) ;
#80299=STYLED_ITEM('',(#170169),#86009) ;
#80300=STYLED_ITEM('',(#170169),#86010) ;
#80301=STYLED_ITEM('',(#170169),#86011) ;
#80302=STYLED_ITEM('',(#170169),#86012) ;
#80303=STYLED_ITEM('',(#170169),#86013) ;
#80304=STYLED_ITEM('',(#170169),#86014) ;
#80305=STYLED_ITEM('',(#170169),#86015) ;
#80306=STYLED_ITEM('',(#170169),#86016) ;
#80307=STYLED_ITEM('',(#170169),#86017) ;
#80308=STYLED_ITEM('',(#170169),#86018) ;
#80309=STYLED_ITEM('',(#170169),#86019) ;
#80310=STYLED_ITEM('',(#170169),#86020) ;
#80311=STYLED_ITEM('',(#170169),#86021) ;
#80312=STYLED_ITEM('',(#170169),#86022) ;
#80313=STYLED_ITEM('',(#170170),#86023) ;
#80314=STYLED_ITEM('',(#170170),#86024) ;
#80315=STYLED_ITEM('',(#170170),#86025) ;
#80316=STYLED_ITEM('',(#170170),#86026) ;
#80317=STYLED_ITEM('',(#170169),#86027) ;
#80318=STYLED_ITEM('',(#170169),#86028) ;
#80319=STYLED_ITEM('',(#170169),#86029) ;
#80320=STYLED_ITEM('',(#170169),#86030) ;
#80321=STYLED_ITEM('',(#170169),#86031) ;
#80322=STYLED_ITEM('',(#170169),#86032) ;
#80323=STYLED_ITEM('',(#170169),#86033) ;
#80324=STYLED_ITEM('',(#170169),#86034) ;
#80325=STYLED_ITEM('',(#170169),#86035) ;
#80326=STYLED_ITEM('',(#170169),#86036) ;
#80327=STYLED_ITEM('',(#170169),#86037) ;
#80328=STYLED_ITEM('',(#170169),#86038) ;
#80329=STYLED_ITEM('',(#170169),#86039) ;
#80330=STYLED_ITEM('',(#170169),#86040) ;
#80331=STYLED_ITEM('',(#170169),#86041) ;
#80332=STYLED_ITEM('',(#170169),#86042) ;
#80333=STYLED_ITEM('',(#170169),#86043) ;
#80334=STYLED_ITEM('',(#170169),#86044) ;
#80335=STYLED_ITEM('',(#170169),#86045) ;
#80336=STYLED_ITEM('',(#170169),#86046) ;
#80337=STYLED_ITEM('',(#170169),#86047) ;
#80338=STYLED_ITEM('',(#170169),#86048) ;
#80339=STYLED_ITEM('',(#170169),#86049) ;
#80340=STYLED_ITEM('',(#170169),#86050) ;
#80341=STYLED_ITEM('',(#170169),#86051) ;
#80342=STYLED_ITEM('',(#170169),#86052) ;
#80343=STYLED_ITEM('',(#170169),#86053) ;
#80344=STYLED_ITEM('',(#170169),#86054) ;
#80345=STYLED_ITEM('',(#170169),#86055) ;
#80346=STYLED_ITEM('',(#170169),#86056) ;
#80347=STYLED_ITEM('',(#170169),#86057) ;
#80348=STYLED_ITEM('',(#170169),#86058) ;
#80349=STYLED_ITEM('',(#170169),#86059) ;
#80350=STYLED_ITEM('',(#170169),#86060) ;
#80351=STYLED_ITEM('',(#170169),#86061) ;
#80352=STYLED_ITEM('',(#170169),#86062) ;
#80353=STYLED_ITEM('',(#170170),#86063) ;
#80354=STYLED_ITEM('',(#170169),#86064) ;
#80355=STYLED_ITEM('',(#170169),#86065) ;
#80356=STYLED_ITEM('',(#170169),#86066) ;
#80357=STYLED_ITEM('',(#170169),#86067) ;
#80358=STYLED_ITEM('',(#170169),#86068) ;
#80359=STYLED_ITEM('',(#170169),#86069) ;
#80360=STYLED_ITEM('',(#170171),#86070) ;
#80361=STYLED_ITEM('',(#170169),#86071) ;
#80362=STYLED_ITEM('',(#170169),#86072) ;
#80363=STYLED_ITEM('',(#170169),#86073) ;
#80364=STYLED_ITEM('',(#170169),#86074) ;
#80365=STYLED_ITEM('',(#170169),#86075) ;
#80366=STYLED_ITEM('',(#170169),#86076) ;
#80367=STYLED_ITEM('',(#170169),#86077) ;
#80368=STYLED_ITEM('',(#170169),#86078) ;
#80369=STYLED_ITEM('',(#170169),#86079) ;
#80370=STYLED_ITEM('',(#170169),#86080) ;
#80371=STYLED_ITEM('',(#170169),#86081) ;
#80372=STYLED_ITEM('',(#170169),#86082) ;
#80373=STYLED_ITEM('',(#170169),#86083) ;
#80374=STYLED_ITEM('',(#170169),#86084) ;
#80375=STYLED_ITEM('',(#170169),#86085) ;
#80376=STYLED_ITEM('',(#170169),#86086) ;
#80377=STYLED_ITEM('',(#170169),#86087) ;
#80378=STYLED_ITEM('',(#170169),#86088) ;
#80379=STYLED_ITEM('',(#170169),#86089) ;
#80380=STYLED_ITEM('',(#170170),#86090) ;
#80381=STYLED_ITEM('',(#170170),#86091) ;
#80382=STYLED_ITEM('',(#170170),#86092) ;
#80383=STYLED_ITEM('',(#170170),#86093) ;
#80384=STYLED_ITEM('',(#170169),#86094) ;
#80385=STYLED_ITEM('',(#170169),#86095) ;
#80386=STYLED_ITEM('',(#170169),#86096) ;
#80387=STYLED_ITEM('',(#170169),#86097) ;
#80388=STYLED_ITEM('',(#170169),#86098) ;
#80389=STYLED_ITEM('',(#170169),#86099) ;
#80390=STYLED_ITEM('',(#170169),#86100) ;
#80391=STYLED_ITEM('',(#170169),#86101) ;
#80392=STYLED_ITEM('',(#170169),#86102) ;
#80393=STYLED_ITEM('',(#170169),#86103) ;
#80394=STYLED_ITEM('',(#170169),#86104) ;
#80395=STYLED_ITEM('',(#170169),#86105) ;
#80396=STYLED_ITEM('',(#170169),#86106) ;
#80397=STYLED_ITEM('',(#170169),#86107) ;
#80398=STYLED_ITEM('',(#170169),#86108) ;
#80399=STYLED_ITEM('',(#170169),#86109) ;
#80400=STYLED_ITEM('',(#170169),#86110) ;
#80401=STYLED_ITEM('',(#170169),#86111) ;
#80402=STYLED_ITEM('',(#170171),#86112) ;
#80403=STYLED_ITEM('',(#170169),#86113) ;
#80404=STYLED_ITEM('',(#170169),#86114) ;
#80405=STYLED_ITEM('',(#170169),#86115) ;
#80406=STYLED_ITEM('',(#170169),#86116) ;
#80407=STYLED_ITEM('',(#170169),#86117) ;
#80408=STYLED_ITEM('',(#170169),#86118) ;
#80409=STYLED_ITEM('',(#170169),#86119) ;
#80410=STYLED_ITEM('',(#170169),#86120) ;
#80411=STYLED_ITEM('',(#170169),#86121) ;
#80412=STYLED_ITEM('',(#170169),#86122) ;
#80413=STYLED_ITEM('',(#170169),#86123) ;
#80414=STYLED_ITEM('',(#170169),#86124) ;
#80415=STYLED_ITEM('',(#170169),#86125) ;
#80416=STYLED_ITEM('',(#170169),#86126) ;
#80417=STYLED_ITEM('',(#170169),#86127) ;
#80418=STYLED_ITEM('',(#170169),#86128) ;
#80419=STYLED_ITEM('',(#170169),#86129) ;
#80420=STYLED_ITEM('',(#170169),#86130) ;
#80421=STYLED_ITEM('',(#170169),#86131) ;
#80422=STYLED_ITEM('',(#170169),#86132) ;
#80423=STYLED_ITEM('',(#170169),#86133) ;
#80424=STYLED_ITEM('',(#170169),#86134) ;
#80425=STYLED_ITEM('',(#170169),#86135) ;
#80426=STYLED_ITEM('',(#170169),#86136) ;
#80427=STYLED_ITEM('',(#170169),#86137) ;
#80428=STYLED_ITEM('',(#170169),#86138) ;
#80429=STYLED_ITEM('',(#170169),#86139) ;
#80430=STYLED_ITEM('',(#170169),#86140) ;
#80431=STYLED_ITEM('',(#170169),#86141) ;
#80432=STYLED_ITEM('',(#170169),#86142) ;
#80433=STYLED_ITEM('',(#170169),#86143) ;
#80434=STYLED_ITEM('',(#170169),#86144) ;
#80435=STYLED_ITEM('',(#170169),#86145) ;
#80436=STYLED_ITEM('',(#170169),#86146) ;
#80437=STYLED_ITEM('',(#170169),#86147) ;
#80438=STYLED_ITEM('',(#170169),#86148) ;
#80439=STYLED_ITEM('',(#170169),#86149) ;
#80440=STYLED_ITEM('',(#170169),#86150) ;
#80441=STYLED_ITEM('',(#170169),#86151) ;
#80442=STYLED_ITEM('',(#170169),#86152) ;
#80443=STYLED_ITEM('',(#170169),#86153) ;
#80444=STYLED_ITEM('',(#170169),#86154) ;
#80445=STYLED_ITEM('',(#170169),#86155) ;
#80446=STYLED_ITEM('',(#170169),#86156) ;
#80447=STYLED_ITEM('',(#170169),#86157) ;
#80448=STYLED_ITEM('',(#170169),#86158) ;
#80449=STYLED_ITEM('',(#170169),#86159) ;
#80450=STYLED_ITEM('',(#170169),#86160) ;
#80451=STYLED_ITEM('',(#170169),#86161) ;
#80452=STYLED_ITEM('',(#170169),#86162) ;
#80453=STYLED_ITEM('',(#170169),#86163) ;
#80454=STYLED_ITEM('',(#170169),#86164) ;
#80455=STYLED_ITEM('',(#170169),#86165) ;
#80456=STYLED_ITEM('',(#170169),#86166) ;
#80457=STYLED_ITEM('',(#170169),#86167) ;
#80458=STYLED_ITEM('',(#170169),#86168) ;
#80459=STYLED_ITEM('',(#170169),#86169) ;
#80460=STYLED_ITEM('',(#170169),#86170) ;
#80461=STYLED_ITEM('',(#170169),#86171) ;
#80462=STYLED_ITEM('',(#170169),#86172) ;
#80463=STYLED_ITEM('',(#170169),#86173) ;
#80464=STYLED_ITEM('',(#170169),#86174) ;
#80465=STYLED_ITEM('',(#170169),#86175) ;
#80466=STYLED_ITEM('',(#170169),#86176) ;
#80467=STYLED_ITEM('',(#170169),#86177) ;
#80468=STYLED_ITEM('',(#170169),#86178) ;
#80469=STYLED_ITEM('',(#170169),#86179) ;
#80470=STYLED_ITEM('',(#170169),#86180) ;
#80471=STYLED_ITEM('',(#170169),#86181) ;
#80472=STYLED_ITEM('',(#170169),#86182) ;
#80473=STYLED_ITEM('',(#170169),#86183) ;
#80474=STYLED_ITEM('',(#170169),#86184) ;
#80475=STYLED_ITEM('',(#170169),#86185) ;
#80476=STYLED_ITEM('',(#170169),#86186) ;
#80477=STYLED_ITEM('',(#170169),#86187) ;
#80478=STYLED_ITEM('',(#170169),#86188) ;
#80479=STYLED_ITEM('',(#170169),#86189) ;
#80480=STYLED_ITEM('',(#170169),#86190) ;
#80481=STYLED_ITEM('',(#170169),#86191) ;
#80482=STYLED_ITEM('',(#170169),#86192) ;
#80483=STYLED_ITEM('',(#170169),#86193) ;
#80484=STYLED_ITEM('',(#170169),#86194) ;
#80485=STYLED_ITEM('',(#170169),#86195) ;
#80486=STYLED_ITEM('',(#170169),#86196) ;
#80487=STYLED_ITEM('',(#170169),#86197) ;
#80488=STYLED_ITEM('',(#170169),#86198) ;
#80489=STYLED_ITEM('',(#170169),#86199) ;
#80490=STYLED_ITEM('',(#170169),#86200) ;
#80491=STYLED_ITEM('',(#170169),#86201) ;
#80492=STYLED_ITEM('',(#170169),#86202) ;
#80493=STYLED_ITEM('',(#170169),#86203) ;
#80494=STYLED_ITEM('',(#170169),#86204) ;
#80495=STYLED_ITEM('',(#170169),#86205) ;
#80496=STYLED_ITEM('',(#170169),#86206) ;
#80497=STYLED_ITEM('',(#170169),#86207) ;
#80498=STYLED_ITEM('',(#170169),#86208) ;
#80499=STYLED_ITEM('',(#170169),#86209) ;
#80500=STYLED_ITEM('',(#170169),#86210) ;
#80501=STYLED_ITEM('',(#170169),#86211) ;
#80502=STYLED_ITEM('',(#170169),#86212) ;
#80503=STYLED_ITEM('',(#170169),#86213) ;
#80504=STYLED_ITEM('',(#170169),#86214) ;
#80505=STYLED_ITEM('',(#170170),#86215) ;
#80506=STYLED_ITEM('',(#170170),#86216) ;
#80507=STYLED_ITEM('',(#170170),#86217) ;
#80508=STYLED_ITEM('',(#170170),#86218) ;
#80509=STYLED_ITEM('',(#170169),#86219) ;
#80510=STYLED_ITEM('',(#170169),#86220) ;
#80511=STYLED_ITEM('',(#170169),#86221) ;
#80512=STYLED_ITEM('',(#170169),#86222) ;
#80513=STYLED_ITEM('',(#170169),#86223) ;
#80514=STYLED_ITEM('',(#170169),#86224) ;
#80515=STYLED_ITEM('',(#170169),#86225) ;
#80516=STYLED_ITEM('',(#170169),#86226) ;
#80517=STYLED_ITEM('',(#170169),#86227) ;
#80518=STYLED_ITEM('',(#170169),#86228) ;
#80519=STYLED_ITEM('',(#170169),#86229) ;
#80520=STYLED_ITEM('',(#170169),#86230) ;
#80521=STYLED_ITEM('',(#170169),#86231) ;
#80522=STYLED_ITEM('',(#170169),#86232) ;
#80523=STYLED_ITEM('',(#170169),#86233) ;
#80524=STYLED_ITEM('',(#170169),#86234) ;
#80525=STYLED_ITEM('',(#170169),#86235) ;
#80526=STYLED_ITEM('',(#170169),#86236) ;
#80527=STYLED_ITEM('',(#170169),#86237) ;
#80528=STYLED_ITEM('',(#170169),#86238) ;
#80529=STYLED_ITEM('',(#170169),#86239) ;
#80530=STYLED_ITEM('',(#170169),#86240) ;
#80531=STYLED_ITEM('',(#170169),#86241) ;
#80532=STYLED_ITEM('',(#170169),#86242) ;
#80533=STYLED_ITEM('',(#170169),#86243) ;
#80534=STYLED_ITEM('',(#170169),#86244) ;
#80535=STYLED_ITEM('',(#170169),#86245) ;
#80536=STYLED_ITEM('',(#170169),#86246) ;
#80537=STYLED_ITEM('',(#170169),#86247) ;
#80538=STYLED_ITEM('',(#170169),#86248) ;
#80539=STYLED_ITEM('',(#170169),#86249) ;
#80540=STYLED_ITEM('',(#170169),#86250) ;
#80541=STYLED_ITEM('',(#170169),#86251) ;
#80542=STYLED_ITEM('',(#170169),#86252) ;
#80543=STYLED_ITEM('',(#170169),#86253) ;
#80544=STYLED_ITEM('',(#170169),#86254) ;
#80545=STYLED_ITEM('',(#170169),#86255) ;
#80546=STYLED_ITEM('',(#170169),#86256) ;
#80547=STYLED_ITEM('',(#170169),#86257) ;
#80548=STYLED_ITEM('',(#170169),#86258) ;
#80549=STYLED_ITEM('',(#170169),#86259) ;
#80550=STYLED_ITEM('',(#170169),#86260) ;
#80551=STYLED_ITEM('',(#170169),#86261) ;
#80552=STYLED_ITEM('',(#170169),#86262) ;
#80553=STYLED_ITEM('',(#170168),#30) ;
#80554=STYLED_ITEM('',(#170169),#86263) ;
#80555=STYLED_ITEM('',(#170169),#86264) ;
#80556=STYLED_ITEM('',(#170169),#86265) ;
#80557=STYLED_ITEM('',(#170169),#86266) ;
#80558=STYLED_ITEM('',(#170169),#86267) ;
#80559=STYLED_ITEM('',(#170169),#86268) ;
#80560=STYLED_ITEM('',(#170169),#86269) ;
#80561=STYLED_ITEM('',(#170169),#86270) ;
#80562=STYLED_ITEM('',(#170169),#86271) ;
#80563=STYLED_ITEM('',(#170169),#86272) ;
#80564=STYLED_ITEM('',(#170169),#86273) ;
#80565=STYLED_ITEM('',(#170169),#86274) ;
#80566=STYLED_ITEM('',(#170169),#86275) ;
#80567=STYLED_ITEM('',(#170169),#86276) ;
#80568=STYLED_ITEM('',(#170169),#86277) ;
#80569=STYLED_ITEM('',(#170170),#86278) ;
#80570=STYLED_ITEM('',(#170169),#86279) ;
#80571=STYLED_ITEM('',(#170169),#86280) ;
#80572=STYLED_ITEM('',(#170169),#86281) ;
#80573=STYLED_ITEM('',(#170169),#86282) ;
#80574=STYLED_ITEM('',(#170169),#86283) ;
#80575=STYLED_ITEM('',(#170169),#86284) ;
#80576=STYLED_ITEM('',(#170169),#86285) ;
#80577=STYLED_ITEM('',(#170169),#86286) ;
#80578=STYLED_ITEM('',(#170169),#86287) ;
#80579=STYLED_ITEM('',(#170169),#86288) ;
#80580=STYLED_ITEM('',(#170169),#86289) ;
#80581=STYLED_ITEM('',(#170169),#86290) ;
#80582=STYLED_ITEM('',(#170169),#86291) ;
#80583=STYLED_ITEM('',(#170169),#86292) ;
#80584=STYLED_ITEM('',(#170169),#86293) ;
#80585=STYLED_ITEM('',(#170169),#86294) ;
#80586=STYLED_ITEM('',(#170169),#86295) ;
#80587=STYLED_ITEM('',(#170169),#86296) ;
#80588=STYLED_ITEM('',(#170169),#86297) ;
#80589=STYLED_ITEM('',(#170169),#86298) ;
#80590=STYLED_ITEM('',(#170169),#86299) ;
#80591=STYLED_ITEM('',(#170169),#86300) ;
#80592=STYLED_ITEM('',(#170169),#86301) ;
#80593=STYLED_ITEM('',(#170169),#86302) ;
#80594=STYLED_ITEM('',(#170171),#86303) ;
#80595=STYLED_ITEM('',(#170169),#86304) ;
#80596=STYLED_ITEM('',(#170169),#86305) ;
#80597=STYLED_ITEM('',(#170169),#86306) ;
#80598=STYLED_ITEM('',(#170169),#86307) ;
#80599=STYLED_ITEM('',(#170169),#86308) ;
#80600=STYLED_ITEM('',(#170169),#86309) ;
#80601=STYLED_ITEM('',(#170169),#86310) ;
#80602=STYLED_ITEM('',(#170169),#86311) ;
#80603=STYLED_ITEM('',(#170169),#86312) ;
#80604=STYLED_ITEM('',(#170169),#86313) ;
#80605=STYLED_ITEM('',(#170169),#86314) ;
#80606=STYLED_ITEM('',(#170169),#86315) ;
#80607=STYLED_ITEM('',(#170169),#86316) ;
#80608=STYLED_ITEM('',(#170169),#86317) ;
#80609=STYLED_ITEM('',(#170169),#86318) ;
#80610=STYLED_ITEM('',(#170169),#86319) ;
#80611=STYLED_ITEM('',(#170169),#86320) ;
#80612=STYLED_ITEM('',(#170169),#86321) ;
#80613=STYLED_ITEM('',(#170169),#86322) ;
#80614=STYLED_ITEM('',(#170170),#86323) ;
#80615=STYLED_ITEM('',(#170170),#86324) ;
#80616=STYLED_ITEM('',(#170170),#86325) ;
#80617=STYLED_ITEM('',(#170170),#86326) ;
#80618=STYLED_ITEM('',(#170169),#86327) ;
#80619=STYLED_ITEM('',(#170169),#86328) ;
#80620=STYLED_ITEM('',(#170169),#86329) ;
#80621=STYLED_ITEM('',(#170169),#86330) ;
#80622=STYLED_ITEM('',(#170169),#86331) ;
#80623=STYLED_ITEM('',(#170169),#86332) ;
#80624=STYLED_ITEM('',(#170169),#86333) ;
#80625=STYLED_ITEM('',(#170169),#86334) ;
#80626=STYLED_ITEM('',(#170169),#86335) ;
#80627=STYLED_ITEM('',(#170169),#86336) ;
#80628=STYLED_ITEM('',(#170169),#86337) ;
#80629=STYLED_ITEM('',(#170169),#86338) ;
#80630=STYLED_ITEM('',(#170169),#86339) ;
#80631=STYLED_ITEM('',(#170169),#86340) ;
#80632=STYLED_ITEM('',(#170169),#86341) ;
#80633=STYLED_ITEM('',(#170169),#86342) ;
#80634=STYLED_ITEM('',(#170169),#86343) ;
#80635=STYLED_ITEM('',(#170169),#86344) ;
#80636=STYLED_ITEM('',(#170171),#86345) ;
#80637=STYLED_ITEM('',(#170169),#86346) ;
#80638=STYLED_ITEM('',(#170169),#86347) ;
#80639=STYLED_ITEM('',(#170169),#86348) ;
#80640=STYLED_ITEM('',(#170169),#86349) ;
#80641=STYLED_ITEM('',(#170169),#86350) ;
#80642=STYLED_ITEM('',(#170169),#86351) ;
#80643=STYLED_ITEM('',(#170169),#86352) ;
#80644=STYLED_ITEM('',(#170169),#86353) ;
#80645=STYLED_ITEM('',(#170169),#86354) ;
#80646=STYLED_ITEM('',(#170169),#86355) ;
#80647=STYLED_ITEM('',(#170169),#86356) ;
#80648=STYLED_ITEM('',(#170169),#86357) ;
#80649=STYLED_ITEM('',(#170169),#86358) ;
#80650=STYLED_ITEM('',(#170169),#86359) ;
#80651=STYLED_ITEM('',(#170169),#86360) ;
#80652=STYLED_ITEM('',(#170169),#86361) ;
#80653=STYLED_ITEM('',(#170169),#86362) ;
#80654=STYLED_ITEM('',(#170169),#86363) ;
#80655=STYLED_ITEM('',(#170169),#86364) ;
#80656=STYLED_ITEM('',(#170169),#86365) ;
#80657=STYLED_ITEM('',(#170169),#86366) ;
#80658=STYLED_ITEM('',(#170169),#86367) ;
#80659=STYLED_ITEM('',(#170169),#86368) ;
#80660=STYLED_ITEM('',(#170169),#86369) ;
#80661=STYLED_ITEM('',(#170169),#86370) ;
#80662=STYLED_ITEM('',(#170169),#86371) ;
#80663=STYLED_ITEM('',(#170169),#86372) ;
#80664=STYLED_ITEM('',(#170169),#86373) ;
#80665=STYLED_ITEM('',(#170169),#86374) ;
#80666=STYLED_ITEM('',(#170169),#86375) ;
#80667=STYLED_ITEM('',(#170169),#86376) ;
#80668=STYLED_ITEM('',(#170169),#86377) ;
#80669=STYLED_ITEM('',(#170169),#86378) ;
#80670=STYLED_ITEM('',(#170169),#86379) ;
#80671=STYLED_ITEM('',(#170169),#86380) ;
#80672=STYLED_ITEM('',(#170169),#86381) ;
#80673=STYLED_ITEM('',(#170169),#86382) ;
#80674=STYLED_ITEM('',(#170169),#86383) ;
#80675=STYLED_ITEM('',(#170169),#86384) ;
#80676=STYLED_ITEM('',(#170169),#86385) ;
#80677=STYLED_ITEM('',(#170169),#86386) ;
#80678=STYLED_ITEM('',(#170169),#86387) ;
#80679=STYLED_ITEM('',(#170169),#86388) ;
#80680=STYLED_ITEM('',(#170169),#86389) ;
#80681=STYLED_ITEM('',(#170169),#86390) ;
#80682=STYLED_ITEM('',(#170169),#86391) ;
#80683=STYLED_ITEM('',(#170169),#86392) ;
#80684=STYLED_ITEM('',(#170169),#86393) ;
#80685=STYLED_ITEM('',(#170169),#86394) ;
#80686=STYLED_ITEM('',(#170169),#86395) ;
#80687=STYLED_ITEM('',(#170169),#86396) ;
#80688=STYLED_ITEM('',(#170169),#86397) ;
#80689=STYLED_ITEM('',(#170169),#86398) ;
#80690=STYLED_ITEM('',(#170169),#86399) ;
#80691=STYLED_ITEM('',(#170169),#86400) ;
#80692=STYLED_ITEM('',(#170169),#86401) ;
#80693=STYLED_ITEM('',(#170169),#86402) ;
#80694=STYLED_ITEM('',(#170169),#86403) ;
#80695=STYLED_ITEM('',(#170169),#86404) ;
#80696=STYLED_ITEM('',(#170169),#86405) ;
#80697=STYLED_ITEM('',(#170169),#86406) ;
#80698=STYLED_ITEM('',(#170169),#86407) ;
#80699=STYLED_ITEM('',(#170169),#86408) ;
#80700=STYLED_ITEM('',(#170169),#86409) ;
#80701=STYLED_ITEM('',(#170169),#86410) ;
#80702=STYLED_ITEM('',(#170169),#86411) ;
#80703=STYLED_ITEM('',(#170169),#86412) ;
#80704=STYLED_ITEM('',(#170169),#86413) ;
#80705=STYLED_ITEM('',(#170169),#86414) ;
#80706=STYLED_ITEM('',(#170169),#86415) ;
#80707=STYLED_ITEM('',(#170169),#86416) ;
#80708=STYLED_ITEM('',(#170169),#86417) ;
#80709=STYLED_ITEM('',(#170169),#86418) ;
#80710=STYLED_ITEM('',(#170169),#86419) ;
#80711=STYLED_ITEM('',(#170169),#86420) ;
#80712=STYLED_ITEM('',(#170169),#86421) ;
#80713=STYLED_ITEM('',(#170169),#86422) ;
#80714=STYLED_ITEM('',(#170169),#86423) ;
#80715=STYLED_ITEM('',(#170169),#86424) ;
#80716=STYLED_ITEM('',(#170169),#86425) ;
#80717=STYLED_ITEM('',(#170169),#86426) ;
#80718=STYLED_ITEM('',(#170169),#86427) ;
#80719=STYLED_ITEM('',(#170169),#86428) ;
#80720=STYLED_ITEM('',(#170169),#86429) ;
#80721=STYLED_ITEM('',(#170169),#86430) ;
#80722=STYLED_ITEM('',(#170169),#86431) ;
#80723=STYLED_ITEM('',(#170169),#86432) ;
#80724=STYLED_ITEM('',(#170169),#86433) ;
#80725=STYLED_ITEM('',(#170169),#86434) ;
#80726=STYLED_ITEM('',(#170169),#86435) ;
#80727=STYLED_ITEM('',(#170169),#86436) ;
#80728=STYLED_ITEM('',(#170169),#86437) ;
#80729=STYLED_ITEM('',(#170169),#86438) ;
#80730=STYLED_ITEM('',(#170169),#86439) ;
#80731=STYLED_ITEM('',(#170169),#86440) ;
#80732=STYLED_ITEM('',(#170169),#86441) ;
#80733=STYLED_ITEM('',(#170169),#86442) ;
#80734=STYLED_ITEM('',(#170169),#86443) ;
#80735=STYLED_ITEM('',(#170169),#86444) ;
#80736=STYLED_ITEM('',(#170169),#86445) ;
#80737=STYLED_ITEM('',(#170169),#86446) ;
#80738=STYLED_ITEM('',(#170169),#86447) ;
#80739=STYLED_ITEM('',(#170169),#86448) ;
#80740=STYLED_ITEM('',(#170169),#86449) ;
#80741=STYLED_ITEM('',(#170169),#86450) ;
#80742=STYLED_ITEM('',(#170169),#86451) ;
#80743=STYLED_ITEM('',(#170169),#86452) ;
#80744=STYLED_ITEM('',(#170169),#86453) ;
#80745=STYLED_ITEM('',(#170169),#86454) ;
#80746=STYLED_ITEM('',(#170169),#86455) ;
#80747=STYLED_ITEM('',(#170169),#86456) ;
#80748=STYLED_ITEM('',(#170170),#86457) ;
#80749=STYLED_ITEM('',(#170170),#86458) ;
#80750=STYLED_ITEM('',(#170170),#86459) ;
#80751=STYLED_ITEM('',(#170170),#86460) ;
#80752=STYLED_ITEM('',(#170169),#86461) ;
#80753=STYLED_ITEM('',(#170169),#86462) ;
#80754=STYLED_ITEM('',(#170169),#86463) ;
#80755=STYLED_ITEM('',(#170169),#86464) ;
#80756=STYLED_ITEM('',(#170169),#86465) ;
#80757=STYLED_ITEM('',(#170169),#86466) ;
#80758=STYLED_ITEM('',(#170169),#86467) ;
#80759=STYLED_ITEM('',(#170169),#86468) ;
#80760=STYLED_ITEM('',(#170169),#86469) ;
#80761=STYLED_ITEM('',(#170169),#86470) ;
#80762=STYLED_ITEM('',(#170169),#86471) ;
#80763=STYLED_ITEM('',(#170169),#86472) ;
#80764=STYLED_ITEM('',(#170169),#86473) ;
#80765=STYLED_ITEM('',(#170169),#86474) ;
#80766=STYLED_ITEM('',(#170169),#86475) ;
#80767=STYLED_ITEM('',(#170169),#86476) ;
#80768=STYLED_ITEM('',(#170169),#86477) ;
#80769=STYLED_ITEM('',(#170169),#86478) ;
#80770=STYLED_ITEM('',(#170169),#86479) ;
#80771=STYLED_ITEM('',(#170169),#86480) ;
#80772=STYLED_ITEM('',(#170169),#86481) ;
#80773=STYLED_ITEM('',(#170169),#86482) ;
#80774=STYLED_ITEM('',(#170169),#86483) ;
#80775=STYLED_ITEM('',(#170169),#86484) ;
#80776=STYLED_ITEM('',(#170169),#86485) ;
#80777=STYLED_ITEM('',(#170169),#86486) ;
#80778=STYLED_ITEM('',(#170169),#86487) ;
#80779=STYLED_ITEM('',(#170168),#31) ;
#85367=ADVANCED_FACE('',(#17047),#78907,.F.) ;
#85368=ADVANCED_FACE('',(#17048),#78908,.T.) ;
#85369=ADVANCED_FACE('',(#17049),#78909,.F.) ;
#85370=ADVANCED_FACE('',(#17050),#78910,.T.) ;
#85371=ADVANCED_FACE('',(#17051),#78911,.T.) ;
#85372=ADVANCED_FACE('',(#17052),#16155,.T.) ;
#85373=ADVANCED_FACE('',(#17053),#13538,.F.) ;
#85374=ADVANCED_FACE('',(#17054),#16156,.T.) ;
#85375=ADVANCED_FACE('',(#17055),#2415,.F.) ;
#85376=ADVANCED_FACE('',(#17056),#13539,.F.) ;
#85377=ADVANCED_FACE('',(#17057),#13540,.F.) ;
#85378=ADVANCED_FACE('',(#17058),#78912,.F.) ;
#85379=ADVANCED_FACE('',(#17059),#13541,.F.) ;
#85380=ADVANCED_FACE('',(#17060),#78913,.T.) ;
#85381=ADVANCED_FACE('',(#17061),#78914,.F.) ;
#85382=ADVANCED_FACE('',(#17062),#78915,.T.) ;
#85383=ADVANCED_FACE('',(#17063),#78916,.T.) ;
#85384=ADVANCED_FACE('',(#17064),#16157,.T.) ;
#85385=ADVANCED_FACE('',(#17065),#13542,.F.) ;
#85386=ADVANCED_FACE('',(#17066),#16158,.T.) ;
#85387=ADVANCED_FACE('',(#17067),#2416,.F.) ;
#85388=ADVANCED_FACE('',(#17068),#13543,.F.) ;
#85389=ADVANCED_FACE('',(#17069),#13544,.F.) ;
#85390=ADVANCED_FACE('',(#17070,#647),#794,.F.) ;
#85391=ADVANCED_FACE('',(#17071),#795,.F.) ;
#85392=ADVANCED_FACE('',(#17072),#796,.F.) ;
#85393=ADVANCED_FACE('',(#17073),#797,.F.) ;
#85394=ADVANCED_FACE('',(#17074),#13545,.T.) ;
#85395=ADVANCED_FACE('',(#17075),#13546,.F.) ;
#85396=ADVANCED_FACE('',(#17076),#13547,.F.) ;
#85397=ADVANCED_FACE('',(#17077),#13548,.T.) ;
#85398=ADVANCED_FACE('',(#17078),#798,.F.) ;
#85399=ADVANCED_FACE('',(#17079),#799,.F.) ;
#85400=ADVANCED_FACE('',(#17080),#800,.F.) ;
#85401=ADVANCED_FACE('',(#17081),#801,.T.) ;
#85402=ADVANCED_FACE('',(#17082,#648,#649),#802,.F.) ;
#85403=ADVANCED_FACE('',(#17083),#803,.F.) ;
#85404=ADVANCED_FACE('',(#17084),#804,.F.) ;
#85405=ADVANCED_FACE('',(#17085),#805,.F.) ;
#85406=ADVANCED_FACE('',(#17086),#806,.F.) ;
#85407=ADVANCED_FACE('',(#17087,#650,#651,#652,#653),#807,.F.) ;
#85408=ADVANCED_FACE('',(#17088),#808,.F.) ;
#85409=ADVANCED_FACE('',(#17089),#809,.F.) ;
#85410=ADVANCED_FACE('',(#17090),#810,.F.) ;
#85411=ADVANCED_FACE('',(#17091,#654,#655),#811,.F.) ;
#85412=ADVANCED_FACE('',(#17092,#656,#657),#812,.F.) ;
#85413=ADVANCED_FACE('',(#17093),#813,.F.) ;
#85414=ADVANCED_FACE('',(#17094),#814,.F.) ;
#85415=ADVANCED_FACE('',(#17095),#815,.F.) ;
#85416=ADVANCED_FACE('',(#17096),#816,.F.) ;
#85417=ADVANCED_FACE('',(#17097),#817,.T.) ;
#85418=ADVANCED_FACE('',(#17098),#818,.T.) ;
#85419=ADVANCED_FACE('',(#17099),#819,.T.) ;
#85420=ADVANCED_FACE('',(#17100),#820,.T.) ;
#85421=ADVANCED_FACE('',(#17101),#821,.T.) ;
#85422=ADVANCED_FACE('',(#17102),#822,.T.) ;
#85423=ADVANCED_FACE('',(#17103),#823,.F.) ;
#85424=ADVANCED_FACE('',(#17104),#824,.T.) ;
#85425=ADVANCED_FACE('',(#17105),#825,.T.) ;
#85426=ADVANCED_FACE('',(#17106),#826,.F.) ;
#85427=ADVANCED_FACE('',(#17107),#827,.F.) ;
#85428=ADVANCED_FACE('',(#17108),#828,.F.) ;
#85429=ADVANCED_FACE('',(#17109),#829,.F.) ;
#85430=ADVANCED_FACE('',(#17110),#830,.F.) ;
#85431=ADVANCED_FACE('',(#17111,#658),#831,.T.) ;
#85432=ADVANCED_FACE('',(#17112),#13549,.T.) ;
#85433=ADVANCED_FACE('',(#17113),#832,.T.) ;
#85434=ADVANCED_FACE('',(#17114),#13550,.T.) ;
#85435=ADVANCED_FACE('',(#17115),#833,.T.) ;
#85436=ADVANCED_FACE('',(#17116),#13551,.T.) ;
#85437=ADVANCED_FACE('',(#17117),#834,.T.) ;
#85438=ADVANCED_FACE('',(#17118),#13552,.T.) ;
#85439=ADVANCED_FACE('',(#17119),#835,.T.) ;
#85440=ADVANCED_FACE('',(#17120),#836,.T.) ;
#85441=ADVANCED_FACE('',(#17121),#837,.T.) ;
#85442=ADVANCED_FACE('',(#17122),#838,.F.) ;
#85443=ADVANCED_FACE('',(#17123),#839,.F.) ;
#85444=ADVANCED_FACE('',(#17124),#840,.T.) ;
#85445=ADVANCED_FACE('',(#17125),#841,.F.) ;
#85446=ADVANCED_FACE('',(#17126),#842,.F.) ;
#85447=ADVANCED_FACE('',(#17127),#843,.F.) ;
#85448=ADVANCED_FACE('',(#17128),#844,.F.) ;
#85449=ADVANCED_FACE('',(#17129,#659),#845,.T.) ;
#85450=ADVANCED_FACE('',(#17130),#13553,.T.) ;
#85451=ADVANCED_FACE('',(#17131),#846,.T.) ;
#85452=ADVANCED_FACE('',(#17132),#13554,.T.) ;
#85453=ADVANCED_FACE('',(#17133),#847,.T.) ;
#85454=ADVANCED_FACE('',(#17134),#13555,.T.) ;
#85455=ADVANCED_FACE('',(#17135),#848,.T.) ;
#85456=ADVANCED_FACE('',(#17136),#13556,.T.) ;
#85457=ADVANCED_FACE('',(#17137),#849,.T.) ;
#85458=ADVANCED_FACE('',(#17138),#850,.T.) ;
#85459=ADVANCED_FACE('',(#17139),#851,.F.) ;
#85460=ADVANCED_FACE('',(#17140),#852,.F.) ;
#85461=ADVANCED_FACE('',(#17141),#853,.F.) ;
#85462=ADVANCED_FACE('',(#17142),#854,.F.) ;
#85463=ADVANCED_FACE('',(#17143),#855,.T.) ;
#85464=ADVANCED_FACE('',(#17144),#13557,.T.) ;
#85465=ADVANCED_FACE('',(#17145),#34,.T.) ;
#85466=ADVANCED_FACE('',(#17146),#13558,.F.) ;
#85467=ADVANCED_FACE('',(#17147),#35,.F.) ;
#85468=ADVANCED_FACE('',(#17148),#13559,.F.) ;
#85469=ADVANCED_FACE('',(#17149),#13560,.F.) ;
#85470=ADVANCED_FACE('',(#17150),#13561,.T.) ;
#85471=ADVANCED_FACE('',(#17151),#13562,.T.) ;
#85472=ADVANCED_FACE('',(#17152),#13563,.T.) ;
#85473=ADVANCED_FACE('',(#17153),#13564,.F.) ;
#85474=ADVANCED_FACE('',(#17154),#16159,.F.) ;
#85475=ADVANCED_FACE('',(#17155),#36,.T.) ;
#85476=ADVANCED_FACE('',(#17156),#37,.T.) ;
#85477=ADVANCED_FACE('',(#17157),#38,.F.) ;
#85478=ADVANCED_FACE('',(#17158),#13565,.F.) ;
#85479=ADVANCED_FACE('',(#17159),#13566,.F.) ;
#85480=ADVANCED_FACE('',(#17160),#13567,.T.) ;
#85481=ADVANCED_FACE('',(#17161),#13568,.T.) ;
#85482=ADVANCED_FACE('',(#17162),#13569,.F.) ;
#85483=ADVANCED_FACE('',(#17163),#13570,.F.) ;
#85484=ADVANCED_FACE('',(#17164),#16160,.F.) ;
#85485=ADVANCED_FACE('',(#17165),#39,.T.) ;
#85486=ADVANCED_FACE('',(#17166),#16161,.F.) ;
#85487=ADVANCED_FACE('',(#17167),#13571,.F.) ;
#85488=ADVANCED_FACE('',(#17168),#13572,.F.) ;
#85489=ADVANCED_FACE('',(#17169),#13573,.F.) ;
#85490=ADVANCED_FACE('',(#17170),#13574,.F.) ;
#85491=ADVANCED_FACE('',(#17171),#40,.F.) ;
#85492=ADVANCED_FACE('',(#17172),#16162,.F.) ;
#85493=ADVANCED_FACE('',(#17173),#13575,.T.) ;
#85494=ADVANCED_FACE('',(#17174),#13576,.F.) ;
#85495=ADVANCED_FACE('',(#17175),#41,.F.) ;
#85496=ADVANCED_FACE('',(#17176),#13577,.F.) ;
#85497=ADVANCED_FACE('',(#17177),#13578,.T.) ;
#85498=ADVANCED_FACE('',(#17178),#13579,.T.) ;
#85499=ADVANCED_FACE('',(#17179),#13580,.F.) ;
#85500=ADVANCED_FACE('',(#17180),#13581,.T.) ;
#85501=ADVANCED_FACE('',(#17181),#13582,.T.) ;
#85502=ADVANCED_FACE('',(#17182),#13583,.F.) ;
#85503=ADVANCED_FACE('',(#17183),#78917,.T.) ;
#85504=ADVANCED_FACE('',(#17184),#13584,.T.) ;
#85505=ADVANCED_FACE('',(#17185),#13585,.T.) ;
#85506=ADVANCED_FACE('',(#17186),#13586,.T.) ;
#85507=ADVANCED_FACE('',(#17187),#13587,.T.) ;
#85508=ADVANCED_FACE('',(#17188),#16163,.T.) ;
#85509=ADVANCED_FACE('',(#17189),#13588,.T.) ;
#85510=ADVANCED_FACE('',(#17190),#13589,.T.) ;
#85511=ADVANCED_FACE('',(#17191),#16164,.T.) ;
#85512=ADVANCED_FACE('',(#17192),#16165,.T.) ;
#85513=ADVANCED_FACE('',(#17193),#13590,.T.) ;
#85514=ADVANCED_FACE('',(#17194),#13591,.T.) ;
#85515=ADVANCED_FACE('',(#17195),#16166,.T.) ;
#85516=ADVANCED_FACE('',(#17196),#13592,.T.) ;
#85517=ADVANCED_FACE('',(#17197),#78918,.T.) ;
#85518=ADVANCED_FACE('',(#17198),#78919,.T.) ;
#85519=ADVANCED_FACE('',(#17199),#13593,.T.) ;
#85520=ADVANCED_FACE('',(#17200),#13594,.F.) ;
#85521=ADVANCED_FACE('',(#17201),#13595,.F.) ;
#85522=ADVANCED_FACE('',(#17202),#13596,.F.) ;
#85523=ADVANCED_FACE('',(#17203),#13597,.T.) ;
#85524=ADVANCED_FACE('',(#17204),#13598,.T.) ;
#85525=ADVANCED_FACE('',(#17205),#78920,.T.) ;
#85526=ADVANCED_FACE('',(#17206),#16167,.F.) ;
#85527=ADVANCED_FACE('',(#17207),#16168,.F.) ;
#85528=ADVANCED_FACE('',(#17208),#78921,.T.) ;
#85529=ADVANCED_FACE('',(#17209),#13599,.F.) ;
#85530=ADVANCED_FACE('',(#17210),#13600,.F.) ;
#85531=ADVANCED_FACE('',(#17211),#13601,.F.) ;
#85532=ADVANCED_FACE('',(#17212),#13602,.F.) ;
#85533=ADVANCED_FACE('',(#17213),#16169,.F.) ;
#85534=ADVANCED_FACE('',(#17214),#16170,.F.) ;
#85535=ADVANCED_FACE('',(#17215),#13603,.F.) ;
#85536=ADVANCED_FACE('',(#17216),#13604,.T.) ;
#85537=ADVANCED_FACE('',(#17217),#78922,.T.) ;
#85538=ADVANCED_FACE('',(#17218),#78923,.T.) ;
#85539=ADVANCED_FACE('',(#17219),#13605,.T.) ;
#85540=ADVANCED_FACE('',(#17220),#13606,.F.) ;
#85541=ADVANCED_FACE('',(#17221),#13607,.F.) ;
#85542=ADVANCED_FACE('',(#17222),#13608,.F.) ;
#85543=ADVANCED_FACE('',(#17223),#13609,.T.) ;
#85544=ADVANCED_FACE('',(#17224),#13610,.T.) ;
#85545=ADVANCED_FACE('',(#17225),#78924,.T.) ;
#85546=ADVANCED_FACE('',(#17226),#16171,.F.) ;
#85547=ADVANCED_FACE('',(#17227),#16172,.F.) ;
#85548=ADVANCED_FACE('',(#17228),#78925,.T.) ;
#85549=ADVANCED_FACE('',(#17229),#13611,.F.) ;
#85550=ADVANCED_FACE('',(#17230),#13612,.F.) ;
#85551=ADVANCED_FACE('',(#17231),#13613,.F.) ;
#85552=ADVANCED_FACE('',(#17232),#13614,.F.) ;
#85553=ADVANCED_FACE('',(#17233),#16173,.F.) ;
#85554=ADVANCED_FACE('',(#17234),#16174,.F.) ;
#85555=ADVANCED_FACE('',(#17235),#13615,.F.) ;
#85556=ADVANCED_FACE('',(#17236),#78926,.F.) ;
#85557=ADVANCED_FACE('',(#17237),#13616,.F.) ;
#85558=ADVANCED_FACE('',(#17238),#16175,.F.) ;
#85559=ADVANCED_FACE('',(#17239),#13617,.F.) ;
#85560=ADVANCED_FACE('',(#17240),#13618,.T.) ;
#85561=ADVANCED_FACE('',(#17241),#78927,.T.) ;
#85562=ADVANCED_FACE('',(#17242),#78928,.T.) ;
#85563=ADVANCED_FACE('',(#17243),#13619,.T.) ;
#85564=ADVANCED_FACE('',(#17244),#78929,.T.) ;
#85565=ADVANCED_FACE('',(#17245),#13620,.F.) ;
#85566=ADVANCED_FACE('',(#17246),#13621,.F.) ;
#85567=ADVANCED_FACE('',(#17247),#16176,.F.) ;
#85568=ADVANCED_FACE('',(#17248),#78930,.F.) ;
#85569=ADVANCED_FACE('',(#17249),#13622,.F.) ;
#85570=ADVANCED_FACE('',(#17250),#13623,.T.) ;
#85571=ADVANCED_FACE('',(#17251),#13624,.T.) ;
#85572=ADVANCED_FACE('',(#17252),#13625,.T.) ;
#85573=ADVANCED_FACE('',(#17253),#13626,.T.) ;
#85574=ADVANCED_FACE('',(#17254),#13627,.T.) ;
#85575=ADVANCED_FACE('',(#17255),#13628,.F.) ;
#85576=ADVANCED_FACE('',(#17256),#13629,.F.) ;
#85577=ADVANCED_FACE('',(#17257),#13630,.T.) ;
#85578=ADVANCED_FACE('',(#17258),#13631,.T.) ;
#85579=ADVANCED_FACE('',(#17259),#13632,.T.) ;
#85580=ADVANCED_FACE('',(#17260),#13633,.T.) ;
#85581=ADVANCED_FACE('',(#17261),#13634,.F.) ;
#85582=ADVANCED_FACE('',(#17262),#16177,.F.) ;
#85583=ADVANCED_FACE('',(#17263),#13635,.F.) ;
#85584=ADVANCED_FACE('',(#17264),#78931,.F.) ;
#85585=ADVANCED_FACE('',(#17265),#42,.F.) ;
#85586=ADVANCED_FACE('',(#17266),#43,.F.) ;
#85587=ADVANCED_FACE('',(#17267),#13636,.F.) ;
#85588=ADVANCED_FACE('',(#17268),#13637,.F.) ;
#85589=ADVANCED_FACE('',(#17269),#44,.F.) ;
#85590=ADVANCED_FACE('',(#17270),#45,.F.) ;
#85591=ADVANCED_FACE('',(#17271),#13638,.F.) ;
#85592=ADVANCED_FACE('',(#17272),#16178,.F.) ;
#85593=ADVANCED_FACE('',(#17273),#78932,.T.) ;
#85594=ADVANCED_FACE('',(#17274),#13639,.T.) ;
#85595=ADVANCED_FACE('',(#17275),#46,.T.) ;
#85596=ADVANCED_FACE('',(#17276),#13640,.T.) ;
#85597=ADVANCED_FACE('',(#17277),#47,.T.) ;
#85598=ADVANCED_FACE('',(#17278),#48,.F.) ;
#85599=ADVANCED_FACE('',(#17279),#49,.F.) ;
#85600=ADVANCED_FACE('',(#17280),#50,.F.) ;
#85601=ADVANCED_FACE('',(#17281),#51,.F.) ;
#85602=ADVANCED_FACE('',(#17282),#856,.F.) ;
#85603=ADVANCED_FACE('',(#17283),#857,.T.) ;
#85604=ADVANCED_FACE('',(#17284),#13641,.T.) ;
#85605=ADVANCED_FACE('',(#17285),#858,.T.) ;
#85606=ADVANCED_FACE('',(#17286),#13642,.T.) ;
#85607=ADVANCED_FACE('',(#17287),#859,.T.) ;
#85608=ADVANCED_FACE('',(#17288),#13643,.T.) ;
#85609=ADVANCED_FACE('',(#17289),#860,.T.) ;
#85610=ADVANCED_FACE('',(#17290),#13644,.F.) ;
#85611=ADVANCED_FACE('',(#17291),#861,.T.) ;
#85612=ADVANCED_FACE('',(#17292),#862,.F.) ;
#85613=ADVANCED_FACE('',(#17293),#863,.T.) ;
#85614=ADVANCED_FACE('',(#17294),#864,.F.) ;
#85615=ADVANCED_FACE('',(#17295),#865,.F.) ;
#85616=ADVANCED_FACE('',(#17296),#866,.T.) ;
#85617=ADVANCED_FACE('',(#17297),#867,.F.) ;
#85618=ADVANCED_FACE('',(#17298),#868,.F.) ;
#85619=ADVANCED_FACE('',(#17299),#869,.T.) ;
#85620=ADVANCED_FACE('',(#17300),#870,.T.) ;
#85621=ADVANCED_FACE('',(#17301),#871,.T.) ;
#85622=ADVANCED_FACE('',(#17302),#872,.T.) ;
#85623=ADVANCED_FACE('',(#17303),#873,.T.) ;
#85624=ADVANCED_FACE('',(#17304),#874,.F.) ;
#85625=ADVANCED_FACE('',(#17305),#875,.T.) ;
#85626=ADVANCED_FACE('',(#17306),#876,.T.) ;
#85627=ADVANCED_FACE('',(#17307),#877,.F.) ;
#85628=ADVANCED_FACE('',(#17308),#878,.F.) ;
#85629=ADVANCED_FACE('',(#17309),#879,.F.) ;
#85630=ADVANCED_FACE('',(#17310),#880,.F.) ;
#85631=ADVANCED_FACE('',(#17311),#881,.F.) ;
#85632=ADVANCED_FACE('',(#17312,#660),#882,.T.) ;
#85633=ADVANCED_FACE('',(#17313),#13645,.T.) ;
#85634=ADVANCED_FACE('',(#17314),#883,.T.) ;
#85635=ADVANCED_FACE('',(#17315),#13646,.T.) ;
#85636=ADVANCED_FACE('',(#17316),#884,.T.) ;
#85637=ADVANCED_FACE('',(#17317),#13647,.T.) ;
#85638=ADVANCED_FACE('',(#17318),#885,.T.) ;
#85639=ADVANCED_FACE('',(#17319),#13648,.T.) ;
#85640=ADVANCED_FACE('',(#17320),#886,.T.) ;
#85641=ADVANCED_FACE('',(#17321),#887,.T.) ;
#85642=ADVANCED_FACE('',(#17322),#888,.T.) ;
#85643=ADVANCED_FACE('',(#17323),#889,.F.) ;
#85644=ADVANCED_FACE('',(#17324),#890,.F.) ;
#85645=ADVANCED_FACE('',(#17325),#891,.T.) ;
#85646=ADVANCED_FACE('',(#17326),#892,.F.) ;
#85647=ADVANCED_FACE('',(#17327),#893,.F.) ;
#85648=ADVANCED_FACE('',(#17328),#894,.F.) ;
#85649=ADVANCED_FACE('',(#17329),#895,.F.) ;
#85650=ADVANCED_FACE('',(#17330,#661),#896,.T.) ;
#85651=ADVANCED_FACE('',(#17331),#13649,.T.) ;
#85652=ADVANCED_FACE('',(#17332),#897,.T.) ;
#85653=ADVANCED_FACE('',(#17333),#13650,.T.) ;
#85654=ADVANCED_FACE('',(#17334),#898,.T.) ;
#85655=ADVANCED_FACE('',(#17335),#13651,.T.) ;
#85656=ADVANCED_FACE('',(#17336),#899,.T.) ;
#85657=ADVANCED_FACE('',(#17337),#13652,.T.) ;
#85658=ADVANCED_FACE('',(#17338),#900,.T.) ;
#85659=ADVANCED_FACE('',(#17339),#901,.T.) ;
#85660=ADVANCED_FACE('',(#17340),#902,.F.) ;
#85661=ADVANCED_FACE('',(#17341),#903,.F.) ;
#85662=ADVANCED_FACE('',(#17342),#904,.F.) ;
#85663=ADVANCED_FACE('',(#17343),#905,.F.) ;
#85664=ADVANCED_FACE('',(#17344),#906,.T.) ;
#85665=ADVANCED_FACE('',(#17345),#13653,.T.) ;
#85666=ADVANCED_FACE('',(#17346),#52,.T.) ;
#85667=ADVANCED_FACE('',(#17347),#13654,.F.) ;
#85668=ADVANCED_FACE('',(#17348),#53,.F.) ;
#85669=ADVANCED_FACE('',(#17349),#13655,.F.) ;
#85670=ADVANCED_FACE('',(#17350),#13656,.F.) ;
#85671=ADVANCED_FACE('',(#17351),#13657,.T.) ;
#85672=ADVANCED_FACE('',(#17352),#13658,.T.) ;
#85673=ADVANCED_FACE('',(#17353),#13659,.T.) ;
#85674=ADVANCED_FACE('',(#17354),#13660,.F.) ;
#85675=ADVANCED_FACE('',(#17355),#16179,.F.) ;
#85676=ADVANCED_FACE('',(#17356),#54,.T.) ;
#85677=ADVANCED_FACE('',(#17357),#55,.T.) ;
#85678=ADVANCED_FACE('',(#17358),#56,.F.) ;
#85679=ADVANCED_FACE('',(#17359),#13661,.F.) ;
#85680=ADVANCED_FACE('',(#17360),#13662,.F.) ;
#85681=ADVANCED_FACE('',(#17361),#13663,.T.) ;
#85682=ADVANCED_FACE('',(#17362),#13664,.T.) ;
#85683=ADVANCED_FACE('',(#17363),#13665,.F.) ;
#85684=ADVANCED_FACE('',(#17364),#13666,.F.) ;
#85685=ADVANCED_FACE('',(#17365),#16180,.F.) ;
#85686=ADVANCED_FACE('',(#17366),#57,.T.) ;
#85687=ADVANCED_FACE('',(#17367),#16181,.F.) ;
#85688=ADVANCED_FACE('',(#17368),#13667,.F.) ;
#85689=ADVANCED_FACE('',(#17369),#13668,.F.) ;
#85690=ADVANCED_FACE('',(#17370),#13669,.F.) ;
#85691=ADVANCED_FACE('',(#17371),#13670,.F.) ;
#85692=ADVANCED_FACE('',(#17372),#58,.F.) ;
#85693=ADVANCED_FACE('',(#17373),#16182,.F.) ;
#85694=ADVANCED_FACE('',(#17374),#13671,.T.) ;
#85695=ADVANCED_FACE('',(#17375),#13672,.F.) ;
#85696=ADVANCED_FACE('',(#17376),#59,.F.) ;
#85697=ADVANCED_FACE('',(#17377),#13673,.F.) ;
#85698=ADVANCED_FACE('',(#17378),#13674,.T.) ;
#85699=ADVANCED_FACE('',(#17379),#13675,.T.) ;
#85700=ADVANCED_FACE('',(#17380),#13676,.F.) ;
#85701=ADVANCED_FACE('',(#17381),#13677,.T.) ;
#85702=ADVANCED_FACE('',(#17382),#13678,.T.) ;
#85703=ADVANCED_FACE('',(#17383),#13679,.F.) ;
#85704=ADVANCED_FACE('',(#17384),#78933,.T.) ;
#85705=ADVANCED_FACE('',(#17385),#13680,.T.) ;
#85706=ADVANCED_FACE('',(#17386),#13681,.T.) ;
#85707=ADVANCED_FACE('',(#17387),#13682,.T.) ;
#85708=ADVANCED_FACE('',(#17388),#16183,.T.) ;
#85709=ADVANCED_FACE('',(#17389),#13683,.T.) ;
#85710=ADVANCED_FACE('',(#17390),#13684,.T.) ;
#85711=ADVANCED_FACE('',(#17391),#16184,.T.) ;
#85712=ADVANCED_FACE('',(#17392),#16185,.T.) ;
#85713=ADVANCED_FACE('',(#17393),#13685,.T.) ;
#85714=ADVANCED_FACE('',(#17394),#13686,.T.) ;
#85715=ADVANCED_FACE('',(#17395),#16186,.T.) ;
#85716=ADVANCED_FACE('',(#17396),#13687,.T.) ;
#85717=ADVANCED_FACE('',(#17397),#78934,.T.) ;
#85718=ADVANCED_FACE('',(#17398),#78935,.T.) ;
#85719=ADVANCED_FACE('',(#17399),#13688,.T.) ;
#85720=ADVANCED_FACE('',(#17400),#13689,.F.) ;
#85721=ADVANCED_FACE('',(#17401),#13690,.F.) ;
#85722=ADVANCED_FACE('',(#17402),#13691,.F.) ;
#85723=ADVANCED_FACE('',(#17403),#13692,.T.) ;
#85724=ADVANCED_FACE('',(#17404),#13693,.T.) ;
#85725=ADVANCED_FACE('',(#17405),#78936,.T.) ;
#85726=ADVANCED_FACE('',(#17406),#16187,.F.) ;
#85727=ADVANCED_FACE('',(#17407),#16188,.F.) ;
#85728=ADVANCED_FACE('',(#17408),#78937,.T.) ;
#85729=ADVANCED_FACE('',(#17409),#13694,.F.) ;
#85730=ADVANCED_FACE('',(#17410),#13695,.F.) ;
#85731=ADVANCED_FACE('',(#17411),#13696,.F.) ;
#85732=ADVANCED_FACE('',(#17412),#13697,.F.) ;
#85733=ADVANCED_FACE('',(#17413),#16189,.F.) ;
#85734=ADVANCED_FACE('',(#17414),#16190,.F.) ;
#85735=ADVANCED_FACE('',(#17415),#13698,.F.) ;
#85736=ADVANCED_FACE('',(#17416),#13699,.T.) ;
#85737=ADVANCED_FACE('',(#17417),#78938,.T.) ;
#85738=ADVANCED_FACE('',(#17418),#78939,.T.) ;
#85739=ADVANCED_FACE('',(#17419),#13700,.T.) ;
#85740=ADVANCED_FACE('',(#17420),#13701,.F.) ;
#85741=ADVANCED_FACE('',(#17421),#13702,.F.) ;
#85742=ADVANCED_FACE('',(#17422),#13703,.F.) ;
#85743=ADVANCED_FACE('',(#17423),#13704,.T.) ;
#85744=ADVANCED_FACE('',(#17424),#13705,.T.) ;
#85745=ADVANCED_FACE('',(#17425),#78940,.T.) ;
#85746=ADVANCED_FACE('',(#17426),#16191,.F.) ;
#85747=ADVANCED_FACE('',(#17427),#16192,.F.) ;
#85748=ADVANCED_FACE('',(#17428),#78941,.T.) ;
#85749=ADVANCED_FACE('',(#17429),#13706,.F.) ;
#85750=ADVANCED_FACE('',(#17430),#13707,.F.) ;
#85751=ADVANCED_FACE('',(#17431),#13708,.F.) ;
#85752=ADVANCED_FACE('',(#17432),#13709,.F.) ;
#85753=ADVANCED_FACE('',(#17433),#16193,.F.) ;
#85754=ADVANCED_FACE('',(#17434),#16194,.F.) ;
#85755=ADVANCED_FACE('',(#17435),#13710,.F.) ;
#85756=ADVANCED_FACE('',(#17436),#78942,.F.) ;
#85757=ADVANCED_FACE('',(#17437),#16195,.F.) ;
#85758=ADVANCED_FACE('',(#17438),#13711,.F.) ;
#85759=ADVANCED_FACE('',(#17439),#78943,.T.) ;
#85760=ADVANCED_FACE('',(#17440),#78944,.T.) ;
#85761=ADVANCED_FACE('',(#17441),#13712,.T.) ;
#85762=ADVANCED_FACE('',(#17442),#78945,.T.) ;
#85763=ADVANCED_FACE('',(#17443),#13713,.F.) ;
#85764=ADVANCED_FACE('',(#17444),#13714,.F.) ;
#85765=ADVANCED_FACE('',(#17445),#16196,.F.) ;
#85766=ADVANCED_FACE('',(#17446),#78946,.F.) ;
#85767=ADVANCED_FACE('',(#17447),#13715,.F.) ;
#85768=ADVANCED_FACE('',(#17448),#13716,.F.) ;
#85769=ADVANCED_FACE('',(#17449),#13717,.T.) ;
#85770=ADVANCED_FACE('',(#17450),#13718,.T.) ;
#85771=ADVANCED_FACE('',(#17451),#16197,.F.) ;
#85772=ADVANCED_FACE('',(#17452),#13719,.F.) ;
#85773=ADVANCED_FACE('',(#17453),#78947,.F.) ;
#85774=ADVANCED_FACE('',(#17454),#60,.F.) ;
#85775=ADVANCED_FACE('',(#17455),#61,.F.) ;
#85776=ADVANCED_FACE('',(#17456),#13720,.F.) ;
#85777=ADVANCED_FACE('',(#17457),#62,.F.) ;
#85778=ADVANCED_FACE('',(#17458),#63,.F.) ;
#85779=ADVANCED_FACE('',(#17459),#13721,.F.) ;
#85780=ADVANCED_FACE('',(#17460),#16198,.F.) ;
#85781=ADVANCED_FACE('',(#17461),#78948,.T.) ;
#85782=ADVANCED_FACE('',(#17462),#64,.T.) ;
#85783=ADVANCED_FACE('',(#17463),#13722,.T.) ;
#85784=ADVANCED_FACE('',(#17464),#65,.T.) ;
#85785=ADVANCED_FACE('',(#17465),#66,.F.) ;
#85786=ADVANCED_FACE('',(#17466),#67,.F.) ;
#85787=ADVANCED_FACE('',(#17467),#68,.F.) ;
#85788=ADVANCED_FACE('',(#17468),#69,.F.) ;
#85789=ADVANCED_FACE('',(#17469),#16199,.T.) ;
#85790=ADVANCED_FACE('',(#17470),#16200,.T.) ;
#85791=ADVANCED_FACE('',(#17471),#13723,.T.) ;
#85792=ADVANCED_FACE('',(#17472),#13724,.T.) ;
#85793=ADVANCED_FACE('',(#17473),#13725,.T.) ;
#85794=ADVANCED_FACE('',(#17474),#13726,.T.) ;
#85795=ADVANCED_FACE('',(#17475),#16201,.T.) ;
#85796=ADVANCED_FACE('',(#17476),#16202,.T.) ;
#85797=ADVANCED_FACE('',(#17477),#16203,.T.) ;
#85798=ADVANCED_FACE('',(#17478),#16204,.T.) ;
#85799=ADVANCED_FACE('',(#17479),#13727,.T.) ;
#85800=ADVANCED_FACE('',(#17480),#13728,.T.) ;
#85801=ADVANCED_FACE('',(#17481),#13729,.F.) ;
#85802=ADVANCED_FACE('',(#17482),#13730,.T.) ;
#85803=ADVANCED_FACE('',(#17483),#13731,.T.) ;
#85804=ADVANCED_FACE('',(#17484),#78949,.T.) ;
#85805=ADVANCED_FACE('',(#17485),#70,.F.) ;
#85806=ADVANCED_FACE('',(#17486),#71,.F.) ;
#85807=ADVANCED_FACE('',(#17487),#78950,.T.) ;
#85808=ADVANCED_FACE('',(#17488),#13732,.T.) ;
#85809=ADVANCED_FACE('',(#17489),#13733,.F.) ;
#85810=ADVANCED_FACE('',(#17490),#13734,.F.) ;
#85811=ADVANCED_FACE('',(#17491),#13735,.T.) ;
#85812=ADVANCED_FACE('',(#17492),#78951,.F.) ;
#85813=ADVANCED_FACE('',(#17493),#78952,.F.) ;
#85814=ADVANCED_FACE('',(#17494),#13736,.F.) ;
#85815=ADVANCED_FACE('',(#17495),#78953,.F.) ;
#85816=ADVANCED_FACE('',(#17496),#78954,.T.) ;
#85817=ADVANCED_FACE('',(#17497),#78955,.F.) ;
#85818=ADVANCED_FACE('',(#17498),#78956,.T.) ;
#85819=ADVANCED_FACE('',(#17499),#78957,.T.) ;
#85820=ADVANCED_FACE('',(#17500),#16205,.T.) ;
#85821=ADVANCED_FACE('',(#17501),#13737,.F.) ;
#85822=ADVANCED_FACE('',(#17502),#16206,.T.) ;
#85823=ADVANCED_FACE('',(#17503),#2417,.F.) ;
#85824=ADVANCED_FACE('',(#17504),#13738,.F.) ;
#85825=ADVANCED_FACE('',(#17505),#13739,.F.) ;
#85826=ADVANCED_FACE('',(#17506),#78958,.F.) ;
#85827=ADVANCED_FACE('',(#17507),#13740,.F.) ;
#85828=ADVANCED_FACE('',(#17508),#78959,.T.) ;
#85829=ADVANCED_FACE('',(#17509),#78960,.F.) ;
#85830=ADVANCED_FACE('',(#17510),#78961,.T.) ;
#85831=ADVANCED_FACE('',(#17511),#78962,.T.) ;
#85832=ADVANCED_FACE('',(#17512),#16207,.T.) ;
#85833=ADVANCED_FACE('',(#17513),#13741,.F.) ;
#85834=ADVANCED_FACE('',(#17514),#16208,.T.) ;
#85835=ADVANCED_FACE('',(#17515),#2418,.F.) ;
#85836=ADVANCED_FACE('',(#17516),#13742,.F.) ;
#85837=ADVANCED_FACE('',(#17517),#13743,.F.) ;
#85838=ADVANCED_FACE('',(#17518,#662),#907,.F.) ;
#85839=ADVANCED_FACE('',(#17519),#908,.F.) ;
#85840=ADVANCED_FACE('',(#17520),#909,.F.) ;
#85841=ADVANCED_FACE('',(#17521),#910,.F.) ;
#85842=ADVANCED_FACE('',(#17522),#13744,.T.) ;
#85843=ADVANCED_FACE('',(#17523),#13745,.F.) ;
#85844=ADVANCED_FACE('',(#17524),#13746,.F.) ;
#85845=ADVANCED_FACE('',(#17525),#13747,.T.) ;
#85846=ADVANCED_FACE('',(#17526),#911,.F.) ;
#85847=ADVANCED_FACE('',(#17527),#912,.F.) ;
#85848=ADVANCED_FACE('',(#17528),#913,.F.) ;
#85849=ADVANCED_FACE('',(#17529),#914,.T.) ;
#85850=ADVANCED_FACE('',(#17530,#663,#664),#915,.F.) ;
#85851=ADVANCED_FACE('',(#17531),#916,.F.) ;
#85852=ADVANCED_FACE('',(#17532),#917,.F.) ;
#85853=ADVANCED_FACE('',(#17533),#918,.F.) ;
#85854=ADVANCED_FACE('',(#17534),#919,.F.) ;
#85855=ADVANCED_FACE('',(#17535,#665,#666,#667,#668),#920,.F.) ;
#85856=ADVANCED_FACE('',(#17536),#921,.F.) ;
#85857=ADVANCED_FACE('',(#17537),#922,.F.) ;
#85858=ADVANCED_FACE('',(#17538),#923,.F.) ;
#85859=ADVANCED_FACE('',(#17539,#669,#670),#924,.F.) ;
#85860=ADVANCED_FACE('',(#17540,#671,#672),#925,.F.) ;
#85861=ADVANCED_FACE('',(#17541),#926,.F.) ;
#85862=ADVANCED_FACE('',(#17542),#927,.F.) ;
#85863=ADVANCED_FACE('',(#17543),#928,.F.) ;
#85864=ADVANCED_FACE('',(#17544),#929,.F.) ;
#85865=ADVANCED_FACE('',(#17545),#930,.F.) ;
#85866=ADVANCED_FACE('',(#17546),#931,.T.) ;
#85867=ADVANCED_FACE('',(#17547),#932,.T.) ;
#85868=ADVANCED_FACE('',(#17548),#933,.T.) ;
#85869=ADVANCED_FACE('',(#17549),#934,.T.) ;
#85870=ADVANCED_FACE('',(#17550),#935,.T.) ;
#85871=ADVANCED_FACE('',(#17551),#936,.F.) ;
#85872=ADVANCED_FACE('',(#17552),#937,.T.) ;
#85873=ADVANCED_FACE('',(#17553),#938,.T.) ;
#85874=ADVANCED_FACE('',(#17554),#939,.F.) ;
#85875=ADVANCED_FACE('',(#17555),#940,.F.) ;
#85876=ADVANCED_FACE('',(#17556),#941,.F.) ;
#85877=ADVANCED_FACE('',(#17557),#942,.F.) ;
#85878=ADVANCED_FACE('',(#17558),#943,.F.) ;
#85879=ADVANCED_FACE('',(#17559,#673),#944,.T.) ;
#85880=ADVANCED_FACE('',(#17560),#13748,.T.) ;
#85881=ADVANCED_FACE('',(#17561),#945,.T.) ;
#85882=ADVANCED_FACE('',(#17562),#13749,.T.) ;
#85883=ADVANCED_FACE('',(#17563),#946,.T.) ;
#85884=ADVANCED_FACE('',(#17564),#13750,.T.) ;
#85885=ADVANCED_FACE('',(#17565),#947,.T.) ;
#85886=ADVANCED_FACE('',(#17566),#13751,.T.) ;
#85887=ADVANCED_FACE('',(#17567),#948,.T.) ;
#85888=ADVANCED_FACE('',(#17568),#949,.T.) ;
#85889=ADVANCED_FACE('',(#17569),#950,.T.) ;
#85890=ADVANCED_FACE('',(#17570),#951,.F.) ;
#85891=ADVANCED_FACE('',(#17571),#952,.F.) ;
#85892=ADVANCED_FACE('',(#17572),#953,.T.) ;
#85893=ADVANCED_FACE('',(#17573),#954,.F.) ;
#85894=ADVANCED_FACE('',(#17574),#955,.F.) ;
#85895=ADVANCED_FACE('',(#17575),#956,.F.) ;
#85896=ADVANCED_FACE('',(#17576),#957,.F.) ;
#85897=ADVANCED_FACE('',(#17577,#674),#958,.T.) ;
#85898=ADVANCED_FACE('',(#17578),#13752,.T.) ;
#85899=ADVANCED_FACE('',(#17579),#959,.T.) ;
#85900=ADVANCED_FACE('',(#17580),#13753,.T.) ;
#85901=ADVANCED_FACE('',(#17581),#960,.T.) ;
#85902=ADVANCED_FACE('',(#17582),#13754,.T.) ;
#85903=ADVANCED_FACE('',(#17583),#961,.T.) ;
#85904=ADVANCED_FACE('',(#17584),#13755,.T.) ;
#85905=ADVANCED_FACE('',(#17585),#962,.T.) ;
#85906=ADVANCED_FACE('',(#17586),#963,.T.) ;
#85907=ADVANCED_FACE('',(#17587),#964,.F.) ;
#85908=ADVANCED_FACE('',(#17588),#965,.F.) ;
#85909=ADVANCED_FACE('',(#17589),#966,.F.) ;
#85910=ADVANCED_FACE('',(#17590),#967,.F.) ;
#85911=ADVANCED_FACE('',(#17591),#968,.T.) ;
#85912=ADVANCED_FACE('',(#17592),#13756,.T.) ;
#85913=ADVANCED_FACE('',(#17593),#72,.T.) ;
#85914=ADVANCED_FACE('',(#17594),#13757,.F.) ;
#85915=ADVANCED_FACE('',(#17595),#73,.F.) ;
#85916=ADVANCED_FACE('',(#17596),#13758,.F.) ;
#85917=ADVANCED_FACE('',(#17597),#13759,.F.) ;
#85918=ADVANCED_FACE('',(#17598),#13760,.T.) ;
#85919=ADVANCED_FACE('',(#17599),#13761,.T.) ;
#85920=ADVANCED_FACE('',(#17600),#13762,.T.) ;
#85921=ADVANCED_FACE('',(#17601),#13763,.F.) ;
#85922=ADVANCED_FACE('',(#17602),#16209,.F.) ;
#85923=ADVANCED_FACE('',(#17603),#74,.T.) ;
#85924=ADVANCED_FACE('',(#17604),#75,.T.) ;
#85925=ADVANCED_FACE('',(#17605),#76,.F.) ;
#85926=ADVANCED_FACE('',(#17606),#13764,.F.) ;
#85927=ADVANCED_FACE('',(#17607),#13765,.F.) ;
#85928=ADVANCED_FACE('',(#17608),#13766,.T.) ;
#85929=ADVANCED_FACE('',(#17609),#13767,.T.) ;
#85930=ADVANCED_FACE('',(#17610),#13768,.F.) ;
#85931=ADVANCED_FACE('',(#17611),#13769,.F.) ;
#85932=ADVANCED_FACE('',(#17612),#16210,.F.) ;
#85933=ADVANCED_FACE('',(#17613),#77,.T.) ;
#85934=ADVANCED_FACE('',(#17614),#16211,.F.) ;
#85935=ADVANCED_FACE('',(#17615),#13770,.F.) ;
#85936=ADVANCED_FACE('',(#17616),#13771,.F.) ;
#85937=ADVANCED_FACE('',(#17617),#13772,.F.) ;
#85938=ADVANCED_FACE('',(#17618),#13773,.F.) ;
#85939=ADVANCED_FACE('',(#17619),#78,.F.) ;
#85940=ADVANCED_FACE('',(#17620),#16212,.F.) ;
#85941=ADVANCED_FACE('',(#17621),#13774,.T.) ;
#85942=ADVANCED_FACE('',(#17622),#13775,.F.) ;
#85943=ADVANCED_FACE('',(#17623),#79,.F.) ;
#85944=ADVANCED_FACE('',(#17624),#13776,.F.) ;
#85945=ADVANCED_FACE('',(#17625),#13777,.T.) ;
#85946=ADVANCED_FACE('',(#17626),#13778,.T.) ;
#85947=ADVANCED_FACE('',(#17627),#13779,.F.) ;
#85948=ADVANCED_FACE('',(#17628),#13780,.T.) ;
#85949=ADVANCED_FACE('',(#17629),#13781,.T.) ;
#85950=ADVANCED_FACE('',(#17630),#13782,.F.) ;
#85951=ADVANCED_FACE('',(#17631),#78963,.T.) ;
#85952=ADVANCED_FACE('',(#17632),#13783,.T.) ;
#85953=ADVANCED_FACE('',(#17633),#13784,.T.) ;
#85954=ADVANCED_FACE('',(#17634),#13785,.T.) ;
#85955=ADVANCED_FACE('',(#17635),#13786,.T.) ;
#85956=ADVANCED_FACE('',(#17636),#16213,.T.) ;
#85957=ADVANCED_FACE('',(#17637),#13787,.T.) ;
#85958=ADVANCED_FACE('',(#17638),#13788,.T.) ;
#85959=ADVANCED_FACE('',(#17639),#16214,.T.) ;
#85960=ADVANCED_FACE('',(#17640),#16215,.T.) ;
#85961=ADVANCED_FACE('',(#17641),#13789,.T.) ;
#85962=ADVANCED_FACE('',(#17642),#13790,.T.) ;
#85963=ADVANCED_FACE('',(#17643),#16216,.T.) ;
#85964=ADVANCED_FACE('',(#17644),#13791,.T.) ;
#85965=ADVANCED_FACE('',(#17645),#78964,.T.) ;
#85966=ADVANCED_FACE('',(#17646),#78965,.T.) ;
#85967=ADVANCED_FACE('',(#17647),#13792,.T.) ;
#85968=ADVANCED_FACE('',(#17648),#13793,.F.) ;
#85969=ADVANCED_FACE('',(#17649),#13794,.F.) ;
#85970=ADVANCED_FACE('',(#17650),#13795,.F.) ;
#85971=ADVANCED_FACE('',(#17651),#13796,.T.) ;
#85972=ADVANCED_FACE('',(#17652),#13797,.T.) ;
#85973=ADVANCED_FACE('',(#17653),#78966,.T.) ;
#85974=ADVANCED_FACE('',(#17654),#16217,.F.) ;
#85975=ADVANCED_FACE('',(#17655),#16218,.F.) ;
#85976=ADVANCED_FACE('',(#17656),#78967,.T.) ;
#85977=ADVANCED_FACE('',(#17657),#13798,.F.) ;
#85978=ADVANCED_FACE('',(#17658),#13799,.F.) ;
#85979=ADVANCED_FACE('',(#17659),#13800,.F.) ;
#85980=ADVANCED_FACE('',(#17660),#13801,.F.) ;
#85981=ADVANCED_FACE('',(#17661),#16219,.F.) ;
#85982=ADVANCED_FACE('',(#17662),#16220,.F.) ;
#85983=ADVANCED_FACE('',(#17663),#13802,.F.) ;
#85984=ADVANCED_FACE('',(#17664),#13803,.T.) ;
#85985=ADVANCED_FACE('',(#17665),#78968,.T.) ;
#85986=ADVANCED_FACE('',(#17666),#78969,.T.) ;
#85987=ADVANCED_FACE('',(#17667),#13804,.T.) ;
#85988=ADVANCED_FACE('',(#17668),#13805,.F.) ;
#85989=ADVANCED_FACE('',(#17669),#13806,.F.) ;
#85990=ADVANCED_FACE('',(#17670),#13807,.F.) ;
#85991=ADVANCED_FACE('',(#17671),#13808,.T.) ;
#85992=ADVANCED_FACE('',(#17672),#13809,.T.) ;
#85993=ADVANCED_FACE('',(#17673),#78970,.T.) ;
#85994=ADVANCED_FACE('',(#17674),#16221,.F.) ;
#85995=ADVANCED_FACE('',(#17675),#16222,.F.) ;
#85996=ADVANCED_FACE('',(#17676),#78971,.T.) ;
#85997=ADVANCED_FACE('',(#17677),#13810,.F.) ;
#85998=ADVANCED_FACE('',(#17678),#13811,.F.) ;
#85999=ADVANCED_FACE('',(#17679),#13812,.F.) ;
#86000=ADVANCED_FACE('',(#17680),#13813,.F.) ;
#86001=ADVANCED_FACE('',(#17681),#16223,.F.) ;
#86002=ADVANCED_FACE('',(#17682),#16224,.F.) ;
#86003=ADVANCED_FACE('',(#17683),#13814,.F.) ;
#86004=ADVANCED_FACE('',(#17684),#78972,.F.) ;
#86005=ADVANCED_FACE('',(#17685),#13815,.F.) ;
#86006=ADVANCED_FACE('',(#17686),#16225,.F.) ;
#86007=ADVANCED_FACE('',(#17687),#13816,.F.) ;
#86008=ADVANCED_FACE('',(#17688),#13817,.T.) ;
#86009=ADVANCED_FACE('',(#17689),#78973,.T.) ;
#86010=ADVANCED_FACE('',(#17690),#78974,.T.) ;
#86011=ADVANCED_FACE('',(#17691),#13818,.T.) ;
#86012=ADVANCED_FACE('',(#17692),#78975,.T.) ;
#86013=ADVANCED_FACE('',(#17693),#13819,.F.) ;
#86014=ADVANCED_FACE('',(#17694),#13820,.F.) ;
#86015=ADVANCED_FACE('',(#17695),#16226,.F.) ;
#86016=ADVANCED_FACE('',(#17696),#78976,.F.) ;
#86017=ADVANCED_FACE('',(#17697),#13821,.F.) ;
#86018=ADVANCED_FACE('',(#17698),#13822,.T.) ;
#86019=ADVANCED_FACE('',(#17699),#13823,.T.) ;
#86020=ADVANCED_FACE('',(#17700),#13824,.T.) ;
#86021=ADVANCED_FACE('',(#17701),#13825,.T.) ;
#86022=ADVANCED_FACE('',(#17702),#13826,.T.) ;
#86023=ADVANCED_FACE('',(#17703),#13827,.F.) ;
#86024=ADVANCED_FACE('',(#17704),#13828,.F.) ;
#86025=ADVANCED_FACE('',(#17705),#13829,.T.) ;
#86026=ADVANCED_FACE('',(#17706),#13830,.T.) ;
#86027=ADVANCED_FACE('',(#17707),#13831,.T.) ;
#86028=ADVANCED_FACE('',(#17708),#13832,.T.) ;
#86029=ADVANCED_FACE('',(#17709),#13833,.F.) ;
#86030=ADVANCED_FACE('',(#17710),#16227,.F.) ;
#86031=ADVANCED_FACE('',(#17711),#13834,.F.) ;
#86032=ADVANCED_FACE('',(#17712),#78977,.F.) ;
#86033=ADVANCED_FACE('',(#17713),#80,.F.) ;
#86034=ADVANCED_FACE('',(#17714),#81,.F.) ;
#86035=ADVANCED_FACE('',(#17715),#13835,.F.) ;
#86036=ADVANCED_FACE('',(#17716),#13836,.F.) ;
#86037=ADVANCED_FACE('',(#17717),#82,.F.) ;
#86038=ADVANCED_FACE('',(#17718),#83,.F.) ;
#86039=ADVANCED_FACE('',(#17719),#13837,.F.) ;
#86040=ADVANCED_FACE('',(#17720),#16228,.F.) ;
#86041=ADVANCED_FACE('',(#17721),#78978,.T.) ;
#86042=ADVANCED_FACE('',(#17722),#13838,.T.) ;
#86043=ADVANCED_FACE('',(#17723),#84,.T.) ;
#86044=ADVANCED_FACE('',(#17724),#13839,.T.) ;
#86045=ADVANCED_FACE('',(#17725),#85,.T.) ;
#86046=ADVANCED_FACE('',(#17726),#86,.F.) ;
#86047=ADVANCED_FACE('',(#17727),#87,.F.) ;
#86048=ADVANCED_FACE('',(#17728),#88,.F.) ;
#86049=ADVANCED_FACE('',(#17729),#89,.F.) ;
#86050=ADVANCED_FACE('',(#17730),#969,.F.) ;
#86051=ADVANCED_FACE('',(#17731),#970,.T.) ;
#86052=ADVANCED_FACE('',(#17732),#13840,.T.) ;
#86053=ADVANCED_FACE('',(#17733),#971,.T.) ;
#86054=ADVANCED_FACE('',(#17734),#13841,.T.) ;
#86055=ADVANCED_FACE('',(#17735),#972,.T.) ;
#86056=ADVANCED_FACE('',(#17736),#13842,.T.) ;
#86057=ADVANCED_FACE('',(#17737),#973,.T.) ;
#86058=ADVANCED_FACE('',(#17738),#13843,.F.) ;
#86059=ADVANCED_FACE('',(#17739),#974,.T.) ;
#86060=ADVANCED_FACE('',(#17740),#975,.F.) ;
#86061=ADVANCED_FACE('',(#17741),#976,.T.) ;
#86062=ADVANCED_FACE('',(#17742),#977,.F.) ;
#86063=ADVANCED_FACE('',(#17743),#978,.T.) ;
#86064=ADVANCED_FACE('',(#17744),#979,.F.) ;
#86065=ADVANCED_FACE('',(#17745),#980,.F.) ;
#86066=ADVANCED_FACE('',(#17746),#981,.T.) ;
#86067=ADVANCED_FACE('',(#17747),#982,.T.) ;
#86068=ADVANCED_FACE('',(#17748),#983,.T.) ;
#86069=ADVANCED_FACE('',(#17749),#984,.T.) ;
#86070=ADVANCED_FACE('',(#17750),#985,.T.) ;
#86071=ADVANCED_FACE('',(#17751),#986,.T.) ;
#86072=ADVANCED_FACE('',(#17752),#987,.F.) ;
#86073=ADVANCED_FACE('',(#17753),#988,.T.) ;
#86074=ADVANCED_FACE('',(#17754),#989,.T.) ;
#86075=ADVANCED_FACE('',(#17755),#990,.F.) ;
#86076=ADVANCED_FACE('',(#17756),#991,.F.) ;
#86077=ADVANCED_FACE('',(#17757),#992,.F.) ;
#86078=ADVANCED_FACE('',(#17758),#993,.F.) ;
#86079=ADVANCED_FACE('',(#17759),#994,.F.) ;
#86080=ADVANCED_FACE('',(#17760,#675),#995,.T.) ;
#86081=ADVANCED_FACE('',(#17761),#13844,.T.) ;
#86082=ADVANCED_FACE('',(#17762),#996,.T.) ;
#86083=ADVANCED_FACE('',(#17763),#13845,.T.) ;
#86084=ADVANCED_FACE('',(#17764),#997,.T.) ;
#86085=ADVANCED_FACE('',(#17765),#13846,.T.) ;
#86086=ADVANCED_FACE('',(#17766),#998,.T.) ;
#86087=ADVANCED_FACE('',(#17767),#13847,.T.) ;
#86088=ADVANCED_FACE('',(#17768),#999,.T.) ;
#86089=ADVANCED_FACE('',(#17769),#1000,.T.) ;
#86090=ADVANCED_FACE('',(#17770),#1001,.T.) ;
#86091=ADVANCED_FACE('',(#17771),#1002,.F.) ;
#86092=ADVANCED_FACE('',(#17772),#1003,.F.) ;
#86093=ADVANCED_FACE('',(#17773),#1004,.T.) ;
#86094=ADVANCED_FACE('',(#17774),#1005,.F.) ;
#86095=ADVANCED_FACE('',(#17775),#1006,.F.) ;
#86096=ADVANCED_FACE('',(#17776),#1007,.F.) ;
#86097=ADVANCED_FACE('',(#17777),#1008,.F.) ;
#86098=ADVANCED_FACE('',(#17778,#676),#1009,.T.) ;
#86099=ADVANCED_FACE('',(#17779),#13848,.T.) ;
#86100=ADVANCED_FACE('',(#17780),#1010,.T.) ;
#86101=ADVANCED_FACE('',(#17781),#13849,.T.) ;
#86102=ADVANCED_FACE('',(#17782),#1011,.T.) ;
#86103=ADVANCED_FACE('',(#17783),#13850,.T.) ;
#86104=ADVANCED_FACE('',(#17784),#1012,.T.) ;
#86105=ADVANCED_FACE('',(#17785),#13851,.T.) ;
#86106=ADVANCED_FACE('',(#17786),#1013,.T.) ;
#86107=ADVANCED_FACE('',(#17787),#1014,.T.) ;
#86108=ADVANCED_FACE('',(#17788),#1015,.F.) ;
#86109=ADVANCED_FACE('',(#17789),#1016,.F.) ;
#86110=ADVANCED_FACE('',(#17790),#1017,.F.) ;
#86111=ADVANCED_FACE('',(#17791),#1018,.F.) ;
#86112=ADVANCED_FACE('',(#17792),#1019,.T.) ;
#86113=ADVANCED_FACE('',(#17793),#13852,.T.) ;
#86114=ADVANCED_FACE('',(#17794),#90,.T.) ;
#86115=ADVANCED_FACE('',(#17795),#13853,.F.) ;
#86116=ADVANCED_FACE('',(#17796),#91,.F.) ;
#86117=ADVANCED_FACE('',(#17797),#13854,.F.) ;
#86118=ADVANCED_FACE('',(#17798),#13855,.F.) ;
#86119=ADVANCED_FACE('',(#17799),#13856,.T.) ;
#86120=ADVANCED_FACE('',(#17800),#13857,.T.) ;
#86121=ADVANCED_FACE('',(#17801),#13858,.T.) ;
#86122=ADVANCED_FACE('',(#17802),#13859,.F.) ;
#86123=ADVANCED_FACE('',(#17803),#16229,.F.) ;
#86124=ADVANCED_FACE('',(#17804),#92,.T.) ;
#86125=ADVANCED_FACE('',(#17805),#93,.T.) ;
#86126=ADVANCED_FACE('',(#17806),#94,.F.) ;
#86127=ADVANCED_FACE('',(#17807),#13860,.F.) ;
#86128=ADVANCED_FACE('',(#17808),#13861,.F.) ;
#86129=ADVANCED_FACE('',(#17809),#13862,.T.) ;
#86130=ADVANCED_FACE('',(#17810),#13863,.T.) ;
#86131=ADVANCED_FACE('',(#17811),#13864,.F.) ;
#86132=ADVANCED_FACE('',(#17812),#13865,.F.) ;
#86133=ADVANCED_FACE('',(#17813),#16230,.F.) ;
#86134=ADVANCED_FACE('',(#17814),#95,.T.) ;
#86135=ADVANCED_FACE('',(#17815),#16231,.F.) ;
#86136=ADVANCED_FACE('',(#17816),#13866,.F.) ;
#86137=ADVANCED_FACE('',(#17817),#13867,.F.) ;
#86138=ADVANCED_FACE('',(#17818),#13868,.F.) ;
#86139=ADVANCED_FACE('',(#17819),#13869,.F.) ;
#86140=ADVANCED_FACE('',(#17820),#96,.F.) ;
#86141=ADVANCED_FACE('',(#17821),#16232,.F.) ;
#86142=ADVANCED_FACE('',(#17822),#13870,.T.) ;
#86143=ADVANCED_FACE('',(#17823),#13871,.F.) ;
#86144=ADVANCED_FACE('',(#17824),#97,.F.) ;
#86145=ADVANCED_FACE('',(#17825),#13872,.F.) ;
#86146=ADVANCED_FACE('',(#17826),#13873,.T.) ;
#86147=ADVANCED_FACE('',(#17827),#13874,.F.) ;
#86148=ADVANCED_FACE('',(#17828),#13875,.T.) ;
#86149=ADVANCED_FACE('',(#17829),#13876,.T.) ;
#86150=ADVANCED_FACE('',(#17830),#13877,.F.) ;
#86151=ADVANCED_FACE('',(#17831),#78979,.T.) ;
#86152=ADVANCED_FACE('',(#17832),#13878,.T.) ;
#86153=ADVANCED_FACE('',(#17833),#13879,.T.) ;
#86154=ADVANCED_FACE('',(#17834),#13880,.T.) ;
#86155=ADVANCED_FACE('',(#17835),#13881,.T.) ;
#86156=ADVANCED_FACE('',(#17836),#16233,.T.) ;
#86157=ADVANCED_FACE('',(#17837),#13882,.T.) ;
#86158=ADVANCED_FACE('',(#17838),#13883,.T.) ;
#86159=ADVANCED_FACE('',(#17839),#16234,.T.) ;
#86160=ADVANCED_FACE('',(#17840),#16235,.T.) ;
#86161=ADVANCED_FACE('',(#17841),#13884,.T.) ;
#86162=ADVANCED_FACE('',(#17842),#13885,.T.) ;
#86163=ADVANCED_FACE('',(#17843),#16236,.T.) ;
#86164=ADVANCED_FACE('',(#17844),#13886,.T.) ;
#86165=ADVANCED_FACE('',(#17845),#78980,.T.) ;
#86166=ADVANCED_FACE('',(#17846),#78981,.T.) ;
#86167=ADVANCED_FACE('',(#17847),#13887,.T.) ;
#86168=ADVANCED_FACE('',(#17848),#13888,.F.) ;
#86169=ADVANCED_FACE('',(#17849),#13889,.F.) ;
#86170=ADVANCED_FACE('',(#17850),#13890,.F.) ;
#86171=ADVANCED_FACE('',(#17851),#13891,.T.) ;
#86172=ADVANCED_FACE('',(#17852),#13892,.T.) ;
#86173=ADVANCED_FACE('',(#17853),#78982,.T.) ;
#86174=ADVANCED_FACE('',(#17854),#16237,.F.) ;
#86175=ADVANCED_FACE('',(#17855),#16238,.F.) ;
#86176=ADVANCED_FACE('',(#17856),#78983,.T.) ;
#86177=ADVANCED_FACE('',(#17857),#13893,.F.) ;
#86178=ADVANCED_FACE('',(#17858),#13894,.F.) ;
#86179=ADVANCED_FACE('',(#17859),#13895,.F.) ;
#86180=ADVANCED_FACE('',(#17860),#13896,.F.) ;
#86181=ADVANCED_FACE('',(#17861),#16239,.F.) ;
#86182=ADVANCED_FACE('',(#17862),#16240,.F.) ;
#86183=ADVANCED_FACE('',(#17863),#13897,.F.) ;
#86184=ADVANCED_FACE('',(#17864),#13898,.T.) ;
#86185=ADVANCED_FACE('',(#17865),#78984,.T.) ;
#86186=ADVANCED_FACE('',(#17866),#78985,.T.) ;
#86187=ADVANCED_FACE('',(#17867),#13899,.T.) ;
#86188=ADVANCED_FACE('',(#17868),#13900,.F.) ;
#86189=ADVANCED_FACE('',(#17869),#13901,.F.) ;
#86190=ADVANCED_FACE('',(#17870),#13902,.F.) ;
#86191=ADVANCED_FACE('',(#17871),#13903,.T.) ;
#86192=ADVANCED_FACE('',(#17872),#13904,.T.) ;
#86193=ADVANCED_FACE('',(#17873),#78986,.T.) ;
#86194=ADVANCED_FACE('',(#17874),#16241,.F.) ;
#86195=ADVANCED_FACE('',(#17875),#16242,.F.) ;
#86196=ADVANCED_FACE('',(#17876),#78987,.T.) ;
#86197=ADVANCED_FACE('',(#17877),#13905,.F.) ;
#86198=ADVANCED_FACE('',(#17878),#13906,.F.) ;
#86199=ADVANCED_FACE('',(#17879),#13907,.F.) ;
#86200=ADVANCED_FACE('',(#17880),#13908,.F.) ;
#86201=ADVANCED_FACE('',(#17881),#16243,.F.) ;
#86202=ADVANCED_FACE('',(#17882),#16244,.F.) ;
#86203=ADVANCED_FACE('',(#17883),#13909,.F.) ;
#86204=ADVANCED_FACE('',(#17884),#78988,.F.) ;
#86205=ADVANCED_FACE('',(#17885),#13910,.F.) ;
#86206=ADVANCED_FACE('',(#17886),#16245,.F.) ;
#86207=ADVANCED_FACE('',(#17887),#13911,.F.) ;
#86208=ADVANCED_FACE('',(#17888),#13912,.T.) ;
#86209=ADVANCED_FACE('',(#17889),#78989,.T.) ;
#86210=ADVANCED_FACE('',(#17890),#78990,.T.) ;
#86211=ADVANCED_FACE('',(#17891),#78991,.T.) ;
#86212=ADVANCED_FACE('',(#17892),#13913,.F.) ;
#86213=ADVANCED_FACE('',(#17893),#16246,.F.) ;
#86214=ADVANCED_FACE('',(#17894),#78992,.F.) ;
#86215=ADVANCED_FACE('',(#17895),#13914,.F.) ;
#86216=ADVANCED_FACE('',(#17896),#13915,.F.) ;
#86217=ADVANCED_FACE('',(#17897),#13916,.T.) ;
#86218=ADVANCED_FACE('',(#17898),#13917,.T.) ;
#86219=ADVANCED_FACE('',(#17899),#16247,.F.) ;
#86220=ADVANCED_FACE('',(#17900),#13918,.F.) ;
#86221=ADVANCED_FACE('',(#17901),#78993,.F.) ;
#86222=ADVANCED_FACE('',(#17902),#98,.F.) ;
#86223=ADVANCED_FACE('',(#17903),#99,.F.) ;
#86224=ADVANCED_FACE('',(#17904),#13919,.F.) ;
#86225=ADVANCED_FACE('',(#17905),#100,.F.) ;
#86226=ADVANCED_FACE('',(#17906),#101,.F.) ;
#86227=ADVANCED_FACE('',(#17907),#13920,.F.) ;
#86228=ADVANCED_FACE('',(#17908),#16248,.F.) ;
#86229=ADVANCED_FACE('',(#17909),#78994,.T.) ;
#86230=ADVANCED_FACE('',(#17910),#13921,.T.) ;
#86231=ADVANCED_FACE('',(#17911),#102,.T.) ;
#86232=ADVANCED_FACE('',(#17912),#103,.T.) ;
#86233=ADVANCED_FACE('',(#17913),#104,.F.) ;
#86234=ADVANCED_FACE('',(#17914),#105,.F.) ;
#86235=ADVANCED_FACE('',(#17915),#106,.F.) ;
#86236=ADVANCED_FACE('',(#17916),#107,.F.) ;
#86237=ADVANCED_FACE('',(#17917),#16249,.T.) ;
#86238=ADVANCED_FACE('',(#17918),#16250,.T.) ;
#86239=ADVANCED_FACE('',(#17919),#13922,.T.) ;
#86240=ADVANCED_FACE('',(#17920),#13923,.T.) ;
#86241=ADVANCED_FACE('',(#17921),#13924,.T.) ;
#86242=ADVANCED_FACE('',(#17922),#13925,.T.) ;
#86243=ADVANCED_FACE('',(#17923),#16251,.T.) ;
#86244=ADVANCED_FACE('',(#17924),#16252,.T.) ;
#86245=ADVANCED_FACE('',(#17925),#16253,.T.) ;
#86246=ADVANCED_FACE('',(#17926),#16254,.T.) ;
#86247=ADVANCED_FACE('',(#17927),#13926,.T.) ;
#86248=ADVANCED_FACE('',(#17928),#13927,.T.) ;
#86249=ADVANCED_FACE('',(#17929),#13928,.F.) ;
#86250=ADVANCED_FACE('',(#17930),#13929,.T.) ;
#86251=ADVANCED_FACE('',(#17931),#13930,.T.) ;
#86252=ADVANCED_FACE('',(#17932),#78995,.T.) ;
#86253=ADVANCED_FACE('',(#17933),#108,.F.) ;
#86254=ADVANCED_FACE('',(#17934),#109,.F.) ;
#86255=ADVANCED_FACE('',(#17935),#78996,.T.) ;
#86256=ADVANCED_FACE('',(#17936),#13931,.T.) ;
#86257=ADVANCED_FACE('',(#17937),#13932,.F.) ;
#86258=ADVANCED_FACE('',(#17938),#13933,.F.) ;
#86259=ADVANCED_FACE('',(#17939),#13934,.T.) ;
#86260=ADVANCED_FACE('',(#17940),#78997,.F.) ;
#86261=ADVANCED_FACE('',(#17941),#78998,.F.) ;
#86262=ADVANCED_FACE('',(#17942),#13935,.F.) ;
#86263=ADVANCED_FACE('',(#17943),#78999,.F.) ;
#86264=ADVANCED_FACE('',(#17944),#13936,.F.) ;
#86265=ADVANCED_FACE('',(#17945),#79000,.T.) ;
#86266=ADVANCED_FACE('',(#17946),#79001,.F.) ;
#86267=ADVANCED_FACE('',(#17947),#79002,.T.) ;
#86268=ADVANCED_FACE('',(#17948),#79003,.T.) ;
#86269=ADVANCED_FACE('',(#17949),#16255,.T.) ;
#86270=ADVANCED_FACE('',(#17950),#13937,.F.) ;
#86271=ADVANCED_FACE('',(#17951),#16256,.T.) ;
#86272=ADVANCED_FACE('',(#17952),#2419,.F.) ;
#86273=ADVANCED_FACE('',(#17953),#13938,.F.) ;
#86274=ADVANCED_FACE('',(#17954),#13939,.F.) ;
#86275=ADVANCED_FACE('',(#17955),#1020,.F.) ;
#86276=ADVANCED_FACE('',(#17956),#1021,.F.) ;
#86277=ADVANCED_FACE('',(#17957),#1022,.F.) ;
#86278=ADVANCED_FACE('',(#17958),#1023,.T.) ;
#86279=ADVANCED_FACE('',(#17959,#677),#1024,.F.) ;
#86280=ADVANCED_FACE('',(#17960),#1025,.F.) ;
#86281=ADVANCED_FACE('',(#17961),#1026,.F.) ;
#86282=ADVANCED_FACE('',(#17962),#1027,.F.) ;
#86283=ADVANCED_FACE('',(#17963),#1028,.F.) ;
#86284=ADVANCED_FACE('',(#17964),#1029,.F.) ;
#86285=ADVANCED_FACE('',(#17965),#1030,.F.) ;
#86286=ADVANCED_FACE('',(#17966),#1031,.F.) ;
#86287=ADVANCED_FACE('',(#17967),#1032,.F.) ;
#86288=ADVANCED_FACE('',(#17968,#678,#679),#1033,.F.) ;
#86289=ADVANCED_FACE('',(#17969),#1034,.F.) ;
#86290=ADVANCED_FACE('',(#17970),#1035,.F.) ;
#86291=ADVANCED_FACE('',(#17971),#1036,.F.) ;
#86292=ADVANCED_FACE('',(#17972,#680),#1037,.F.) ;
#86293=ADVANCED_FACE('',(#17973,#681),#1038,.F.) ;
#86294=ADVANCED_FACE('',(#17974),#1039,.F.) ;
#86295=ADVANCED_FACE('',(#17975),#1040,.F.) ;
#86296=ADVANCED_FACE('',(#17976),#1041,.F.) ;
#86297=ADVANCED_FACE('',(#17977),#1042,.F.) ;
#86298=ADVANCED_FACE('',(#17978),#1043,.T.) ;
#86299=ADVANCED_FACE('',(#17979),#1044,.F.) ;
#86300=ADVANCED_FACE('',(#17980),#1045,.T.) ;
#86301=ADVANCED_FACE('',(#17981),#1046,.T.) ;
#86302=ADVANCED_FACE('',(#17982),#1047,.T.) ;
#86303=ADVANCED_FACE('',(#17983),#1048,.T.) ;
#86304=ADVANCED_FACE('',(#17984),#1049,.T.) ;
#86305=ADVANCED_FACE('',(#17985),#1050,.F.) ;
#86306=ADVANCED_FACE('',(#17986),#1051,.T.) ;
#86307=ADVANCED_FACE('',(#17987),#1052,.T.) ;
#86308=ADVANCED_FACE('',(#17988),#1053,.F.) ;
#86309=ADVANCED_FACE('',(#17989),#1054,.F.) ;
#86310=ADVANCED_FACE('',(#17990),#1055,.F.) ;
#86311=ADVANCED_FACE('',(#17991),#1056,.F.) ;
#86312=ADVANCED_FACE('',(#17992),#1057,.F.) ;
#86313=ADVANCED_FACE('',(#17993,#682),#1058,.T.) ;
#86314=ADVANCED_FACE('',(#17994),#13940,.T.) ;
#86315=ADVANCED_FACE('',(#17995),#1059,.T.) ;
#86316=ADVANCED_FACE('',(#17996),#13941,.T.) ;
#86317=ADVANCED_FACE('',(#17997),#1060,.T.) ;
#86318=ADVANCED_FACE('',(#17998),#13942,.T.) ;
#86319=ADVANCED_FACE('',(#17999),#1061,.T.) ;
#86320=ADVANCED_FACE('',(#18000),#13943,.T.) ;
#86321=ADVANCED_FACE('',(#18001),#1062,.T.) ;
#86322=ADVANCED_FACE('',(#18002),#1063,.T.) ;
#86323=ADVANCED_FACE('',(#18003),#1064,.T.) ;
#86324=ADVANCED_FACE('',(#18004),#1065,.F.) ;
#86325=ADVANCED_FACE('',(#18005),#1066,.F.) ;
#86326=ADVANCED_FACE('',(#18006),#1067,.T.) ;
#86327=ADVANCED_FACE('',(#18007),#1068,.F.) ;
#86328=ADVANCED_FACE('',(#18008),#1069,.F.) ;
#86329=ADVANCED_FACE('',(#18009),#1070,.F.) ;
#86330=ADVANCED_FACE('',(#18010),#1071,.F.) ;
#86331=ADVANCED_FACE('',(#18011,#683),#1072,.T.) ;
#86332=ADVANCED_FACE('',(#18012),#13944,.T.) ;
#86333=ADVANCED_FACE('',(#18013),#1073,.T.) ;
#86334=ADVANCED_FACE('',(#18014),#13945,.T.) ;
#86335=ADVANCED_FACE('',(#18015),#1074,.T.) ;
#86336=ADVANCED_FACE('',(#18016),#13946,.T.) ;
#86337=ADVANCED_FACE('',(#18017),#1075,.T.) ;
#86338=ADVANCED_FACE('',(#18018),#13947,.T.) ;
#86339=ADVANCED_FACE('',(#18019),#1076,.T.) ;
#86340=ADVANCED_FACE('',(#18020),#1077,.T.) ;
#86341=ADVANCED_FACE('',(#18021),#1078,.F.) ;
#86342=ADVANCED_FACE('',(#18022),#1079,.F.) ;
#86343=ADVANCED_FACE('',(#18023),#1080,.F.) ;
#86344=ADVANCED_FACE('',(#18024),#1081,.F.) ;
#86345=ADVANCED_FACE('',(#18025),#1082,.T.) ;
#86346=ADVANCED_FACE('',(#18026),#13948,.T.) ;
#86347=ADVANCED_FACE('',(#18027),#110,.T.) ;
#86348=ADVANCED_FACE('',(#18028),#13949,.F.) ;
#86349=ADVANCED_FACE('',(#18029),#111,.F.) ;
#86350=ADVANCED_FACE('',(#18030),#13950,.F.) ;
#86351=ADVANCED_FACE('',(#18031),#13951,.F.) ;
#86352=ADVANCED_FACE('',(#18032),#13952,.T.) ;
#86353=ADVANCED_FACE('',(#18033),#13953,.T.) ;
#86354=ADVANCED_FACE('',(#18034),#13954,.T.) ;
#86355=ADVANCED_FACE('',(#18035),#13955,.F.) ;
#86356=ADVANCED_FACE('',(#18036),#16257,.F.) ;
#86357=ADVANCED_FACE('',(#18037),#112,.T.) ;
#86358=ADVANCED_FACE('',(#18038),#113,.T.) ;
#86359=ADVANCED_FACE('',(#18039),#114,.F.) ;
#86360=ADVANCED_FACE('',(#18040),#13956,.F.) ;
#86361=ADVANCED_FACE('',(#18041),#13957,.F.) ;
#86362=ADVANCED_FACE('',(#18042),#13958,.T.) ;
#86363=ADVANCED_FACE('',(#18043),#13959,.T.) ;
#86364=ADVANCED_FACE('',(#18044),#13960,.F.) ;
#86365=ADVANCED_FACE('',(#18045),#13961,.F.) ;
#86366=ADVANCED_FACE('',(#18046),#16258,.F.) ;
#86367=ADVANCED_FACE('',(#18047),#115,.T.) ;
#86368=ADVANCED_FACE('',(#18048),#16259,.F.) ;
#86369=ADVANCED_FACE('',(#18049),#13962,.F.) ;
#86370=ADVANCED_FACE('',(#18050),#13963,.F.) ;
#86371=ADVANCED_FACE('',(#18051),#13964,.F.) ;
#86372=ADVANCED_FACE('',(#18052),#13965,.F.) ;
#86373=ADVANCED_FACE('',(#18053),#116,.F.) ;
#86374=ADVANCED_FACE('',(#18054),#16260,.F.) ;
#86375=ADVANCED_FACE('',(#18055),#13966,.T.) ;
#86376=ADVANCED_FACE('',(#18056),#13967,.F.) ;
#86377=ADVANCED_FACE('',(#18057),#117,.F.) ;
#86378=ADVANCED_FACE('',(#18058),#13968,.F.) ;
#86379=ADVANCED_FACE('',(#18059),#13969,.T.) ;
#86380=ADVANCED_FACE('',(#18060),#13970,.T.) ;
#86381=ADVANCED_FACE('',(#18061),#13971,.F.) ;
#86382=ADVANCED_FACE('',(#18062),#13972,.T.) ;
#86383=ADVANCED_FACE('',(#18063),#13973,.T.) ;
#86384=ADVANCED_FACE('',(#18064),#13974,.F.) ;
#86385=ADVANCED_FACE('',(#18065),#79004,.T.) ;
#86386=ADVANCED_FACE('',(#18066),#13975,.T.) ;
#86387=ADVANCED_FACE('',(#18067),#13976,.T.) ;
#86388=ADVANCED_FACE('',(#18068),#13977,.T.) ;
#86389=ADVANCED_FACE('',(#18069),#13978,.T.) ;
#86390=ADVANCED_FACE('',(#18070),#16261,.T.) ;
#86391=ADVANCED_FACE('',(#18071),#13979,.T.) ;
#86392=ADVANCED_FACE('',(#18072),#13980,.T.) ;
#86393=ADVANCED_FACE('',(#18073),#16262,.T.) ;
#86394=ADVANCED_FACE('',(#18074),#16263,.T.) ;
#86395=ADVANCED_FACE('',(#18075),#13981,.T.) ;
#86396=ADVANCED_FACE('',(#18076),#13982,.T.) ;
#86397=ADVANCED_FACE('',(#18077),#16264,.T.) ;
#86398=ADVANCED_FACE('',(#18078),#13983,.T.) ;
#86399=ADVANCED_FACE('',(#18079),#79005,.T.) ;
#86400=ADVANCED_FACE('',(#18080),#79006,.T.) ;
#86401=ADVANCED_FACE('',(#18081),#13984,.T.) ;
#86402=ADVANCED_FACE('',(#18082),#13985,.F.) ;
#86403=ADVANCED_FACE('',(#18083),#13986,.F.) ;
#86404=ADVANCED_FACE('',(#18084),#13987,.F.) ;
#86405=ADVANCED_FACE('',(#18085),#13988,.T.) ;
#86406=ADVANCED_FACE('',(#18086),#13989,.T.) ;
#86407=ADVANCED_FACE('',(#18087),#79007,.T.) ;
#86408=ADVANCED_FACE('',(#18088),#16265,.F.) ;
#86409=ADVANCED_FACE('',(#18089),#16266,.F.) ;
#86410=ADVANCED_FACE('',(#18090),#79008,.T.) ;
#86411=ADVANCED_FACE('',(#18091),#13990,.F.) ;
#86412=ADVANCED_FACE('',(#18092),#13991,.F.) ;
#86413=ADVANCED_FACE('',(#18093),#13992,.F.) ;
#86414=ADVANCED_FACE('',(#18094),#13993,.F.) ;
#86415=ADVANCED_FACE('',(#18095),#16267,.F.) ;
#86416=ADVANCED_FACE('',(#18096),#16268,.F.) ;
#86417=ADVANCED_FACE('',(#18097),#13994,.F.) ;
#86418=ADVANCED_FACE('',(#18098),#13995,.T.) ;
#86419=ADVANCED_FACE('',(#18099),#79009,.T.) ;
#86420=ADVANCED_FACE('',(#18100),#79010,.T.) ;
#86421=ADVANCED_FACE('',(#18101),#13996,.T.) ;
#86422=ADVANCED_FACE('',(#18102),#13997,.F.) ;
#86423=ADVANCED_FACE('',(#18103),#13998,.F.) ;
#86424=ADVANCED_FACE('',(#18104),#13999,.F.) ;
#86425=ADVANCED_FACE('',(#18105),#14000,.T.) ;
#86426=ADVANCED_FACE('',(#18106),#14001,.T.) ;
#86427=ADVANCED_FACE('',(#18107),#79011,.T.) ;
#86428=ADVANCED_FACE('',(#18108),#16269,.F.) ;
#86429=ADVANCED_FACE('',(#18109),#16270,.F.) ;
#86430=ADVANCED_FACE('',(#18110),#79012,.T.) ;
#86431=ADVANCED_FACE('',(#18111),#14002,.F.) ;
#86432=ADVANCED_FACE('',(#18112),#14003,.F.) ;
#86433=ADVANCED_FACE('',(#18113),#14004,.F.) ;
#86434=ADVANCED_FACE('',(#18114),#14005,.F.) ;
#86435=ADVANCED_FACE('',(#18115),#16271,.F.) ;
#86436=ADVANCED_FACE('',(#18116),#16272,.F.) ;
#86437=ADVANCED_FACE('',(#18117),#14006,.F.) ;
#86438=ADVANCED_FACE('',(#18118),#79013,.F.) ;
#86439=ADVANCED_FACE('',(#18119),#14007,.F.) ;
#86440=ADVANCED_FACE('',(#18120),#16273,.F.) ;
#86441=ADVANCED_FACE('',(#18121),#14008,.F.) ;
#86442=ADVANCED_FACE('',(#18122),#14009,.T.) ;
#86443=ADVANCED_FACE('',(#18123),#79014,.T.) ;
#86444=ADVANCED_FACE('',(#18124),#79015,.T.) ;
#86445=ADVANCED_FACE('',(#18125),#14010,.T.) ;
#86446=ADVANCED_FACE('',(#18126),#79016,.T.) ;
#86447=ADVANCED_FACE('',(#18127),#14011,.F.) ;
#86448=ADVANCED_FACE('',(#18128),#14012,.F.) ;
#86449=ADVANCED_FACE('',(#18129),#16274,.F.) ;
#86450=ADVANCED_FACE('',(#18130),#79017,.F.) ;
#86451=ADVANCED_FACE('',(#18131),#14013,.F.) ;
#86452=ADVANCED_FACE('',(#18132),#14014,.T.) ;
#86453=ADVANCED_FACE('',(#18133),#14015,.T.) ;
#86454=ADVANCED_FACE('',(#18134),#14016,.T.) ;
#86455=ADVANCED_FACE('',(#18135),#14017,.T.) ;
#86456=ADVANCED_FACE('',(#18136),#14018,.T.) ;
#86457=ADVANCED_FACE('',(#18137),#14019,.F.) ;
#86458=ADVANCED_FACE('',(#18138),#14020,.F.) ;
#86459=ADVANCED_FACE('',(#18139),#14021,.T.) ;
#86460=ADVANCED_FACE('',(#18140),#14022,.T.) ;
#86461=ADVANCED_FACE('',(#18141),#14023,.T.) ;
#86462=ADVANCED_FACE('',(#18142),#14024,.T.) ;
#86463=ADVANCED_FACE('',(#18143),#14025,.F.) ;
#86464=ADVANCED_FACE('',(#18144),#14026,.F.) ;
#86465=ADVANCED_FACE('',(#18145),#14027,.T.) ;
#86466=ADVANCED_FACE('',(#18146),#14028,.T.) ;
#86467=ADVANCED_FACE('',(#18147),#14029,.F.) ;
#86468=ADVANCED_FACE('',(#18148),#16275,.F.) ;
#86469=ADVANCED_FACE('',(#18149),#14030,.F.) ;
#86470=ADVANCED_FACE('',(#18150),#79018,.F.) ;
#86471=ADVANCED_FACE('',(#18151),#118,.F.) ;
#86472=ADVANCED_FACE('',(#18152),#119,.F.) ;
#86473=ADVANCED_FACE('',(#18153),#14031,.F.) ;
#86474=ADVANCED_FACE('',(#18154),#14032,.F.) ;
#86475=ADVANCED_FACE('',(#18155),#120,.F.) ;
#86476=ADVANCED_FACE('',(#18156),#121,.F.) ;
#86477=ADVANCED_FACE('',(#18157),#14033,.F.) ;
#86478=ADVANCED_FACE('',(#18158),#16276,.F.) ;
#86479=ADVANCED_FACE('',(#18159),#79019,.T.) ;
#86480=ADVANCED_FACE('',(#18160),#14034,.T.) ;
#86481=ADVANCED_FACE('',(#18161),#122,.T.) ;
#86482=ADVANCED_FACE('',(#18162),#14035,.T.) ;
#86483=ADVANCED_FACE('',(#18163),#123,.T.) ;
#86484=ADVANCED_FACE('',(#18164),#124,.F.) ;
#86485=ADVANCED_FACE('',(#18165),#125,.F.) ;
#86486=ADVANCED_FACE('',(#18166),#126,.F.) ;
#86487=ADVANCED_FACE('',(#18167),#127,.F.) ;
#91083=CLOSED_SHELL('',(#85367,#85368,#85369,#85370,#85371,#85372,#85373,
#85374,#85375,#85376,#85377,#85378,#85379,#85380,#85381,#85382,#85383,#85384,
#85385,#85386,#85387,#85388,#85389,#85390,#85391,#85392,#85393,#85394,#85395,
#85396,#85397,#85398,#85399,#85400,#85401,#85402,#85403,#85404,#85405,#85406,
#85407,#85408,#85409,#85410,#85411,#85412,#85413,#85414,#85415,#85416,#85417,
#85418,#85419,#85420,#85421,#85422,#85423,#85424,#85425,#85426,#85427,#85428,
#85429,#85430,#85431,#85432,#85433,#85434,#85435,#85436,#85437,#85438,#85439,
#85440,#85441,#85442,#85443,#85444,#85445,#85446,#85447,#85448,#85449,#85450,
#85451,#85452,#85453,#85454,#85455,#85456,#85457,#85458,#85459,#85460,#85461,
#85462,#85463,#85464,#85465,#85466,#85467,#85468,#85469,#85470,#85471,#85472,
#85473,#85474,#85475,#85476,#85477,#85478,#85479,#85480,#85481,#85482,#85483,
#85484,#85485,#85486,#85487,#85488,#85489,#85490,#85491,#85492,#85493,#85494,
#85495,#85496,#85497,#85498,#85499,#85500,#85501,#85502,#85503,#85504,#85505,
#85506,#85507,#85508,#85509,#85510,#85511,#85512,#85513,#85514,#85515,#85516,
#85517,#85518,#85519,#85520,#85521,#85522,#85523,#85524,#85525,#85526,#85527,
#85528,#85529,#85530,#85531,#85532,#85533,#85534,#85535,#85536,#85537,#85538,
#85539,#85540,#85541,#85542,#85543,#85544,#85545,#85546,#85547,#85548,#85549,
#85550,#85551,#85552,#85553,#85554,#85555,#85556,#85557,#85558,#85559,#85560,
#85561,#85562,#85563,#85564,#85565,#85566,#85567,#85568,#85569,#85570,#85571,
#85572,#85573,#85574,#85575,#85576,#85577,#85578,#85579,#85580,#85581,#85582,
#85583,#85584,#85585,#85586,#85587,#85588,#85589,#85590,#85591,#85592,#85593,
#85594,#85595,#85596,#85597,#85598,#85599,#85600,#85601,#85602,#85603,#85604,
#85605,#85606,#85607,#85608,#85609,#85610,#85611,#85612,#85613,#85614,#85615,
#85616,#85617,#85618,#85619,#85620,#85621,#85622,#85623,#85624,#85625,#85626,
#85627,#85628,#85629,#85630,#85631,#85632,#85633,#85634,#85635,#85636,#85637,
#85638,#85639,#85640,#85641,#85642,#85643,#85644,#85645,#85646,#85647,#85648,
#85649,#85650,#85651,#85652,#85653,#85654,#85655,#85656,#85657,#85658,#85659,
#85660,#85661,#85662,#85663,#85664,#85665,#85666,#85667,#85668,#85669,#85670,
#85671,#85672,#85673,#85674,#85675,#85676,#85677,#85678,#85679,#85680,#85681,
#85682,#85683,#85684,#85685,#85686,#85687,#85688,#85689,#85690,#85691,#85692,
#85693,#85694,#85695,#85696,#85697,#85698,#85699,#85700,#85701,#85702,#85703,
#85704,#85705,#85706,#85707,#85708,#85709,#85710,#85711,#85712,#85713,#85714,
#85715,#85716,#85717,#85718,#85719,#85720,#85721,#85722,#85723,#85724,#85725,
#85726,#85727,#85728,#85729,#85730,#85731,#85732,#85733,#85734,#85735,#85736,
#85737,#85738,#85739,#85740,#85741,#85742,#85743,#85744,#85745,#85746,#85747,
#85748,#85749,#85750,#85751,#85752,#85753,#85754,#85755,#85756,#85757,#85758,
#85759,#85760,#85761,#85762,#85763,#85764,#85765,#85766,#85767,#85768,#85769,
#85770,#85771,#85772,#85773,#85774,#85775,#85776,#85777,#85778,#85779,#85780,
#85781,#85782,#85783,#85784,#85785,#85786,#85787,#85788,#85789,#85790,#85791,
#85792,#85793,#85794,#85795,#85796,#85797,#85798,#85799,#85800,#85801,#85802,
#85803,#85804,#85805,#85806,#85807,#85808,#85809,#85810,#85811,#85812,#85813,
#85814)) ;
#91084=CLOSED_SHELL('',(#85815,#85816,#85817,#85818,#85819,#85820,#85821,
#85822,#85823,#85824,#85825,#85826,#85827,#85828,#85829,#85830,#85831,#85832,
#85833,#85834,#85835,#85836,#85837,#85838,#85839,#85840,#85841,#85842,#85843,
#85844,#85845,#85846,#85847,#85848,#85849,#85850,#85851,#85852,#85853,#85854,
#85855,#85856,#85857,#85858,#85859,#85860,#85861,#85862,#85863,#85864,#85865,
#85866,#85867,#85868,#85869,#85870,#85871,#85872,#85873,#85874,#85875,#85876,
#85877,#85878,#85879,#85880,#85881,#85882,#85883,#85884,#85885,#85886,#85887,
#85888,#85889,#85890,#85891,#85892,#85893,#85894,#85895,#85896,#85897,#85898,
#85899,#85900,#85901,#85902,#85903,#85904,#85905,#85906,#85907,#85908,#85909,
#85910,#85911,#85912,#85913,#85914,#85915,#85916,#85917,#85918,#85919,#85920,
#85921,#85922,#85923,#85924,#85925,#85926,#85927,#85928,#85929,#85930,#85931,
#85932,#85933,#85934,#85935,#85936,#85937,#85938,#85939,#85940,#85941,#85942,
#85943,#85944,#85945,#85946,#85947,#85948,#85949,#85950,#85951,#85952,#85953,
#85954,#85955,#85956,#85957,#85958,#85959,#85960,#85961,#85962,#85963,#85964,
#85965,#85966,#85967,#85968,#85969,#85970,#85971,#85972,#85973,#85974,#85975,
#85976,#85977,#85978,#85979,#85980,#85981,#85982,#85983,#85984,#85985,#85986,
#85987,#85988,#85989,#85990,#85991,#85992,#85993,#85994,#85995,#85996,#85997,
#85998,#85999,#86000,#86001,#86002,#86003,#86004,#86005,#86006,#86007,#86008,
#86009,#86010,#86011,#86012,#86013,#86014,#86015,#86016,#86017,#86018,#86019,
#86020,#86021,#86022,#86023,#86024,#86025,#86026,#86027,#86028,#86029,#86030,
#86031,#86032,#86033,#86034,#86035,#86036,#86037,#86038,#86039,#86040,#86041,
#86042,#86043,#86044,#86045,#86046,#86047,#86048,#86049,#86050,#86051,#86052,
#86053,#86054,#86055,#86056,#86057,#86058,#86059,#86060,#86061,#86062,#86063,
#86064,#86065,#86066,#86067,#86068,#86069,#86070,#86071,#86072,#86073,#86074,
#86075,#86076,#86077,#86078,#86079,#86080,#86081,#86082,#86083,#86084,#86085,
#86086,#86087,#86088,#86089,#86090,#86091,#86092,#86093,#86094,#86095,#86096,
#86097,#86098,#86099,#86100,#86101,#86102,#86103,#86104,#86105,#86106,#86107,
#86108,#86109,#86110,#86111,#86112,#86113,#86114,#86115,#86116,#86117,#86118,
#86119,#86120,#86121,#86122,#86123,#86124,#86125,#86126,#86127,#86128,#86129,
#86130,#86131,#86132,#86133,#86134,#86135,#86136,#86137,#86138,#86139,#86140,
#86141,#86142,#86143,#86144,#86145,#86146,#86147,#86148,#86149,#86150,#86151,
#86152,#86153,#86154,#86155,#86156,#86157,#86158,#86159,#86160,#86161,#86162,
#86163,#86164,#86165,#86166,#86167,#86168,#86169,#86170,#86171,#86172,#86173,
#86174,#86175,#86176,#86177,#86178,#86179,#86180,#86181,#86182,#86183,#86184,
#86185,#86186,#86187,#86188,#86189,#86190,#86191,#86192,#86193,#86194,#86195,
#86196,#86197,#86198,#86199,#86200,#86201,#86202,#86203,#86204,#86205,#86206,
#86207,#86208,#86209,#86210,#86211,#86212,#86213,#86214,#86215,#86216,#86217,
#86218,#86219,#86220,#86221,#86222,#86223,#86224,#86225,#86226,#86227,#86228,
#86229,#86230,#86231,#86232,#86233,#86234,#86235,#86236,#86237,#86238,#86239,
#86240,#86241,#86242,#86243,#86244,#86245,#86246,#86247,#86248,#86249,#86250,
#86251,#86252,#86253,#86254,#86255,#86256,#86257,#86258,#86259,#86260,#86261,
#86262)) ;
#91085=CLOSED_SHELL('',(#86263,#86264,#86265,#86266,#86267,#86268,#86269,
#86270,#86271,#86272,#86273,#86274,#86275,#86276,#86277,#86278,#86279,#86280,
#86281,#86282,#86283,#86284,#86285,#86286,#86287,#86288,#86289,#86290,#86291,
#86292,#86293,#86294,#86295,#86296,#86297,#86298,#86299,#86300,#86301,#86302,
#86303,#86304,#86305,#86306,#86307,#86308,#86309,#86310,#86311,#86312,#86313,
#86314,#86315,#86316,#86317,#86318,#86319,#86320,#86321,#86322,#86323,#86324,
#86325,#86326,#86327,#86328,#86329,#86330,#86331,#86332,#86333,#86334,#86335,
#86336,#86337,#86338,#86339,#86340,#86341,#86342,#86343,#86344,#86345,#86346,
#86347,#86348,#86349,#86350,#86351,#86352,#86353,#86354,#86355,#86356,#86357,
#86358,#86359,#86360,#86361,#86362,#86363,#86364,#86365,#86366,#86367,#86368,
#86369,#86370,#86371,#86372,#86373,#86374,#86375,#86376,#86377,#86378,#86379,
#86380,#86381,#86382,#86383,#86384,#86385,#86386,#86387,#86388,#86389,#86390,
#86391,#86392,#86393,#86394,#86395,#86396,#86397,#86398,#86399,#86400,#86401,
#86402,#86403,#86404,#86405,#86406,#86407,#86408,#86409,#86410,#86411,#86412,
#86413,#86414,#86415,#86416,#86417,#86418,#86419,#86420,#86421,#86422,#86423,
#86424,#86425,#86426,#86427,#86428,#86429,#86430,#86431,#86432,#86433,#86434,
#86435,#86436,#86437,#86438,#86439,#86440,#86441,#86442,#86443,#86444,#86445,
#86446,#86447,#86448,#86449,#86450,#86451,#86452,#86453,#86454,#86455,#86456,
#86457,#86458,#86459,#86460,#86461,#86462,#86463,#86464,#86465,#86466,#86467,
#86468,#86469,#86470,#86471,#86472,#86473,#86474,#86475,#86476,#86477,#86478,
#86479,#86480,#86481,#86482,#86483,#86484,#86485,#86486,#86487)) ;
#91123=AXIS2_PLACEMENT_3D('',#132551,#103082,#103083) ;
#91124=AXIS2_PLACEMENT_3D('',#132552,#103084,#103085) ;
#91125=AXIS2_PLACEMENT_3D('',#132555,#103086,#103087) ;
#91126=AXIS2_PLACEMENT_3D('',#132557,#103088,#103089) ;
#91127=AXIS2_PLACEMENT_3D('',#132559,#103090,#103091) ;
#91128=AXIS2_PLACEMENT_3D('',#132560,#103092,#103093) ;
#91129=AXIS2_PLACEMENT_3D('',#132561,#103094,#103095) ;
#91130=AXIS2_PLACEMENT_3D('',#132563,#103096,#103097) ;
#91131=AXIS2_PLACEMENT_3D('',#132565,#103098,#103099) ;
#91132=AXIS2_PLACEMENT_3D('',#132567,#103100,#103101) ;
#91133=AXIS2_PLACEMENT_3D('',#132568,#103102,#103103) ;
#91134=AXIS2_PLACEMENT_3D('',#132569,#103104,#103105) ;
#91135=AXIS2_PLACEMENT_3D('',#132571,#103106,#103107) ;
#91136=AXIS2_PLACEMENT_3D('',#132573,#103108,#103109) ;
#91137=AXIS2_PLACEMENT_3D('',#132574,#103110,#103111) ;
#91138=AXIS2_PLACEMENT_3D('',#132575,#103112,#103113) ;
#91139=AXIS2_PLACEMENT_3D('',#132577,#103114,#103115) ;
#91140=AXIS2_PLACEMENT_3D('',#132579,#103116,#103117) ;
#91141=AXIS2_PLACEMENT_3D('',#132581,#103118,#103119) ;
#91142=AXIS2_PLACEMENT_3D('',#132582,#103120,#103121) ;
#91143=AXIS2_PLACEMENT_3D('',#132583,#103122,#103123) ;
#91144=AXIS2_PLACEMENT_3D('',#132586,#103124,#103125) ;
#91145=AXIS2_PLACEMENT_3D('',#132588,#103126,#103127) ;
#91146=AXIS2_PLACEMENT_3D('',#132590,#103128,#103129) ;
#91147=AXIS2_PLACEMENT_3D('',#132591,#103130,#103131) ;
#91148=AXIS2_PLACEMENT_3D('',#132592,#103132,#103133) ;
#91149=AXIS2_PLACEMENT_3D('',#132595,#103134,#103135) ;
#91150=AXIS2_PLACEMENT_3D('',#132597,#103136,#103137) ;
#91151=AXIS2_PLACEMENT_3D('',#132598,#103138,#103139) ;
#91152=AXIS2_PLACEMENT_3D('',#132599,#103140,#103141) ;
#91153=AXIS2_PLACEMENT_3D('',#132603,#103143,#103144) ;
#91154=AXIS2_PLACEMENT_3D('',#132605,#103146,#103147) ;
#91155=AXIS2_PLACEMENT_3D('',#132608,#103148,#103149) ;
#91156=AXIS2_PLACEMENT_3D('',#132610,#103150,#103151) ;
#91157=AXIS2_PLACEMENT_3D('',#132611,#103152,#103153) ;
#91158=AXIS2_PLACEMENT_3D('',#132612,#103154,#103155) ;
#91159=AXIS2_PLACEMENT_3D('',#132614,#103156,#103157) ;
#91160=AXIS2_PLACEMENT_3D('',#132616,#103159,#103160) ;
#91161=AXIS2_PLACEMENT_3D('',#132618,#103162,#103163) ;
#91162=AXIS2_PLACEMENT_3D('',#132621,#103164,#103165) ;
#91163=AXIS2_PLACEMENT_3D('',#132647,#103167,#103168) ;
#91164=AXIS2_PLACEMENT_3D('',#132694,#103170,#103171) ;
#91165=AXIS2_PLACEMENT_3D('',#132720,#103173,#103174) ;
#91166=AXIS2_PLACEMENT_3D('',#132766,#103176,#103177) ;
#91167=AXIS2_PLACEMENT_3D('',#132768,#103179,#103180) ;
#91168=AXIS2_PLACEMENT_3D('',#132771,#103181,#103182) ;
#91169=AXIS2_PLACEMENT_3D('',#132773,#103183,#103184) ;
#91170=AXIS2_PLACEMENT_3D('',#132775,#103185,#103186) ;
#91171=AXIS2_PLACEMENT_3D('',#132776,#103187,#103188) ;
#91172=AXIS2_PLACEMENT_3D('',#132777,#103189,#103190) ;
#91173=AXIS2_PLACEMENT_3D('',#132780,#103191,#103192) ;
#91174=AXIS2_PLACEMENT_3D('',#132784,#103194,#103195) ;
#91175=AXIS2_PLACEMENT_3D('',#132786,#103197,#103198) ;
#91176=AXIS2_PLACEMENT_3D('',#132788,#103199,#103200) ;
#91177=AXIS2_PLACEMENT_3D('',#132790,#103201,#103202) ;
#91178=AXIS2_PLACEMENT_3D('',#132792,#103203,#103204) ;
#91179=AXIS2_PLACEMENT_3D('',#132793,#103205,#103206) ;
#91180=AXIS2_PLACEMENT_3D('',#132794,#103207,#103208) ;
#91181=AXIS2_PLACEMENT_3D('',#132796,#103209,#103210) ;
#91182=AXIS2_PLACEMENT_3D('',#132798,#103211,#103212) ;
#91183=AXIS2_PLACEMENT_3D('',#132799,#103213,#103214) ;
#91184=AXIS2_PLACEMENT_3D('',#132800,#103215,#103216) ;
#91185=AXIS2_PLACEMENT_3D('',#132802,#103217,#103218) ;
#91186=AXIS2_PLACEMENT_3D('',#132804,#103219,#103220) ;
#91187=AXIS2_PLACEMENT_3D('',#132806,#103221,#103222) ;
#91188=AXIS2_PLACEMENT_3D('',#132807,#103223,#103224) ;
#91189=AXIS2_PLACEMENT_3D('',#132808,#103225,#103226) ;
#91190=AXIS2_PLACEMENT_3D('',#132811,#103227,#103228) ;
#91191=AXIS2_PLACEMENT_3D('',#132813,#103229,#103230) ;
#91192=AXIS2_PLACEMENT_3D('',#132815,#103231,#103232) ;
#91193=AXIS2_PLACEMENT_3D('',#132816,#103233,#103234) ;
#91194=AXIS2_PLACEMENT_3D('',#132817,#103235,#103236) ;
#91195=AXIS2_PLACEMENT_3D('',#132820,#103237,#103238) ;
#91196=AXIS2_PLACEMENT_3D('',#132822,#103239,#103240) ;
#91197=AXIS2_PLACEMENT_3D('',#132823,#103241,#103242) ;
#91198=AXIS2_PLACEMENT_3D('',#132824,#103243,#103244) ;
#91199=AXIS2_PLACEMENT_3D('',#132828,#103246,#103247) ;
#91200=AXIS2_PLACEMENT_3D('',#132830,#103249,#103250) ;
#91201=AXIS2_PLACEMENT_3D('',#132833,#103251,#103252) ;
#91202=AXIS2_PLACEMENT_3D('',#132835,#103253,#103254) ;
#91203=AXIS2_PLACEMENT_3D('',#132836,#103255,#103256) ;
#91204=AXIS2_PLACEMENT_3D('',#132837,#103257,#103258) ;
#91205=AXIS2_PLACEMENT_3D('',#132839,#103259,#103260) ;
#91206=AXIS2_PLACEMENT_3D('',#132841,#103262,#103263) ;
#91207=AXIS2_PLACEMENT_3D('',#132843,#103265,#103266) ;
#91208=AXIS2_PLACEMENT_3D('',#132846,#103267,#103268) ;
#91209=AXIS2_PLACEMENT_3D('',#132872,#103270,#103271) ;
#91210=AXIS2_PLACEMENT_3D('',#132919,#103273,#103274) ;
#91211=AXIS2_PLACEMENT_3D('',#132945,#103276,#103277) ;
#91212=AXIS2_PLACEMENT_3D('',#132991,#103279,#103280) ;
#91213=AXIS2_PLACEMENT_3D('',#132993,#103282,#103283) ;
#91214=AXIS2_PLACEMENT_3D('',#133004,#103288,#103289) ;
#91215=AXIS2_PLACEMENT_3D('',#133022,#103293,#103294) ;
#91216=AXIS2_PLACEMENT_3D('',#133024,#103296,#103297) ;
#91217=AXIS2_PLACEMENT_3D('',#133033,#103302,#103303) ;
#91218=AXIS2_PLACEMENT_3D('',#133042,#103308,#103309) ;
#91219=AXIS2_PLACEMENT_3D('',#133051,#103314,#103315) ;
#91220=AXIS2_PLACEMENT_3D('',#133055,#103317,#103318) ;
#91221=AXIS2_PLACEMENT_3D('',#133056,#103319,#103320) ;
#91222=AXIS2_PLACEMENT_3D('',#133057,#103321,#103322) ;
#91223=AXIS2_PLACEMENT_3D('',#133058,#103323,#103324) ;
#91224=AXIS2_PLACEMENT_3D('',#133059,#103325,#103326) ;
#91225=AXIS2_PLACEMENT_3D('',#133060,#103327,#103328) ;
#91226=AXIS2_PLACEMENT_3D('',#133061,#103329,#103330) ;
#91227=AXIS2_PLACEMENT_3D('',#133062,#103331,#103332) ;
#91228=AXIS2_PLACEMENT_3D('',#133063,#103333,#103334) ;
#91229=AXIS2_PLACEMENT_3D('',#133065,#103335,#103336) ;
#91230=AXIS2_PLACEMENT_3D('',#133069,#103338,#103339) ;
#91231=AXIS2_PLACEMENT_3D('',#133072,#103341,#103342) ;
#91232=AXIS2_PLACEMENT_3D('',#133073,#103343,#103344) ;
#91233=AXIS2_PLACEMENT_3D('',#133076,#103345,#103346) ;
#91234=AXIS2_PLACEMENT_3D('',#133080,#103348,#103349) ;
#91235=AXIS2_PLACEMENT_3D('',#133082,#103351,#103352) ;
#91236=AXIS2_PLACEMENT_3D('',#133091,#103357,#103358) ;
#91237=AXIS2_PLACEMENT_3D('',#133098,#103363,#103364) ;
#91238=AXIS2_PLACEMENT_3D('',#133100,#103366,#103367) ;
#91239=AXIS2_PLACEMENT_3D('',#133109,#103372,#103373) ;
#91240=AXIS2_PLACEMENT_3D('',#133111,#103374,#103375) ;
#91241=AXIS2_PLACEMENT_3D('',#133113,#103376,#103377) ;
#91242=AXIS2_PLACEMENT_3D('',#133117,#103379,#103380) ;
#91243=AXIS2_PLACEMENT_3D('',#133119,#103381,#103382) ;
#91244=AXIS2_PLACEMENT_3D('',#133121,#103383,#103384) ;
#91245=AXIS2_PLACEMENT_3D('',#133130,#103389,#103390) ;
#91246=AXIS2_PLACEMENT_3D('',#133137,#103395,#103396) ;
#91247=AXIS2_PLACEMENT_3D('',#133139,#103398,#103399) ;
#91248=AXIS2_PLACEMENT_3D('',#133147,#103404,#103405) ;
#91249=AXIS2_PLACEMENT_3D('',#133154,#103408,#103409) ;
#91250=AXIS2_PLACEMENT_3D('',#133158,#103411,#103412) ;
#91251=AXIS2_PLACEMENT_3D('',#133162,#103414,#103415) ;
#91252=AXIS2_PLACEMENT_3D('',#133166,#103417,#103418) ;
#91253=AXIS2_PLACEMENT_3D('',#133172,#103422,#103423) ;
#91254=AXIS2_PLACEMENT_3D('',#133178,#103427,#103428) ;
#91255=AXIS2_PLACEMENT_3D('',#133185,#103433,#103434) ;
#91256=AXIS2_PLACEMENT_3D('',#133196,#103439,#103440) ;
#91257=AXIS2_PLACEMENT_3D('',#133200,#103442,#103443) ;
#91258=AXIS2_PLACEMENT_3D('',#133204,#103445,#103446) ;
#91259=AXIS2_PLACEMENT_3D('',#133208,#103448,#103449) ;
#91260=AXIS2_PLACEMENT_3D('',#133212,#103451,#103452) ;
#91261=AXIS2_PLACEMENT_3D('',#133216,#103454,#103455) ;
#91262=AXIS2_PLACEMENT_3D('',#133220,#103457,#103458) ;
#91263=AXIS2_PLACEMENT_3D('',#133224,#103460,#103461) ;
#91264=AXIS2_PLACEMENT_3D('',#133226,#103463,#103464) ;
#91265=AXIS2_PLACEMENT_3D('',#133235,#103469,#103470) ;
#91266=AXIS2_PLACEMENT_3D('',#133241,#103474,#103475) ;
#91267=AXIS2_PLACEMENT_3D('',#133247,#103479,#103480) ;
#91268=AXIS2_PLACEMENT_3D('',#133328,#103493,#103494) ;
#91269=AXIS2_PLACEMENT_3D('',#133339,#103499,#103500) ;
#91270=AXIS2_PLACEMENT_3D('',#133343,#103502,#103503) ;
#91271=AXIS2_PLACEMENT_3D('',#133347,#103505,#103506) ;
#91272=AXIS2_PLACEMENT_3D('',#133351,#103508,#103509) ;
#91273=AXIS2_PLACEMENT_3D('',#133355,#103511,#103512) ;
#91274=AXIS2_PLACEMENT_3D('',#133359,#103514,#103515) ;
#91275=AXIS2_PLACEMENT_3D('',#133363,#103517,#103518) ;
#91276=AXIS2_PLACEMENT_3D('',#133367,#103520,#103521) ;
#91277=AXIS2_PLACEMENT_3D('',#133369,#103523,#103524) ;
#91278=AXIS2_PLACEMENT_3D('',#133378,#103529,#103530) ;
#91279=AXIS2_PLACEMENT_3D('',#133557,#103537,#103538) ;
#91280=AXIS2_PLACEMENT_3D('',#133564,#103541,#103542) ;
#91281=AXIS2_PLACEMENT_3D('',#133566,#103544,#103545) ;
#91282=AXIS2_PLACEMENT_3D('',#133575,#103550,#103551) ;
#91283=AXIS2_PLACEMENT_3D('',#133576,#103552,#103553) ;
#91284=AXIS2_PLACEMENT_3D('',#133577,#103554,#103555) ;
#91285=AXIS2_PLACEMENT_3D('',#133578,#103556,#103557) ;
#91286=AXIS2_PLACEMENT_3D('',#133579,#103558,#103559) ;
#91287=AXIS2_PLACEMENT_3D('',#133580,#103560,#103561) ;
#91288=AXIS2_PLACEMENT_3D('',#133581,#103562,#103563) ;
#91289=AXIS2_PLACEMENT_3D('',#133582,#103564,#103565) ;
#91290=AXIS2_PLACEMENT_3D('',#133583,#103566,#103567) ;
#91291=AXIS2_PLACEMENT_3D('',#133584,#103568,#103569) ;
#91292=AXIS2_PLACEMENT_3D('',#133585,#103570,#103571) ;
#91293=AXIS2_PLACEMENT_3D('',#133586,#103572,#103573) ;
#91294=AXIS2_PLACEMENT_3D('',#133587,#103574,#103575) ;
#91295=AXIS2_PLACEMENT_3D('',#133588,#103576,#103577) ;
#91296=AXIS2_PLACEMENT_3D('',#133589,#103578,#103579) ;
#91297=AXIS2_PLACEMENT_3D('',#133590,#103580,#103581) ;
#91298=AXIS2_PLACEMENT_3D('',#133599,#103586,#103587) ;
#91299=AXIS2_PLACEMENT_3D('',#133608,#103592,#103593) ;
#91300=AXIS2_PLACEMENT_3D('',#133611,#103594,#103595) ;
#91301=AXIS2_PLACEMENT_3D('',#133619,#103599,#103600) ;
#91302=AXIS2_PLACEMENT_3D('',#133625,#103604,#103605) ;
#91303=AXIS2_PLACEMENT_3D('',#133630,#103607,#103608) ;
#91304=AXIS2_PLACEMENT_3D('',#133633,#103610,#103611) ;
#91305=AXIS2_PLACEMENT_3D('',#133635,#103612,#103613) ;
#91306=AXIS2_PLACEMENT_3D('',#133638,#103615,#103616) ;
#91307=AXIS2_PLACEMENT_3D('',#133639,#103617,#103618) ;
#91308=AXIS2_PLACEMENT_3D('',#133642,#103619,#103620) ;
#91309=AXIS2_PLACEMENT_3D('',#133647,#103623,#103624) ;
#91310=AXIS2_PLACEMENT_3D('',#133653,#103628,#103629) ;
#91311=AXIS2_PLACEMENT_3D('',#133659,#103633,#103634) ;
#91312=AXIS2_PLACEMENT_3D('',#133665,#103638,#103639) ;
#91313=AXIS2_PLACEMENT_3D('',#133678,#103646,#103647) ;
#91314=AXIS2_PLACEMENT_3D('',#133691,#103654,#103655) ;
#91315=AXIS2_PLACEMENT_3D('',#133700,#103660,#103661) ;
#91316=AXIS2_PLACEMENT_3D('',#133709,#103666,#103667) ;
#91317=AXIS2_PLACEMENT_3D('',#133718,#103672,#103673) ;
#91318=AXIS2_PLACEMENT_3D('',#133727,#103678,#103679) ;
#91319=AXIS2_PLACEMENT_3D('',#133740,#103685,#103686) ;
#91320=AXIS2_PLACEMENT_3D('',#133744,#103688,#103689) ;
#91321=AXIS2_PLACEMENT_3D('',#133748,#103691,#103692) ;
#91322=AXIS2_PLACEMENT_3D('',#133751,#103694,#103695) ;
#91323=AXIS2_PLACEMENT_3D('',#133752,#103696,#103697) ;
#91324=AXIS2_PLACEMENT_3D('',#133755,#103698,#103699) ;
#91325=AXIS2_PLACEMENT_3D('',#133758,#103702,#103703) ;
#91326=AXIS2_PLACEMENT_3D('',#133762,#103706,#103707) ;
#91327=AXIS2_PLACEMENT_3D('',#133764,#103708,#103709) ;
#91328=AXIS2_PLACEMENT_3D('',#133766,#103711,#103712) ;
#91329=AXIS2_PLACEMENT_3D('',#133770,#103715,#103716) ;
#91330=AXIS2_PLACEMENT_3D('',#133772,#103717,#103718) ;
#91331=AXIS2_PLACEMENT_3D('',#133774,#103720,#103721) ;
#91332=AXIS2_PLACEMENT_3D('',#133778,#103724,#103725) ;
#91333=AXIS2_PLACEMENT_3D('',#133780,#103726,#103727) ;
#91334=AXIS2_PLACEMENT_3D('',#133782,#103729,#103730) ;
#91335=AXIS2_PLACEMENT_3D('',#133784,#103732,#103733) ;
#91336=AXIS2_PLACEMENT_3D('',#133785,#103734,#103735) ;
#91337=AXIS2_PLACEMENT_3D('',#133787,#103737,#103738) ;
#91338=AXIS2_PLACEMENT_3D('',#133790,#103741,#103742) ;
#91339=AXIS2_PLACEMENT_3D('',#133793,#103745,#103746) ;
#91340=AXIS2_PLACEMENT_3D('',#133796,#103749,#103750) ;
#91341=AXIS2_PLACEMENT_3D('',#133805,#103755,#103756) ;
#91342=AXIS2_PLACEMENT_3D('',#133814,#103761,#103762) ;
#91343=AXIS2_PLACEMENT_3D('',#133823,#103767,#103768) ;
#91344=AXIS2_PLACEMENT_3D('',#133832,#103773,#103774) ;
#91345=AXIS2_PLACEMENT_3D('',#133845,#103780,#103781) ;
#91346=AXIS2_PLACEMENT_3D('',#133849,#103783,#103784) ;
#91347=AXIS2_PLACEMENT_3D('',#133853,#103786,#103787) ;
#91348=AXIS2_PLACEMENT_3D('',#133856,#103789,#103790) ;
#91349=AXIS2_PLACEMENT_3D('',#133857,#103791,#103792) ;
#91350=AXIS2_PLACEMENT_3D('',#133861,#103794,#103795) ;
#91351=AXIS2_PLACEMENT_3D('',#133863,#103797,#103798) ;
#91352=AXIS2_PLACEMENT_3D('',#133867,#103801,#103802) ;
#91353=AXIS2_PLACEMENT_3D('',#133869,#103803,#103804) ;
#91354=AXIS2_PLACEMENT_3D('',#133871,#103806,#103807) ;
#91355=AXIS2_PLACEMENT_3D('',#133875,#103810,#103811) ;
#91356=AXIS2_PLACEMENT_3D('',#133877,#103812,#103813) ;
#91357=AXIS2_PLACEMENT_3D('',#133879,#103815,#103816) ;
#91358=AXIS2_PLACEMENT_3D('',#133883,#103819,#103820) ;
#91359=AXIS2_PLACEMENT_3D('',#133885,#103821,#103822) ;
#91360=AXIS2_PLACEMENT_3D('',#133887,#103824,#103825) ;
#91361=AXIS2_PLACEMENT_3D('',#133889,#103827,#103828) ;
#91362=AXIS2_PLACEMENT_3D('',#133898,#103833,#103834) ;
#91363=AXIS2_PLACEMENT_3D('',#133905,#103839,#103840) ;
#91364=AXIS2_PLACEMENT_3D('',#133911,#103844,#103845) ;
#91365=AXIS2_PLACEMENT_3D('',#133916,#103849,#103850) ;
#91366=AXIS2_PLACEMENT_3D('',#133920,#103852,#103853) ;
#91367=AXIS2_PLACEMENT_3D('',#133926,#103857,#103858) ;
#91368=AXIS2_PLACEMENT_3D('',#133927,#103859,#103860) ;
#91369=AXIS2_PLACEMENT_3D('',#133930,#103861,#103862) ;
#91370=AXIS2_PLACEMENT_3D('',#133932,#103863,#103864) ;
#91371=AXIS2_PLACEMENT_3D('',#133934,#103865,#103866) ;
#91372=AXIS2_PLACEMENT_3D('',#133938,#103868,#103869) ;
#91373=AXIS2_PLACEMENT_3D('',#133958,#103871,#103872) ;
#91374=AXIS2_PLACEMENT_3D('',#133965,#103873,#103874) ;
#91375=AXIS2_PLACEMENT_3D('',#133966,#103875,#103876) ;
#91376=AXIS2_PLACEMENT_3D('',#133967,#103877,#103878) ;
#91377=AXIS2_PLACEMENT_3D('',#133980,#103879,#103880) ;
#91378=AXIS2_PLACEMENT_3D('',#133981,#103881,#103882) ;
#91379=AXIS2_PLACEMENT_3D('',#133982,#103883,#103884) ;
#91380=AXIS2_PLACEMENT_3D('',#133983,#103885,#103886) ;
#91381=AXIS2_PLACEMENT_3D('',#133984,#103887,#103888) ;
#91382=AXIS2_PLACEMENT_3D('',#133985,#103889,#103890) ;
#91383=AXIS2_PLACEMENT_3D('',#133986,#103891,#103892) ;
#91384=AXIS2_PLACEMENT_3D('',#133987,#103893,#103894) ;
#91385=AXIS2_PLACEMENT_3D('',#133988,#103895,#103896) ;
#91386=AXIS2_PLACEMENT_3D('',#133989,#103897,#103898) ;
#91387=AXIS2_PLACEMENT_3D('',#133990,#103899,#103900) ;
#91388=AXIS2_PLACEMENT_3D('',#133991,#103901,#103902) ;
#91389=AXIS2_PLACEMENT_3D('',#133992,#103903,#103904) ;
#91390=AXIS2_PLACEMENT_3D('',#133993,#103905,#103906) ;
#91391=AXIS2_PLACEMENT_3D('',#133994,#103907,#103908) ;
#91392=AXIS2_PLACEMENT_3D('',#133995,#103909,#103910) ;
#91393=AXIS2_PLACEMENT_3D('',#134014,#103911,#103912) ;
#91394=AXIS2_PLACEMENT_3D('',#134015,#103913,#103914) ;
#91395=AXIS2_PLACEMENT_3D('',#134034,#103915,#103916) ;
#91396=AXIS2_PLACEMENT_3D('',#134053,#103917,#103918) ;
#91397=AXIS2_PLACEMENT_3D('',#134054,#103919,#103920) ;
#91398=AXIS2_PLACEMENT_3D('',#134055,#103921,#103922) ;
#91399=AXIS2_PLACEMENT_3D('',#134056,#103923,#103924) ;
#91400=AXIS2_PLACEMENT_3D('',#134057,#103925,#103926) ;
#91401=AXIS2_PLACEMENT_3D('',#134058,#103927,#103928) ;
#91402=AXIS2_PLACEMENT_3D('',#134059,#103929,#103930) ;
#91403=AXIS2_PLACEMENT_3D('',#134060,#103931,#103932) ;
#91404=AXIS2_PLACEMENT_3D('',#134061,#103933,#103934) ;
#91405=AXIS2_PLACEMENT_3D('',#134062,#103935,#103936) ;
#91406=AXIS2_PLACEMENT_3D('',#134063,#103937,#103938) ;
#91407=AXIS2_PLACEMENT_3D('',#134064,#103939,#103940) ;
#91408=AXIS2_PLACEMENT_3D('',#134065,#103941,#103942) ;
#91409=AXIS2_PLACEMENT_3D('',#134066,#103943,#103944) ;
#91410=AXIS2_PLACEMENT_3D('',#134067,#103945,#103946) ;
#91411=AXIS2_PLACEMENT_3D('',#134086,#103947,#103948) ;
#91412=AXIS2_PLACEMENT_3D('',#134087,#103949,#103950) ;
#91413=AXIS2_PLACEMENT_3D('',#134088,#103951,#103952) ;
#91414=AXIS2_PLACEMENT_3D('',#134089,#103953,#103954) ;
#91415=AXIS2_PLACEMENT_3D('',#134090,#103955,#103956) ;
#91416=AXIS2_PLACEMENT_3D('',#134091,#103957,#103958) ;
#91417=AXIS2_PLACEMENT_3D('',#134092,#103959,#103960) ;
#91418=AXIS2_PLACEMENT_3D('',#134093,#103961,#103962) ;
#91419=AXIS2_PLACEMENT_3D('',#134094,#103963,#103964) ;
#91420=AXIS2_PLACEMENT_3D('',#134095,#103965,#103966) ;
#91421=AXIS2_PLACEMENT_3D('',#134096,#103967,#103968) ;
#91422=AXIS2_PLACEMENT_3D('',#134109,#103969,#103970) ;
#91423=AXIS2_PLACEMENT_3D('',#134110,#103971,#103972) ;
#91424=AXIS2_PLACEMENT_3D('',#134111,#103973,#103974) ;
#91425=AXIS2_PLACEMENT_3D('',#134112,#103975,#103976) ;
#91426=AXIS2_PLACEMENT_3D('',#134113,#103977,#103978) ;
#91427=AXIS2_PLACEMENT_3D('',#134114,#103979,#103980) ;
#91428=AXIS2_PLACEMENT_3D('',#134115,#103981,#103982) ;
#91429=AXIS2_PLACEMENT_3D('',#134128,#103983,#103984) ;
#91430=AXIS2_PLACEMENT_3D('',#134129,#103985,#103986) ;
#91431=AXIS2_PLACEMENT_3D('',#134130,#103987,#103988) ;
#91432=AXIS2_PLACEMENT_3D('',#134131,#103989,#103990) ;
#91433=AXIS2_PLACEMENT_3D('',#134133,#103991,#103992) ;
#91434=AXIS2_PLACEMENT_3D('',#134153,#103993,#103994) ;
#91435=AXIS2_PLACEMENT_3D('',#134154,#103995,#103996) ;
#91436=AXIS2_PLACEMENT_3D('',#134155,#103997,#103998) ;
#91437=AXIS2_PLACEMENT_3D('',#134156,#103999,#104000) ;
#91438=AXIS2_PLACEMENT_3D('',#134157,#104001,#104002) ;
#91439=AXIS2_PLACEMENT_3D('',#134158,#104003,#104004) ;
#91440=AXIS2_PLACEMENT_3D('',#134187,#104005,#104006) ;
#91441=AXIS2_PLACEMENT_3D('',#134188,#104007,#104008) ;
#91442=AXIS2_PLACEMENT_3D('',#134189,#104009,#104010) ;
#91443=AXIS2_PLACEMENT_3D('',#134190,#104011,#104012) ;
#91444=AXIS2_PLACEMENT_3D('',#134191,#104013,#104014) ;
#91445=AXIS2_PLACEMENT_3D('',#134192,#104015,#104016) ;
#91446=AXIS2_PLACEMENT_3D('',#134193,#104017,#104018) ;
#91447=AXIS2_PLACEMENT_3D('',#134215,#104019,#104020) ;
#91448=AXIS2_PLACEMENT_3D('',#134216,#104021,#104022) ;
#91449=AXIS2_PLACEMENT_3D('',#134217,#104023,#104024) ;
#91450=AXIS2_PLACEMENT_3D('',#134218,#104025,#104026) ;
#91451=AXIS2_PLACEMENT_3D('',#134219,#104027,#104028) ;
#91452=AXIS2_PLACEMENT_3D('',#134220,#104029,#104030) ;
#91453=AXIS2_PLACEMENT_3D('',#134221,#104031,#104032) ;
#91454=AXIS2_PLACEMENT_3D('',#134222,#104033,#104034) ;
#91455=AXIS2_PLACEMENT_3D('',#134223,#104035,#104036) ;
#91456=AXIS2_PLACEMENT_3D('',#134224,#104037,#104038) ;
#91457=AXIS2_PLACEMENT_3D('',#134225,#104039,#104040) ;
#91458=AXIS2_PLACEMENT_3D('',#134226,#104041,#104042) ;
#91459=AXIS2_PLACEMENT_3D('',#134227,#104043,#104044) ;
#91460=AXIS2_PLACEMENT_3D('',#134228,#104045,#104046) ;
#91461=AXIS2_PLACEMENT_3D('',#134229,#104047,#104048) ;
#91462=AXIS2_PLACEMENT_3D('',#134230,#104049,#104050) ;
#91463=AXIS2_PLACEMENT_3D('',#134231,#104051,#104052) ;
#91464=AXIS2_PLACEMENT_3D('',#134232,#104053,#104054) ;
#91465=AXIS2_PLACEMENT_3D('',#134233,#104055,#104056) ;
#91466=AXIS2_PLACEMENT_3D('',#134234,#104057,#104058) ;
#91467=AXIS2_PLACEMENT_3D('',#134235,#104059,#104060) ;
#91468=AXIS2_PLACEMENT_3D('',#134236,#104061,#104062) ;
#91469=AXIS2_PLACEMENT_3D('',#134237,#104063,#104064) ;
#91470=AXIS2_PLACEMENT_3D('',#134238,#104065,#104066) ;
#91471=AXIS2_PLACEMENT_3D('',#134239,#104067,#104068) ;
#91472=AXIS2_PLACEMENT_3D('',#134240,#104069,#104070) ;
#91473=AXIS2_PLACEMENT_3D('',#134241,#104071,#104072) ;
#91474=AXIS2_PLACEMENT_3D('',#134242,#104073,#104074) ;
#91475=AXIS2_PLACEMENT_3D('',#134243,#104075,#104076) ;
#91476=AXIS2_PLACEMENT_3D('',#134244,#104077,#104078) ;
#91477=AXIS2_PLACEMENT_3D('',#134245,#104079,#104080) ;
#91478=AXIS2_PLACEMENT_3D('',#134246,#104081,#104082) ;
#91479=AXIS2_PLACEMENT_3D('',#134247,#104083,#104084) ;
#91480=AXIS2_PLACEMENT_3D('',#134248,#104085,#104086) ;
#91481=AXIS2_PLACEMENT_3D('',#134249,#104087,#104088) ;
#91482=AXIS2_PLACEMENT_3D('',#134250,#104089,#104090) ;
#91483=AXIS2_PLACEMENT_3D('',#134251,#104091,#104092) ;
#91484=AXIS2_PLACEMENT_3D('',#134252,#104093,#104094) ;
#91485=AXIS2_PLACEMENT_3D('',#134253,#104095,#104096) ;
#91486=AXIS2_PLACEMENT_3D('',#134254,#104097,#104098) ;
#91487=AXIS2_PLACEMENT_3D('',#134255,#104099,#104100) ;
#91488=AXIS2_PLACEMENT_3D('',#134256,#104101,#104102) ;
#91489=AXIS2_PLACEMENT_3D('',#134257,#104103,#104104) ;
#91490=AXIS2_PLACEMENT_3D('',#134258,#104105,#104106) ;
#91491=AXIS2_PLACEMENT_3D('',#134259,#104107,#104108) ;
#91492=AXIS2_PLACEMENT_3D('',#134260,#104109,#104110) ;
#91493=AXIS2_PLACEMENT_3D('',#134261,#104111,#104112) ;
#91494=AXIS2_PLACEMENT_3D('',#134262,#104113,#104114) ;
#91495=AXIS2_PLACEMENT_3D('',#134263,#104115,#104116) ;
#91496=AXIS2_PLACEMENT_3D('',#134264,#104117,#104118) ;
#91497=AXIS2_PLACEMENT_3D('',#134265,#104119,#104120) ;
#91498=AXIS2_PLACEMENT_3D('',#134266,#104121,#104122) ;
#91499=AXIS2_PLACEMENT_3D('',#134267,#104123,#104124) ;
#91500=AXIS2_PLACEMENT_3D('',#134268,#104125,#104126) ;
#91501=AXIS2_PLACEMENT_3D('',#134269,#104127,#104128) ;
#91502=AXIS2_PLACEMENT_3D('',#134270,#104129,#104130) ;
#91503=AXIS2_PLACEMENT_3D('',#134271,#104131,#104132) ;
#91504=AXIS2_PLACEMENT_3D('',#134272,#104133,#104134) ;
#91505=AXIS2_PLACEMENT_3D('',#134273,#104135,#104136) ;
#91506=AXIS2_PLACEMENT_3D('',#134274,#104137,#104138) ;
#91507=AXIS2_PLACEMENT_3D('',#134275,#104139,#104140) ;
#91508=AXIS2_PLACEMENT_3D('',#134276,#104141,#104142) ;
#91509=AXIS2_PLACEMENT_3D('',#134277,#104143,#104144) ;
#91510=AXIS2_PLACEMENT_3D('',#134278,#104145,#104146) ;
#91511=AXIS2_PLACEMENT_3D('',#134279,#104147,#104148) ;
#91512=AXIS2_PLACEMENT_3D('',#134280,#104149,#104150) ;
#91513=AXIS2_PLACEMENT_3D('',#134281,#104151,#104152) ;
#91514=AXIS2_PLACEMENT_3D('',#134282,#104153,#104154) ;
#91515=AXIS2_PLACEMENT_3D('',#134283,#104155,#104156) ;
#91516=AXIS2_PLACEMENT_3D('',#134284,#104157,#104158) ;
#91517=AXIS2_PLACEMENT_3D('',#134285,#104159,#104160) ;
#91518=AXIS2_PLACEMENT_3D('',#134286,#104161,#104162) ;
#91519=AXIS2_PLACEMENT_3D('',#134287,#104163,#104164) ;
#91520=AXIS2_PLACEMENT_3D('',#134288,#104165,#104166) ;
#91521=AXIS2_PLACEMENT_3D('',#134289,#104167,#104168) ;
#91522=AXIS2_PLACEMENT_3D('',#134290,#104169,#104170) ;
#91523=AXIS2_PLACEMENT_3D('',#134291,#104171,#104172) ;
#91524=AXIS2_PLACEMENT_3D('',#134292,#104173,#104174) ;
#91525=AXIS2_PLACEMENT_3D('',#134293,#104175,#104176) ;
#91526=AXIS2_PLACEMENT_3D('',#134294,#104177,#104178) ;
#91527=AXIS2_PLACEMENT_3D('',#134295,#104179,#104180) ;
#91528=AXIS2_PLACEMENT_3D('',#134296,#104181,#104182) ;
#91529=AXIS2_PLACEMENT_3D('',#134297,#104183,#104184) ;
#91530=AXIS2_PLACEMENT_3D('',#134298,#104185,#104186) ;
#91531=AXIS2_PLACEMENT_3D('',#134299,#104187,#104188) ;
#91532=AXIS2_PLACEMENT_3D('',#134300,#104189,#104190) ;
#91533=AXIS2_PLACEMENT_3D('',#134301,#104191,#104192) ;
#91534=AXIS2_PLACEMENT_3D('',#134302,#104193,#104194) ;
#91535=AXIS2_PLACEMENT_3D('',#134303,#104195,#104196) ;
#91536=AXIS2_PLACEMENT_3D('',#134304,#104197,#104198) ;
#91537=AXIS2_PLACEMENT_3D('',#134305,#104199,#104200) ;
#91538=AXIS2_PLACEMENT_3D('',#134306,#104201,#104202) ;
#91539=AXIS2_PLACEMENT_3D('',#134307,#104203,#104204) ;
#91540=AXIS2_PLACEMENT_3D('',#134308,#104205,#104206) ;
#91541=AXIS2_PLACEMENT_3D('',#134309,#104207,#104208) ;
#91542=AXIS2_PLACEMENT_3D('',#134310,#104209,#104210) ;
#91543=AXIS2_PLACEMENT_3D('',#134311,#104211,#104212) ;
#91544=AXIS2_PLACEMENT_3D('',#134312,#104213,#104214) ;
#91545=AXIS2_PLACEMENT_3D('',#134313,#104215,#104216) ;
#91546=AXIS2_PLACEMENT_3D('',#134314,#104217,#104218) ;
#91547=AXIS2_PLACEMENT_3D('',#134315,#104219,#104220) ;
#91548=AXIS2_PLACEMENT_3D('',#134316,#104221,#104222) ;
#91549=AXIS2_PLACEMENT_3D('',#134317,#104223,#104224) ;
#91550=AXIS2_PLACEMENT_3D('',#134318,#104225,#104226) ;
#91551=AXIS2_PLACEMENT_3D('',#134319,#104227,#104228) ;
#91552=AXIS2_PLACEMENT_3D('',#134320,#104229,#104230) ;
#91553=AXIS2_PLACEMENT_3D('',#134321,#104231,#104232) ;
#91554=AXIS2_PLACEMENT_3D('',#134322,#104233,#104234) ;
#91555=AXIS2_PLACEMENT_3D('',#134323,#104235,#104236) ;
#91556=AXIS2_PLACEMENT_3D('',#134336,#104237,#104238) ;
#91557=AXIS2_PLACEMENT_3D('',#134337,#104239,#104240) ;
#91558=AXIS2_PLACEMENT_3D('',#134338,#104241,#104242) ;
#91559=AXIS2_PLACEMENT_3D('',#134339,#104243,#104244) ;
#91560=AXIS2_PLACEMENT_3D('',#134340,#104245,#104246) ;
#91561=AXIS2_PLACEMENT_3D('',#134341,#104247,#104248) ;
#91562=AXIS2_PLACEMENT_3D('',#134342,#104249,#104250) ;
#91563=AXIS2_PLACEMENT_3D('',#134343,#104251,#104252) ;
#91564=AXIS2_PLACEMENT_3D('',#134344,#104253,#104254) ;
#91565=AXIS2_PLACEMENT_3D('',#134345,#104255,#104256) ;
#91566=AXIS2_PLACEMENT_3D('',#134346,#104257,#104258) ;
#91567=AXIS2_PLACEMENT_3D('',#134347,#104259,#104260) ;
#91568=AXIS2_PLACEMENT_3D('',#134348,#104261,#104262) ;
#91569=AXIS2_PLACEMENT_3D('',#134349,#104263,#104264) ;
#91570=AXIS2_PLACEMENT_3D('',#134350,#104265,#104266) ;
#91571=AXIS2_PLACEMENT_3D('',#134351,#104267,#104268) ;
#91572=AXIS2_PLACEMENT_3D('',#134352,#104269,#104270) ;
#91573=AXIS2_PLACEMENT_3D('',#134353,#104271,#104272) ;
#91574=AXIS2_PLACEMENT_3D('',#134354,#104273,#104274) ;
#91575=AXIS2_PLACEMENT_3D('',#134355,#104275,#104276) ;
#91576=AXIS2_PLACEMENT_3D('',#134356,#104277,#104278) ;
#91577=AXIS2_PLACEMENT_3D('',#134357,#104279,#104280) ;
#91578=AXIS2_PLACEMENT_3D('',#134358,#104281,#104282) ;
#91579=AXIS2_PLACEMENT_3D('',#134359,#104283,#104284) ;
#91580=AXIS2_PLACEMENT_3D('',#134360,#104285,#104286) ;
#91581=AXIS2_PLACEMENT_3D('',#134361,#104287,#104288) ;
#91582=AXIS2_PLACEMENT_3D('',#134374,#104289,#104290) ;
#91583=AXIS2_PLACEMENT_3D('',#134375,#104291,#104292) ;
#91584=AXIS2_PLACEMENT_3D('',#134376,#104293,#104294) ;
#91585=AXIS2_PLACEMENT_3D('',#134377,#104295,#104296) ;
#91586=AXIS2_PLACEMENT_3D('',#134378,#104297,#104298) ;
#91587=AXIS2_PLACEMENT_3D('',#134379,#104299,#104300) ;
#91588=AXIS2_PLACEMENT_3D('',#134380,#104301,#104302) ;
#91589=AXIS2_PLACEMENT_3D('',#134381,#104303,#104304) ;
#91590=AXIS2_PLACEMENT_3D('',#134382,#104305,#104306) ;
#91591=AXIS2_PLACEMENT_3D('',#134383,#104307,#104308) ;
#91592=AXIS2_PLACEMENT_3D('',#134384,#104309,#104310) ;
#91593=AXIS2_PLACEMENT_3D('',#134385,#104311,#104312) ;
#91594=AXIS2_PLACEMENT_3D('',#134386,#104313,#104314) ;
#91595=AXIS2_PLACEMENT_3D('',#134387,#104315,#104316) ;
#91596=AXIS2_PLACEMENT_3D('',#134388,#104317,#104318) ;
#91597=AXIS2_PLACEMENT_3D('',#134389,#104319,#104320) ;
#91598=AXIS2_PLACEMENT_3D('',#134390,#104321,#104322) ;
#91599=AXIS2_PLACEMENT_3D('',#134391,#104323,#104324) ;
#91600=AXIS2_PLACEMENT_3D('',#134392,#104325,#104326) ;
#91601=AXIS2_PLACEMENT_3D('',#134393,#104327,#104328) ;
#91602=AXIS2_PLACEMENT_3D('',#134394,#104329,#104330) ;
#91603=AXIS2_PLACEMENT_3D('',#134395,#104331,#104332) ;
#91604=AXIS2_PLACEMENT_3D('',#134396,#104333,#104334) ;
#91605=AXIS2_PLACEMENT_3D('',#134397,#104335,#104336) ;
#91606=AXIS2_PLACEMENT_3D('',#134398,#104337,#104338) ;
#91607=AXIS2_PLACEMENT_3D('',#134399,#104339,#104340) ;
#91608=AXIS2_PLACEMENT_3D('',#134400,#104341,#104342) ;
#91609=AXIS2_PLACEMENT_3D('',#134401,#104343,#104344) ;
#91610=AXIS2_PLACEMENT_3D('',#134414,#104345,#104346) ;
#91611=AXIS2_PLACEMENT_3D('',#134427,#104347,#104348) ;
#91612=AXIS2_PLACEMENT_3D('',#134428,#104349,#104350) ;
#91613=AXIS2_PLACEMENT_3D('',#134429,#104351,#104352) ;
#91614=AXIS2_PLACEMENT_3D('',#134430,#104353,#104354) ;
#91615=AXIS2_PLACEMENT_3D('',#134431,#104355,#104356) ;
#91616=AXIS2_PLACEMENT_3D('',#134444,#104357,#104358) ;
#91617=AXIS2_PLACEMENT_3D('',#134457,#104359,#104360) ;
#91618=AXIS2_PLACEMENT_3D('',#134458,#104361,#104362) ;
#91619=AXIS2_PLACEMENT_3D('',#134459,#104363,#104364) ;
#91620=AXIS2_PLACEMENT_3D('',#134460,#104365,#104366) ;
#91621=AXIS2_PLACEMENT_3D('',#134538,#104367,#104368) ;
#91622=AXIS2_PLACEMENT_3D('',#134539,#104369,#104370) ;
#91623=AXIS2_PLACEMENT_3D('',#134608,#104371,#104372) ;
#91624=AXIS2_PLACEMENT_3D('',#134609,#104373,#104374) ;
#91625=AXIS2_PLACEMENT_3D('',#134610,#104375,#104376) ;
#91626=AXIS2_PLACEMENT_3D('',#134725,#104377,#104378) ;
#91627=AXIS2_PLACEMENT_3D('',#134756,#104379,#104380) ;
#91628=AXIS2_PLACEMENT_3D('',#134787,#104381,#104382) ;
#91629=AXIS2_PLACEMENT_3D('',#134836,#104383,#104384) ;
#91630=AXIS2_PLACEMENT_3D('',#134837,#104385,#104386) ;
#91631=AXIS2_PLACEMENT_3D('',#134846,#104391,#104392) ;
#91632=AXIS2_PLACEMENT_3D('',#134848,#104393,#104394) ;
#91633=AXIS2_PLACEMENT_3D('',#134851,#104396,#104397) ;
#91634=AXIS2_PLACEMENT_3D('',#134852,#104398,#104399) ;
#91635=AXIS2_PLACEMENT_3D('',#134858,#104403,#104404) ;
#91636=AXIS2_PLACEMENT_3D('',#134860,#104405,#104406) ;
#91637=AXIS2_PLACEMENT_3D('',#134863,#104408,#104409) ;
#91638=AXIS2_PLACEMENT_3D('',#134864,#104410,#104411) ;
#91639=AXIS2_PLACEMENT_3D('',#134870,#104415,#104416) ;
#91640=AXIS2_PLACEMENT_3D('',#134872,#104417,#104418) ;
#91641=AXIS2_PLACEMENT_3D('',#134875,#104420,#104421) ;
#91642=AXIS2_PLACEMENT_3D('',#134876,#104422,#104423) ;
#91643=AXIS2_PLACEMENT_3D('',#134882,#104427,#104428) ;
#91644=AXIS2_PLACEMENT_3D('',#134884,#104429,#104430) ;
#91645=AXIS2_PLACEMENT_3D('',#134887,#104432,#104433) ;
#91646=AXIS2_PLACEMENT_3D('',#134888,#104434,#104435) ;
#91647=AXIS2_PLACEMENT_3D('',#134894,#104439,#104440) ;
#91648=AXIS2_PLACEMENT_3D('',#134897,#104441,#104442) ;
#91649=AXIS2_PLACEMENT_3D('',#134909,#104449,#104450) ;
#91650=AXIS2_PLACEMENT_3D('',#134920,#104455,#104456) ;
#91651=AXIS2_PLACEMENT_3D('',#134924,#104459,#104460) ;
#91652=AXIS2_PLACEMENT_3D('',#134927,#104461,#104462) ;
#91653=AXIS2_PLACEMENT_3D('',#134933,#104466,#104467) ;
#91654=AXIS2_PLACEMENT_3D('',#134941,#104472,#104473) ;
#91655=AXIS2_PLACEMENT_3D('',#134943,#104475,#104476) ;
#91656=AXIS2_PLACEMENT_3D('',#134952,#104481,#104482) ;
#91657=AXIS2_PLACEMENT_3D('',#134953,#104483,#104484) ;
#91658=AXIS2_PLACEMENT_3D('',#134954,#104485,#104486) ;
#91659=AXIS2_PLACEMENT_3D('',#134955,#104487,#104488) ;
#91660=AXIS2_PLACEMENT_3D('',#134956,#104489,#104490) ;
#91661=AXIS2_PLACEMENT_3D('',#134957,#104491,#104492) ;
#91662=AXIS2_PLACEMENT_3D('',#134958,#104493,#104494) ;
#91663=AXIS2_PLACEMENT_3D('',#134967,#104499,#104500) ;
#91664=AXIS2_PLACEMENT_3D('',#134976,#104505,#104506) ;
#91665=AXIS2_PLACEMENT_3D('',#134979,#104507,#104508) ;
#91666=AXIS2_PLACEMENT_3D('',#134987,#104512,#104513) ;
#91667=AXIS2_PLACEMENT_3D('',#134993,#104517,#104518) ;
#91668=AXIS2_PLACEMENT_3D('',#134998,#104520,#104521) ;
#91669=AXIS2_PLACEMENT_3D('',#135001,#104523,#104524) ;
#91670=AXIS2_PLACEMENT_3D('',#135003,#104525,#104526) ;
#91671=AXIS2_PLACEMENT_3D('',#135006,#104528,#104529) ;
#91672=AXIS2_PLACEMENT_3D('',#135007,#104530,#104531) ;
#91673=AXIS2_PLACEMENT_3D('',#135010,#104532,#104533) ;
#91674=AXIS2_PLACEMENT_3D('',#135015,#104536,#104537) ;
#91675=AXIS2_PLACEMENT_3D('',#135021,#104541,#104542) ;
#91676=AXIS2_PLACEMENT_3D('',#135027,#104546,#104547) ;
#91677=AXIS2_PLACEMENT_3D('',#135033,#104551,#104552) ;
#91678=AXIS2_PLACEMENT_3D('',#135046,#104559,#104560) ;
#91679=AXIS2_PLACEMENT_3D('',#135059,#104567,#104568) ;
#91680=AXIS2_PLACEMENT_3D('',#135068,#104573,#104574) ;
#91681=AXIS2_PLACEMENT_3D('',#135077,#104579,#104580) ;
#91682=AXIS2_PLACEMENT_3D('',#135086,#104585,#104586) ;
#91683=AXIS2_PLACEMENT_3D('',#135095,#104591,#104592) ;
#91684=AXIS2_PLACEMENT_3D('',#135108,#104598,#104599) ;
#91685=AXIS2_PLACEMENT_3D('',#135112,#104601,#104602) ;
#91686=AXIS2_PLACEMENT_3D('',#135116,#104604,#104605) ;
#91687=AXIS2_PLACEMENT_3D('',#135119,#104607,#104608) ;
#91688=AXIS2_PLACEMENT_3D('',#135120,#104609,#104610) ;
#91689=AXIS2_PLACEMENT_3D('',#135123,#104611,#104612) ;
#91690=AXIS2_PLACEMENT_3D('',#135126,#104615,#104616) ;
#91691=AXIS2_PLACEMENT_3D('',#135130,#104619,#104620) ;
#91692=AXIS2_PLACEMENT_3D('',#135132,#104621,#104622) ;
#91693=AXIS2_PLACEMENT_3D('',#135134,#104624,#104625) ;
#91694=AXIS2_PLACEMENT_3D('',#135138,#104628,#104629) ;
#91695=AXIS2_PLACEMENT_3D('',#135140,#104630,#104631) ;
#91696=AXIS2_PLACEMENT_3D('',#135142,#104633,#104634) ;
#91697=AXIS2_PLACEMENT_3D('',#135146,#104637,#104638) ;
#91698=AXIS2_PLACEMENT_3D('',#135148,#104639,#104640) ;
#91699=AXIS2_PLACEMENT_3D('',#135150,#104642,#104643) ;
#91700=AXIS2_PLACEMENT_3D('',#135152,#104645,#104646) ;
#91701=AXIS2_PLACEMENT_3D('',#135153,#104647,#104648) ;
#91702=AXIS2_PLACEMENT_3D('',#135155,#104650,#104651) ;
#91703=AXIS2_PLACEMENT_3D('',#135158,#104654,#104655) ;
#91704=AXIS2_PLACEMENT_3D('',#135161,#104658,#104659) ;
#91705=AXIS2_PLACEMENT_3D('',#135164,#104662,#104663) ;
#91706=AXIS2_PLACEMENT_3D('',#135173,#104668,#104669) ;
#91707=AXIS2_PLACEMENT_3D('',#135182,#104674,#104675) ;
#91708=AXIS2_PLACEMENT_3D('',#135191,#104680,#104681) ;
#91709=AXIS2_PLACEMENT_3D('',#135200,#104686,#104687) ;
#91710=AXIS2_PLACEMENT_3D('',#135213,#104693,#104694) ;
#91711=AXIS2_PLACEMENT_3D('',#135217,#104696,#104697) ;
#91712=AXIS2_PLACEMENT_3D('',#135221,#104699,#104700) ;
#91713=AXIS2_PLACEMENT_3D('',#135224,#104702,#104703) ;
#91714=AXIS2_PLACEMENT_3D('',#135225,#104704,#104705) ;
#91715=AXIS2_PLACEMENT_3D('',#135229,#104707,#104708) ;
#91716=AXIS2_PLACEMENT_3D('',#135231,#104710,#104711) ;
#91717=AXIS2_PLACEMENT_3D('',#135235,#104714,#104715) ;
#91718=AXIS2_PLACEMENT_3D('',#135237,#104716,#104717) ;
#91719=AXIS2_PLACEMENT_3D('',#135239,#104719,#104720) ;
#91720=AXIS2_PLACEMENT_3D('',#135243,#104723,#104724) ;
#91721=AXIS2_PLACEMENT_3D('',#135245,#104725,#104726) ;
#91722=AXIS2_PLACEMENT_3D('',#135247,#104728,#104729) ;
#91723=AXIS2_PLACEMENT_3D('',#135251,#104732,#104733) ;
#91724=AXIS2_PLACEMENT_3D('',#135253,#104734,#104735) ;
#91725=AXIS2_PLACEMENT_3D('',#135255,#104737,#104738) ;
#91726=AXIS2_PLACEMENT_3D('',#135257,#104740,#104741) ;
#91727=AXIS2_PLACEMENT_3D('',#135266,#104746,#104747) ;
#91728=AXIS2_PLACEMENT_3D('',#135273,#104752,#104753) ;
#91729=AXIS2_PLACEMENT_3D('',#135279,#104757,#104758) ;
#91730=AXIS2_PLACEMENT_3D('',#135284,#104762,#104763) ;
#91731=AXIS2_PLACEMENT_3D('',#135288,#104765,#104766) ;
#91732=AXIS2_PLACEMENT_3D('',#135294,#104770,#104771) ;
#91733=AXIS2_PLACEMENT_3D('',#135295,#104772,#104773) ;
#91734=AXIS2_PLACEMENT_3D('',#135298,#104774,#104775) ;
#91735=AXIS2_PLACEMENT_3D('',#135300,#104776,#104777) ;
#91736=AXIS2_PLACEMENT_3D('',#135302,#104778,#104779) ;
#91737=AXIS2_PLACEMENT_3D('',#135306,#104781,#104782) ;
#91738=AXIS2_PLACEMENT_3D('',#135326,#104784,#104785) ;
#91739=AXIS2_PLACEMENT_3D('',#135333,#104786,#104787) ;
#91740=AXIS2_PLACEMENT_3D('',#135334,#104788,#104789) ;
#91741=AXIS2_PLACEMENT_3D('',#135335,#104790,#104791) ;
#91742=AXIS2_PLACEMENT_3D('',#135348,#104792,#104793) ;
#91743=AXIS2_PLACEMENT_3D('',#135349,#104794,#104795) ;
#91744=AXIS2_PLACEMENT_3D('',#135350,#104796,#104797) ;
#91745=AXIS2_PLACEMENT_3D('',#135351,#104798,#104799) ;
#91746=AXIS2_PLACEMENT_3D('',#135352,#104800,#104801) ;
#91747=AXIS2_PLACEMENT_3D('',#135353,#104802,#104803) ;
#91748=AXIS2_PLACEMENT_3D('',#135354,#104804,#104805) ;
#91749=AXIS2_PLACEMENT_3D('',#135355,#104806,#104807) ;
#91750=AXIS2_PLACEMENT_3D('',#135356,#104808,#104809) ;
#91751=AXIS2_PLACEMENT_3D('',#135357,#104810,#104811) ;
#91752=AXIS2_PLACEMENT_3D('',#135358,#104812,#104813) ;
#91753=AXIS2_PLACEMENT_3D('',#135359,#104814,#104815) ;
#91754=AXIS2_PLACEMENT_3D('',#135360,#104816,#104817) ;
#91755=AXIS2_PLACEMENT_3D('',#135361,#104818,#104819) ;
#91756=AXIS2_PLACEMENT_3D('',#135362,#104820,#104821) ;
#91757=AXIS2_PLACEMENT_3D('',#135363,#104822,#104823) ;
#91758=AXIS2_PLACEMENT_3D('',#135382,#104824,#104825) ;
#91759=AXIS2_PLACEMENT_3D('',#135383,#104826,#104827) ;
#91760=AXIS2_PLACEMENT_3D('',#135402,#104828,#104829) ;
#91761=AXIS2_PLACEMENT_3D('',#135421,#104830,#104831) ;
#91762=AXIS2_PLACEMENT_3D('',#135422,#104832,#104833) ;
#91763=AXIS2_PLACEMENT_3D('',#135423,#104834,#104835) ;
#91764=AXIS2_PLACEMENT_3D('',#135424,#104836,#104837) ;
#91765=AXIS2_PLACEMENT_3D('',#135425,#104838,#104839) ;
#91766=AXIS2_PLACEMENT_3D('',#135426,#104840,#104841) ;
#91767=AXIS2_PLACEMENT_3D('',#135427,#104842,#104843) ;
#91768=AXIS2_PLACEMENT_3D('',#135428,#104844,#104845) ;
#91769=AXIS2_PLACEMENT_3D('',#135429,#104846,#104847) ;
#91770=AXIS2_PLACEMENT_3D('',#135430,#104848,#104849) ;
#91771=AXIS2_PLACEMENT_3D('',#135431,#104850,#104851) ;
#91772=AXIS2_PLACEMENT_3D('',#135432,#104852,#104853) ;
#91773=AXIS2_PLACEMENT_3D('',#135433,#104854,#104855) ;
#91774=AXIS2_PLACEMENT_3D('',#135434,#104856,#104857) ;
#91775=AXIS2_PLACEMENT_3D('',#135435,#104858,#104859) ;
#91776=AXIS2_PLACEMENT_3D('',#135454,#104860,#104861) ;
#91777=AXIS2_PLACEMENT_3D('',#135455,#104862,#104863) ;
#91778=AXIS2_PLACEMENT_3D('',#135456,#104864,#104865) ;
#91779=AXIS2_PLACEMENT_3D('',#135457,#104866,#104867) ;
#91780=AXIS2_PLACEMENT_3D('',#135458,#104868,#104869) ;
#91781=AXIS2_PLACEMENT_3D('',#135459,#104870,#104871) ;
#91782=AXIS2_PLACEMENT_3D('',#135460,#104872,#104873) ;
#91783=AXIS2_PLACEMENT_3D('',#135461,#104874,#104875) ;
#91784=AXIS2_PLACEMENT_3D('',#135462,#104876,#104877) ;
#91785=AXIS2_PLACEMENT_3D('',#135463,#104878,#104879) ;
#91786=AXIS2_PLACEMENT_3D('',#135464,#104880,#104881) ;
#91787=AXIS2_PLACEMENT_3D('',#135477,#104882,#104883) ;
#91788=AXIS2_PLACEMENT_3D('',#135478,#104884,#104885) ;
#91789=AXIS2_PLACEMENT_3D('',#135479,#104886,#104887) ;
#91790=AXIS2_PLACEMENT_3D('',#135480,#104888,#104889) ;
#91791=AXIS2_PLACEMENT_3D('',#135481,#104890,#104891) ;
#91792=AXIS2_PLACEMENT_3D('',#135482,#104892,#104893) ;
#91793=AXIS2_PLACEMENT_3D('',#135483,#104894,#104895) ;
#91794=AXIS2_PLACEMENT_3D('',#135496,#104896,#104897) ;
#91795=AXIS2_PLACEMENT_3D('',#135497,#104898,#104899) ;
#91796=AXIS2_PLACEMENT_3D('',#135498,#104900,#104901) ;
#91797=AXIS2_PLACEMENT_3D('',#135499,#104902,#104903) ;
#91798=AXIS2_PLACEMENT_3D('',#135501,#104904,#104905) ;
#91799=AXIS2_PLACEMENT_3D('',#135521,#104906,#104907) ;
#91800=AXIS2_PLACEMENT_3D('',#135522,#104908,#104909) ;
#91801=AXIS2_PLACEMENT_3D('',#135523,#104910,#104911) ;
#91802=AXIS2_PLACEMENT_3D('',#135524,#104912,#104913) ;
#91803=AXIS2_PLACEMENT_3D('',#135525,#104914,#104915) ;
#91804=AXIS2_PLACEMENT_3D('',#135526,#104916,#104917) ;
#91805=AXIS2_PLACEMENT_3D('',#135555,#104918,#104919) ;
#91806=AXIS2_PLACEMENT_3D('',#135556,#104920,#104921) ;
#91807=AXIS2_PLACEMENT_3D('',#135557,#104922,#104923) ;
#91808=AXIS2_PLACEMENT_3D('',#135558,#104924,#104925) ;
#91809=AXIS2_PLACEMENT_3D('',#135559,#104926,#104927) ;
#91810=AXIS2_PLACEMENT_3D('',#135560,#104928,#104929) ;
#91811=AXIS2_PLACEMENT_3D('',#135582,#104930,#104931) ;
#91812=AXIS2_PLACEMENT_3D('',#135583,#104932,#104933) ;
#91813=AXIS2_PLACEMENT_3D('',#135584,#104934,#104935) ;
#91814=AXIS2_PLACEMENT_3D('',#135585,#104936,#104937) ;
#91815=AXIS2_PLACEMENT_3D('',#135586,#104938,#104939) ;
#91816=AXIS2_PLACEMENT_3D('',#135587,#104940,#104941) ;
#91817=AXIS2_PLACEMENT_3D('',#135588,#104942,#104943) ;
#91818=AXIS2_PLACEMENT_3D('',#135589,#104944,#104945) ;
#91819=AXIS2_PLACEMENT_3D('',#135590,#104946,#104947) ;
#91820=AXIS2_PLACEMENT_3D('',#135591,#104948,#104949) ;
#91821=AXIS2_PLACEMENT_3D('',#135592,#104950,#104951) ;
#91822=AXIS2_PLACEMENT_3D('',#135593,#104952,#104953) ;
#91823=AXIS2_PLACEMENT_3D('',#135594,#104954,#104955) ;
#91824=AXIS2_PLACEMENT_3D('',#135595,#104956,#104957) ;
#91825=AXIS2_PLACEMENT_3D('',#135596,#104958,#104959) ;
#91826=AXIS2_PLACEMENT_3D('',#135597,#104960,#104961) ;
#91827=AXIS2_PLACEMENT_3D('',#135598,#104962,#104963) ;
#91828=AXIS2_PLACEMENT_3D('',#135599,#104964,#104965) ;
#91829=AXIS2_PLACEMENT_3D('',#135600,#104966,#104967) ;
#91830=AXIS2_PLACEMENT_3D('',#135601,#104968,#104969) ;
#91831=AXIS2_PLACEMENT_3D('',#135602,#104970,#104971) ;
#91832=AXIS2_PLACEMENT_3D('',#135603,#104972,#104973) ;
#91833=AXIS2_PLACEMENT_3D('',#135604,#104974,#104975) ;
#91834=AXIS2_PLACEMENT_3D('',#135605,#104976,#104977) ;
#91835=AXIS2_PLACEMENT_3D('',#135606,#104978,#104979) ;
#91836=AXIS2_PLACEMENT_3D('',#135607,#104980,#104981) ;
#91837=AXIS2_PLACEMENT_3D('',#135608,#104982,#104983) ;
#91838=AXIS2_PLACEMENT_3D('',#135609,#104984,#104985) ;
#91839=AXIS2_PLACEMENT_3D('',#135610,#104986,#104987) ;
#91840=AXIS2_PLACEMENT_3D('',#135611,#104988,#104989) ;
#91841=AXIS2_PLACEMENT_3D('',#135612,#104990,#104991) ;
#91842=AXIS2_PLACEMENT_3D('',#135613,#104992,#104993) ;
#91843=AXIS2_PLACEMENT_3D('',#135614,#104994,#104995) ;
#91844=AXIS2_PLACEMENT_3D('',#135615,#104996,#104997) ;
#91845=AXIS2_PLACEMENT_3D('',#135616,#104998,#104999) ;
#91846=AXIS2_PLACEMENT_3D('',#135617,#105000,#105001) ;
#91847=AXIS2_PLACEMENT_3D('',#135618,#105002,#105003) ;
#91848=AXIS2_PLACEMENT_3D('',#135619,#105004,#105005) ;
#91849=AXIS2_PLACEMENT_3D('',#135620,#105006,#105007) ;
#91850=AXIS2_PLACEMENT_3D('',#135621,#105008,#105009) ;
#91851=AXIS2_PLACEMENT_3D('',#135622,#105010,#105011) ;
#91852=AXIS2_PLACEMENT_3D('',#135623,#105012,#105013) ;
#91853=AXIS2_PLACEMENT_3D('',#135624,#105014,#105015) ;
#91854=AXIS2_PLACEMENT_3D('',#135625,#105016,#105017) ;
#91855=AXIS2_PLACEMENT_3D('',#135626,#105018,#105019) ;
#91856=AXIS2_PLACEMENT_3D('',#135627,#105020,#105021) ;
#91857=AXIS2_PLACEMENT_3D('',#135628,#105022,#105023) ;
#91858=AXIS2_PLACEMENT_3D('',#135629,#105024,#105025) ;
#91859=AXIS2_PLACEMENT_3D('',#135630,#105026,#105027) ;
#91860=AXIS2_PLACEMENT_3D('',#135631,#105028,#105029) ;
#91861=AXIS2_PLACEMENT_3D('',#135632,#105030,#105031) ;
#91862=AXIS2_PLACEMENT_3D('',#135633,#105032,#105033) ;
#91863=AXIS2_PLACEMENT_3D('',#135634,#105034,#105035) ;
#91864=AXIS2_PLACEMENT_3D('',#135635,#105036,#105037) ;
#91865=AXIS2_PLACEMENT_3D('',#135636,#105038,#105039) ;
#91866=AXIS2_PLACEMENT_3D('',#135637,#105040,#105041) ;
#91867=AXIS2_PLACEMENT_3D('',#135638,#105042,#105043) ;
#91868=AXIS2_PLACEMENT_3D('',#135639,#105044,#105045) ;
#91869=AXIS2_PLACEMENT_3D('',#135640,#105046,#105047) ;
#91870=AXIS2_PLACEMENT_3D('',#135641,#105048,#105049) ;
#91871=AXIS2_PLACEMENT_3D('',#135642,#105050,#105051) ;
#91872=AXIS2_PLACEMENT_3D('',#135643,#105052,#105053) ;
#91873=AXIS2_PLACEMENT_3D('',#135644,#105054,#105055) ;
#91874=AXIS2_PLACEMENT_3D('',#135645,#105056,#105057) ;
#91875=AXIS2_PLACEMENT_3D('',#135646,#105058,#105059) ;
#91876=AXIS2_PLACEMENT_3D('',#135647,#105060,#105061) ;
#91877=AXIS2_PLACEMENT_3D('',#135648,#105062,#105063) ;
#91878=AXIS2_PLACEMENT_3D('',#135649,#105064,#105065) ;
#91879=AXIS2_PLACEMENT_3D('',#135650,#105066,#105067) ;
#91880=AXIS2_PLACEMENT_3D('',#135651,#105068,#105069) ;
#91881=AXIS2_PLACEMENT_3D('',#135652,#105070,#105071) ;
#91882=AXIS2_PLACEMENT_3D('',#135653,#105072,#105073) ;
#91883=AXIS2_PLACEMENT_3D('',#135654,#105074,#105075) ;
#91884=AXIS2_PLACEMENT_3D('',#135655,#105076,#105077) ;
#91885=AXIS2_PLACEMENT_3D('',#135656,#105078,#105079) ;
#91886=AXIS2_PLACEMENT_3D('',#135657,#105080,#105081) ;
#91887=AXIS2_PLACEMENT_3D('',#135658,#105082,#105083) ;
#91888=AXIS2_PLACEMENT_3D('',#135659,#105084,#105085) ;
#91889=AXIS2_PLACEMENT_3D('',#135660,#105086,#105087) ;
#91890=AXIS2_PLACEMENT_3D('',#135661,#105088,#105089) ;
#91891=AXIS2_PLACEMENT_3D('',#135662,#105090,#105091) ;
#91892=AXIS2_PLACEMENT_3D('',#135663,#105092,#105093) ;
#91893=AXIS2_PLACEMENT_3D('',#135664,#105094,#105095) ;
#91894=AXIS2_PLACEMENT_3D('',#135665,#105096,#105097) ;
#91895=AXIS2_PLACEMENT_3D('',#135666,#105098,#105099) ;
#91896=AXIS2_PLACEMENT_3D('',#135667,#105100,#105101) ;
#91897=AXIS2_PLACEMENT_3D('',#135668,#105102,#105103) ;
#91898=AXIS2_PLACEMENT_3D('',#135669,#105104,#105105) ;
#91899=AXIS2_PLACEMENT_3D('',#135670,#105106,#105107) ;
#91900=AXIS2_PLACEMENT_3D('',#135671,#105108,#105109) ;
#91901=AXIS2_PLACEMENT_3D('',#135672,#105110,#105111) ;
#91902=AXIS2_PLACEMENT_3D('',#135673,#105112,#105113) ;
#91903=AXIS2_PLACEMENT_3D('',#135674,#105114,#105115) ;
#91904=AXIS2_PLACEMENT_3D('',#135675,#105116,#105117) ;
#91905=AXIS2_PLACEMENT_3D('',#135676,#105118,#105119) ;
#91906=AXIS2_PLACEMENT_3D('',#135677,#105120,#105121) ;
#91907=AXIS2_PLACEMENT_3D('',#135678,#105122,#105123) ;
#91908=AXIS2_PLACEMENT_3D('',#135679,#105124,#105125) ;
#91909=AXIS2_PLACEMENT_3D('',#135680,#105126,#105127) ;
#91910=AXIS2_PLACEMENT_3D('',#135681,#105128,#105129) ;
#91911=AXIS2_PLACEMENT_3D('',#135682,#105130,#105131) ;
#91912=AXIS2_PLACEMENT_3D('',#135683,#105132,#105133) ;
#91913=AXIS2_PLACEMENT_3D('',#135684,#105134,#105135) ;
#91914=AXIS2_PLACEMENT_3D('',#135685,#105136,#105137) ;
#91915=AXIS2_PLACEMENT_3D('',#135686,#105138,#105139) ;
#91916=AXIS2_PLACEMENT_3D('',#135687,#105140,#105141) ;
#91917=AXIS2_PLACEMENT_3D('',#135688,#105142,#105143) ;
#91918=AXIS2_PLACEMENT_3D('',#135689,#105144,#105145) ;
#91919=AXIS2_PLACEMENT_3D('',#135690,#105146,#105147) ;
#91920=AXIS2_PLACEMENT_3D('',#135703,#105148,#105149) ;
#91921=AXIS2_PLACEMENT_3D('',#135704,#105150,#105151) ;
#91922=AXIS2_PLACEMENT_3D('',#135705,#105152,#105153) ;
#91923=AXIS2_PLACEMENT_3D('',#135706,#105154,#105155) ;
#91924=AXIS2_PLACEMENT_3D('',#135707,#105156,#105157) ;
#91925=AXIS2_PLACEMENT_3D('',#135708,#105158,#105159) ;
#91926=AXIS2_PLACEMENT_3D('',#135709,#105160,#105161) ;
#91927=AXIS2_PLACEMENT_3D('',#135710,#105162,#105163) ;
#91928=AXIS2_PLACEMENT_3D('',#135711,#105164,#105165) ;
#91929=AXIS2_PLACEMENT_3D('',#135712,#105166,#105167) ;
#91930=AXIS2_PLACEMENT_3D('',#135713,#105168,#105169) ;
#91931=AXIS2_PLACEMENT_3D('',#135714,#105170,#105171) ;
#91932=AXIS2_PLACEMENT_3D('',#135715,#105172,#105173) ;
#91933=AXIS2_PLACEMENT_3D('',#135716,#105174,#105175) ;
#91934=AXIS2_PLACEMENT_3D('',#135717,#105176,#105177) ;
#91935=AXIS2_PLACEMENT_3D('',#135718,#105178,#105179) ;
#91936=AXIS2_PLACEMENT_3D('',#135719,#105180,#105181) ;
#91937=AXIS2_PLACEMENT_3D('',#135720,#105182,#105183) ;
#91938=AXIS2_PLACEMENT_3D('',#135721,#105184,#105185) ;
#91939=AXIS2_PLACEMENT_3D('',#135722,#105186,#105187) ;
#91940=AXIS2_PLACEMENT_3D('',#135735,#105188,#105189) ;
#91941=AXIS2_PLACEMENT_3D('',#135736,#105190,#105191) ;
#91942=AXIS2_PLACEMENT_3D('',#135737,#105192,#105193) ;
#91943=AXIS2_PLACEMENT_3D('',#135738,#105194,#105195) ;
#91944=AXIS2_PLACEMENT_3D('',#135739,#105196,#105197) ;
#91945=AXIS2_PLACEMENT_3D('',#135740,#105198,#105199) ;
#91946=AXIS2_PLACEMENT_3D('',#135741,#105200,#105201) ;
#91947=AXIS2_PLACEMENT_3D('',#135742,#105202,#105203) ;
#91948=AXIS2_PLACEMENT_3D('',#135743,#105204,#105205) ;
#91949=AXIS2_PLACEMENT_3D('',#135744,#105206,#105207) ;
#91950=AXIS2_PLACEMENT_3D('',#135757,#105208,#105209) ;
#91951=AXIS2_PLACEMENT_3D('',#135770,#105210,#105211) ;
#91952=AXIS2_PLACEMENT_3D('',#135771,#105212,#105213) ;
#91953=AXIS2_PLACEMENT_3D('',#135784,#105214,#105215) ;
#91954=AXIS2_PLACEMENT_3D('',#135797,#105216,#105217) ;
#91955=AXIS2_PLACEMENT_3D('',#135798,#105218,#105219) ;
#91956=AXIS2_PLACEMENT_3D('',#135799,#105220,#105221) ;
#91957=AXIS2_PLACEMENT_3D('',#135800,#105222,#105223) ;
#91958=AXIS2_PLACEMENT_3D('',#135946,#105224,#105225) ;
#91959=AXIS2_PLACEMENT_3D('',#135947,#105226,#105227) ;
#91960=AXIS2_PLACEMENT_3D('',#136062,#105228,#105229) ;
#91961=AXIS2_PLACEMENT_3D('',#136093,#105230,#105231) ;
#91962=AXIS2_PLACEMENT_3D('',#136124,#105232,#105233) ;
#91963=AXIS2_PLACEMENT_3D('',#136173,#105234,#105235) ;
#91964=AXIS2_PLACEMENT_3D('',#136174,#105236,#105237) ;
#91965=AXIS2_PLACEMENT_3D('',#136175,#105238,#105239) ;
#91966=AXIS2_PLACEMENT_3D('',#136176,#105240,#105241) ;
#91967=AXIS2_PLACEMENT_3D('',#136177,#105242,#105243) ;
#91968=AXIS2_PLACEMENT_3D('',#136178,#105244,#105245) ;
#91969=AXIS2_PLACEMENT_3D('',#136179,#105246,#105247) ;
#91970=AXIS2_PLACEMENT_3D('',#136180,#105248,#105249) ;
#91971=AXIS2_PLACEMENT_3D('',#136181,#105250,#105251) ;
#91972=AXIS2_PLACEMENT_3D('',#136182,#105252,#105253) ;
#91973=AXIS2_PLACEMENT_3D('',#136183,#105254,#105255) ;
#91974=AXIS2_PLACEMENT_3D('',#136184,#105256,#105257) ;
#91975=AXIS2_PLACEMENT_3D('',#136185,#105258,#105259) ;
#91976=AXIS2_PLACEMENT_3D('',#136186,#105260,#105261) ;
#91977=AXIS2_PLACEMENT_3D('',#136187,#105262,#105263) ;
#91978=AXIS2_PLACEMENT_3D('',#136188,#105264,#105265) ;
#91979=AXIS2_PLACEMENT_3D('',#136189,#105266,#105267) ;
#91980=AXIS2_PLACEMENT_3D('',#136190,#105268,#105269) ;
#91981=AXIS2_PLACEMENT_3D('',#136191,#105270,#105271) ;
#91982=AXIS2_PLACEMENT_3D('',#136192,#105272,#105273) ;
#91983=AXIS2_PLACEMENT_3D('',#136193,#105274,#105275) ;
#91984=AXIS2_PLACEMENT_3D('',#136194,#105276,#105277) ;
#91985=AXIS2_PLACEMENT_3D('',#136195,#105278,#105279) ;
#91986=AXIS2_PLACEMENT_3D('',#136196,#105280,#105281) ;
#91987=AXIS2_PLACEMENT_3D('',#136197,#105282,#105283) ;
#91988=AXIS2_PLACEMENT_3D('',#136202,#105284,#105285) ;
#91989=AXIS2_PLACEMENT_3D('',#136203,#105286,#105287) ;
#91990=AXIS2_PLACEMENT_3D('',#136204,#105288,#105289) ;
#91991=AXIS2_PLACEMENT_3D('',#136205,#105290,#105291) ;
#91992=AXIS2_PLACEMENT_3D('',#136210,#105292,#105293) ;
#91993=AXIS2_PLACEMENT_3D('',#136211,#105294,#105295) ;
#91994=AXIS2_PLACEMENT_3D('',#136212,#105296,#105297) ;
#91995=AXIS2_PLACEMENT_3D('',#136213,#105298,#105299) ;
#91996=AXIS2_PLACEMENT_3D('',#136226,#105300,#105301) ;
#91997=AXIS2_PLACEMENT_3D('',#136239,#105302,#105303) ;
#91998=AXIS2_PLACEMENT_3D('',#136240,#105304,#105305) ;
#91999=AXIS2_PLACEMENT_3D('',#136241,#105306,#105307) ;
#92000=AXIS2_PLACEMENT_3D('',#136242,#105308,#105309) ;
#92001=AXIS2_PLACEMENT_3D('',#136243,#105310,#105311) ;
#92002=AXIS2_PLACEMENT_3D('',#136244,#105312,#105313) ;
#92003=AXIS2_PLACEMENT_3D('',#136245,#105314,#105315) ;
#92004=AXIS2_PLACEMENT_3D('',#136246,#105316,#105317) ;
#92005=AXIS2_PLACEMENT_3D('',#136247,#105318,#105319) ;
#92006=AXIS2_PLACEMENT_3D('',#136248,#105320,#105321) ;
#92007=AXIS2_PLACEMENT_3D('',#136249,#105322,#105323) ;
#92008=AXIS2_PLACEMENT_3D('',#136250,#105324,#105325) ;
#92009=AXIS2_PLACEMENT_3D('',#136251,#105326,#105327) ;
#92010=AXIS2_PLACEMENT_3D('',#136252,#105328,#105329) ;
#92011=AXIS2_PLACEMENT_3D('',#136253,#105330,#105331) ;
#92012=AXIS2_PLACEMENT_3D('',#136254,#105332,#105333) ;
#92013=AXIS2_PLACEMENT_3D('',#136255,#105334,#105335) ;
#92014=AXIS2_PLACEMENT_3D('',#136258,#105336,#105337) ;
#92015=AXIS2_PLACEMENT_3D('',#136260,#105338,#105339) ;
#92016=AXIS2_PLACEMENT_3D('',#136262,#105340,#105341) ;
#92017=AXIS2_PLACEMENT_3D('',#136263,#105342,#105343) ;
#92018=AXIS2_PLACEMENT_3D('',#136264,#105344,#105345) ;
#92019=AXIS2_PLACEMENT_3D('',#136266,#105346,#105347) ;
#92020=AXIS2_PLACEMENT_3D('',#136268,#105348,#105349) ;
#92021=AXIS2_PLACEMENT_3D('',#136270,#105350,#105351) ;
#92022=AXIS2_PLACEMENT_3D('',#136271,#105352,#105353) ;
#92023=AXIS2_PLACEMENT_3D('',#136272,#105354,#105355) ;
#92024=AXIS2_PLACEMENT_3D('',#136274,#105356,#105357) ;
#92025=AXIS2_PLACEMENT_3D('',#136276,#105358,#105359) ;
#92026=AXIS2_PLACEMENT_3D('',#136277,#105360,#105361) ;
#92027=AXIS2_PLACEMENT_3D('',#136278,#105362,#105363) ;
#92028=AXIS2_PLACEMENT_3D('',#136280,#105364,#105365) ;
#92029=AXIS2_PLACEMENT_3D('',#136282,#105366,#105367) ;
#92030=AXIS2_PLACEMENT_3D('',#136284,#105368,#105369) ;
#92031=AXIS2_PLACEMENT_3D('',#136285,#105370,#105371) ;
#92032=AXIS2_PLACEMENT_3D('',#136286,#105372,#105373) ;
#92033=AXIS2_PLACEMENT_3D('',#136289,#105374,#105375) ;
#92034=AXIS2_PLACEMENT_3D('',#136291,#105376,#105377) ;
#92035=AXIS2_PLACEMENT_3D('',#136293,#105378,#105379) ;
#92036=AXIS2_PLACEMENT_3D('',#136294,#105380,#105381) ;
#92037=AXIS2_PLACEMENT_3D('',#136295,#105382,#105383) ;
#92038=AXIS2_PLACEMENT_3D('',#136298,#105384,#105385) ;
#92039=AXIS2_PLACEMENT_3D('',#136300,#105386,#105387) ;
#92040=AXIS2_PLACEMENT_3D('',#136301,#105388,#105389) ;
#92041=AXIS2_PLACEMENT_3D('',#136302,#105390,#105391) ;
#92042=AXIS2_PLACEMENT_3D('',#136306,#105393,#105394) ;
#92043=AXIS2_PLACEMENT_3D('',#136308,#105396,#105397) ;
#92044=AXIS2_PLACEMENT_3D('',#136311,#105398,#105399) ;
#92045=AXIS2_PLACEMENT_3D('',#136313,#105400,#105401) ;
#92046=AXIS2_PLACEMENT_3D('',#136314,#105402,#105403) ;
#92047=AXIS2_PLACEMENT_3D('',#136315,#105404,#105405) ;
#92048=AXIS2_PLACEMENT_3D('',#136317,#105406,#105407) ;
#92049=AXIS2_PLACEMENT_3D('',#136319,#105409,#105410) ;
#92050=AXIS2_PLACEMENT_3D('',#136321,#105412,#105413) ;
#92051=AXIS2_PLACEMENT_3D('',#136324,#105414,#105415) ;
#92052=AXIS2_PLACEMENT_3D('',#136350,#105417,#105418) ;
#92053=AXIS2_PLACEMENT_3D('',#136397,#105420,#105421) ;
#92054=AXIS2_PLACEMENT_3D('',#136423,#105423,#105424) ;
#92055=AXIS2_PLACEMENT_3D('',#136469,#105426,#105427) ;
#92056=AXIS2_PLACEMENT_3D('',#136471,#105429,#105430) ;
#92057=AXIS2_PLACEMENT_3D('',#136474,#105431,#105432) ;
#92058=AXIS2_PLACEMENT_3D('',#136476,#105433,#105434) ;
#92059=AXIS2_PLACEMENT_3D('',#136478,#105435,#105436) ;
#92060=AXIS2_PLACEMENT_3D('',#136479,#105437,#105438) ;
#92061=AXIS2_PLACEMENT_3D('',#136480,#105439,#105440) ;
#92062=AXIS2_PLACEMENT_3D('',#136483,#105441,#105442) ;
#92063=AXIS2_PLACEMENT_3D('',#136487,#105444,#105445) ;
#92064=AXIS2_PLACEMENT_3D('',#136489,#105447,#105448) ;
#92065=AXIS2_PLACEMENT_3D('',#136491,#105449,#105450) ;
#92066=AXIS2_PLACEMENT_3D('',#136493,#105451,#105452) ;
#92067=AXIS2_PLACEMENT_3D('',#136495,#105453,#105454) ;
#92068=AXIS2_PLACEMENT_3D('',#136496,#105455,#105456) ;
#92069=AXIS2_PLACEMENT_3D('',#136497,#105457,#105458) ;
#92070=AXIS2_PLACEMENT_3D('',#136499,#105459,#105460) ;
#92071=AXIS2_PLACEMENT_3D('',#136501,#105461,#105462) ;
#92072=AXIS2_PLACEMENT_3D('',#136502,#105463,#105464) ;
#92073=AXIS2_PLACEMENT_3D('',#136503,#105465,#105466) ;
#92074=AXIS2_PLACEMENT_3D('',#136505,#105467,#105468) ;
#92075=AXIS2_PLACEMENT_3D('',#136507,#105469,#105470) ;
#92076=AXIS2_PLACEMENT_3D('',#136509,#105471,#105472) ;
#92077=AXIS2_PLACEMENT_3D('',#136510,#105473,#105474) ;
#92078=AXIS2_PLACEMENT_3D('',#136511,#105475,#105476) ;
#92079=AXIS2_PLACEMENT_3D('',#136514,#105477,#105478) ;
#92080=AXIS2_PLACEMENT_3D('',#136516,#105479,#105480) ;
#92081=AXIS2_PLACEMENT_3D('',#136518,#105481,#105482) ;
#92082=AXIS2_PLACEMENT_3D('',#136519,#105483,#105484) ;
#92083=AXIS2_PLACEMENT_3D('',#136520,#105485,#105486) ;
#92084=AXIS2_PLACEMENT_3D('',#136523,#105487,#105488) ;
#92085=AXIS2_PLACEMENT_3D('',#136525,#105489,#105490) ;
#92086=AXIS2_PLACEMENT_3D('',#136526,#105491,#105492) ;
#92087=AXIS2_PLACEMENT_3D('',#136527,#105493,#105494) ;
#92088=AXIS2_PLACEMENT_3D('',#136531,#105496,#105497) ;
#92089=AXIS2_PLACEMENT_3D('',#136533,#105499,#105500) ;
#92090=AXIS2_PLACEMENT_3D('',#136536,#105501,#105502) ;
#92091=AXIS2_PLACEMENT_3D('',#136538,#105503,#105504) ;
#92092=AXIS2_PLACEMENT_3D('',#136539,#105505,#105506) ;
#92093=AXIS2_PLACEMENT_3D('',#136540,#105507,#105508) ;
#92094=AXIS2_PLACEMENT_3D('',#136542,#105509,#105510) ;
#92095=AXIS2_PLACEMENT_3D('',#136544,#105512,#105513) ;
#92096=AXIS2_PLACEMENT_3D('',#136546,#105515,#105516) ;
#92097=AXIS2_PLACEMENT_3D('',#136549,#105517,#105518) ;
#92098=AXIS2_PLACEMENT_3D('',#136575,#105520,#105521) ;
#92099=AXIS2_PLACEMENT_3D('',#136622,#105523,#105524) ;
#92100=AXIS2_PLACEMENT_3D('',#136648,#105526,#105527) ;
#92101=AXIS2_PLACEMENT_3D('',#136694,#105529,#105530) ;
#92102=AXIS2_PLACEMENT_3D('',#136696,#105532,#105533) ;
#92103=AXIS2_PLACEMENT_3D('',#136707,#105538,#105539) ;
#92104=AXIS2_PLACEMENT_3D('',#136725,#105543,#105544) ;
#92105=AXIS2_PLACEMENT_3D('',#136727,#105546,#105547) ;
#92106=AXIS2_PLACEMENT_3D('',#136736,#105552,#105553) ;
#92107=AXIS2_PLACEMENT_3D('',#136745,#105558,#105559) ;
#92108=AXIS2_PLACEMENT_3D('',#136754,#105564,#105565) ;
#92109=AXIS2_PLACEMENT_3D('',#136756,#105566,#105567) ;
#92110=AXIS2_PLACEMENT_3D('',#136759,#105569,#105570) ;
#92111=AXIS2_PLACEMENT_3D('',#136760,#105571,#105572) ;
#92112=AXIS2_PLACEMENT_3D('',#136761,#105573,#105574) ;
#92113=AXIS2_PLACEMENT_3D('',#136762,#105575,#105576) ;
#92114=AXIS2_PLACEMENT_3D('',#136763,#105577,#105578) ;
#92115=AXIS2_PLACEMENT_3D('',#136764,#105579,#105580) ;
#92116=AXIS2_PLACEMENT_3D('',#136765,#105581,#105582) ;
#92117=AXIS2_PLACEMENT_3D('',#136766,#105583,#105584) ;
#92118=AXIS2_PLACEMENT_3D('',#136769,#105585,#105586) ;
#92119=AXIS2_PLACEMENT_3D('',#136772,#105588,#105589) ;
#92120=AXIS2_PLACEMENT_3D('',#136774,#105590,#105591) ;
#92121=AXIS2_PLACEMENT_3D('',#136776,#105593,#105594) ;
#92122=AXIS2_PLACEMENT_3D('',#136779,#105595,#105596) ;
#92123=AXIS2_PLACEMENT_3D('',#136785,#105600,#105601) ;
#92124=AXIS2_PLACEMENT_3D('',#136794,#105606,#105607) ;
#92125=AXIS2_PLACEMENT_3D('',#136802,#105612,#105613) ;
#92126=AXIS2_PLACEMENT_3D('',#136804,#105615,#105616) ;
#92127=AXIS2_PLACEMENT_3D('',#136810,#105620,#105621) ;
#92128=AXIS2_PLACEMENT_3D('',#136820,#105627,#105628) ;
#92129=AXIS2_PLACEMENT_3D('',#136822,#105629,#105630) ;
#92130=AXIS2_PLACEMENT_3D('',#136824,#105631,#105632) ;
#92131=AXIS2_PLACEMENT_3D('',#136828,#105634,#105635) ;
#92132=AXIS2_PLACEMENT_3D('',#136830,#105636,#105637) ;
#92133=AXIS2_PLACEMENT_3D('',#136832,#105638,#105639) ;
#92134=AXIS2_PLACEMENT_3D('',#136841,#105644,#105645) ;
#92135=AXIS2_PLACEMENT_3D('',#136843,#105647,#105648) ;
#92136=AXIS2_PLACEMENT_3D('',#136850,#105653,#105654) ;
#92137=AXIS2_PLACEMENT_3D('',#136859,#105658,#105659) ;
#92138=AXIS2_PLACEMENT_3D('',#136863,#105661,#105662) ;
#92139=AXIS2_PLACEMENT_3D('',#136867,#105664,#105665) ;
#92140=AXIS2_PLACEMENT_3D('',#136871,#105667,#105668) ;
#92141=AXIS2_PLACEMENT_3D('',#136875,#105671,#105672) ;
#92142=AXIS2_PLACEMENT_3D('',#136881,#105676,#105677) ;
#92143=AXIS2_PLACEMENT_3D('',#136888,#105682,#105683) ;
#92144=AXIS2_PLACEMENT_3D('',#136899,#105688,#105689) ;
#92145=AXIS2_PLACEMENT_3D('',#136903,#105691,#105692) ;
#92146=AXIS2_PLACEMENT_3D('',#136907,#105694,#105695) ;
#92147=AXIS2_PLACEMENT_3D('',#136911,#105697,#105698) ;
#92148=AXIS2_PLACEMENT_3D('',#136915,#105700,#105701) ;
#92149=AXIS2_PLACEMENT_3D('',#136919,#105703,#105704) ;
#92150=AXIS2_PLACEMENT_3D('',#136923,#105706,#105707) ;
#92151=AXIS2_PLACEMENT_3D('',#136927,#105709,#105710) ;
#92152=AXIS2_PLACEMENT_3D('',#136929,#105712,#105713) ;
#92153=AXIS2_PLACEMENT_3D('',#136938,#105718,#105719) ;
#92154=AXIS2_PLACEMENT_3D('',#136944,#105723,#105724) ;
#92155=AXIS2_PLACEMENT_3D('',#136950,#105728,#105729) ;
#92156=AXIS2_PLACEMENT_3D('',#137031,#105742,#105743) ;
#92157=AXIS2_PLACEMENT_3D('',#137042,#105748,#105749) ;
#92158=AXIS2_PLACEMENT_3D('',#137046,#105751,#105752) ;
#92159=AXIS2_PLACEMENT_3D('',#137050,#105754,#105755) ;
#92160=AXIS2_PLACEMENT_3D('',#137054,#105757,#105758) ;
#92161=AXIS2_PLACEMENT_3D('',#137058,#105760,#105761) ;
#92162=AXIS2_PLACEMENT_3D('',#137062,#105763,#105764) ;
#92163=AXIS2_PLACEMENT_3D('',#137066,#105766,#105767) ;
#92164=AXIS2_PLACEMENT_3D('',#137070,#105769,#105770) ;
#92165=AXIS2_PLACEMENT_3D('',#137072,#105772,#105773) ;
#92166=AXIS2_PLACEMENT_3D('',#137081,#105778,#105779) ;
#92167=AXIS2_PLACEMENT_3D('',#137260,#105786,#105787) ;
#92168=AXIS2_PLACEMENT_3D('',#137265,#105789,#105790) ;
#92169=AXIS2_PLACEMENT_3D('',#137268,#105792,#105793) ;
#92170=AXIS2_PLACEMENT_3D('',#137269,#105794,#105795) ;
#92171=AXIS2_PLACEMENT_3D('',#137278,#105800,#105801) ;
#92172=AXIS2_PLACEMENT_3D('',#137279,#105802,#105803) ;
#92173=AXIS2_PLACEMENT_3D('',#137280,#105804,#105805) ;
#92174=AXIS2_PLACEMENT_3D('',#137281,#105806,#105807) ;
#92175=AXIS2_PLACEMENT_3D('',#137282,#105808,#105809) ;
#92176=AXIS2_PLACEMENT_3D('',#137283,#105810,#105811) ;
#92177=AXIS2_PLACEMENT_3D('',#137284,#105812,#105813) ;
#92178=AXIS2_PLACEMENT_3D('',#137285,#105814,#105815) ;
#92179=AXIS2_PLACEMENT_3D('',#137286,#105816,#105817) ;
#92180=AXIS2_PLACEMENT_3D('',#137287,#105818,#105819) ;
#92181=AXIS2_PLACEMENT_3D('',#137288,#105820,#105821) ;
#92182=AXIS2_PLACEMENT_3D('',#137289,#105822,#105823) ;
#92183=AXIS2_PLACEMENT_3D('',#137290,#105824,#105825) ;
#92184=AXIS2_PLACEMENT_3D('',#137291,#105826,#105827) ;
#92185=AXIS2_PLACEMENT_3D('',#137292,#105828,#105829) ;
#92186=AXIS2_PLACEMENT_3D('',#137293,#105830,#105831) ;
#92187=AXIS2_PLACEMENT_3D('',#137302,#105836,#105837) ;
#92188=AXIS2_PLACEMENT_3D('',#137311,#105842,#105843) ;
#92189=AXIS2_PLACEMENT_3D('',#137314,#105844,#105845) ;
#92190=AXIS2_PLACEMENT_3D('',#137322,#105849,#105850) ;
#92191=AXIS2_PLACEMENT_3D('',#137328,#105854,#105855) ;
#92192=AXIS2_PLACEMENT_3D('',#137333,#105857,#105858) ;
#92193=AXIS2_PLACEMENT_3D('',#137336,#105860,#105861) ;
#92194=AXIS2_PLACEMENT_3D('',#137338,#105862,#105863) ;
#92195=AXIS2_PLACEMENT_3D('',#137341,#105865,#105866) ;
#92196=AXIS2_PLACEMENT_3D('',#137342,#105867,#105868) ;
#92197=AXIS2_PLACEMENT_3D('',#137345,#105869,#105870) ;
#92198=AXIS2_PLACEMENT_3D('',#137350,#105873,#105874) ;
#92199=AXIS2_PLACEMENT_3D('',#137356,#105878,#105879) ;
#92200=AXIS2_PLACEMENT_3D('',#137362,#105883,#105884) ;
#92201=AXIS2_PLACEMENT_3D('',#137368,#105888,#105889) ;
#92202=AXIS2_PLACEMENT_3D('',#137381,#105896,#105897) ;
#92203=AXIS2_PLACEMENT_3D('',#137394,#105904,#105905) ;
#92204=AXIS2_PLACEMENT_3D('',#137403,#105910,#105911) ;
#92205=AXIS2_PLACEMENT_3D('',#137412,#105916,#105917) ;
#92206=AXIS2_PLACEMENT_3D('',#137421,#105922,#105923) ;
#92207=AXIS2_PLACEMENT_3D('',#137430,#105928,#105929) ;
#92208=AXIS2_PLACEMENT_3D('',#137443,#105935,#105936) ;
#92209=AXIS2_PLACEMENT_3D('',#137447,#105938,#105939) ;
#92210=AXIS2_PLACEMENT_3D('',#137451,#105941,#105942) ;
#92211=AXIS2_PLACEMENT_3D('',#137454,#105944,#105945) ;
#92212=AXIS2_PLACEMENT_3D('',#137455,#105946,#105947) ;
#92213=AXIS2_PLACEMENT_3D('',#137458,#105948,#105949) ;
#92214=AXIS2_PLACEMENT_3D('',#137461,#105952,#105953) ;
#92215=AXIS2_PLACEMENT_3D('',#137465,#105956,#105957) ;
#92216=AXIS2_PLACEMENT_3D('',#137467,#105958,#105959) ;
#92217=AXIS2_PLACEMENT_3D('',#137469,#105961,#105962) ;
#92218=AXIS2_PLACEMENT_3D('',#137473,#105965,#105966) ;
#92219=AXIS2_PLACEMENT_3D('',#137475,#105967,#105968) ;
#92220=AXIS2_PLACEMENT_3D('',#137477,#105970,#105971) ;
#92221=AXIS2_PLACEMENT_3D('',#137481,#105974,#105975) ;
#92222=AXIS2_PLACEMENT_3D('',#137483,#105976,#105977) ;
#92223=AXIS2_PLACEMENT_3D('',#137485,#105979,#105980) ;
#92224=AXIS2_PLACEMENT_3D('',#137487,#105982,#105983) ;
#92225=AXIS2_PLACEMENT_3D('',#137488,#105984,#105985) ;
#92226=AXIS2_PLACEMENT_3D('',#137490,#105987,#105988) ;
#92227=AXIS2_PLACEMENT_3D('',#137493,#105991,#105992) ;
#92228=AXIS2_PLACEMENT_3D('',#137496,#105995,#105996) ;
#92229=AXIS2_PLACEMENT_3D('',#137499,#105999,#106000) ;
#92230=AXIS2_PLACEMENT_3D('',#137508,#106005,#106006) ;
#92231=AXIS2_PLACEMENT_3D('',#137517,#106011,#106012) ;
#92232=AXIS2_PLACEMENT_3D('',#137526,#106017,#106018) ;
#92233=AXIS2_PLACEMENT_3D('',#137535,#106023,#106024) ;
#92234=AXIS2_PLACEMENT_3D('',#137548,#106030,#106031) ;
#92235=AXIS2_PLACEMENT_3D('',#137552,#106033,#106034) ;
#92236=AXIS2_PLACEMENT_3D('',#137556,#106036,#106037) ;
#92237=AXIS2_PLACEMENT_3D('',#137559,#106039,#106040) ;
#92238=AXIS2_PLACEMENT_3D('',#137560,#106041,#106042) ;
#92239=AXIS2_PLACEMENT_3D('',#137564,#106044,#106045) ;
#92240=AXIS2_PLACEMENT_3D('',#137566,#106047,#106048) ;
#92241=AXIS2_PLACEMENT_3D('',#137570,#106051,#106052) ;
#92242=AXIS2_PLACEMENT_3D('',#137572,#106053,#106054) ;
#92243=AXIS2_PLACEMENT_3D('',#137574,#106056,#106057) ;
#92244=AXIS2_PLACEMENT_3D('',#137578,#106060,#106061) ;
#92245=AXIS2_PLACEMENT_3D('',#137580,#106062,#106063) ;
#92246=AXIS2_PLACEMENT_3D('',#137582,#106065,#106066) ;
#92247=AXIS2_PLACEMENT_3D('',#137586,#106069,#106070) ;
#92248=AXIS2_PLACEMENT_3D('',#137588,#106071,#106072) ;
#92249=AXIS2_PLACEMENT_3D('',#137590,#106074,#106075) ;
#92250=AXIS2_PLACEMENT_3D('',#137592,#106077,#106078) ;
#92251=AXIS2_PLACEMENT_3D('',#137601,#106083,#106084) ;
#92252=AXIS2_PLACEMENT_3D('',#137608,#106089,#106090) ;
#92253=AXIS2_PLACEMENT_3D('',#137614,#106094,#106095) ;
#92254=AXIS2_PLACEMENT_3D('',#137619,#106099,#106100) ;
#92255=AXIS2_PLACEMENT_3D('',#137623,#106102,#106103) ;
#92256=AXIS2_PLACEMENT_3D('',#137629,#106107,#106108) ;
#92257=AXIS2_PLACEMENT_3D('',#137630,#106109,#106110) ;
#92258=AXIS2_PLACEMENT_3D('',#137633,#106111,#106112) ;
#92259=AXIS2_PLACEMENT_3D('',#137635,#106113,#106114) ;
#92260=AXIS2_PLACEMENT_3D('',#137637,#106115,#106116) ;
#92261=AXIS2_PLACEMENT_3D('',#137641,#106118,#106119) ;
#92262=AXIS2_PLACEMENT_3D('',#137661,#106121,#106122) ;
#92263=AXIS2_PLACEMENT_3D('',#137668,#106123,#106124) ;
#92264=AXIS2_PLACEMENT_3D('',#137669,#106125,#106126) ;
#92265=AXIS2_PLACEMENT_3D('',#137670,#106127,#106128) ;
#92266=AXIS2_PLACEMENT_3D('',#137683,#106129,#106130) ;
#92267=AXIS2_PLACEMENT_3D('',#137684,#106131,#106132) ;
#92268=AXIS2_PLACEMENT_3D('',#137685,#106133,#106134) ;
#92269=AXIS2_PLACEMENT_3D('',#137686,#106135,#106136) ;
#92270=AXIS2_PLACEMENT_3D('',#137687,#106137,#106138) ;
#92271=AXIS2_PLACEMENT_3D('',#137688,#106139,#106140) ;
#92272=AXIS2_PLACEMENT_3D('',#137689,#106141,#106142) ;
#92273=AXIS2_PLACEMENT_3D('',#137690,#106143,#106144) ;
#92274=AXIS2_PLACEMENT_3D('',#137691,#106145,#106146) ;
#92275=AXIS2_PLACEMENT_3D('',#137692,#106147,#106148) ;
#92276=AXIS2_PLACEMENT_3D('',#137693,#106149,#106150) ;
#92277=AXIS2_PLACEMENT_3D('',#137694,#106151,#106152) ;
#92278=AXIS2_PLACEMENT_3D('',#137695,#106153,#106154) ;
#92279=AXIS2_PLACEMENT_3D('',#137696,#106155,#106156) ;
#92280=AXIS2_PLACEMENT_3D('',#137697,#106157,#106158) ;
#92281=AXIS2_PLACEMENT_3D('',#137698,#106159,#106160) ;
#92282=AXIS2_PLACEMENT_3D('',#137717,#106161,#106162) ;
#92283=AXIS2_PLACEMENT_3D('',#137718,#106163,#106164) ;
#92284=AXIS2_PLACEMENT_3D('',#137737,#106165,#106166) ;
#92285=AXIS2_PLACEMENT_3D('',#137756,#106167,#106168) ;
#92286=AXIS2_PLACEMENT_3D('',#137757,#106169,#106170) ;
#92287=AXIS2_PLACEMENT_3D('',#137758,#106171,#106172) ;
#92288=AXIS2_PLACEMENT_3D('',#137759,#106173,#106174) ;
#92289=AXIS2_PLACEMENT_3D('',#137760,#106175,#106176) ;
#92290=AXIS2_PLACEMENT_3D('',#137761,#106177,#106178) ;
#92291=AXIS2_PLACEMENT_3D('',#137762,#106179,#106180) ;
#92292=AXIS2_PLACEMENT_3D('',#137763,#106181,#106182) ;
#92293=AXIS2_PLACEMENT_3D('',#137764,#106183,#106184) ;
#92294=AXIS2_PLACEMENT_3D('',#137765,#106185,#106186) ;
#92295=AXIS2_PLACEMENT_3D('',#137766,#106187,#106188) ;
#92296=AXIS2_PLACEMENT_3D('',#137767,#106189,#106190) ;
#92297=AXIS2_PLACEMENT_3D('',#137768,#106191,#106192) ;
#92298=AXIS2_PLACEMENT_3D('',#137769,#106193,#106194) ;
#92299=AXIS2_PLACEMENT_3D('',#137770,#106195,#106196) ;
#92300=AXIS2_PLACEMENT_3D('',#137789,#106197,#106198) ;
#92301=AXIS2_PLACEMENT_3D('',#137790,#106199,#106200) ;
#92302=AXIS2_PLACEMENT_3D('',#137791,#106201,#106202) ;
#92303=AXIS2_PLACEMENT_3D('',#137792,#106203,#106204) ;
#92304=AXIS2_PLACEMENT_3D('',#137793,#106205,#106206) ;
#92305=AXIS2_PLACEMENT_3D('',#137794,#106207,#106208) ;
#92306=AXIS2_PLACEMENT_3D('',#137795,#106209,#106210) ;
#92307=AXIS2_PLACEMENT_3D('',#137796,#106211,#106212) ;
#92308=AXIS2_PLACEMENT_3D('',#137797,#106213,#106214) ;
#92309=AXIS2_PLACEMENT_3D('',#137798,#106215,#106216) ;
#92310=AXIS2_PLACEMENT_3D('',#137799,#106217,#106218) ;
#92311=AXIS2_PLACEMENT_3D('',#137812,#106219,#106220) ;
#92312=AXIS2_PLACEMENT_3D('',#137813,#106221,#106222) ;
#92313=AXIS2_PLACEMENT_3D('',#137814,#106223,#106224) ;
#92314=AXIS2_PLACEMENT_3D('',#137815,#106225,#106226) ;
#92315=AXIS2_PLACEMENT_3D('',#137816,#106227,#106228) ;
#92316=AXIS2_PLACEMENT_3D('',#137817,#106229,#106230) ;
#92317=AXIS2_PLACEMENT_3D('',#137818,#106231,#106232) ;
#92318=AXIS2_PLACEMENT_3D('',#137831,#106233,#106234) ;
#92319=AXIS2_PLACEMENT_3D('',#137832,#106235,#106236) ;
#92320=AXIS2_PLACEMENT_3D('',#137833,#106237,#106238) ;
#92321=AXIS2_PLACEMENT_3D('',#137834,#106239,#106240) ;
#92322=AXIS2_PLACEMENT_3D('',#137836,#106241,#106242) ;
#92323=AXIS2_PLACEMENT_3D('',#137856,#106243,#106244) ;
#92324=AXIS2_PLACEMENT_3D('',#137857,#106245,#106246) ;
#92325=AXIS2_PLACEMENT_3D('',#137858,#106247,#106248) ;
#92326=AXIS2_PLACEMENT_3D('',#137859,#106249,#106250) ;
#92327=AXIS2_PLACEMENT_3D('',#137860,#106251,#106252) ;
#92328=AXIS2_PLACEMENT_3D('',#137861,#106253,#106254) ;
#92329=AXIS2_PLACEMENT_3D('',#137890,#106255,#106256) ;
#92330=AXIS2_PLACEMENT_3D('',#137891,#106257,#106258) ;
#92331=AXIS2_PLACEMENT_3D('',#137892,#106259,#106260) ;
#92332=AXIS2_PLACEMENT_3D('',#137893,#106261,#106262) ;
#92333=AXIS2_PLACEMENT_3D('',#137894,#106263,#106264) ;
#92334=AXIS2_PLACEMENT_3D('',#137895,#106265,#106266) ;
#92335=AXIS2_PLACEMENT_3D('',#137896,#106267,#106268) ;
#92336=AXIS2_PLACEMENT_3D('',#137918,#106269,#106270) ;
#92337=AXIS2_PLACEMENT_3D('',#137919,#106271,#106272) ;
#92338=AXIS2_PLACEMENT_3D('',#137920,#106273,#106274) ;
#92339=AXIS2_PLACEMENT_3D('',#137921,#106275,#106276) ;
#92340=AXIS2_PLACEMENT_3D('',#137922,#106277,#106278) ;
#92341=AXIS2_PLACEMENT_3D('',#137923,#106279,#106280) ;
#92342=AXIS2_PLACEMENT_3D('',#137924,#106281,#106282) ;
#92343=AXIS2_PLACEMENT_3D('',#137925,#106283,#106284) ;
#92344=AXIS2_PLACEMENT_3D('',#137926,#106285,#106286) ;
#92345=AXIS2_PLACEMENT_3D('',#137927,#106287,#106288) ;
#92346=AXIS2_PLACEMENT_3D('',#137928,#106289,#106290) ;
#92347=AXIS2_PLACEMENT_3D('',#137929,#106291,#106292) ;
#92348=AXIS2_PLACEMENT_3D('',#137930,#106293,#106294) ;
#92349=AXIS2_PLACEMENT_3D('',#137931,#106295,#106296) ;
#92350=AXIS2_PLACEMENT_3D('',#137932,#106297,#106298) ;
#92351=AXIS2_PLACEMENT_3D('',#137933,#106299,#106300) ;
#92352=AXIS2_PLACEMENT_3D('',#137934,#106301,#106302) ;
#92353=AXIS2_PLACEMENT_3D('',#137935,#106303,#106304) ;
#92354=AXIS2_PLACEMENT_3D('',#137936,#106305,#106306) ;
#92355=AXIS2_PLACEMENT_3D('',#137937,#106307,#106308) ;
#92356=AXIS2_PLACEMENT_3D('',#137938,#106309,#106310) ;
#92357=AXIS2_PLACEMENT_3D('',#137939,#106311,#106312) ;
#92358=AXIS2_PLACEMENT_3D('',#137940,#106313,#106314) ;
#92359=AXIS2_PLACEMENT_3D('',#137941,#106315,#106316) ;
#92360=AXIS2_PLACEMENT_3D('',#137942,#106317,#106318) ;
#92361=AXIS2_PLACEMENT_3D('',#137943,#106319,#106320) ;
#92362=AXIS2_PLACEMENT_3D('',#137944,#106321,#106322) ;
#92363=AXIS2_PLACEMENT_3D('',#137945,#106323,#106324) ;
#92364=AXIS2_PLACEMENT_3D('',#137946,#106325,#106326) ;
#92365=AXIS2_PLACEMENT_3D('',#137947,#106327,#106328) ;
#92366=AXIS2_PLACEMENT_3D('',#137948,#106329,#106330) ;
#92367=AXIS2_PLACEMENT_3D('',#137949,#106331,#106332) ;
#92368=AXIS2_PLACEMENT_3D('',#137950,#106333,#106334) ;
#92369=AXIS2_PLACEMENT_3D('',#137951,#106335,#106336) ;
#92370=AXIS2_PLACEMENT_3D('',#137952,#106337,#106338) ;
#92371=AXIS2_PLACEMENT_3D('',#137953,#106339,#106340) ;
#92372=AXIS2_PLACEMENT_3D('',#137954,#106341,#106342) ;
#92373=AXIS2_PLACEMENT_3D('',#137955,#106343,#106344) ;
#92374=AXIS2_PLACEMENT_3D('',#137956,#106345,#106346) ;
#92375=AXIS2_PLACEMENT_3D('',#137957,#106347,#106348) ;
#92376=AXIS2_PLACEMENT_3D('',#137958,#106349,#106350) ;
#92377=AXIS2_PLACEMENT_3D('',#137959,#106351,#106352) ;
#92378=AXIS2_PLACEMENT_3D('',#137960,#106353,#106354) ;
#92379=AXIS2_PLACEMENT_3D('',#137961,#106355,#106356) ;
#92380=AXIS2_PLACEMENT_3D('',#137962,#106357,#106358) ;
#92381=AXIS2_PLACEMENT_3D('',#137963,#106359,#106360) ;
#92382=AXIS2_PLACEMENT_3D('',#137964,#106361,#106362) ;
#92383=AXIS2_PLACEMENT_3D('',#137965,#106363,#106364) ;
#92384=AXIS2_PLACEMENT_3D('',#137966,#106365,#106366) ;
#92385=AXIS2_PLACEMENT_3D('',#137967,#106367,#106368) ;
#92386=AXIS2_PLACEMENT_3D('',#137968,#106369,#106370) ;
#92387=AXIS2_PLACEMENT_3D('',#137969,#106371,#106372) ;
#92388=AXIS2_PLACEMENT_3D('',#137970,#106373,#106374) ;
#92389=AXIS2_PLACEMENT_3D('',#137971,#106375,#106376) ;
#92390=AXIS2_PLACEMENT_3D('',#137972,#106377,#106378) ;
#92391=AXIS2_PLACEMENT_3D('',#137973,#106379,#106380) ;
#92392=AXIS2_PLACEMENT_3D('',#137974,#106381,#106382) ;
#92393=AXIS2_PLACEMENT_3D('',#137975,#106383,#106384) ;
#92394=AXIS2_PLACEMENT_3D('',#137976,#106385,#106386) ;
#92395=AXIS2_PLACEMENT_3D('',#137977,#106387,#106388) ;
#92396=AXIS2_PLACEMENT_3D('',#137978,#106389,#106390) ;
#92397=AXIS2_PLACEMENT_3D('',#137979,#106391,#106392) ;
#92398=AXIS2_PLACEMENT_3D('',#137980,#106393,#106394) ;
#92399=AXIS2_PLACEMENT_3D('',#137981,#106395,#106396) ;
#92400=AXIS2_PLACEMENT_3D('',#137982,#106397,#106398) ;
#92401=AXIS2_PLACEMENT_3D('',#137983,#106399,#106400) ;
#92402=AXIS2_PLACEMENT_3D('',#137984,#106401,#106402) ;
#92403=AXIS2_PLACEMENT_3D('',#137985,#106403,#106404) ;
#92404=AXIS2_PLACEMENT_3D('',#137986,#106405,#106406) ;
#92405=AXIS2_PLACEMENT_3D('',#137987,#106407,#106408) ;
#92406=AXIS2_PLACEMENT_3D('',#137988,#106409,#106410) ;
#92407=AXIS2_PLACEMENT_3D('',#137989,#106411,#106412) ;
#92408=AXIS2_PLACEMENT_3D('',#137990,#106413,#106414) ;
#92409=AXIS2_PLACEMENT_3D('',#137991,#106415,#106416) ;
#92410=AXIS2_PLACEMENT_3D('',#137992,#106417,#106418) ;
#92411=AXIS2_PLACEMENT_3D('',#137993,#106419,#106420) ;
#92412=AXIS2_PLACEMENT_3D('',#137994,#106421,#106422) ;
#92413=AXIS2_PLACEMENT_3D('',#137995,#106423,#106424) ;
#92414=AXIS2_PLACEMENT_3D('',#137996,#106425,#106426) ;
#92415=AXIS2_PLACEMENT_3D('',#137997,#106427,#106428) ;
#92416=AXIS2_PLACEMENT_3D('',#137998,#106429,#106430) ;
#92417=AXIS2_PLACEMENT_3D('',#137999,#106431,#106432) ;
#92418=AXIS2_PLACEMENT_3D('',#138000,#106433,#106434) ;
#92419=AXIS2_PLACEMENT_3D('',#138001,#106435,#106436) ;
#92420=AXIS2_PLACEMENT_3D('',#138002,#106437,#106438) ;
#92421=AXIS2_PLACEMENT_3D('',#138003,#106439,#106440) ;
#92422=AXIS2_PLACEMENT_3D('',#138004,#106441,#106442) ;
#92423=AXIS2_PLACEMENT_3D('',#138005,#106443,#106444) ;
#92424=AXIS2_PLACEMENT_3D('',#138006,#106445,#106446) ;
#92425=AXIS2_PLACEMENT_3D('',#138007,#106447,#106448) ;
#92426=AXIS2_PLACEMENT_3D('',#138008,#106449,#106450) ;
#92427=AXIS2_PLACEMENT_3D('',#138009,#106451,#106452) ;
#92428=AXIS2_PLACEMENT_3D('',#138010,#106453,#106454) ;
#92429=AXIS2_PLACEMENT_3D('',#138011,#106455,#106456) ;
#92430=AXIS2_PLACEMENT_3D('',#138012,#106457,#106458) ;
#92431=AXIS2_PLACEMENT_3D('',#138013,#106459,#106460) ;
#92432=AXIS2_PLACEMENT_3D('',#138014,#106461,#106462) ;
#92433=AXIS2_PLACEMENT_3D('',#138015,#106463,#106464) ;
#92434=AXIS2_PLACEMENT_3D('',#138016,#106465,#106466) ;
#92435=AXIS2_PLACEMENT_3D('',#138017,#106467,#106468) ;
#92436=AXIS2_PLACEMENT_3D('',#138018,#106469,#106470) ;
#92437=AXIS2_PLACEMENT_3D('',#138019,#106471,#106472) ;
#92438=AXIS2_PLACEMENT_3D('',#138020,#106473,#106474) ;
#92439=AXIS2_PLACEMENT_3D('',#138021,#106475,#106476) ;
#92440=AXIS2_PLACEMENT_3D('',#138022,#106477,#106478) ;
#92441=AXIS2_PLACEMENT_3D('',#138023,#106479,#106480) ;
#92442=AXIS2_PLACEMENT_3D('',#138024,#106481,#106482) ;
#92443=AXIS2_PLACEMENT_3D('',#138025,#106483,#106484) ;
#92444=AXIS2_PLACEMENT_3D('',#138026,#106485,#106486) ;
#92445=AXIS2_PLACEMENT_3D('',#138039,#106487,#106488) ;
#92446=AXIS2_PLACEMENT_3D('',#138040,#106489,#106490) ;
#92447=AXIS2_PLACEMENT_3D('',#138041,#106491,#106492) ;
#92448=AXIS2_PLACEMENT_3D('',#138042,#106493,#106494) ;
#92449=AXIS2_PLACEMENT_3D('',#138043,#106495,#106496) ;
#92450=AXIS2_PLACEMENT_3D('',#138044,#106497,#106498) ;
#92451=AXIS2_PLACEMENT_3D('',#138045,#106499,#106500) ;
#92452=AXIS2_PLACEMENT_3D('',#138046,#106501,#106502) ;
#92453=AXIS2_PLACEMENT_3D('',#138047,#106503,#106504) ;
#92454=AXIS2_PLACEMENT_3D('',#138048,#106505,#106506) ;
#92455=AXIS2_PLACEMENT_3D('',#138049,#106507,#106508) ;
#92456=AXIS2_PLACEMENT_3D('',#138050,#106509,#106510) ;
#92457=AXIS2_PLACEMENT_3D('',#138051,#106511,#106512) ;
#92458=AXIS2_PLACEMENT_3D('',#138052,#106513,#106514) ;
#92459=AXIS2_PLACEMENT_3D('',#138053,#106515,#106516) ;
#92460=AXIS2_PLACEMENT_3D('',#138054,#106517,#106518) ;
#92461=AXIS2_PLACEMENT_3D('',#138055,#106519,#106520) ;
#92462=AXIS2_PLACEMENT_3D('',#138056,#106521,#106522) ;
#92463=AXIS2_PLACEMENT_3D('',#138057,#106523,#106524) ;
#92464=AXIS2_PLACEMENT_3D('',#138058,#106525,#106526) ;
#92465=AXIS2_PLACEMENT_3D('',#138059,#106527,#106528) ;
#92466=AXIS2_PLACEMENT_3D('',#138060,#106529,#106530) ;
#92467=AXIS2_PLACEMENT_3D('',#138061,#106531,#106532) ;
#92468=AXIS2_PLACEMENT_3D('',#138062,#106533,#106534) ;
#92469=AXIS2_PLACEMENT_3D('',#138063,#106535,#106536) ;
#92470=AXIS2_PLACEMENT_3D('',#138064,#106537,#106538) ;
#92471=AXIS2_PLACEMENT_3D('',#138077,#106539,#106540) ;
#92472=AXIS2_PLACEMENT_3D('',#138078,#106541,#106542) ;
#92473=AXIS2_PLACEMENT_3D('',#138079,#106543,#106544) ;
#92474=AXIS2_PLACEMENT_3D('',#138080,#106545,#106546) ;
#92475=AXIS2_PLACEMENT_3D('',#138081,#106547,#106548) ;
#92476=AXIS2_PLACEMENT_3D('',#138082,#106549,#106550) ;
#92477=AXIS2_PLACEMENT_3D('',#138083,#106551,#106552) ;
#92478=AXIS2_PLACEMENT_3D('',#138084,#106553,#106554) ;
#92479=AXIS2_PLACEMENT_3D('',#138085,#106555,#106556) ;
#92480=AXIS2_PLACEMENT_3D('',#138086,#106557,#106558) ;
#92481=AXIS2_PLACEMENT_3D('',#138087,#106559,#106560) ;
#92482=AXIS2_PLACEMENT_3D('',#138088,#106561,#106562) ;
#92483=AXIS2_PLACEMENT_3D('',#138089,#106563,#106564) ;
#92484=AXIS2_PLACEMENT_3D('',#138090,#106565,#106566) ;
#92485=AXIS2_PLACEMENT_3D('',#138091,#106567,#106568) ;
#92486=AXIS2_PLACEMENT_3D('',#138092,#106569,#106570) ;
#92487=AXIS2_PLACEMENT_3D('',#138093,#106571,#106572) ;
#92488=AXIS2_PLACEMENT_3D('',#138094,#106573,#106574) ;
#92489=AXIS2_PLACEMENT_3D('',#138095,#106575,#106576) ;
#92490=AXIS2_PLACEMENT_3D('',#138096,#106577,#106578) ;
#92491=AXIS2_PLACEMENT_3D('',#138097,#106579,#106580) ;
#92492=AXIS2_PLACEMENT_3D('',#138098,#106581,#106582) ;
#92493=AXIS2_PLACEMENT_3D('',#138099,#106583,#106584) ;
#92494=AXIS2_PLACEMENT_3D('',#138100,#106585,#106586) ;
#92495=AXIS2_PLACEMENT_3D('',#138101,#106587,#106588) ;
#92496=AXIS2_PLACEMENT_3D('',#138102,#106589,#106590) ;
#92497=AXIS2_PLACEMENT_3D('',#138103,#106591,#106592) ;
#92498=AXIS2_PLACEMENT_3D('',#138104,#106593,#106594) ;
#92499=AXIS2_PLACEMENT_3D('',#138117,#106595,#106596) ;
#92500=AXIS2_PLACEMENT_3D('',#138130,#106597,#106598) ;
#92501=AXIS2_PLACEMENT_3D('',#138131,#106599,#106600) ;
#92502=AXIS2_PLACEMENT_3D('',#138132,#106601,#106602) ;
#92503=AXIS2_PLACEMENT_3D('',#138133,#106603,#106604) ;
#92504=AXIS2_PLACEMENT_3D('',#138134,#106605,#106606) ;
#92505=AXIS2_PLACEMENT_3D('',#138147,#106607,#106608) ;
#92506=AXIS2_PLACEMENT_3D('',#138160,#106609,#106610) ;
#92507=AXIS2_PLACEMENT_3D('',#138161,#106611,#106612) ;
#92508=AXIS2_PLACEMENT_3D('',#138162,#106613,#106614) ;
#92509=AXIS2_PLACEMENT_3D('',#138163,#106615,#106616) ;
#92510=AXIS2_PLACEMENT_3D('',#138241,#106617,#106618) ;
#92511=AXIS2_PLACEMENT_3D('',#138242,#106619,#106620) ;
#92512=AXIS2_PLACEMENT_3D('',#138243,#106621,#106622) ;
#92513=AXIS2_PLACEMENT_3D('',#138312,#106623,#106624) ;
#92514=AXIS2_PLACEMENT_3D('',#138313,#106625,#106626) ;
#92515=AXIS2_PLACEMENT_3D('',#138428,#106627,#106628) ;
#92516=AXIS2_PLACEMENT_3D('',#138459,#106629,#106630) ;
#92517=AXIS2_PLACEMENT_3D('',#138490,#106631,#106632) ;
#92518=AXIS2_PLACEMENT_3D('',#138539,#106633,#106634) ;
#92519=AXIS2_PLACEMENT_3D('',#138540,#106635,#106636) ;
#92520=AXIS2_PLACEMENT_3D('',#138549,#106641,#106642) ;
#92521=AXIS2_PLACEMENT_3D('',#138551,#106643,#106644) ;
#92522=AXIS2_PLACEMENT_3D('',#138554,#106646,#106647) ;
#92523=AXIS2_PLACEMENT_3D('',#138555,#106648,#106649) ;
#92524=AXIS2_PLACEMENT_3D('',#138561,#106653,#106654) ;
#92525=AXIS2_PLACEMENT_3D('',#138563,#106655,#106656) ;
#92526=AXIS2_PLACEMENT_3D('',#138566,#106658,#106659) ;
#92527=AXIS2_PLACEMENT_3D('',#138567,#106660,#106661) ;
#92528=AXIS2_PLACEMENT_3D('',#138573,#106665,#106666) ;
#92529=AXIS2_PLACEMENT_3D('',#138575,#106667,#106668) ;
#92530=AXIS2_PLACEMENT_3D('',#138578,#106670,#106671) ;
#92531=AXIS2_PLACEMENT_3D('',#138579,#106672,#106673) ;
#92532=AXIS2_PLACEMENT_3D('',#138585,#106677,#106678) ;
#92533=AXIS2_PLACEMENT_3D('',#138587,#106679,#106680) ;
#92534=AXIS2_PLACEMENT_3D('',#138590,#106682,#106683) ;
#92535=AXIS2_PLACEMENT_3D('',#138591,#106684,#106685) ;
#92536=AXIS2_PLACEMENT_3D('',#138597,#106689,#106690) ;
#92537=AXIS2_PLACEMENT_3D('',#138600,#106691,#106692) ;
#92538=AXIS2_PLACEMENT_3D('',#138612,#106699,#106700) ;
#92539=AXIS2_PLACEMENT_3D('',#138623,#106705,#106706) ;
#92540=AXIS2_PLACEMENT_3D('',#138627,#106709,#106710) ;
#92541=AXIS2_PLACEMENT_3D('',#138636,#106715,#106716) ;
#92542=AXIS2_PLACEMENT_3D('',#138638,#106718,#106719) ;
#92543=AXIS2_PLACEMENT_3D('',#138646,#106724,#106725) ;
#92544=AXIS2_PLACEMENT_3D('',#138653,#106728,#106729) ;
#92545=AXIS2_PLACEMENT_3D('',#138655,#106731,#106732) ;
#92546=AXIS2_PLACEMENT_3D('',#138656,#106733,#106734) ;
#92547=AXIS2_PLACEMENT_3D('',#138657,#106735,#106736) ;
#92548=AXIS2_PLACEMENT_3D('',#138658,#106737,#106738) ;
#92549=AXIS2_PLACEMENT_3D('',#138659,#106739,#106740) ;
#92550=AXIS2_PLACEMENT_3D('',#138660,#106741,#106742) ;
#92551=AXIS2_PLACEMENT_3D('',#138661,#106743,#106744) ;
#92552=AXIS2_PLACEMENT_3D('',#138670,#106749,#106750) ;
#92553=AXIS2_PLACEMENT_3D('',#138679,#106755,#106756) ;
#92554=AXIS2_PLACEMENT_3D('',#138682,#106757,#106758) ;
#92555=AXIS2_PLACEMENT_3D('',#138690,#106762,#106763) ;
#92556=AXIS2_PLACEMENT_3D('',#138696,#106767,#106768) ;
#92557=AXIS2_PLACEMENT_3D('',#138701,#106770,#106771) ;
#92558=AXIS2_PLACEMENT_3D('',#138704,#106773,#106774) ;
#92559=AXIS2_PLACEMENT_3D('',#138706,#106775,#106776) ;
#92560=AXIS2_PLACEMENT_3D('',#138709,#106778,#106779) ;
#92561=AXIS2_PLACEMENT_3D('',#138710,#106780,#106781) ;
#92562=AXIS2_PLACEMENT_3D('',#138713,#106782,#106783) ;
#92563=AXIS2_PLACEMENT_3D('',#138718,#106786,#106787) ;
#92564=AXIS2_PLACEMENT_3D('',#138724,#106791,#106792) ;
#92565=AXIS2_PLACEMENT_3D('',#138730,#106796,#106797) ;
#92566=AXIS2_PLACEMENT_3D('',#138736,#106801,#106802) ;
#92567=AXIS2_PLACEMENT_3D('',#138749,#106809,#106810) ;
#92568=AXIS2_PLACEMENT_3D('',#138762,#106817,#106818) ;
#92569=AXIS2_PLACEMENT_3D('',#138771,#106823,#106824) ;
#92570=AXIS2_PLACEMENT_3D('',#138780,#106829,#106830) ;
#92571=AXIS2_PLACEMENT_3D('',#138789,#106835,#106836) ;
#92572=AXIS2_PLACEMENT_3D('',#138798,#106841,#106842) ;
#92573=AXIS2_PLACEMENT_3D('',#138811,#106848,#106849) ;
#92574=AXIS2_PLACEMENT_3D('',#138815,#106851,#106852) ;
#92575=AXIS2_PLACEMENT_3D('',#138819,#106854,#106855) ;
#92576=AXIS2_PLACEMENT_3D('',#138822,#106857,#106858) ;
#92577=AXIS2_PLACEMENT_3D('',#138823,#106859,#106860) ;
#92578=AXIS2_PLACEMENT_3D('',#138826,#106861,#106862) ;
#92579=AXIS2_PLACEMENT_3D('',#138829,#106865,#106866) ;
#92580=AXIS2_PLACEMENT_3D('',#138833,#106869,#106870) ;
#92581=AXIS2_PLACEMENT_3D('',#138835,#106871,#106872) ;
#92582=AXIS2_PLACEMENT_3D('',#138837,#106874,#106875) ;
#92583=AXIS2_PLACEMENT_3D('',#138841,#106878,#106879) ;
#92584=AXIS2_PLACEMENT_3D('',#138843,#106880,#106881) ;
#92585=AXIS2_PLACEMENT_3D('',#138845,#106883,#106884) ;
#92586=AXIS2_PLACEMENT_3D('',#138849,#106887,#106888) ;
#92587=AXIS2_PLACEMENT_3D('',#138851,#106889,#106890) ;
#92588=AXIS2_PLACEMENT_3D('',#138853,#106892,#106893) ;
#92589=AXIS2_PLACEMENT_3D('',#138855,#106895,#106896) ;
#92590=AXIS2_PLACEMENT_3D('',#138856,#106897,#106898) ;
#92591=AXIS2_PLACEMENT_3D('',#138858,#106900,#106901) ;
#92592=AXIS2_PLACEMENT_3D('',#138861,#106904,#106905) ;
#92593=AXIS2_PLACEMENT_3D('',#138864,#106908,#106909) ;
#92594=AXIS2_PLACEMENT_3D('',#138867,#106912,#106913) ;
#92595=AXIS2_PLACEMENT_3D('',#138876,#106918,#106919) ;
#92596=AXIS2_PLACEMENT_3D('',#138885,#106924,#106925) ;
#92597=AXIS2_PLACEMENT_3D('',#138894,#106930,#106931) ;
#92598=AXIS2_PLACEMENT_3D('',#138903,#106936,#106937) ;
#92599=AXIS2_PLACEMENT_3D('',#138916,#106943,#106944) ;
#92600=AXIS2_PLACEMENT_3D('',#138920,#106946,#106947) ;
#92601=AXIS2_PLACEMENT_3D('',#138924,#106949,#106950) ;
#92602=AXIS2_PLACEMENT_3D('',#138927,#106952,#106953) ;
#92603=AXIS2_PLACEMENT_3D('',#138928,#106954,#106955) ;
#92604=AXIS2_PLACEMENT_3D('',#138932,#106957,#106958) ;
#92605=AXIS2_PLACEMENT_3D('',#138934,#106960,#106961) ;
#92606=AXIS2_PLACEMENT_3D('',#138938,#106964,#106965) ;
#92607=AXIS2_PLACEMENT_3D('',#138940,#106966,#106967) ;
#92608=AXIS2_PLACEMENT_3D('',#138942,#106969,#106970) ;
#92609=AXIS2_PLACEMENT_3D('',#138946,#106973,#106974) ;
#92610=AXIS2_PLACEMENT_3D('',#138948,#106975,#106976) ;
#92611=AXIS2_PLACEMENT_3D('',#138950,#106978,#106979) ;
#92612=AXIS2_PLACEMENT_3D('',#138954,#106982,#106983) ;
#92613=AXIS2_PLACEMENT_3D('',#138956,#106984,#106985) ;
#92614=AXIS2_PLACEMENT_3D('',#138958,#106987,#106988) ;
#92615=AXIS2_PLACEMENT_3D('',#138960,#106990,#106991) ;
#92616=AXIS2_PLACEMENT_3D('',#138969,#106996,#106997) ;
#92617=AXIS2_PLACEMENT_3D('',#138976,#107002,#107003) ;
#92618=AXIS2_PLACEMENT_3D('',#138982,#107007,#107008) ;
#92619=AXIS2_PLACEMENT_3D('',#138987,#107012,#107013) ;
#92620=AXIS2_PLACEMENT_3D('',#138991,#107015,#107016) ;
#92621=AXIS2_PLACEMENT_3D('',#138997,#107020,#107021) ;
#92622=AXIS2_PLACEMENT_3D('',#138998,#107022,#107023) ;
#92623=AXIS2_PLACEMENT_3D('',#139001,#107024,#107025) ;
#92624=AXIS2_PLACEMENT_3D('',#139003,#107026,#107027) ;
#92625=AXIS2_PLACEMENT_3D('',#139005,#107028,#107029) ;
#92626=AXIS2_PLACEMENT_3D('',#139009,#107031,#107032) ;
#92627=AXIS2_PLACEMENT_3D('',#139029,#107034,#107035) ;
#92628=AXIS2_PLACEMENT_3D('',#139036,#107036,#107037) ;
#92629=AXIS2_PLACEMENT_3D('',#139037,#107038,#107039) ;
#92630=AXIS2_PLACEMENT_3D('',#139038,#107040,#107041) ;
#92631=AXIS2_PLACEMENT_3D('',#139051,#107042,#107043) ;
#92632=AXIS2_PLACEMENT_3D('',#139052,#107044,#107045) ;
#92633=AXIS2_PLACEMENT_3D('',#139053,#107046,#107047) ;
#92634=AXIS2_PLACEMENT_3D('',#139054,#107048,#107049) ;
#92635=AXIS2_PLACEMENT_3D('',#139055,#107050,#107051) ;
#92636=AXIS2_PLACEMENT_3D('',#139056,#107052,#107053) ;
#92637=AXIS2_PLACEMENT_3D('',#139057,#107054,#107055) ;
#92638=AXIS2_PLACEMENT_3D('',#139058,#107056,#107057) ;
#92639=AXIS2_PLACEMENT_3D('',#139059,#107058,#107059) ;
#92640=AXIS2_PLACEMENT_3D('',#139060,#107060,#107061) ;
#92641=AXIS2_PLACEMENT_3D('',#139061,#107062,#107063) ;
#92642=AXIS2_PLACEMENT_3D('',#139062,#107064,#107065) ;
#92643=AXIS2_PLACEMENT_3D('',#139063,#107066,#107067) ;
#92644=AXIS2_PLACEMENT_3D('',#139064,#107068,#107069) ;
#92645=AXIS2_PLACEMENT_3D('',#139065,#107070,#107071) ;
#92646=AXIS2_PLACEMENT_3D('',#139066,#107072,#107073) ;
#92647=AXIS2_PLACEMENT_3D('',#139085,#107074,#107075) ;
#92648=AXIS2_PLACEMENT_3D('',#139086,#107076,#107077) ;
#92649=AXIS2_PLACEMENT_3D('',#139105,#107078,#107079) ;
#92650=AXIS2_PLACEMENT_3D('',#139124,#107080,#107081) ;
#92651=AXIS2_PLACEMENT_3D('',#139125,#107082,#107083) ;
#92652=AXIS2_PLACEMENT_3D('',#139126,#107084,#107085) ;
#92653=AXIS2_PLACEMENT_3D('',#139127,#107086,#107087) ;
#92654=AXIS2_PLACEMENT_3D('',#139128,#107088,#107089) ;
#92655=AXIS2_PLACEMENT_3D('',#139129,#107090,#107091) ;
#92656=AXIS2_PLACEMENT_3D('',#139130,#107092,#107093) ;
#92657=AXIS2_PLACEMENT_3D('',#139131,#107094,#107095) ;
#92658=AXIS2_PLACEMENT_3D('',#139132,#107096,#107097) ;
#92659=AXIS2_PLACEMENT_3D('',#139133,#107098,#107099) ;
#92660=AXIS2_PLACEMENT_3D('',#139134,#107100,#107101) ;
#92661=AXIS2_PLACEMENT_3D('',#139135,#107102,#107103) ;
#92662=AXIS2_PLACEMENT_3D('',#139136,#107104,#107105) ;
#92663=AXIS2_PLACEMENT_3D('',#139137,#107106,#107107) ;
#92664=AXIS2_PLACEMENT_3D('',#139138,#107108,#107109) ;
#92665=AXIS2_PLACEMENT_3D('',#139157,#107110,#107111) ;
#92666=AXIS2_PLACEMENT_3D('',#139158,#107112,#107113) ;
#92667=AXIS2_PLACEMENT_3D('',#139159,#107114,#107115) ;
#92668=AXIS2_PLACEMENT_3D('',#139160,#107116,#107117) ;
#92669=AXIS2_PLACEMENT_3D('',#139161,#107118,#107119) ;
#92670=AXIS2_PLACEMENT_3D('',#139162,#107120,#107121) ;
#92671=AXIS2_PLACEMENT_3D('',#139163,#107122,#107123) ;
#92672=AXIS2_PLACEMENT_3D('',#139164,#107124,#107125) ;
#92673=AXIS2_PLACEMENT_3D('',#139165,#107126,#107127) ;
#92674=AXIS2_PLACEMENT_3D('',#139166,#107128,#107129) ;
#92675=AXIS2_PLACEMENT_3D('',#139167,#107130,#107131) ;
#92676=AXIS2_PLACEMENT_3D('',#139180,#107132,#107133) ;
#92677=AXIS2_PLACEMENT_3D('',#139181,#107134,#107135) ;
#92678=AXIS2_PLACEMENT_3D('',#139182,#107136,#107137) ;
#92679=AXIS2_PLACEMENT_3D('',#139183,#107138,#107139) ;
#92680=AXIS2_PLACEMENT_3D('',#139184,#107140,#107141) ;
#92681=AXIS2_PLACEMENT_3D('',#139185,#107142,#107143) ;
#92682=AXIS2_PLACEMENT_3D('',#139186,#107144,#107145) ;
#92683=AXIS2_PLACEMENT_3D('',#139199,#107146,#107147) ;
#92684=AXIS2_PLACEMENT_3D('',#139200,#107148,#107149) ;
#92685=AXIS2_PLACEMENT_3D('',#139201,#107150,#107151) ;
#92686=AXIS2_PLACEMENT_3D('',#139203,#107152,#107153) ;
#92687=AXIS2_PLACEMENT_3D('',#139223,#107154,#107155) ;
#92688=AXIS2_PLACEMENT_3D('',#139224,#107156,#107157) ;
#92689=AXIS2_PLACEMENT_3D('',#139225,#107158,#107159) ;
#92690=AXIS2_PLACEMENT_3D('',#139226,#107160,#107161) ;
#92691=AXIS2_PLACEMENT_3D('',#139227,#107162,#107163) ;
#92692=AXIS2_PLACEMENT_3D('',#139228,#107164,#107165) ;
#92693=AXIS2_PLACEMENT_3D('',#139257,#107166,#107167) ;
#92694=AXIS2_PLACEMENT_3D('',#139258,#107168,#107169) ;
#92695=AXIS2_PLACEMENT_3D('',#139259,#107170,#107171) ;
#92696=AXIS2_PLACEMENT_3D('',#139260,#107172,#107173) ;
#92697=AXIS2_PLACEMENT_3D('',#139261,#107174,#107175) ;
#92698=AXIS2_PLACEMENT_3D('',#139262,#107176,#107177) ;
#92699=AXIS2_PLACEMENT_3D('',#139263,#107178,#107179) ;
#92700=AXIS2_PLACEMENT_3D('',#139285,#107180,#107181) ;
#92701=AXIS2_PLACEMENT_3D('',#139286,#107182,#107183) ;
#92702=AXIS2_PLACEMENT_3D('',#139287,#107184,#107185) ;
#92703=AXIS2_PLACEMENT_3D('',#139288,#107186,#107187) ;
#92704=AXIS2_PLACEMENT_3D('',#139289,#107188,#107189) ;
#92705=AXIS2_PLACEMENT_3D('',#139290,#107190,#107191) ;
#92706=AXIS2_PLACEMENT_3D('',#139291,#107192,#107193) ;
#92707=AXIS2_PLACEMENT_3D('',#139292,#107194,#107195) ;
#92708=AXIS2_PLACEMENT_3D('',#139293,#107196,#107197) ;
#92709=AXIS2_PLACEMENT_3D('',#139294,#107198,#107199) ;
#92710=AXIS2_PLACEMENT_3D('',#139295,#107200,#107201) ;
#92711=AXIS2_PLACEMENT_3D('',#139296,#107202,#107203) ;
#92712=AXIS2_PLACEMENT_3D('',#139297,#107204,#107205) ;
#92713=AXIS2_PLACEMENT_3D('',#139298,#107206,#107207) ;
#92714=AXIS2_PLACEMENT_3D('',#139299,#107208,#107209) ;
#92715=AXIS2_PLACEMENT_3D('',#139300,#107210,#107211) ;
#92716=AXIS2_PLACEMENT_3D('',#139301,#107212,#107213) ;
#92717=AXIS2_PLACEMENT_3D('',#139302,#107214,#107215) ;
#92718=AXIS2_PLACEMENT_3D('',#139303,#107216,#107217) ;
#92719=AXIS2_PLACEMENT_3D('',#139304,#107218,#107219) ;
#92720=AXIS2_PLACEMENT_3D('',#139305,#107220,#107221) ;
#92721=AXIS2_PLACEMENT_3D('',#139306,#107222,#107223) ;
#92722=AXIS2_PLACEMENT_3D('',#139307,#107224,#107225) ;
#92723=AXIS2_PLACEMENT_3D('',#139308,#107226,#107227) ;
#92724=AXIS2_PLACEMENT_3D('',#139309,#107228,#107229) ;
#92725=AXIS2_PLACEMENT_3D('',#139310,#107230,#107231) ;
#92726=AXIS2_PLACEMENT_3D('',#139311,#107232,#107233) ;
#92727=AXIS2_PLACEMENT_3D('',#139312,#107234,#107235) ;
#92728=AXIS2_PLACEMENT_3D('',#139313,#107236,#107237) ;
#92729=AXIS2_PLACEMENT_3D('',#139314,#107238,#107239) ;
#92730=AXIS2_PLACEMENT_3D('',#139315,#107240,#107241) ;
#92731=AXIS2_PLACEMENT_3D('',#139316,#107242,#107243) ;
#92732=AXIS2_PLACEMENT_3D('',#139317,#107244,#107245) ;
#92733=AXIS2_PLACEMENT_3D('',#139318,#107246,#107247) ;
#92734=AXIS2_PLACEMENT_3D('',#139319,#107248,#107249) ;
#92735=AXIS2_PLACEMENT_3D('',#139320,#107250,#107251) ;
#92736=AXIS2_PLACEMENT_3D('',#139321,#107252,#107253) ;
#92737=AXIS2_PLACEMENT_3D('',#139322,#107254,#107255) ;
#92738=AXIS2_PLACEMENT_3D('',#139323,#107256,#107257) ;
#92739=AXIS2_PLACEMENT_3D('',#139324,#107258,#107259) ;
#92740=AXIS2_PLACEMENT_3D('',#139325,#107260,#107261) ;
#92741=AXIS2_PLACEMENT_3D('',#139326,#107262,#107263) ;
#92742=AXIS2_PLACEMENT_3D('',#139327,#107264,#107265) ;
#92743=AXIS2_PLACEMENT_3D('',#139328,#107266,#107267) ;
#92744=AXIS2_PLACEMENT_3D('',#139329,#107268,#107269) ;
#92745=AXIS2_PLACEMENT_3D('',#139330,#107270,#107271) ;
#92746=AXIS2_PLACEMENT_3D('',#139331,#107272,#107273) ;
#92747=AXIS2_PLACEMENT_3D('',#139332,#107274,#107275) ;
#92748=AXIS2_PLACEMENT_3D('',#139333,#107276,#107277) ;
#92749=AXIS2_PLACEMENT_3D('',#139334,#107278,#107279) ;
#92750=AXIS2_PLACEMENT_3D('',#139335,#107280,#107281) ;
#92751=AXIS2_PLACEMENT_3D('',#139336,#107282,#107283) ;
#92752=AXIS2_PLACEMENT_3D('',#139337,#107284,#107285) ;
#92753=AXIS2_PLACEMENT_3D('',#139338,#107286,#107287) ;
#92754=AXIS2_PLACEMENT_3D('',#139339,#107288,#107289) ;
#92755=AXIS2_PLACEMENT_3D('',#139340,#107290,#107291) ;
#92756=AXIS2_PLACEMENT_3D('',#139341,#107292,#107293) ;
#92757=AXIS2_PLACEMENT_3D('',#139342,#107294,#107295) ;
#92758=AXIS2_PLACEMENT_3D('',#139343,#107296,#107297) ;
#92759=AXIS2_PLACEMENT_3D('',#139344,#107298,#107299) ;
#92760=AXIS2_PLACEMENT_3D('',#139345,#107300,#107301) ;
#92761=AXIS2_PLACEMENT_3D('',#139346,#107302,#107303) ;
#92762=AXIS2_PLACEMENT_3D('',#139347,#107304,#107305) ;
#92763=AXIS2_PLACEMENT_3D('',#139348,#107306,#107307) ;
#92764=AXIS2_PLACEMENT_3D('',#139349,#107308,#107309) ;
#92765=AXIS2_PLACEMENT_3D('',#139350,#107310,#107311) ;
#92766=AXIS2_PLACEMENT_3D('',#139351,#107312,#107313) ;
#92767=AXIS2_PLACEMENT_3D('',#139352,#107314,#107315) ;
#92768=AXIS2_PLACEMENT_3D('',#139353,#107316,#107317) ;
#92769=AXIS2_PLACEMENT_3D('',#139354,#107318,#107319) ;
#92770=AXIS2_PLACEMENT_3D('',#139355,#107320,#107321) ;
#92771=AXIS2_PLACEMENT_3D('',#139356,#107322,#107323) ;
#92772=AXIS2_PLACEMENT_3D('',#139357,#107324,#107325) ;
#92773=AXIS2_PLACEMENT_3D('',#139358,#107326,#107327) ;
#92774=AXIS2_PLACEMENT_3D('',#139359,#107328,#107329) ;
#92775=AXIS2_PLACEMENT_3D('',#139360,#107330,#107331) ;
#92776=AXIS2_PLACEMENT_3D('',#139361,#107332,#107333) ;
#92777=AXIS2_PLACEMENT_3D('',#139362,#107334,#107335) ;
#92778=AXIS2_PLACEMENT_3D('',#139363,#107336,#107337) ;
#92779=AXIS2_PLACEMENT_3D('',#139364,#107338,#107339) ;
#92780=AXIS2_PLACEMENT_3D('',#139365,#107340,#107341) ;
#92781=AXIS2_PLACEMENT_3D('',#139366,#107342,#107343) ;
#92782=AXIS2_PLACEMENT_3D('',#139367,#107344,#107345) ;
#92783=AXIS2_PLACEMENT_3D('',#139368,#107346,#107347) ;
#92784=AXIS2_PLACEMENT_3D('',#139369,#107348,#107349) ;
#92785=AXIS2_PLACEMENT_3D('',#139370,#107350,#107351) ;
#92786=AXIS2_PLACEMENT_3D('',#139371,#107352,#107353) ;
#92787=AXIS2_PLACEMENT_3D('',#139372,#107354,#107355) ;
#92788=AXIS2_PLACEMENT_3D('',#139373,#107356,#107357) ;
#92789=AXIS2_PLACEMENT_3D('',#139374,#107358,#107359) ;
#92790=AXIS2_PLACEMENT_3D('',#139375,#107360,#107361) ;
#92791=AXIS2_PLACEMENT_3D('',#139376,#107362,#107363) ;
#92792=AXIS2_PLACEMENT_3D('',#139377,#107364,#107365) ;
#92793=AXIS2_PLACEMENT_3D('',#139378,#107366,#107367) ;
#92794=AXIS2_PLACEMENT_3D('',#139379,#107368,#107369) ;
#92795=AXIS2_PLACEMENT_3D('',#139380,#107370,#107371) ;
#92796=AXIS2_PLACEMENT_3D('',#139381,#107372,#107373) ;
#92797=AXIS2_PLACEMENT_3D('',#139382,#107374,#107375) ;
#92798=AXIS2_PLACEMENT_3D('',#139383,#107376,#107377) ;
#92799=AXIS2_PLACEMENT_3D('',#139384,#107378,#107379) ;
#92800=AXIS2_PLACEMENT_3D('',#139385,#107380,#107381) ;
#92801=AXIS2_PLACEMENT_3D('',#139386,#107382,#107383) ;
#92802=AXIS2_PLACEMENT_3D('',#139387,#107384,#107385) ;
#92803=AXIS2_PLACEMENT_3D('',#139388,#107386,#107387) ;
#92804=AXIS2_PLACEMENT_3D('',#139389,#107388,#107389) ;
#92805=AXIS2_PLACEMENT_3D('',#139390,#107390,#107391) ;
#92806=AXIS2_PLACEMENT_3D('',#139391,#107392,#107393) ;
#92807=AXIS2_PLACEMENT_3D('',#139392,#107394,#107395) ;
#92808=AXIS2_PLACEMENT_3D('',#139393,#107396,#107397) ;
#92809=AXIS2_PLACEMENT_3D('',#139406,#107398,#107399) ;
#92810=AXIS2_PLACEMENT_3D('',#139407,#107400,#107401) ;
#92811=AXIS2_PLACEMENT_3D('',#139408,#107402,#107403) ;
#92812=AXIS2_PLACEMENT_3D('',#139409,#107404,#107405) ;
#92813=AXIS2_PLACEMENT_3D('',#139410,#107406,#107407) ;
#92814=AXIS2_PLACEMENT_3D('',#139411,#107408,#107409) ;
#92815=AXIS2_PLACEMENT_3D('',#139412,#107410,#107411) ;
#92816=AXIS2_PLACEMENT_3D('',#139413,#107412,#107413) ;
#92817=AXIS2_PLACEMENT_3D('',#139414,#107414,#107415) ;
#92818=AXIS2_PLACEMENT_3D('',#139415,#107416,#107417) ;
#92819=AXIS2_PLACEMENT_3D('',#139416,#107418,#107419) ;
#92820=AXIS2_PLACEMENT_3D('',#139417,#107420,#107421) ;
#92821=AXIS2_PLACEMENT_3D('',#139418,#107422,#107423) ;
#92822=AXIS2_PLACEMENT_3D('',#139419,#107424,#107425) ;
#92823=AXIS2_PLACEMENT_3D('',#139420,#107426,#107427) ;
#92824=AXIS2_PLACEMENT_3D('',#139421,#107428,#107429) ;
#92825=AXIS2_PLACEMENT_3D('',#139422,#107430,#107431) ;
#92826=AXIS2_PLACEMENT_3D('',#139423,#107432,#107433) ;
#92827=AXIS2_PLACEMENT_3D('',#139424,#107434,#107435) ;
#92828=AXIS2_PLACEMENT_3D('',#139425,#107436,#107437) ;
#92829=AXIS2_PLACEMENT_3D('',#139438,#107438,#107439) ;
#92830=AXIS2_PLACEMENT_3D('',#139439,#107440,#107441) ;
#92831=AXIS2_PLACEMENT_3D('',#139440,#107442,#107443) ;
#92832=AXIS2_PLACEMENT_3D('',#139441,#107444,#107445) ;
#92833=AXIS2_PLACEMENT_3D('',#139442,#107446,#107447) ;
#92834=AXIS2_PLACEMENT_3D('',#139443,#107448,#107449) ;
#92835=AXIS2_PLACEMENT_3D('',#139444,#107450,#107451) ;
#92836=AXIS2_PLACEMENT_3D('',#139445,#107452,#107453) ;
#92837=AXIS2_PLACEMENT_3D('',#139446,#107454,#107455) ;
#92838=AXIS2_PLACEMENT_3D('',#139447,#107456,#107457) ;
#92839=AXIS2_PLACEMENT_3D('',#139460,#107458,#107459) ;
#92840=AXIS2_PLACEMENT_3D('',#139473,#107460,#107461) ;
#92841=AXIS2_PLACEMENT_3D('',#139474,#107462,#107463) ;
#92842=AXIS2_PLACEMENT_3D('',#139487,#107464,#107465) ;
#92843=AXIS2_PLACEMENT_3D('',#139500,#107466,#107467) ;
#92844=AXIS2_PLACEMENT_3D('',#139501,#107468,#107469) ;
#92845=AXIS2_PLACEMENT_3D('',#139502,#107470,#107471) ;
#92846=AXIS2_PLACEMENT_3D('',#139503,#107472,#107473) ;
#92847=AXIS2_PLACEMENT_3D('',#139581,#107474,#107475) ;
#92848=AXIS2_PLACEMENT_3D('',#139582,#107476,#107477) ;
#92849=AXIS2_PLACEMENT_3D('',#139765,#107478,#107479) ;
#92850=AXIS2_PLACEMENT_3D('',#139796,#107480,#107481) ;
#92851=AXIS2_PLACEMENT_3D('',#139827,#107482,#107483) ;
#92852=AXIS2_PLACEMENT_3D('',#139876,#107484,#107485) ;
#92853=AXIS2_PLACEMENT_3D('',#139877,#107486,#107487) ;
#92854=AXIS2_PLACEMENT_3D('',#139878,#107488,#107489) ;
#92855=AXIS2_PLACEMENT_3D('',#139879,#107490,#107491) ;
#92856=AXIS2_PLACEMENT_3D('',#139880,#107492,#107493) ;
#92857=AXIS2_PLACEMENT_3D('',#139881,#107494,#107495) ;
#92858=AXIS2_PLACEMENT_3D('',#139882,#107496,#107497) ;
#92859=AXIS2_PLACEMENT_3D('',#139883,#107498,#107499) ;
#92860=AXIS2_PLACEMENT_3D('',#139884,#107500,#107501) ;
#92861=AXIS2_PLACEMENT_3D('',#139885,#107502,#107503) ;
#92862=AXIS2_PLACEMENT_3D('',#139886,#107504,#107505) ;
#92863=AXIS2_PLACEMENT_3D('',#139887,#107506,#107507) ;
#92864=AXIS2_PLACEMENT_3D('',#139888,#107508,#107509) ;
#92865=AXIS2_PLACEMENT_3D('',#139889,#107510,#107511) ;
#92866=AXIS2_PLACEMENT_3D('',#139890,#107512,#107513) ;
#92867=AXIS2_PLACEMENT_3D('',#139891,#107514,#107515) ;
#92868=AXIS2_PLACEMENT_3D('',#139892,#107516,#107517) ;
#92869=AXIS2_PLACEMENT_3D('',#139893,#107518,#107519) ;
#92870=AXIS2_PLACEMENT_3D('',#139894,#107520,#107521) ;
#92871=AXIS2_PLACEMENT_3D('',#139895,#107522,#107523) ;
#92872=AXIS2_PLACEMENT_3D('',#139896,#107524,#107525) ;
#92873=AXIS2_PLACEMENT_3D('',#139897,#107526,#107527) ;
#92874=AXIS2_PLACEMENT_3D('',#139898,#107528,#107529) ;
#92875=AXIS2_PLACEMENT_3D('',#139899,#107530,#107531) ;
#92876=AXIS2_PLACEMENT_3D('',#139900,#107532,#107533) ;
#92877=AXIS2_PLACEMENT_3D('',#139905,#107534,#107535) ;
#92878=AXIS2_PLACEMENT_3D('',#139906,#107536,#107537) ;
#92879=AXIS2_PLACEMENT_3D('',#139907,#107538,#107539) ;
#92880=AXIS2_PLACEMENT_3D('',#139908,#107540,#107541) ;
#92881=AXIS2_PLACEMENT_3D('',#139913,#107542,#107543) ;
#92882=AXIS2_PLACEMENT_3D('',#139914,#107544,#107545) ;
#92883=AXIS2_PLACEMENT_3D('',#139915,#107546,#107547) ;
#92884=AXIS2_PLACEMENT_3D('',#139916,#107548,#107549) ;
#92885=AXIS2_PLACEMENT_3D('',#139929,#107550,#107551) ;
#92886=AXIS2_PLACEMENT_3D('',#139942,#107552,#107553) ;
#92887=AXIS2_PLACEMENT_3D('',#139943,#107554,#107555) ;
#92888=AXIS2_PLACEMENT_3D('',#139944,#107556,#107557) ;
#92889=AXIS2_PLACEMENT_3D('',#139945,#107558,#107559) ;
#92890=AXIS2_PLACEMENT_3D('',#139946,#107560,#107561) ;
#92891=AXIS2_PLACEMENT_3D('',#139947,#107562,#107563) ;
#92892=AXIS2_PLACEMENT_3D('',#139948,#107564,#107565) ;
#92893=AXIS2_PLACEMENT_3D('',#139949,#107566,#107567) ;
#92894=AXIS2_PLACEMENT_3D('',#139950,#107568,#107569) ;
#92895=AXIS2_PLACEMENT_3D('',#139951,#107570,#107571) ;
#92896=AXIS2_PLACEMENT_3D('',#139952,#107572,#107573) ;
#92897=AXIS2_PLACEMENT_3D('',#139953,#107574,#107575) ;
#92898=AXIS2_PLACEMENT_3D('',#139954,#107576,#107577) ;
#92899=AXIS2_PLACEMENT_3D('',#139955,#107578,#107579) ;
#92900=AXIS2_PLACEMENT_3D('',#139956,#107580,#107581) ;
#92901=AXIS2_PLACEMENT_3D('',#139957,#107582,#107583) ;
#92902=AXIS2_PLACEMENT_3D('',#139958,#107584,#107585) ;
#92903=AXIS2_PLACEMENT_3D('',#139961,#107586,#107587) ;
#92904=AXIS2_PLACEMENT_3D('',#139963,#107588,#107589) ;
#92905=AXIS2_PLACEMENT_3D('',#139965,#107590,#107591) ;
#92906=AXIS2_PLACEMENT_3D('',#139966,#107592,#107593) ;
#92907=AXIS2_PLACEMENT_3D('',#139967,#107594,#107595) ;
#92908=AXIS2_PLACEMENT_3D('',#139970,#107596,#107597) ;
#92909=AXIS2_PLACEMENT_3D('',#139974,#107599,#107600) ;
#92910=AXIS2_PLACEMENT_3D('',#139976,#107602,#107603) ;
#92911=AXIS2_PLACEMENT_3D('',#139978,#107604,#107605) ;
#92912=AXIS2_PLACEMENT_3D('',#139980,#107606,#107607) ;
#92913=AXIS2_PLACEMENT_3D('',#139982,#107608,#107609) ;
#92914=AXIS2_PLACEMENT_3D('',#139983,#107610,#107611) ;
#92915=AXIS2_PLACEMENT_3D('',#139984,#107612,#107613) ;
#92916=AXIS2_PLACEMENT_3D('',#139986,#107614,#107615) ;
#92917=AXIS2_PLACEMENT_3D('',#139988,#107616,#107617) ;
#92918=AXIS2_PLACEMENT_3D('',#139989,#107618,#107619) ;
#92919=AXIS2_PLACEMENT_3D('',#139990,#107620,#107621) ;
#92920=AXIS2_PLACEMENT_3D('',#139992,#107622,#107623) ;
#92921=AXIS2_PLACEMENT_3D('',#139994,#107624,#107625) ;
#92922=AXIS2_PLACEMENT_3D('',#139996,#107626,#107627) ;
#92923=AXIS2_PLACEMENT_3D('',#139997,#107628,#107629) ;
#92924=AXIS2_PLACEMENT_3D('',#139998,#107630,#107631) ;
#92925=AXIS2_PLACEMENT_3D('',#140001,#107632,#107633) ;
#92926=AXIS2_PLACEMENT_3D('',#140003,#107634,#107635) ;
#92927=AXIS2_PLACEMENT_3D('',#140005,#107636,#107637) ;
#92928=AXIS2_PLACEMENT_3D('',#140006,#107638,#107639) ;
#92929=AXIS2_PLACEMENT_3D('',#140007,#107640,#107641) ;
#92930=AXIS2_PLACEMENT_3D('',#140010,#107642,#107643) ;
#92931=AXIS2_PLACEMENT_3D('',#140012,#107644,#107645) ;
#92932=AXIS2_PLACEMENT_3D('',#140013,#107646,#107647) ;
#92933=AXIS2_PLACEMENT_3D('',#140014,#107648,#107649) ;
#92934=AXIS2_PLACEMENT_3D('',#140018,#107651,#107652) ;
#92935=AXIS2_PLACEMENT_3D('',#140020,#107654,#107655) ;
#92936=AXIS2_PLACEMENT_3D('',#140023,#107656,#107657) ;
#92937=AXIS2_PLACEMENT_3D('',#140025,#107658,#107659) ;
#92938=AXIS2_PLACEMENT_3D('',#140026,#107660,#107661) ;
#92939=AXIS2_PLACEMENT_3D('',#140027,#107662,#107663) ;
#92940=AXIS2_PLACEMENT_3D('',#140029,#107664,#107665) ;
#92941=AXIS2_PLACEMENT_3D('',#140031,#107667,#107668) ;
#92942=AXIS2_PLACEMENT_3D('',#140033,#107670,#107671) ;
#92943=AXIS2_PLACEMENT_3D('',#140036,#107672,#107673) ;
#92944=AXIS2_PLACEMENT_3D('',#140062,#107675,#107676) ;
#92945=AXIS2_PLACEMENT_3D('',#140109,#107678,#107679) ;
#92946=AXIS2_PLACEMENT_3D('',#140135,#107681,#107682) ;
#92947=AXIS2_PLACEMENT_3D('',#140181,#107684,#107685) ;
#92948=AXIS2_PLACEMENT_3D('',#140183,#107687,#107688) ;
#92949=AXIS2_PLACEMENT_3D('',#140186,#107689,#107690) ;
#92950=AXIS2_PLACEMENT_3D('',#140192,#107694,#107695) ;
#92951=AXIS2_PLACEMENT_3D('',#140201,#107700,#107701) ;
#92952=AXIS2_PLACEMENT_3D('',#140209,#107706,#107707) ;
#92953=AXIS2_PLACEMENT_3D('',#140211,#107709,#107710) ;
#92954=AXIS2_PLACEMENT_3D('',#140220,#107715,#107716) ;
#92955=AXIS2_PLACEMENT_3D('',#140222,#107717,#107718) ;
#92956=AXIS2_PLACEMENT_3D('',#140224,#107719,#107720) ;
#92957=AXIS2_PLACEMENT_3D('',#140233,#107725,#107726) ;
#92958=AXIS2_PLACEMENT_3D('',#140235,#107728,#107729) ;
#92959=AXIS2_PLACEMENT_3D('',#140243,#107734,#107735) ;
#92960=AXIS2_PLACEMENT_3D('',#140250,#107738,#107739) ;
#92961=AXIS2_PLACEMENT_3D('',#140254,#107741,#107742) ;
#92962=AXIS2_PLACEMENT_3D('',#140260,#107746,#107747) ;
#92963=AXIS2_PLACEMENT_3D('',#140269,#107752,#107753) ;
#92964=AXIS2_PLACEMENT_3D('',#140278,#107758,#107759) ;
#92965=AXIS2_PLACEMENT_3D('',#140287,#107764,#107765) ;
#92966=AXIS2_PLACEMENT_3D('',#140296,#107770,#107771) ;
#92967=AXIS2_PLACEMENT_3D('',#140305,#107776,#107777) ;
#92968=AXIS2_PLACEMENT_3D('',#140314,#107782,#107783) ;
#92969=AXIS2_PLACEMENT_3D('',#140325,#107788,#107789) ;
#92970=AXIS2_PLACEMENT_3D('',#140329,#107791,#107792) ;
#92971=AXIS2_PLACEMENT_3D('',#140333,#107794,#107795) ;
#92972=AXIS2_PLACEMENT_3D('',#140337,#107797,#107798) ;
#92973=AXIS2_PLACEMENT_3D('',#140339,#107800,#107801) ;
#92974=AXIS2_PLACEMENT_3D('',#140348,#107806,#107807) ;
#92975=AXIS2_PLACEMENT_3D('',#140354,#107811,#107812) ;
#92976=AXIS2_PLACEMENT_3D('',#140360,#107816,#107817) ;
#92977=AXIS2_PLACEMENT_3D('',#140405,#107826,#107827) ;
#92978=AXIS2_PLACEMENT_3D('',#140416,#107832,#107833) ;
#92979=AXIS2_PLACEMENT_3D('',#140420,#107835,#107836) ;
#92980=AXIS2_PLACEMENT_3D('',#140424,#107838,#107839) ;
#92981=AXIS2_PLACEMENT_3D('',#140428,#107841,#107842) ;
#92982=AXIS2_PLACEMENT_3D('',#140430,#107844,#107845) ;
#92983=AXIS2_PLACEMENT_3D('',#140439,#107850,#107851) ;
#92984=AXIS2_PLACEMENT_3D('',#140533,#107857,#107858) ;
#92985=AXIS2_PLACEMENT_3D('',#140540,#107861,#107862) ;
#92986=AXIS2_PLACEMENT_3D('',#140542,#107864,#107865) ;
#92987=AXIS2_PLACEMENT_3D('',#140551,#107870,#107871) ;
#92988=AXIS2_PLACEMENT_3D('',#140552,#107872,#107873) ;
#92989=AXIS2_PLACEMENT_3D('',#140553,#107874,#107875) ;
#92990=AXIS2_PLACEMENT_3D('',#140554,#107876,#107877) ;
#92991=AXIS2_PLACEMENT_3D('',#140555,#107878,#107879) ;
#92992=AXIS2_PLACEMENT_3D('',#140556,#107880,#107881) ;
#92993=AXIS2_PLACEMENT_3D('',#140557,#107882,#107883) ;
#92994=AXIS2_PLACEMENT_3D('',#140558,#107884,#107885) ;
#92995=AXIS2_PLACEMENT_3D('',#140559,#107886,#107887) ;
#92996=AXIS2_PLACEMENT_3D('',#140560,#107888,#107889) ;
#92997=AXIS2_PLACEMENT_3D('',#140561,#107890,#107891) ;
#92998=AXIS2_PLACEMENT_3D('',#140562,#107892,#107893) ;
#92999=AXIS2_PLACEMENT_3D('',#140563,#107894,#107895) ;
#93000=AXIS2_PLACEMENT_3D('',#140564,#107896,#107897) ;
#93001=AXIS2_PLACEMENT_3D('',#140565,#107898,#107899) ;
#93002=AXIS2_PLACEMENT_3D('',#140566,#107900,#107901) ;
#93003=AXIS2_PLACEMENT_3D('',#140567,#107902,#107903) ;
#93004=AXIS2_PLACEMENT_3D('',#140568,#107904,#107905) ;
#93005=AXIS2_PLACEMENT_3D('',#140569,#107906,#107907) ;
#93006=AXIS2_PLACEMENT_3D('',#140570,#107908,#107909) ;
#93007=AXIS2_PLACEMENT_3D('',#140571,#107910,#107911) ;
#93008=AXIS2_PLACEMENT_3D('',#140572,#107912,#107913) ;
#93009=AXIS2_PLACEMENT_3D('',#140573,#107914,#107915) ;
#93010=AXIS2_PLACEMENT_3D('',#140574,#107916,#107917) ;
#93011=AXIS2_PLACEMENT_3D('',#140575,#107918,#107919) ;
#93012=AXIS2_PLACEMENT_3D('',#140576,#107920,#107921) ;
#93013=AXIS2_PLACEMENT_3D('',#140577,#107922,#107923) ;
#93014=AXIS2_PLACEMENT_3D('',#140578,#107924,#107925) ;
#93015=AXIS2_PLACEMENT_3D('',#140579,#107926,#107927) ;
#93016=AXIS2_PLACEMENT_3D('',#140580,#107928,#107929) ;
#93017=AXIS2_PLACEMENT_3D('',#140581,#107930,#107931) ;
#93018=AXIS2_PLACEMENT_3D('',#140582,#107932,#107933) ;
#93019=AXIS2_PLACEMENT_3D('',#140583,#107934,#107935) ;
#93020=AXIS2_PLACEMENT_3D('',#140584,#107936,#107937) ;
#93021=AXIS2_PLACEMENT_3D('',#140585,#107938,#107939) ;
#93022=AXIS2_PLACEMENT_3D('',#140586,#107940,#107941) ;
#93023=AXIS2_PLACEMENT_3D('',#140587,#107942,#107943) ;
#93024=AXIS2_PLACEMENT_3D('',#140588,#107944,#107945) ;
#93025=AXIS2_PLACEMENT_3D('',#140589,#107946,#107947) ;
#93026=AXIS2_PLACEMENT_3D('',#140598,#107952,#107953) ;
#93027=AXIS2_PLACEMENT_3D('',#140607,#107958,#107959) ;
#93028=AXIS2_PLACEMENT_3D('',#140610,#107960,#107961) ;
#93029=AXIS2_PLACEMENT_3D('',#140618,#107965,#107966) ;
#93030=AXIS2_PLACEMENT_3D('',#140624,#107970,#107971) ;
#93031=AXIS2_PLACEMENT_3D('',#140629,#107973,#107974) ;
#93032=AXIS2_PLACEMENT_3D('',#140632,#107976,#107977) ;
#93033=AXIS2_PLACEMENT_3D('',#140634,#107978,#107979) ;
#93034=AXIS2_PLACEMENT_3D('',#140637,#107981,#107982) ;
#93035=AXIS2_PLACEMENT_3D('',#140638,#107983,#107984) ;
#93036=AXIS2_PLACEMENT_3D('',#140641,#107985,#107986) ;
#93037=AXIS2_PLACEMENT_3D('',#140646,#107989,#107990) ;
#93038=AXIS2_PLACEMENT_3D('',#140652,#107994,#107995) ;
#93039=AXIS2_PLACEMENT_3D('',#140658,#107999,#108000) ;
#93040=AXIS2_PLACEMENT_3D('',#140664,#108004,#108005) ;
#93041=AXIS2_PLACEMENT_3D('',#140677,#108012,#108013) ;
#93042=AXIS2_PLACEMENT_3D('',#140690,#108020,#108021) ;
#93043=AXIS2_PLACEMENT_3D('',#140699,#108026,#108027) ;
#93044=AXIS2_PLACEMENT_3D('',#140708,#108032,#108033) ;
#93045=AXIS2_PLACEMENT_3D('',#140717,#108038,#108039) ;
#93046=AXIS2_PLACEMENT_3D('',#140726,#108044,#108045) ;
#93047=AXIS2_PLACEMENT_3D('',#140739,#108051,#108052) ;
#93048=AXIS2_PLACEMENT_3D('',#140743,#108054,#108055) ;
#93049=AXIS2_PLACEMENT_3D('',#140747,#108057,#108058) ;
#93050=AXIS2_PLACEMENT_3D('',#140750,#108060,#108061) ;
#93051=AXIS2_PLACEMENT_3D('',#140751,#108062,#108063) ;
#93052=AXIS2_PLACEMENT_3D('',#140754,#108064,#108065) ;
#93053=AXIS2_PLACEMENT_3D('',#140757,#108068,#108069) ;
#93054=AXIS2_PLACEMENT_3D('',#140761,#108072,#108073) ;
#93055=AXIS2_PLACEMENT_3D('',#140763,#108074,#108075) ;
#93056=AXIS2_PLACEMENT_3D('',#140765,#108077,#108078) ;
#93057=AXIS2_PLACEMENT_3D('',#140769,#108081,#108082) ;
#93058=AXIS2_PLACEMENT_3D('',#140771,#108083,#108084) ;
#93059=AXIS2_PLACEMENT_3D('',#140773,#108086,#108087) ;
#93060=AXIS2_PLACEMENT_3D('',#140777,#108090,#108091) ;
#93061=AXIS2_PLACEMENT_3D('',#140779,#108092,#108093) ;
#93062=AXIS2_PLACEMENT_3D('',#140781,#108095,#108096) ;
#93063=AXIS2_PLACEMENT_3D('',#140783,#108098,#108099) ;
#93064=AXIS2_PLACEMENT_3D('',#140784,#108100,#108101) ;
#93065=AXIS2_PLACEMENT_3D('',#140786,#108103,#108104) ;
#93066=AXIS2_PLACEMENT_3D('',#140789,#108107,#108108) ;
#93067=AXIS2_PLACEMENT_3D('',#140792,#108111,#108112) ;
#93068=AXIS2_PLACEMENT_3D('',#140795,#108115,#108116) ;
#93069=AXIS2_PLACEMENT_3D('',#140804,#108121,#108122) ;
#93070=AXIS2_PLACEMENT_3D('',#140813,#108127,#108128) ;
#93071=AXIS2_PLACEMENT_3D('',#140822,#108133,#108134) ;
#93072=AXIS2_PLACEMENT_3D('',#140831,#108139,#108140) ;
#93073=AXIS2_PLACEMENT_3D('',#140844,#108146,#108147) ;
#93074=AXIS2_PLACEMENT_3D('',#140848,#108149,#108150) ;
#93075=AXIS2_PLACEMENT_3D('',#140852,#108152,#108153) ;
#93076=AXIS2_PLACEMENT_3D('',#140855,#108155,#108156) ;
#93077=AXIS2_PLACEMENT_3D('',#140856,#108157,#108158) ;
#93078=AXIS2_PLACEMENT_3D('',#140860,#108160,#108161) ;
#93079=AXIS2_PLACEMENT_3D('',#140862,#108163,#108164) ;
#93080=AXIS2_PLACEMENT_3D('',#140866,#108167,#108168) ;
#93081=AXIS2_PLACEMENT_3D('',#140868,#108169,#108170) ;
#93082=AXIS2_PLACEMENT_3D('',#140870,#108172,#108173) ;
#93083=AXIS2_PLACEMENT_3D('',#140874,#108176,#108177) ;
#93084=AXIS2_PLACEMENT_3D('',#140876,#108178,#108179) ;
#93085=AXIS2_PLACEMENT_3D('',#140878,#108181,#108182) ;
#93086=AXIS2_PLACEMENT_3D('',#140882,#108185,#108186) ;
#93087=AXIS2_PLACEMENT_3D('',#140884,#108187,#108188) ;
#93088=AXIS2_PLACEMENT_3D('',#140886,#108190,#108191) ;
#93089=AXIS2_PLACEMENT_3D('',#140888,#108193,#108194) ;
#93090=AXIS2_PLACEMENT_3D('',#140897,#108199,#108200) ;
#93091=AXIS2_PLACEMENT_3D('',#140904,#108205,#108206) ;
#93092=AXIS2_PLACEMENT_3D('',#140910,#108210,#108211) ;
#93093=AXIS2_PLACEMENT_3D('',#140915,#108215,#108216) ;
#93094=AXIS2_PLACEMENT_3D('',#140919,#108218,#108219) ;
#93095=AXIS2_PLACEMENT_3D('',#140925,#108223,#108224) ;
#93096=AXIS2_PLACEMENT_3D('',#140926,#108225,#108226) ;
#93097=AXIS2_PLACEMENT_3D('',#140929,#108227,#108228) ;
#93098=AXIS2_PLACEMENT_3D('',#140931,#108229,#108230) ;
#93099=AXIS2_PLACEMENT_3D('',#140933,#108231,#108232) ;
#93100=AXIS2_PLACEMENT_3D('',#140937,#108234,#108235) ;
#93101=AXIS2_PLACEMENT_3D('',#140957,#108237,#108238) ;
#93102=AXIS2_PLACEMENT_3D('',#140964,#108239,#108240) ;
#93103=AXIS2_PLACEMENT_3D('',#140965,#108241,#108242) ;
#93104=AXIS2_PLACEMENT_3D('',#140966,#108243,#108244) ;
#93105=AXIS2_PLACEMENT_3D('',#140979,#108245,#108246) ;
#93106=AXIS2_PLACEMENT_3D('',#140980,#108247,#108248) ;
#93107=AXIS2_PLACEMENT_3D('',#140981,#108249,#108250) ;
#93108=AXIS2_PLACEMENT_3D('',#140982,#108251,#108252) ;
#93109=AXIS2_PLACEMENT_3D('',#140983,#108253,#108254) ;
#93110=AXIS2_PLACEMENT_3D('',#140984,#108255,#108256) ;
#93111=AXIS2_PLACEMENT_3D('',#140985,#108257,#108258) ;
#93112=AXIS2_PLACEMENT_3D('',#140986,#108259,#108260) ;
#93113=AXIS2_PLACEMENT_3D('',#140987,#108261,#108262) ;
#93114=AXIS2_PLACEMENT_3D('',#140988,#108263,#108264) ;
#93115=AXIS2_PLACEMENT_3D('',#140989,#108265,#108266) ;
#93116=AXIS2_PLACEMENT_3D('',#140990,#108267,#108268) ;
#93117=AXIS2_PLACEMENT_3D('',#140991,#108269,#108270) ;
#93118=AXIS2_PLACEMENT_3D('',#140992,#108271,#108272) ;
#93119=AXIS2_PLACEMENT_3D('',#140993,#108273,#108274) ;
#93120=AXIS2_PLACEMENT_3D('',#140994,#108275,#108276) ;
#93121=AXIS2_PLACEMENT_3D('',#141013,#108277,#108278) ;
#93122=AXIS2_PLACEMENT_3D('',#141014,#108279,#108280) ;
#93123=AXIS2_PLACEMENT_3D('',#141033,#108281,#108282) ;
#93124=AXIS2_PLACEMENT_3D('',#141052,#108283,#108284) ;
#93125=AXIS2_PLACEMENT_3D('',#141053,#108285,#108286) ;
#93126=AXIS2_PLACEMENT_3D('',#141054,#108287,#108288) ;
#93127=AXIS2_PLACEMENT_3D('',#141055,#108289,#108290) ;
#93128=AXIS2_PLACEMENT_3D('',#141056,#108291,#108292) ;
#93129=AXIS2_PLACEMENT_3D('',#141057,#108293,#108294) ;
#93130=AXIS2_PLACEMENT_3D('',#141058,#108295,#108296) ;
#93131=AXIS2_PLACEMENT_3D('',#141059,#108297,#108298) ;
#93132=AXIS2_PLACEMENT_3D('',#141060,#108299,#108300) ;
#93133=AXIS2_PLACEMENT_3D('',#141061,#108301,#108302) ;
#93134=AXIS2_PLACEMENT_3D('',#141062,#108303,#108304) ;
#93135=AXIS2_PLACEMENT_3D('',#141063,#108305,#108306) ;
#93136=AXIS2_PLACEMENT_3D('',#141064,#108307,#108308) ;
#93137=AXIS2_PLACEMENT_3D('',#141065,#108309,#108310) ;
#93138=AXIS2_PLACEMENT_3D('',#141066,#108311,#108312) ;
#93139=AXIS2_PLACEMENT_3D('',#141085,#108313,#108314) ;
#93140=AXIS2_PLACEMENT_3D('',#141086,#108315,#108316) ;
#93141=AXIS2_PLACEMENT_3D('',#141087,#108317,#108318) ;
#93142=AXIS2_PLACEMENT_3D('',#141088,#108319,#108320) ;
#93143=AXIS2_PLACEMENT_3D('',#141089,#108321,#108322) ;
#93144=AXIS2_PLACEMENT_3D('',#141090,#108323,#108324) ;
#93145=AXIS2_PLACEMENT_3D('',#141091,#108325,#108326) ;
#93146=AXIS2_PLACEMENT_3D('',#141092,#108327,#108328) ;
#93147=AXIS2_PLACEMENT_3D('',#141093,#108329,#108330) ;
#93148=AXIS2_PLACEMENT_3D('',#141094,#108331,#108332) ;
#93149=AXIS2_PLACEMENT_3D('',#141095,#108333,#108334) ;
#93150=AXIS2_PLACEMENT_3D('',#141108,#108335,#108336) ;
#93151=AXIS2_PLACEMENT_3D('',#141109,#108337,#108338) ;
#93152=AXIS2_PLACEMENT_3D('',#141110,#108339,#108340) ;
#93153=AXIS2_PLACEMENT_3D('',#141111,#108341,#108342) ;
#93154=AXIS2_PLACEMENT_3D('',#141112,#108343,#108344) ;
#93155=AXIS2_PLACEMENT_3D('',#141113,#108345,#108346) ;
#93156=AXIS2_PLACEMENT_3D('',#141114,#108347,#108348) ;
#93157=AXIS2_PLACEMENT_3D('',#141127,#108349,#108350) ;
#93158=AXIS2_PLACEMENT_3D('',#141128,#108351,#108352) ;
#93159=AXIS2_PLACEMENT_3D('',#141129,#108353,#108354) ;
#93160=AXIS2_PLACEMENT_3D('',#141130,#108355,#108356) ;
#93161=AXIS2_PLACEMENT_3D('',#141132,#108357,#108358) ;
#93162=AXIS2_PLACEMENT_3D('',#141152,#108359,#108360) ;
#93163=AXIS2_PLACEMENT_3D('',#141153,#108361,#108362) ;
#93164=AXIS2_PLACEMENT_3D('',#141154,#108363,#108364) ;
#93165=AXIS2_PLACEMENT_3D('',#141155,#108365,#108366) ;
#93166=AXIS2_PLACEMENT_3D('',#141156,#108367,#108368) ;
#93167=AXIS2_PLACEMENT_3D('',#141157,#108369,#108370) ;
#93168=AXIS2_PLACEMENT_3D('',#141186,#108371,#108372) ;
#93169=AXIS2_PLACEMENT_3D('',#141187,#108373,#108374) ;
#93170=AXIS2_PLACEMENT_3D('',#141188,#108375,#108376) ;
#93171=AXIS2_PLACEMENT_3D('',#141189,#108377,#108378) ;
#93172=AXIS2_PLACEMENT_3D('',#141190,#108379,#108380) ;
#93173=AXIS2_PLACEMENT_3D('',#141191,#108381,#108382) ;
#93174=AXIS2_PLACEMENT_3D('',#141192,#108383,#108384) ;
#93175=AXIS2_PLACEMENT_3D('',#141214,#108385,#108386) ;
#93176=AXIS2_PLACEMENT_3D('',#141215,#108387,#108388) ;
#93177=AXIS2_PLACEMENT_3D('',#141216,#108389,#108390) ;
#93178=AXIS2_PLACEMENT_3D('',#141217,#108391,#108392) ;
#93179=AXIS2_PLACEMENT_3D('',#141218,#108393,#108394) ;
#93180=AXIS2_PLACEMENT_3D('',#141219,#108395,#108396) ;
#93181=AXIS2_PLACEMENT_3D('',#141220,#108397,#108398) ;
#93182=AXIS2_PLACEMENT_3D('',#141221,#108399,#108400) ;
#93183=AXIS2_PLACEMENT_3D('',#141222,#108401,#108402) ;
#93184=AXIS2_PLACEMENT_3D('',#141223,#108403,#108404) ;
#93185=AXIS2_PLACEMENT_3D('',#141224,#108405,#108406) ;
#93186=AXIS2_PLACEMENT_3D('',#141225,#108407,#108408) ;
#93187=AXIS2_PLACEMENT_3D('',#141226,#108409,#108410) ;
#93188=AXIS2_PLACEMENT_3D('',#141227,#108411,#108412) ;
#93189=AXIS2_PLACEMENT_3D('',#141228,#108413,#108414) ;
#93190=AXIS2_PLACEMENT_3D('',#141229,#108415,#108416) ;
#93191=AXIS2_PLACEMENT_3D('',#141230,#108417,#108418) ;
#93192=AXIS2_PLACEMENT_3D('',#141231,#108419,#108420) ;
#93193=AXIS2_PLACEMENT_3D('',#141232,#108421,#108422) ;
#93194=AXIS2_PLACEMENT_3D('',#141233,#108423,#108424) ;
#93195=AXIS2_PLACEMENT_3D('',#141234,#108425,#108426) ;
#93196=AXIS2_PLACEMENT_3D('',#141235,#108427,#108428) ;
#93197=AXIS2_PLACEMENT_3D('',#141236,#108429,#108430) ;
#93198=AXIS2_PLACEMENT_3D('',#141237,#108431,#108432) ;
#93199=AXIS2_PLACEMENT_3D('',#141238,#108433,#108434) ;
#93200=AXIS2_PLACEMENT_3D('',#141239,#108435,#108436) ;
#93201=AXIS2_PLACEMENT_3D('',#141240,#108437,#108438) ;
#93202=AXIS2_PLACEMENT_3D('',#141241,#108439,#108440) ;
#93203=AXIS2_PLACEMENT_3D('',#141242,#108441,#108442) ;
#93204=AXIS2_PLACEMENT_3D('',#141243,#108443,#108444) ;
#93205=AXIS2_PLACEMENT_3D('',#141244,#108445,#108446) ;
#93206=AXIS2_PLACEMENT_3D('',#141245,#108447,#108448) ;
#93207=AXIS2_PLACEMENT_3D('',#141246,#108449,#108450) ;
#93208=AXIS2_PLACEMENT_3D('',#141247,#108451,#108452) ;
#93209=AXIS2_PLACEMENT_3D('',#141248,#108453,#108454) ;
#93210=AXIS2_PLACEMENT_3D('',#141249,#108455,#108456) ;
#93211=AXIS2_PLACEMENT_3D('',#141250,#108457,#108458) ;
#93212=AXIS2_PLACEMENT_3D('',#141251,#108459,#108460) ;
#93213=AXIS2_PLACEMENT_3D('',#141252,#108461,#108462) ;
#93214=AXIS2_PLACEMENT_3D('',#141253,#108463,#108464) ;
#93215=AXIS2_PLACEMENT_3D('',#141254,#108465,#108466) ;
#93216=AXIS2_PLACEMENT_3D('',#141255,#108467,#108468) ;
#93217=AXIS2_PLACEMENT_3D('',#141256,#108469,#108470) ;
#93218=AXIS2_PLACEMENT_3D('',#141257,#108471,#108472) ;
#93219=AXIS2_PLACEMENT_3D('',#141258,#108473,#108474) ;
#93220=AXIS2_PLACEMENT_3D('',#141259,#108475,#108476) ;
#93221=AXIS2_PLACEMENT_3D('',#141260,#108477,#108478) ;
#93222=AXIS2_PLACEMENT_3D('',#141261,#108479,#108480) ;
#93223=AXIS2_PLACEMENT_3D('',#141262,#108481,#108482) ;
#93224=AXIS2_PLACEMENT_3D('',#141263,#108483,#108484) ;
#93225=AXIS2_PLACEMENT_3D('',#141264,#108485,#108486) ;
#93226=AXIS2_PLACEMENT_3D('',#141265,#108487,#108488) ;
#93227=AXIS2_PLACEMENT_3D('',#141266,#108489,#108490) ;
#93228=AXIS2_PLACEMENT_3D('',#141267,#108491,#108492) ;
#93229=AXIS2_PLACEMENT_3D('',#141268,#108493,#108494) ;
#93230=AXIS2_PLACEMENT_3D('',#141269,#108495,#108496) ;
#93231=AXIS2_PLACEMENT_3D('',#141270,#108497,#108498) ;
#93232=AXIS2_PLACEMENT_3D('',#141271,#108499,#108500) ;
#93233=AXIS2_PLACEMENT_3D('',#141272,#108501,#108502) ;
#93234=AXIS2_PLACEMENT_3D('',#141273,#108503,#108504) ;
#93235=AXIS2_PLACEMENT_3D('',#141274,#108505,#108506) ;
#93236=AXIS2_PLACEMENT_3D('',#141275,#108507,#108508) ;
#93237=AXIS2_PLACEMENT_3D('',#141276,#108509,#108510) ;
#93238=AXIS2_PLACEMENT_3D('',#141277,#108511,#108512) ;
#93239=AXIS2_PLACEMENT_3D('',#141278,#108513,#108514) ;
#93240=AXIS2_PLACEMENT_3D('',#141279,#108515,#108516) ;
#93241=AXIS2_PLACEMENT_3D('',#141280,#108517,#108518) ;
#93242=AXIS2_PLACEMENT_3D('',#141281,#108519,#108520) ;
#93243=AXIS2_PLACEMENT_3D('',#141282,#108521,#108522) ;
#93244=AXIS2_PLACEMENT_3D('',#141283,#108523,#108524) ;
#93245=AXIS2_PLACEMENT_3D('',#141284,#108525,#108526) ;
#93246=AXIS2_PLACEMENT_3D('',#141285,#108527,#108528) ;
#93247=AXIS2_PLACEMENT_3D('',#141286,#108529,#108530) ;
#93248=AXIS2_PLACEMENT_3D('',#141287,#108531,#108532) ;
#93249=AXIS2_PLACEMENT_3D('',#141288,#108533,#108534) ;
#93250=AXIS2_PLACEMENT_3D('',#141289,#108535,#108536) ;
#93251=AXIS2_PLACEMENT_3D('',#141290,#108537,#108538) ;
#93252=AXIS2_PLACEMENT_3D('',#141291,#108539,#108540) ;
#93253=AXIS2_PLACEMENT_3D('',#141292,#108541,#108542) ;
#93254=AXIS2_PLACEMENT_3D('',#141293,#108543,#108544) ;
#93255=AXIS2_PLACEMENT_3D('',#141294,#108545,#108546) ;
#93256=AXIS2_PLACEMENT_3D('',#141295,#108547,#108548) ;
#93257=AXIS2_PLACEMENT_3D('',#141296,#108549,#108550) ;
#93258=AXIS2_PLACEMENT_3D('',#141297,#108551,#108552) ;
#93259=AXIS2_PLACEMENT_3D('',#141298,#108553,#108554) ;
#93260=AXIS2_PLACEMENT_3D('',#141299,#108555,#108556) ;
#93261=AXIS2_PLACEMENT_3D('',#141300,#108557,#108558) ;
#93262=AXIS2_PLACEMENT_3D('',#141301,#108559,#108560) ;
#93263=AXIS2_PLACEMENT_3D('',#141302,#108561,#108562) ;
#93264=AXIS2_PLACEMENT_3D('',#141303,#108563,#108564) ;
#93265=AXIS2_PLACEMENT_3D('',#141304,#108565,#108566) ;
#93266=AXIS2_PLACEMENT_3D('',#141305,#108567,#108568) ;
#93267=AXIS2_PLACEMENT_3D('',#141306,#108569,#108570) ;
#93268=AXIS2_PLACEMENT_3D('',#141307,#108571,#108572) ;
#93269=AXIS2_PLACEMENT_3D('',#141308,#108573,#108574) ;
#93270=AXIS2_PLACEMENT_3D('',#141309,#108575,#108576) ;
#93271=AXIS2_PLACEMENT_3D('',#141310,#108577,#108578) ;
#93272=AXIS2_PLACEMENT_3D('',#141311,#108579,#108580) ;
#93273=AXIS2_PLACEMENT_3D('',#141312,#108581,#108582) ;
#93274=AXIS2_PLACEMENT_3D('',#141313,#108583,#108584) ;
#93275=AXIS2_PLACEMENT_3D('',#141314,#108585,#108586) ;
#93276=AXIS2_PLACEMENT_3D('',#141315,#108587,#108588) ;
#93277=AXIS2_PLACEMENT_3D('',#141316,#108589,#108590) ;
#93278=AXIS2_PLACEMENT_3D('',#141317,#108591,#108592) ;
#93279=AXIS2_PLACEMENT_3D('',#141318,#108593,#108594) ;
#93280=AXIS2_PLACEMENT_3D('',#141319,#108595,#108596) ;
#93281=AXIS2_PLACEMENT_3D('',#141320,#108597,#108598) ;
#93282=AXIS2_PLACEMENT_3D('',#141321,#108599,#108600) ;
#93283=AXIS2_PLACEMENT_3D('',#141322,#108601,#108602) ;
#93284=AXIS2_PLACEMENT_3D('',#141335,#108603,#108604) ;
#93285=AXIS2_PLACEMENT_3D('',#141336,#108605,#108606) ;
#93286=AXIS2_PLACEMENT_3D('',#141337,#108607,#108608) ;
#93287=AXIS2_PLACEMENT_3D('',#141338,#108609,#108610) ;
#93288=AXIS2_PLACEMENT_3D('',#141339,#108611,#108612) ;
#93289=AXIS2_PLACEMENT_3D('',#141340,#108613,#108614) ;
#93290=AXIS2_PLACEMENT_3D('',#141341,#108615,#108616) ;
#93291=AXIS2_PLACEMENT_3D('',#141342,#108617,#108618) ;
#93292=AXIS2_PLACEMENT_3D('',#141343,#108619,#108620) ;
#93293=AXIS2_PLACEMENT_3D('',#141344,#108621,#108622) ;
#93294=AXIS2_PLACEMENT_3D('',#141345,#108623,#108624) ;
#93295=AXIS2_PLACEMENT_3D('',#141346,#108625,#108626) ;
#93296=AXIS2_PLACEMENT_3D('',#141347,#108627,#108628) ;
#93297=AXIS2_PLACEMENT_3D('',#141348,#108629,#108630) ;
#93298=AXIS2_PLACEMENT_3D('',#141349,#108631,#108632) ;
#93299=AXIS2_PLACEMENT_3D('',#141350,#108633,#108634) ;
#93300=AXIS2_PLACEMENT_3D('',#141351,#108635,#108636) ;
#93301=AXIS2_PLACEMENT_3D('',#141352,#108637,#108638) ;
#93302=AXIS2_PLACEMENT_3D('',#141353,#108639,#108640) ;
#93303=AXIS2_PLACEMENT_3D('',#141354,#108641,#108642) ;
#93304=AXIS2_PLACEMENT_3D('',#141355,#108643,#108644) ;
#93305=AXIS2_PLACEMENT_3D('',#141356,#108645,#108646) ;
#93306=AXIS2_PLACEMENT_3D('',#141357,#108647,#108648) ;
#93307=AXIS2_PLACEMENT_3D('',#141358,#108649,#108650) ;
#93308=AXIS2_PLACEMENT_3D('',#141371,#108651,#108652) ;
#93309=AXIS2_PLACEMENT_3D('',#141372,#108653,#108654) ;
#93310=AXIS2_PLACEMENT_3D('',#141373,#108655,#108656) ;
#93311=AXIS2_PLACEMENT_3D('',#141374,#108657,#108658) ;
#93312=AXIS2_PLACEMENT_3D('',#141375,#108659,#108660) ;
#93313=AXIS2_PLACEMENT_3D('',#141376,#108661,#108662) ;
#93314=AXIS2_PLACEMENT_3D('',#141377,#108663,#108664) ;
#93315=AXIS2_PLACEMENT_3D('',#141378,#108665,#108666) ;
#93316=AXIS2_PLACEMENT_3D('',#141379,#108667,#108668) ;
#93317=AXIS2_PLACEMENT_3D('',#141380,#108669,#108670) ;
#93318=AXIS2_PLACEMENT_3D('',#141381,#108671,#108672) ;
#93319=AXIS2_PLACEMENT_3D('',#141382,#108673,#108674) ;
#93320=AXIS2_PLACEMENT_3D('',#141383,#108675,#108676) ;
#93321=AXIS2_PLACEMENT_3D('',#141384,#108677,#108678) ;
#93322=AXIS2_PLACEMENT_3D('',#141385,#108679,#108680) ;
#93323=AXIS2_PLACEMENT_3D('',#141386,#108681,#108682) ;
#93324=AXIS2_PLACEMENT_3D('',#141387,#108683,#108684) ;
#93325=AXIS2_PLACEMENT_3D('',#141388,#108685,#108686) ;
#93326=AXIS2_PLACEMENT_3D('',#141389,#108687,#108688) ;
#93327=AXIS2_PLACEMENT_3D('',#141390,#108689,#108690) ;
#93328=AXIS2_PLACEMENT_3D('',#141391,#108691,#108692) ;
#93329=AXIS2_PLACEMENT_3D('',#141392,#108693,#108694) ;
#93330=AXIS2_PLACEMENT_3D('',#141393,#108695,#108696) ;
#93331=AXIS2_PLACEMENT_3D('',#141406,#108697,#108698) ;
#93332=AXIS2_PLACEMENT_3D('',#141419,#108699,#108700) ;
#93333=AXIS2_PLACEMENT_3D('',#141420,#108701,#108702) ;
#93334=AXIS2_PLACEMENT_3D('',#141421,#108703,#108704) ;
#93335=AXIS2_PLACEMENT_3D('',#141422,#108705,#108706) ;
#93336=AXIS2_PLACEMENT_3D('',#141435,#108707,#108708) ;
#93337=AXIS2_PLACEMENT_3D('',#141448,#108709,#108710) ;
#93338=AXIS2_PLACEMENT_3D('',#141449,#108711,#108712) ;
#93339=AXIS2_PLACEMENT_3D('',#141450,#108713,#108714) ;
#93340=AXIS2_PLACEMENT_3D('',#141451,#108715,#108716) ;
#93341=AXIS2_PLACEMENT_3D('',#141529,#108717,#108718) ;
#93342=AXIS2_PLACEMENT_3D('',#141530,#108719,#108720) ;
#93343=AXIS2_PLACEMENT_3D('',#141599,#108721,#108722) ;
#93344=AXIS2_PLACEMENT_3D('',#141600,#108723,#108724) ;
#93345=AXIS2_PLACEMENT_3D('',#141715,#108725,#108726) ;
#93346=AXIS2_PLACEMENT_3D('',#141746,#108727,#108728) ;
#93347=AXIS2_PLACEMENT_3D('',#141777,#108729,#108730) ;
#103082=DIRECTION('axis',(0.,0.,1.)) ;
#103083=DIRECTION('refdir',(1.,0.,0.)) ;
#103084=DIRECTION('center_axis',(-1.,0.,0.)) ;
#103085=DIRECTION('ref_axis',(0.,0.,1.)) ;
#103086=DIRECTION('center_axis',(-1.,0.,0.)) ;
#103087=DIRECTION('ref_axis',(0.,0.,1.)) ;
#103088=DIRECTION('center_axis',(-3.56483478381767E-16,0.986393923832144,
0.164398987305358)) ;
#103089=DIRECTION('ref_axis',(1.28176283288123E-31,-0.164398987305358,0.986393923832144)) ;
#103090=DIRECTION('center_axis',(1.,0.,0.)) ;
#103091=DIRECTION('ref_axis',(0.,0.,1.)) ;
#103092=DIRECTION('center_axis',(-4.02631181035926E-15,0.928404294083138,
-0.371571617226061)) ;
#103093=DIRECTION('ref_axis',(1.34987128984705E-31,0.371571617226061,0.928404294083138)) ;
#103094=DIRECTION('center_axis',(0.,-1.,0.)) ;
#103095=DIRECTION('ref_axis',(0.,0.,-1.)) ;
#103096=DIRECTION('center_axis',(0.,-1.,0.)) ;
#103097=DIRECTION('ref_axis',(0.,0.,-1.)) ;
#103098=DIRECTION('center_axis',(-1.,0.,-1.22464679914735E-16)) ;
#103099=DIRECTION('ref_axis',(-1.22464679914735E-16,0.,1.)) ;
#103100=DIRECTION('center_axis',(0.,1.,0.)) ;
#103101=DIRECTION('ref_axis',(0.,0.,-1.)) ;
#103102=DIRECTION('center_axis',(0.,1.,0.)) ;
#103103=DIRECTION('ref_axis',(0.,0.,-1.)) ;
#103104=DIRECTION('center_axis',(1.,0.,0.)) ;
#103105=DIRECTION('ref_axis',(0.,0.,-1.)) ;
#103106=DIRECTION('center_axis',(1.,0.,0.)) ;
#103107=DIRECTION('ref_axis',(0.,0.,-1.)) ;
#103108=DIRECTION('center_axis',(0.,1.,1.22464679914735E-16)) ;
#103109=DIRECTION('ref_axis',(0.,-1.22464679914735E-16,1.)) ;
#103110=DIRECTION('center_axis',(-1.,0.,0.)) ;
#103111=DIRECTION('ref_axis',(0.,0.,-1.)) ;
#103112=DIRECTION('center_axis',(-1.,0.,0.)) ;
#103113=DIRECTION('ref_axis',(0.,0.,1.)) ;
#103114=DIRECTION('center_axis',(-1.,0.,0.)) ;
#103115=DIRECTION('ref_axis',(0.,0.,1.)) ;
#103116=DIRECTION('center_axis',(0.,-1.,1.22464679914735E-16)) ;
#103117=DIRECTION('ref_axis',(0.,-1.22464679914735E-16,-1.)) ;
#103118=DIRECTION('center_axis',(1.,0.,0.)) ;
#103119=DIRECTION('ref_axis',(0.,0.,1.)) ;
#103120=DIRECTION('center_axis',(1.,0.,0.)) ;
#103121=DIRECTION('ref_axis',(0.,0.,1.)) ;
#103122=DIRECTION('center_axis',(-1.,0.,0.)) ;
#103123=DIRECTION('ref_axis',(0.,0.,1.)) ;
#103124=DIRECTION('center_axis',(-1.,0.,0.)) ;
#103125=DIRECTION('ref_axis',(0.,0.,1.)) ;
#103126=DIRECTION('center_axis',(0.,0.986393923832144,-0.164398987305358)) ;
#103127=DIRECTION('ref_axis',(0.,-0.164398987305358,-0.986393923832144)) ;
#103128=DIRECTION('center_axis',(1.,0.,0.)) ;
#103129=DIRECTION('ref_axis',(0.,0.,1.)) ;
#103130=DIRECTION('center_axis',(0.,0.,1.)) ;
#103131=DIRECTION('ref_axis',(1.,0.,0.)) ;
#103132=DIRECTION('center_axis',(0.,1.,0.)) ;
#103133=DIRECTION('ref_axis',(1.,0.,0.)) ;
#103134=DIRECTION('center_axis',(1.,0.,0.)) ;
#103135=DIRECTION('ref_axis',(0.,0.,-1.)) ;
#103136=DIRECTION('center_axis',(0.,0.,-1.)) ;
#103137=DIRECTION('ref_axis',(-1.,0.,0.)) ;
#103138=DIRECTION('center_axis',(0.,-0.986393923832144,0.164398987305358)) ;
#103139=DIRECTION('ref_axis',(0.,0.164398987305358,0.986393923832144)) ;
#103140=DIRECTION('center_axis',(-1.,0.,0.)) ;
#103141=DIRECTION('ref_axis',(0.,0.,1.)) ;
#103142=DIRECTION('',(1.,0.,0.)) ;
#103143=DIRECTION('center_axis',(-1.,0.,0.)) ;
#103144=DIRECTION('ref_axis',(0.,0.,1.)) ;
#103145=DIRECTION('',(-1.,0.,0.)) ;
#103146=DIRECTION('center_axis',(0.,1.,0.)) ;
#103147=DIRECTION('ref_axis',(1.,0.,0.)) ;
#103148=DIRECTION('center_axis',(0.,-0.986393923832144,-0.164398987305358)) ;
#103149=DIRECTION('ref_axis',(0.,-0.164398987305358,0.986393923832144)) ;
#103150=DIRECTION('center_axis',(0.,0.,1.)) ;
#103151=DIRECTION('ref_axis',(1.,0.,0.)) ;
#103152=DIRECTION('center_axis',(-1.,0.,0.)) ;
#103153=DIRECTION('ref_axis',(0.,2.6020852139652E-14,-1.)) ;
#103154=DIRECTION('center_axis',(1.,0.,0.)) ;
#103155=DIRECTION('ref_axis',(0.,0.,-1.)) ;
#103156=DIRECTION('center_axis',(1.,0.,0.)) ;
#103157=DIRECTION('ref_axis',(0.,0.,-1.)) ;
#103158=DIRECTION('',(0.707106781186546,-8.65956056235495E-17,0.707106781186549)) ;
#103159=DIRECTION('center_axis',(1.,0.,0.)) ;
#103160=DIRECTION('ref_axis',(0.,0.,-1.)) ;
#103161=DIRECTION('',(1.,0.,0.)) ;
#103162=DIRECTION('center_axis',(0.,1.,0.)) ;
#103163=DIRECTION('ref_axis',(0.,0.,1.)) ;
#103164=DIRECTION('center_axis',(0.,1.,0.)) ;
#103165=DIRECTION('ref_axis',(0.,0.,1.)) ;
#103166=DIRECTION('',(0.,1.,0.)) ;
#103167=DIRECTION('center_axis',(0.,1.,0.)) ;
#103168=DIRECTION('ref_axis',(0.,0.,1.)) ;
#103169=DIRECTION('',(0.,1.,0.)) ;
#103170=DIRECTION('center_axis',(0.,1.,0.)) ;
#103171=DIRECTION('ref_axis',(0.,0.,1.)) ;
#103172=DIRECTION('',(0.,1.,0.)) ;
#103173=DIRECTION('center_axis',(0.,1.,0.)) ;
#103174=DIRECTION('ref_axis',(0.,0.,1.)) ;
#103175=DIRECTION('',(0.,1.,0.)) ;
#103176=DIRECTION('center_axis',(0.,1.,0.)) ;
#103177=DIRECTION('ref_axis',(0.,0.,1.)) ;
#103178=DIRECTION('',(0.,1.,0.)) ;
#103179=DIRECTION('center_axis',(-1.,0.,0.)) ;
#103180=DIRECTION('ref_axis',(0.,0.,1.)) ;
#103181=DIRECTION('center_axis',(-1.,0.,0.)) ;
#103182=DIRECTION('ref_axis',(0.,0.,1.)) ;
#103183=DIRECTION('center_axis',(-3.56483478381767E-16,0.986393923832144,
0.164398987305358)) ;
#103184=DIRECTION('ref_axis',(4.9167668473396E-33,-0.164398987305358,0.986393923832144)) ;
#103185=DIRECTION('center_axis',(1.,0.,0.)) ;
#103186=DIRECTION('ref_axis',(0.,0.,1.)) ;
#103187=DIRECTION('center_axis',(-4.02631181035926E-15,0.928404294083138,
-0.371571617226061)) ;
#103188=DIRECTION('ref_axis',(1.34987128984705E-31,0.371571617226061,0.928404294083138)) ;
#103189=DIRECTION('center_axis',(0.,0.,1.)) ;
#103190=DIRECTION('ref_axis',(1.,0.,0.)) ;
#103191=DIRECTION('center_axis',(0.,0.,1.)) ;
#103192=DIRECTION('ref_axis',(1.,0.,0.)) ;
#103193=DIRECTION('',(0.,0.,-1.)) ;
#103194=DIRECTION('center_axis',(0.,0.,-1.)) ;
#103195=DIRECTION('ref_axis',(1.,0.,0.)) ;
#103196=DIRECTION('',(0.,0.,1.)) ;
#103197=DIRECTION('center_axis',(0.,-1.,0.)) ;
#103198=DIRECTION('ref_axis',(0.,0.,-1.)) ;
#103199=DIRECTION('center_axis',(0.,-1.,0.)) ;
#103200=DIRECTION('ref_axis',(0.,0.,-1.)) ;
#103201=DIRECTION('center_axis',(-1.,0.,-1.22464679914735E-16)) ;
#103202=DIRECTION('ref_axis',(-1.22464679914735E-16,0.,1.)) ;
#103203=DIRECTION('center_axis',(0.,1.,0.)) ;
#103204=DIRECTION('ref_axis',(0.,0.,-1.)) ;
#103205=DIRECTION('center_axis',(0.,1.,0.)) ;
#103206=DIRECTION('ref_axis',(0.,0.,-1.)) ;
#103207=DIRECTION('center_axis',(1.,0.,0.)) ;
#103208=DIRECTION('ref_axis',(0.,0.,-1.)) ;
#103209=DIRECTION('center_axis',(1.,0.,0.)) ;
#103210=DIRECTION('ref_axis',(0.,0.,-1.)) ;
#103211=DIRECTION('center_axis',(0.,1.,1.22464679914735E-16)) ;
#103212=DIRECTION('ref_axis',(0.,-1.22464679914735E-16,1.)) ;
#103213=DIRECTION('center_axis',(-1.,0.,0.)) ;
#103214=DIRECTION('ref_axis',(0.,0.,-1.)) ;
#103215=DIRECTION('center_axis',(-1.,0.,0.)) ;
#103216=DIRECTION('ref_axis',(0.,0.,1.)) ;
#103217=DIRECTION('center_axis',(-1.,0.,0.)) ;
#103218=DIRECTION('ref_axis',(0.,0.,1.)) ;
#103219=DIRECTION('center_axis',(0.,-1.,1.22464679914735E-16)) ;
#103220=DIRECTION('ref_axis',(0.,-1.22464679914735E-16,-1.)) ;
#103221=DIRECTION('center_axis',(1.,0.,0.)) ;
#103222=DIRECTION('ref_axis',(0.,0.,1.)) ;
#103223=DIRECTION('center_axis',(1.,0.,0.)) ;
#103224=DIRECTION('ref_axis',(0.,0.,1.)) ;
#103225=DIRECTION('center_axis',(-1.,0.,0.)) ;
#103226=DIRECTION('ref_axis',(0.,0.,1.)) ;
#103227=DIRECTION('center_axis',(-1.,0.,0.)) ;
#103228=DIRECTION('ref_axis',(0.,0.,1.)) ;
#103229=DIRECTION('center_axis',(0.,0.986393923832144,-0.164398987305358)) ;
#103230=DIRECTION('ref_axis',(0.,-0.164398987305358,-0.986393923832144)) ;
#103231=DIRECTION('center_axis',(1.,0.,0.)) ;
#103232=DIRECTION('ref_axis',(0.,0.,1.)) ;
#103233=DIRECTION('center_axis',(0.,0.,1.)) ;
#103234=DIRECTION('ref_axis',(1.,0.,0.)) ;
#103235=DIRECTION('center_axis',(0.,1.,0.)) ;
#103236=DIRECTION('ref_axis',(1.,0.,0.)) ;
#103237=DIRECTION('center_axis',(1.,0.,0.)) ;
#103238=DIRECTION('ref_axis',(0.,0.,-1.)) ;
#103239=DIRECTION('center_axis',(0.,0.,-1.)) ;
#103240=DIRECTION('ref_axis',(-1.,0.,0.)) ;
#103241=DIRECTION('center_axis',(0.,-0.986393923832144,0.164398987305358)) ;
#103242=DIRECTION('ref_axis',(0.,0.164398987305358,0.986393923832144)) ;
#103243=DIRECTION('center_axis',(-1.,0.,0.)) ;
#103244=DIRECTION('ref_axis',(0.,0.,1.)) ;
#103245=DIRECTION('',(1.,0.,0.)) ;
#103246=DIRECTION('center_axis',(-1.,0.,0.)) ;
#103247=DIRECTION('ref_axis',(0.,0.,1.)) ;
#103248=DIRECTION('',(-1.,0.,0.)) ;
#103249=DIRECTION('center_axis',(0.,1.,0.)) ;
#103250=DIRECTION('ref_axis',(1.,0.,0.)) ;
#103251=DIRECTION('center_axis',(0.,-0.986393923832144,-0.164398987305358)) ;
#103252=DIRECTION('ref_axis',(0.,-0.164398987305358,0.986393923832144)) ;
#103253=DIRECTION('center_axis',(0.,0.,1.)) ;
#103254=DIRECTION('ref_axis',(1.,0.,0.)) ;
#103255=DIRECTION('center_axis',(-1.,0.,0.)) ;
#103256=DIRECTION('ref_axis',(0.,0.,-1.)) ;
#103257=DIRECTION('center_axis',(1.,0.,0.)) ;
#103258=DIRECTION('ref_axis',(0.,0.,-1.)) ;
#103259=DIRECTION('center_axis',(1.,0.,0.)) ;
#103260=DIRECTION('ref_axis',(0.,0.,-1.)) ;
#103261=DIRECTION('',(0.707106781186546,-8.65956056235495E-17,0.707106781186549)) ;
#103262=DIRECTION('center_axis',(1.,0.,0.)) ;
#103263=DIRECTION('ref_axis',(0.,0.,-1.)) ;
#103264=DIRECTION('',(1.,0.,0.)) ;
#103265=DIRECTION('center_axis',(0.,1.,0.)) ;
#103266=DIRECTION('ref_axis',(0.,0.,1.)) ;
#103267=DIRECTION('center_axis',(0.,1.,0.)) ;
#103268=DIRECTION('ref_axis',(0.,0.,1.)) ;
#103269=DIRECTION('',(0.,1.,0.)) ;
#103270=DIRECTION('center_axis',(0.,1.,0.)) ;
#103271=DIRECTION('ref_axis',(0.,0.,1.)) ;
#103272=DIRECTION('',(0.,1.,0.)) ;
#103273=DIRECTION('center_axis',(0.,1.,0.)) ;
#103274=DIRECTION('ref_axis',(0.,0.,1.)) ;
#103275=DIRECTION('',(0.,1.,0.)) ;
#103276=DIRECTION('center_axis',(0.,1.,0.)) ;
#103277=DIRECTION('ref_axis',(0.,0.,1.)) ;
#103278=DIRECTION('',(0.,1.,0.)) ;
#103279=DIRECTION('center_axis',(0.,1.,0.)) ;
#103280=DIRECTION('ref_axis',(0.,0.,1.)) ;
#103281=DIRECTION('',(0.,1.,0.)) ;
#103282=DIRECTION('center_axis',(-1.,0.,0.)) ;
#103283=DIRECTION('ref_axis',(0.,0.,1.)) ;
#103284=DIRECTION('',(0.,1.,0.)) ;
#103285=DIRECTION('',(0.,0.,1.)) ;
#103286=DIRECTION('',(0.,1.,0.)) ;
#103287=DIRECTION('',(0.,0.,-1.)) ;
#103288=DIRECTION('center_axis',(1.,0.,0.)) ;
#103289=DIRECTION('ref_axis',(0.,0.,1.)) ;
#103290=DIRECTION('',(0.,1.,0.)) ;
#103291=DIRECTION('',(0.,0.,-1.)) ;
#103292=DIRECTION('',(0.,-1.,0.)) ;
#103293=DIRECTION('center_axis',(1.,0.,0.)) ;
#103294=DIRECTION('ref_axis',(0.,0.,1.)) ;
#103295=DIRECTION('',(0.,0.,1.)) ;
#103296=DIRECTION('center_axis',(-3.46944695195361E-15,-1.,0.)) ;
#103297=DIRECTION('ref_axis',(1.,-3.46944695195361E-15,0.)) ;
#103298=DIRECTION('',(-1.,3.46944695195361E-15,1.36784797186593E-30)) ;
#103299=DIRECTION('',(0.,0.,-1.)) ;
#103300=DIRECTION('',(-1.,3.46944695195361E-15,0.)) ;
#103301=DIRECTION('',(0.,0.,1.)) ;
#103302=DIRECTION('center_axis',(-1.,0.,0.)) ;
#103303=DIRECTION('ref_axis',(0.,0.,1.)) ;
#103304=DIRECTION('',(0.,1.,3.94255335449274E-16)) ;
#103305=DIRECTION('',(0.,0.,-1.)) ;
#103306=DIRECTION('',(0.,1.,0.)) ;
#103307=DIRECTION('',(0.,0.,1.)) ;
#103308=DIRECTION('center_axis',(0.,1.,0.)) ;
#103309=DIRECTION('ref_axis',(0.,0.,1.)) ;
#103310=DIRECTION('',(1.,0.,0.)) ;
#103311=DIRECTION('',(0.,0.,-1.)) ;
#103312=DIRECTION('',(1.,0.,0.)) ;
#103313=DIRECTION('',(0.,0.,1.)) ;
#103314=DIRECTION('center_axis',(0.,0.,-1.)) ;
#103315=DIRECTION('ref_axis',(-1.,0.,0.)) ;
#103316=DIRECTION('',(0.,0.,-1.)) ;
#103317=DIRECTION('center_axis',(0.,3.94255335449274E-16,-1.)) ;
#103318=DIRECTION('ref_axis',(0.,-1.,-3.94255335449274E-16)) ;
#103319=DIRECTION('center_axis',(0.,0.,-1.)) ;
#103320=DIRECTION('ref_axis',(1.,0.,0.)) ;
#103321=DIRECTION('center_axis',(0.,0.,1.)) ;
#103322=DIRECTION('ref_axis',(1.,0.,0.)) ;
#103323=DIRECTION('center_axis',(0.,3.94255335449274E-16,-1.)) ;
#103324=DIRECTION('ref_axis',(0.,-1.,-3.94255335449274E-16)) ;
#103325=DIRECTION('center_axis',(0.,0.,1.)) ;
#103326=DIRECTION('ref_axis',(1.,0.,0.)) ;
#103327=DIRECTION('center_axis',(0.,0.,1.)) ;
#103328=DIRECTION('ref_axis',(1.,0.,0.)) ;
#103329=DIRECTION('center_axis',(0.,3.94255335449274E-16,-1.)) ;
#103330=DIRECTION('ref_axis',(-4.33680868994204E-15,-1.,-3.94255335449274E-16)) ;
#103331=DIRECTION('center_axis',(0.,0.,1.)) ;
#103332=DIRECTION('ref_axis',(1.,0.,0.)) ;
#103333=DIRECTION('center_axis',(0.,0.,-1.)) ;
#103334=DIRECTION('ref_axis',(-1.,0.,0.)) ;
#103335=DIRECTION('center_axis',(0.,3.94255335449274E-16,-1.)) ;
#103336=DIRECTION('ref_axis',(3.46944695195361E-14,-1.,-3.94255335449274E-16)) ;
#103337=DIRECTION('',(0.,0.,1.)) ;
#103338=DIRECTION('center_axis',(0.,0.,1.)) ;
#103339=DIRECTION('ref_axis',(1.,0.,0.)) ;
#103340=DIRECTION('',(0.,0.,1.)) ;
#103341=DIRECTION('center_axis',(0.,0.,-1.)) ;
#103342=DIRECTION('ref_axis',(1.,0.,0.)) ;
#103343=DIRECTION('center_axis',(-1.,0.,0.)) ;
#103344=DIRECTION('ref_axis',(0.,0.,1.)) ;
#103345=DIRECTION('center_axis',(-1.,0.,0.)) ;
#103346=DIRECTION('ref_axis',(0.,0.,1.)) ;
#103347=DIRECTION('',(0.,0.,-1.)) ;
#103348=DIRECTION('center_axis',(-1.,0.,0.)) ;
#103349=DIRECTION('ref_axis',(0.,0.,1.)) ;
#103350=DIRECTION('',(0.,0.,1.)) ;
#103351=DIRECTION('center_axis',(-2.09002828430941E-16,1.,0.)) ;
#103352=DIRECTION('ref_axis',(-1.,-2.09002828430941E-16,0.)) ;
#103353=DIRECTION('',(1.,2.09002828430941E-16,0.)) ;
#103354=DIRECTION('',(0.,0.,-1.)) ;
#103355=DIRECTION('',(1.,2.09002828430941E-16,0.)) ;
#103356=DIRECTION('',(0.,0.,1.)) ;
#103357=DIRECTION('center_axis',(1.0450141421547E-16,-1.,0.)) ;
#103358=DIRECTION('ref_axis',(1.,1.0450141421547E-16,0.)) ;
#103359=DIRECTION('',(0.,0.,-1.)) ;
#103360=DIRECTION('',(-1.,-1.0450141421547E-16,1.7416902369245E-17)) ;
#103361=DIRECTION('',(0.,0.,1.)) ;
#103362=DIRECTION('',(1.,1.0450141421547E-16,1.7416902369245E-17)) ;
#103363=DIRECTION('center_axis',(0.,1.,0.)) ;
#103364=DIRECTION('ref_axis',(0.,0.,1.)) ;
#103365=DIRECTION('',(0.422618261740697,0.,-0.906307787036651)) ;
#103366=DIRECTION('center_axis',(-1.,0.,0.)) ;
#103367=DIRECTION('ref_axis',(0.,0.,1.)) ;
#103368=DIRECTION('',(0.,0.986393923832144,-0.164398987305357)) ;
#103369=DIRECTION('',(0.,0.,1.)) ;
#103370=DIRECTION('',(0.,1.,0.)) ;
#103371=DIRECTION('',(0.,0.,-1.)) ;
#103372=DIRECTION('center_axis',(1.,0.,0.)) ;
#103373=DIRECTION('ref_axis',(0.,4.33680868994202E-15,1.)) ;
#103374=DIRECTION('center_axis',(1.,0.,0.)) ;
#103375=DIRECTION('ref_axis',(0.,0.,1.)) ;
#103376=DIRECTION('center_axis',(1.,0.,0.)) ;
#103377=DIRECTION('ref_axis',(0.,0.,1.)) ;
#103378=DIRECTION('',(0.,0.,-1.)) ;
#103379=DIRECTION('center_axis',(1.,0.,0.)) ;
#103380=DIRECTION('ref_axis',(0.,-4.33680868994202E-15,1.)) ;
#103381=DIRECTION('center_axis',(1.,0.,0.)) ;
#103382=DIRECTION('ref_axis',(0.,8.88178419700125E-16,1.)) ;
#103383=DIRECTION('center_axis',(1.,0.,0.)) ;
#103384=DIRECTION('ref_axis',(0.,6.50521303491304E-15,1.)) ;
#103385=DIRECTION('',(0.,0.,-1.)) ;
#103386=DIRECTION('',(0.,1.,0.)) ;
#103387=DIRECTION('',(0.,0.,1.)) ;
#103388=DIRECTION('',(0.,-0.986393923832144,-0.164398987305357)) ;
#103389=DIRECTION('center_axis',(1.,0.,0.)) ;
#103390=DIRECTION('ref_axis',(0.,0.,1.)) ;
#103391=DIRECTION('',(0.,0.,1.)) ;
#103392=DIRECTION('',(0.,0.986393923832144,-0.164398987305357)) ;
#103393=DIRECTION('',(0.,0.,1.)) ;
#103394=DIRECTION('',(0.,-0.986393923832144,-0.164398987305357)) ;
#103395=DIRECTION('center_axis',(1.,0.,0.)) ;
#103396=DIRECTION('ref_axis',(0.,0.,1.)) ;
#103397=DIRECTION('',(0.,0.,1.)) ;
#103398=DIRECTION('center_axis',(1.0450141421547E-16,-1.,0.)) ;
#103399=DIRECTION('ref_axis',(1.,1.0450141421547E-16,0.)) ;
#103400=DIRECTION('',(-1.,-1.0450141421547E-16,1.7416902369245E-17)) ;
#103401=DIRECTION('',(0.,0.,1.)) ;
#103402=DIRECTION('',(-1.,-1.0450141421547E-16,0.)) ;
#103403=DIRECTION('',(0.,0.,-1.)) ;
#103404=DIRECTION('center_axis',(-0.876215908676647,-0.481918749772156,
0.)) ;
#103405=DIRECTION('ref_axis',(0.481918749772156,-0.876215908676647,0.)) ;
#103406=DIRECTION('',(-0.481918749772156,0.876215908676647,0.)) ;
#103407=DIRECTION('',(0.,0.,-1.)) ;
#103408=DIRECTION('center_axis',(-0.87621590867663,-0.481918749772186,-1.71185066180799E-15)) ;
#103409=DIRECTION('ref_axis',(0.436954455877847,-0.794462647050564,-0.421781822664167)) ;
#103410=DIRECTION('',(0.,0.,-1.)) ;
#103411=DIRECTION('center_axis',(-0.876215908676628,-0.48191874977219,-1.569734757823E-14)) ;
#103412=DIRECTION('ref_axis',(0.436954455972081,-0.794462647221906,0.421781822243805)) ;
#103413=DIRECTION('',(0.,0.,-1.)) ;
#103414=DIRECTION('center_axis',(-0.876215908676574,-0.481918749772289,
3.39624711488767E-14)) ;
#103415=DIRECTION('ref_axis',(0.436954455864899,-0.794462647026833,-0.421781822722279)) ;
#103416=DIRECTION('',(0.,0.,-1.)) ;
#103417=DIRECTION('center_axis',(-0.87621590867663,-0.481918749772186,-9.62512258910975E-15)) ;
#103418=DIRECTION('ref_axis',(0.436954455963938,-0.794462647207104,0.421781822280121)) ;
#103419=DIRECTION('',(0.,0.,-1.)) ;
#103420=DIRECTION('',(-0.481918749772156,0.876215908676647,0.)) ;
#103421=DIRECTION('',(0.,0.,1.)) ;
#103422=DIRECTION('center_axis',(-0.876215908676647,-0.481918749772156,
0.)) ;
#103423=DIRECTION('ref_axis',(0.481918749772156,-0.876215908676647,0.)) ;
#103424=DIRECTION('',(0.,0.,-1.)) ;
#103425=DIRECTION('',(-0.481918749772156,0.876215908676647,0.)) ;
#103426=DIRECTION('',(-0.481918749772156,0.876215908676647,0.)) ;
#103427=DIRECTION('center_axis',(-1.,0.,0.)) ;
#103428=DIRECTION('ref_axis',(0.,0.,1.)) ;
#103429=DIRECTION('',(0.,1.,0.)) ;
#103430=DIRECTION('',(0.,0.,1.)) ;
#103431=DIRECTION('',(0.,1.,0.)) ;
#103432=DIRECTION('',(0.,-1.,-3.94255335449274E-16)) ;
#103433=DIRECTION('center_axis',(0.,-1.,0.)) ;
#103434=DIRECTION('ref_axis',(0.,0.,-1.)) ;
#103435=DIRECTION('',(0.,0.,-1.)) ;
#103436=DIRECTION('',(-1.,0.,0.)) ;
#103437=DIRECTION('',(0.,0.,1.)) ;
#103438=DIRECTION('',(-1.,0.,0.)) ;
#103439=DIRECTION('center_axis',(0.,1.,0.)) ;
#103440=DIRECTION('ref_axis',(0.,0.,-1.)) ;
#103441=DIRECTION('',(2.16840434497101E-16,0.,1.)) ;
#103442=DIRECTION('center_axis',(0.,1.,0.)) ;
#103443=DIRECTION('ref_axis',(0.,0.,-1.)) ;
#103444=DIRECTION('',(-1.,0.,1.73472347597681E-16)) ;
#103445=DIRECTION('center_axis',(0.,1.,0.)) ;
#103446=DIRECTION('ref_axis',(0.,0.,-1.)) ;
#103447=DIRECTION('',(-2.16840434497101E-16,0.,-1.)) ;
#103448=DIRECTION('center_axis',(0.,1.,0.)) ;
#103449=DIRECTION('ref_axis',(0.,0.,-1.)) ;
#103450=DIRECTION('',(1.,0.,-1.73472347597681E-16)) ;
#103451=DIRECTION('center_axis',(0.,1.,0.)) ;
#103452=DIRECTION('ref_axis',(0.,0.,-1.)) ;
#103453=DIRECTION('',(2.16840434497101E-16,0.,1.)) ;
#103454=DIRECTION('center_axis',(0.,1.,0.)) ;
#103455=DIRECTION('ref_axis',(0.,0.,-1.)) ;
#103456=DIRECTION('',(-1.,0.,1.73472347597681E-16)) ;
#103457=DIRECTION('center_axis',(0.,1.,0.)) ;
#103458=DIRECTION('ref_axis',(0.,0.,-1.)) ;
#103459=DIRECTION('',(-2.16840434497101E-16,0.,-1.)) ;
#103460=DIRECTION('center_axis',(0.,1.,0.)) ;
#103461=DIRECTION('ref_axis',(0.,0.,-1.)) ;
#103462=DIRECTION('',(1.,0.,-1.73472347597681E-16)) ;
#103463=DIRECTION('center_axis',(1.,0.,0.)) ;
#103464=DIRECTION('ref_axis',(0.,0.,-1.)) ;
#103465=DIRECTION('',(0.,0.,-1.)) ;
#103466=DIRECTION('',(0.,-1.,0.)) ;
#103467=DIRECTION('',(0.,0.,1.)) ;
#103468=DIRECTION('',(0.,-1.,0.)) ;
#103469=DIRECTION('center_axis',(0.,1.,0.)) ;
#103470=DIRECTION('ref_axis',(0.,0.,1.)) ;
#103471=DIRECTION('',(0.,0.,-1.)) ;
#103472=DIRECTION('',(1.,0.,0.)) ;
#103473=DIRECTION('',(1.,0.,0.)) ;
#103474=DIRECTION('center_axis',(0.98058067569092,-0.196116135138184,0.)) ;
#103475=DIRECTION('ref_axis',(0.196116135138184,0.98058067569092,0.)) ;
#103476=DIRECTION('',(-0.196116135138184,-0.98058067569092,0.)) ;
#103477=DIRECTION('',(0.,0.,1.)) ;
#103478=DIRECTION('',(-0.196116135138184,-0.98058067569092,0.)) ;
#103479=DIRECTION('center_axis',(1.,0.,0.)) ;
#103480=DIRECTION('ref_axis',(0.,0.,-1.)) ;
#103481=DIRECTION('',(0.,0.,-1.)) ;
#103482=DIRECTION('',(0.,-1.,0.)) ;
#103483=DIRECTION('',(0.,0.,1.)) ;
#103484=DIRECTION('',(0.,-1.,0.)) ;
#103485=DIRECTION('',(0.,0.,1.)) ;
#103486=DIRECTION('',(0.,-1.,0.)) ;
#103487=DIRECTION('',(0.,0.,-1.)) ;
#103488=DIRECTION('',(0.,1.,0.)) ;
#103489=DIRECTION('',(0.,0.,1.)) ;
#103490=DIRECTION('',(0.,-1.,0.)) ;
#103491=DIRECTION('',(0.,0.,-1.)) ;
#103492=DIRECTION('',(0.,1.,0.)) ;
#103493=DIRECTION('center_axis',(0.,1.,0.)) ;
#103494=DIRECTION('ref_axis',(0.,0.,1.)) ;
#103495=DIRECTION('',(0.,0.,-1.)) ;
#103496=DIRECTION('',(1.,0.,0.)) ;
#103497=DIRECTION('',(0.,0.,1.)) ;
#103498=DIRECTION('',(1.,0.,0.)) ;
#103499=DIRECTION('center_axis',(0.,-1.,0.)) ;
#103500=DIRECTION('ref_axis',(0.,0.,1.)) ;
#103501=DIRECTION('',(0.,0.,1.)) ;
#103502=DIRECTION('center_axis',(0.,-1.,0.)) ;
#103503=DIRECTION('ref_axis',(0.,0.,1.)) ;
#103504=DIRECTION('',(1.,0.,1.73472347597681E-16)) ;
#103505=DIRECTION('center_axis',(0.,-1.,0.)) ;
#103506=DIRECTION('ref_axis',(0.,0.,1.)) ;
#103507=DIRECTION('',(4.33680868994202E-16,0.,-1.)) ;
#103508=DIRECTION('center_axis',(0.,-1.,0.)) ;
#103509=DIRECTION('ref_axis',(0.,0.,1.)) ;
#103510=DIRECTION('',(-1.,0.,1.73472347597681E-16)) ;
#103511=DIRECTION('center_axis',(0.,-1.,0.)) ;
#103512=DIRECTION('ref_axis',(0.,0.,1.)) ;
#103513=DIRECTION('',(0.,0.,1.)) ;
#103514=DIRECTION('center_axis',(0.,-1.,0.)) ;
#103515=DIRECTION('ref_axis',(0.,0.,1.)) ;
#103516=DIRECTION('',(1.,0.,1.73472347597681E-16)) ;
#103517=DIRECTION('center_axis',(0.,-1.,0.)) ;
#103518=DIRECTION('ref_axis',(0.,0.,1.)) ;
#103519=DIRECTION('',(4.33680868994202E-16,0.,-1.)) ;
#103520=DIRECTION('center_axis',(0.,-1.,0.)) ;
#103521=DIRECTION('ref_axis',(0.,0.,1.)) ;
#103522=DIRECTION('',(-1.,0.,1.73472347597681E-16)) ;
#103523=DIRECTION('center_axis',(-1.,6.93889390390723E-16,0.)) ;
#103524=DIRECTION('ref_axis',(-6.93889390390723E-16,-1.,0.)) ;
#103525=DIRECTION('',(0.,0.,-1.)) ;
#103526=DIRECTION('',(6.93889390390723E-16,1.,0.)) ;
#103527=DIRECTION('',(0.,0.,1.)) ;
#103528=DIRECTION('',(6.93889390390723E-16,1.,0.)) ;
#103529=DIRECTION('center_axis',(0.,1.,0.)) ;
#103530=DIRECTION('ref_axis',(0.,0.,1.)) ;
#103531=DIRECTION('',(0.,0.,1.)) ;
#103532=DIRECTION('',(1.,0.,0.)) ;
#103533=DIRECTION('',(0.,0.,-1.)) ;
#103534=DIRECTION('',(1.,0.,0.)) ;
#103535=DIRECTION('',(0.,0.,1.)) ;
#103536=DIRECTION('',(0.,0.,1.)) ;
#103537=DIRECTION('center_axis',(-1.,0.,0.)) ;
#103538=DIRECTION('ref_axis',(0.,0.,1.)) ;
#103539=DIRECTION('',(0.,1.,0.)) ;
#103540=DIRECTION('',(0.,0.,-1.)) ;
#103541=DIRECTION('center_axis',(-1.,0.,0.)) ;
#103542=DIRECTION('ref_axis',(0.,0.,1.)) ;
#103543=DIRECTION('',(0.,0.,1.)) ;
#103544=DIRECTION('center_axis',(-2.09002828430941E-16,1.,0.)) ;
#103545=DIRECTION('ref_axis',(-1.,-2.09002828430941E-16,0.)) ;
#103546=DIRECTION('',(-1.,-2.09002828430941E-16,0.)) ;
#103547=DIRECTION('',(0.,0.,-1.)) ;
#103548=DIRECTION('',(1.,2.09002828430941E-16,0.)) ;
#103549=DIRECTION('',(0.,0.,1.)) ;
#103550=DIRECTION('center_axis',(0.,0.,1.)) ;
#103551=DIRECTION('ref_axis',(1.,0.,0.)) ;
#103552=DIRECTION('center_axis',(0.,0.,1.)) ;
#103553=DIRECTION('ref_axis',(1.,0.,0.)) ;
#103554=DIRECTION('center_axis',(0.,0.,1.)) ;
#103555=DIRECTION('ref_axis',(1.,0.,0.)) ;
#103556=DIRECTION('center_axis',(0.,0.,1.)) ;
#103557=DIRECTION('ref_axis',(1.,0.,0.)) ;
#103558=DIRECTION('center_axis',(0.,0.,1.)) ;
#103559=DIRECTION('ref_axis',(1.,0.,0.)) ;
#103560=DIRECTION('center_axis',(0.,0.,1.)) ;
#103561=DIRECTION('ref_axis',(1.,0.,0.)) ;
#103562=DIRECTION('center_axis',(0.,0.,1.)) ;
#103563=DIRECTION('ref_axis',(1.,0.,0.)) ;
#103564=DIRECTION('center_axis',(0.,0.,-1.)) ;
#103565=DIRECTION('ref_axis',(1.,0.,0.)) ;
#103566=DIRECTION('center_axis',(0.,0.,1.)) ;
#103567=DIRECTION('ref_axis',(1.,0.,0.)) ;
#103568=DIRECTION('center_axis',(0.,0.,-1.)) ;
#103569=DIRECTION('ref_axis',(1.,0.,0.)) ;
#103570=DIRECTION('center_axis',(0.,0.,1.)) ;
#103571=DIRECTION('ref_axis',(1.,0.,0.)) ;
#103572=DIRECTION('center_axis',(0.,0.,1.)) ;
#103573=DIRECTION('ref_axis',(1.,0.,0.)) ;
#103574=DIRECTION('center_axis',(0.,0.,-1.)) ;
#103575=DIRECTION('ref_axis',(1.,0.,0.)) ;
#103576=DIRECTION('center_axis',(0.,0.,-1.)) ;
#103577=DIRECTION('ref_axis',(1.,0.,0.)) ;
#103578=DIRECTION('center_axis',(0.,0.,1.)) ;
#103579=DIRECTION('ref_axis',(1.,0.,0.)) ;
#103580=DIRECTION('center_axis',(0.,0.,1.)) ;
#103581=DIRECTION('ref_axis',(1.,0.,0.)) ;
#103582=DIRECTION('',(-0.664363838829919,0.74740931868366,0.)) ;
#103583=DIRECTION('',(0.,-1.,0.)) ;
#103584=DIRECTION('',(0.894427190999917,0.447213595499956,0.)) ;
#103585=DIRECTION('',(0.,1.,0.)) ;
#103586=DIRECTION('center_axis',(0.,0.,-1.)) ;
#103587=DIRECTION('ref_axis',(-1.,0.,0.)) ;
#103588=DIRECTION('',(-0.894427190999917,-0.447213595499956,0.)) ;
#103589=DIRECTION('',(0.,1.,0.)) ;
#103590=DIRECTION('',(0.664363838829919,-0.74740931868366,0.)) ;
#103591=DIRECTION('',(0.,-1.,0.)) ;
#103592=DIRECTION('center_axis',(-0.23745309047699,0.,-0.971399006496778)) ;
#103593=DIRECTION('ref_axis',(-0.971399006496778,0.,0.23745309047699)) ;
#103594=DIRECTION('center_axis',(-0.237453090476991,1.73471514883906E-15,
-0.971399006496777)) ;
#103595=DIRECTION('ref_axis',(0.921799787670948,-0.315455332293223,-0.225328836986233)) ;
#103596=DIRECTION('',(0.971399006496777,0.,-0.23745309047699)) ;
#103597=DIRECTION('',(0.,-1.,0.)) ;
#103598=DIRECTION('',(-0.971399006496777,0.,0.23745309047699)) ;
#103599=DIRECTION('center_axis',(-0.237453090476988,-5.68535949803261E-15,
-0.971399006496778)) ;
#103600=DIRECTION('ref_axis',(0.954559354253041,0.18539258117777,-0.233336731039631)) ;
#103601=DIRECTION('',(-0.873786407766991,-0.436893203883493,0.213592233009709)) ;
#103602=DIRECTION('',(0.,1.,0.)) ;
#103603=DIRECTION('',(0.655772517804503,-0.737744082530068,-0.160299948796656)) ;
#103604=DIRECTION('center_axis',(-1.,0.,0.)) ;
#103605=DIRECTION('ref_axis',(0.,0.,1.)) ;
#103606=DIRECTION('',(0.,-1.,0.)) ;
#103607=DIRECTION('center_axis',(-1.,-6.70078870827233E-15,-6.50913949396058E-15)) ;
#103608=DIRECTION('ref_axis',(6.50913949395829E-15,3.4174057398699E-13,
-1.)) ;
#103609=DIRECTION('',(0.,0.,-1.)) ;
#103610=DIRECTION('center_axis',(-1.,6.70078870827231E-15,-6.50913949396055E-15)) ;
#103611=DIRECTION('ref_axis',(6.50913949394042E-15,-3.00413806900314E-12,
-1.)) ;
#103612=DIRECTION('center_axis',(-1.,6.70078870827234E-15,6.50913949396058E-15)) ;
#103613=DIRECTION('ref_axis',(-6.50913949393696E-15,3.524696385192E-12,
-1.)) ;
#103614=DIRECTION('',(0.,0.,-1.)) ;
#103615=DIRECTION('center_axis',(-1.,6.70078870827234E-15,-6.50913949396058E-15)) ;
#103616=DIRECTION('ref_axis',(6.50913949393646E-15,-3.60019720967755E-12,
-1.)) ;
#103617=DIRECTION('center_axis',(-0.23745309047699,0.,0.971399006496778)) ;
#103618=DIRECTION('ref_axis',(0.971399006496778,0.,0.23745309047699)) ;
#103619=DIRECTION('center_axis',(-0.237453090476982,-3.00511859181728E-14,
0.971399006496779)) ;
#103620=DIRECTION('ref_axis',(0.954559354252495,0.185392581180749,0.233336731039496)) ;
#103621=DIRECTION('',(0.971399006496777,0.,0.23745309047699)) ;
#103622=DIRECTION('',(-0.971399006496777,0.,-0.23745309047699)) ;
#103623=DIRECTION('center_axis',(-0.237453090476993,-4.21287964718113E-15,
0.971399006496777)) ;
#103624=DIRECTION('ref_axis',(0.921799787669916,-0.315455332296417,0.225328836985981)) ;
#103625=DIRECTION('',(-0.655772517804503,0.737744082530068,-0.160299948796656)) ;
#103626=DIRECTION('',(0.,-1.,0.)) ;
#103627=DIRECTION('',(0.873786407766991,0.436893203883493,0.213592233009709)) ;
#103628=DIRECTION('center_axis',(0.,1.,0.)) ;
#103629=DIRECTION('ref_axis',(0.,0.,1.)) ;
#103630=DIRECTION('',(-0.971399006496777,0.,0.23745309047699)) ;
#103631=DIRECTION('',(0.,0.,-1.)) ;
#103632=DIRECTION('',(0.971399006496777,0.,0.23745309047699)) ;
#103633=DIRECTION('center_axis',(0.,1.,0.)) ;
#103634=DIRECTION('ref_axis',(0.,0.,1.)) ;
#103635=DIRECTION('',(-0.971399006496777,0.,-0.23745309047699)) ;
#103636=DIRECTION('',(0.,0.,1.)) ;
#103637=DIRECTION('',(0.971399006496777,0.,-0.23745309047699)) ;
#103638=DIRECTION('center_axis',(-0.447213595499956,0.894427190999917,0.)) ;
#103639=DIRECTION('ref_axis',(0.,0.,-1.)) ;
#103640=DIRECTION('',(0.,0.,-1.)) ;
#103641=DIRECTION('',(-0.873786407766991,-0.436893203883493,-0.213592233009709)) ;
#103642=DIRECTION('',(-0.894427190999917,-0.447213595499956,0.)) ;
#103643=DIRECTION('',(0.,0.,1.)) ;
#103644=DIRECTION('',(0.894427190999917,0.447213595499956,0.)) ;
#103645=DIRECTION('',(0.873786407766991,0.436893203883493,-0.213592233009709)) ;
#103646=DIRECTION('center_axis',(0.74740931868366,0.664363838829919,0.)) ;
#103647=DIRECTION('ref_axis',(0.,0.,1.)) ;
#103648=DIRECTION('',(0.,0.,-1.)) ;
#103649=DIRECTION('',(0.664363838829919,-0.74740931868366,0.)) ;
#103650=DIRECTION('',(0.655772517804503,-0.737744082530068,0.160299948796656)) ;
#103651=DIRECTION('',(0.,0.,1.)) ;
#103652=DIRECTION('',(-0.655772517804503,0.737744082530068,0.160299948796656)) ;
#103653=DIRECTION('',(-0.664363838829919,0.74740931868366,0.)) ;
#103654=DIRECTION('center_axis',(1.,0.,4.33680868994202E-16)) ;
#103655=DIRECTION('ref_axis',(4.33680868994202E-16,0.,-1.)) ;
#103656=DIRECTION('',(0.,1.,0.)) ;
#103657=DIRECTION('',(4.33680868994202E-16,0.,-1.)) ;
#103658=DIRECTION('',(0.,-1.,0.)) ;
#103659=DIRECTION('',(-4.33680868994202E-16,0.,1.)) ;
#103660=DIRECTION('center_axis',(-1.73472347597681E-16,0.,-1.)) ;
#103661=DIRECTION('ref_axis',(-1.,0.,1.73472347597681E-16)) ;
#103662=DIRECTION('',(-1.,0.,1.73472347597681E-16)) ;
#103663=DIRECTION('',(0.,-1.,0.)) ;
#103664=DIRECTION('',(1.,0.,-1.73472347597681E-16)) ;
#103665=DIRECTION('',(0.,1.,0.)) ;
#103666=DIRECTION('center_axis',(-1.,0.,0.)) ;
#103667=DIRECTION('ref_axis',(0.,0.,1.)) ;
#103668=DIRECTION('',(0.,0.,1.)) ;
#103669=DIRECTION('',(0.,-1.,0.)) ;
#103670=DIRECTION('',(0.,0.,-1.)) ;
#103671=DIRECTION('',(0.,1.,0.)) ;
#103672=DIRECTION('center_axis',(-1.73472347597681E-16,0.,1.)) ;
#103673=DIRECTION('ref_axis',(1.,0.,1.73472347597681E-16)) ;
#103674=DIRECTION('',(0.,1.,0.)) ;
#103675=DIRECTION('',(1.,0.,1.73472347597681E-16)) ;
#103676=DIRECTION('',(0.,-1.,0.)) ;
#103677=DIRECTION('',(-1.,0.,-1.73472347597681E-16)) ;
#103678=DIRECTION('center_axis',(0.,-1.,0.)) ;
#103679=DIRECTION('ref_axis',(0.,0.,-1.)) ;
#103680=DIRECTION('',(-1.,0.,-1.73472347597681E-16)) ;
#103681=DIRECTION('',(0.,0.,-1.)) ;
#103682=DIRECTION('',(1.,0.,-1.73472347597681E-16)) ;
#103683=DIRECTION('',(-4.33680868994202E-16,0.,1.)) ;
#103684=DIRECTION('',(1.,0.,0.)) ;
#103685=DIRECTION('center_axis',(0.,-1.,0.)) ;
#103686=DIRECTION('ref_axis',(0.,0.,-1.)) ;
#103687=DIRECTION('',(0.,0.,-1.)) ;
#103688=DIRECTION('center_axis',(0.,-1.,0.)) ;
#103689=DIRECTION('ref_axis',(0.,0.,-1.)) ;
#103690=DIRECTION('',(-1.,0.,0.)) ;
#103691=DIRECTION('center_axis',(0.,-1.,0.)) ;
#103692=DIRECTION('ref_axis',(0.,0.,1.)) ;
#103693=DIRECTION('',(0.,0.,1.)) ;
#103694=DIRECTION('center_axis',(0.,-1.,0.)) ;
#103695=DIRECTION('ref_axis',(0.,0.,-1.)) ;
#103696=DIRECTION('center_axis',(0.,-1.,0.)) ;
#103697=DIRECTION('ref_axis',(0.,0.,-1.)) ;
#103698=DIRECTION('center_axis',(0.,-1.,0.)) ;
#103699=DIRECTION('ref_axis',(0.,0.,-1.)) ;
#103700=DIRECTION('',(0.,-1.,0.)) ;
#103701=DIRECTION('',(0.,-1.,0.)) ;
#103702=DIRECTION('center_axis',(0.,0.,-1.)) ;
#103703=DIRECTION('ref_axis',(-1.,0.,0.)) ;
#103704=DIRECTION('',(1.,0.,0.)) ;
#103705=DIRECTION('',(0.,-1.,0.)) ;
#103706=DIRECTION('center_axis',(0.,-1.,0.)) ;
#103707=DIRECTION('ref_axis',(0.,0.,-1.)) ;
#103708=DIRECTION('center_axis',(0.,-1.,0.)) ;
#103709=DIRECTION('ref_axis',(0.,0.,-1.)) ;
#103710=DIRECTION('',(0.,-1.,0.)) ;
#103711=DIRECTION('center_axis',(-1.,0.,0.)) ;
#103712=DIRECTION('ref_axis',(0.,0.,1.)) ;
#103713=DIRECTION('',(0.,0.,-1.)) ;
#103714=DIRECTION('',(0.,-1.,0.)) ;
#103715=DIRECTION('center_axis',(0.,-1.,0.)) ;
#103716=DIRECTION('ref_axis',(0.,0.,-1.)) ;
#103717=DIRECTION('center_axis',(0.,-1.,0.)) ;
#103718=DIRECTION('ref_axis',(0.,0.,-1.)) ;
#103719=DIRECTION('',(0.,-1.,0.)) ;
#103720=DIRECTION('center_axis',(0.,0.,1.)) ;
#103721=DIRECTION('ref_axis',(1.,0.,0.)) ;
#103722=DIRECTION('',(-1.,0.,0.)) ;
#103723=DIRECTION('',(0.,-1.,0.)) ;
#103724=DIRECTION('center_axis',(0.,-1.,0.)) ;
#103725=DIRECTION('ref_axis',(0.,0.,-1.)) ;
#103726=DIRECTION('center_axis',(0.,-1.,0.)) ;
#103727=DIRECTION('ref_axis',(0.,0.,1.)) ;
#103728=DIRECTION('',(0.,-1.,0.)) ;
#103729=DIRECTION('center_axis',(1.,0.,0.)) ;
#103730=DIRECTION('ref_axis',(0.,0.,-1.)) ;
#103731=DIRECTION('',(0.,0.,1.)) ;
#103732=DIRECTION('center_axis',(0.,-1.,0.)) ;
#103733=DIRECTION('ref_axis',(0.,0.,-1.)) ;
#103734=DIRECTION('center_axis',(0.,1.,0.)) ;
#103735=DIRECTION('ref_axis',(0.,0.,1.)) ;
#103736=DIRECTION('',(-0.422618261740697,0.,0.906307787036651)) ;
#103737=DIRECTION('center_axis',(0.906307787036651,0.,0.422618261740697)) ;
#103738=DIRECTION('ref_axis',(0.422618261740697,0.,-0.906307787036651)) ;
#103739=DIRECTION('',(-0.422618261740697,0.,0.906307787036651)) ;
#103740=DIRECTION('',(0.422618261740697,0.,-0.906307787036651)) ;
#103741=DIRECTION('center_axis',(-0.906307787036651,0.,-0.422618261740697)) ;
#103742=DIRECTION('ref_axis',(-0.422618261740697,0.,0.906307787036651)) ;
#103743=DIRECTION('',(0.422618261740697,0.,-0.906307787036651)) ;
#103744=DIRECTION('',(-0.422618261740697,0.,0.906307787036651)) ;
#103745=DIRECTION('center_axis',(0.,1.,0.)) ;
#103746=DIRECTION('ref_axis',(0.,0.,1.)) ;
#103747=DIRECTION('',(-0.422618261740697,0.,0.906307787036651)) ;
#103748=DIRECTION('',(0.422618261740697,0.,-0.906307787036651)) ;
#103749=DIRECTION('center_axis',(1.,0.,-2.16840434497101E-16)) ;
#103750=DIRECTION('ref_axis',(-2.16840434497101E-16,0.,-1.)) ;
#103751=DIRECTION('',(2.16840434497101E-16,0.,1.)) ;
#103752=DIRECTION('',(0.,1.,0.)) ;
#103753=DIRECTION('',(-2.16840434497101E-16,0.,-1.)) ;
#103754=DIRECTION('',(0.,-1.,0.)) ;
#103755=DIRECTION('center_axis',(1.73472347597681E-16,0.,1.)) ;
#103756=DIRECTION('ref_axis',(1.,0.,-1.73472347597681E-16)) ;
#103757=DIRECTION('',(0.,-1.,0.)) ;
#103758=DIRECTION('',(-1.,0.,1.73472347597681E-16)) ;
#103759=DIRECTION('',(0.,1.,0.)) ;
#103760=DIRECTION('',(1.,0.,-1.73472347597681E-16)) ;
#103761=DIRECTION('center_axis',(-1.,0.,2.16840434497101E-16)) ;
#103762=DIRECTION('ref_axis',(2.16840434497101E-16,0.,1.)) ;
#103763=DIRECTION('',(0.,-1.,0.)) ;
#103764=DIRECTION('',(-2.16840434497101E-16,0.,-1.)) ;
#103765=DIRECTION('',(0.,1.,0.)) ;
#103766=DIRECTION('',(2.16840434497101E-16,0.,1.)) ;
#103767=DIRECTION('center_axis',(-1.73472347597681E-16,0.,-1.)) ;
#103768=DIRECTION('ref_axis',(-1.,0.,1.73472347597681E-16)) ;
#103769=DIRECTION('',(1.,0.,-1.73472347597681E-16)) ;
#103770=DIRECTION('',(0.,1.,0.)) ;
#103771=DIRECTION('',(-1.,0.,1.73472347597681E-16)) ;
#103772=DIRECTION('',(0.,-1.,0.)) ;
#103773=DIRECTION('center_axis',(0.,1.,0.)) ;
#103774=DIRECTION('ref_axis',(0.,0.,1.)) ;
#103775=DIRECTION('',(1.,0.,-1.73472347597681E-16)) ;
#103776=DIRECTION('',(-2.16840434497101E-16,0.,-1.)) ;
#103777=DIRECTION('',(-1.,0.,1.73472347597681E-16)) ;
#103778=DIRECTION('',(2.16840434497101E-16,0.,1.)) ;
#103779=DIRECTION('',(1.,0.,0.)) ;
#103780=DIRECTION('center_axis',(0.,1.,0.)) ;
#103781=DIRECTION('ref_axis',(0.,0.,1.)) ;
#103782=DIRECTION('',(0.,0.,1.)) ;
#103783=DIRECTION('center_axis',(0.,1.,0.)) ;
#103784=DIRECTION('ref_axis',(0.,0.,1.)) ;
#103785=DIRECTION('',(-1.,0.,0.)) ;
#103786=DIRECTION('center_axis',(0.,1.,0.)) ;
#103787=DIRECTION('ref_axis',(0.,0.,-1.)) ;
#103788=DIRECTION('',(0.,0.,-1.)) ;
#103789=DIRECTION('center_axis',(0.,1.,0.)) ;
#103790=DIRECTION('ref_axis',(0.,0.,1.)) ;
#103791=DIRECTION('center_axis',(0.,1.,0.)) ;
#103792=DIRECTION('ref_axis',(0.,0.,1.)) ;
#103793=DIRECTION('',(0.,1.,0.)) ;
#103794=DIRECTION('center_axis',(0.,-1.,0.)) ;
#103795=DIRECTION('ref_axis',(2.60208521396521E-14,0.,1.)) ;
#103796=DIRECTION('',(0.,1.,0.)) ;
#103797=DIRECTION('center_axis',(0.,0.,1.)) ;
#103798=DIRECTION('ref_axis',(1.,0.,0.)) ;
#103799=DIRECTION('',(-1.,0.,0.)) ;
#103800=DIRECTION('',(0.,1.,0.)) ;
#103801=DIRECTION('center_axis',(0.,1.,0.)) ;
#103802=DIRECTION('ref_axis',(0.,0.,1.)) ;
#103803=DIRECTION('center_axis',(0.,-1.,0.)) ;
#103804=DIRECTION('ref_axis',(0.,0.,1.)) ;
#103805=DIRECTION('',(0.,1.,0.)) ;
#103806=DIRECTION('center_axis',(-1.,0.,0.)) ;
#103807=DIRECTION('ref_axis',(0.,0.,1.)) ;
#103808=DIRECTION('',(0.,0.,-1.)) ;
#103809=DIRECTION('',(0.,1.,0.)) ;
#103810=DIRECTION('center_axis',(0.,1.,0.)) ;
#103811=DIRECTION('ref_axis',(0.,0.,1.)) ;
#103812=DIRECTION('center_axis',(0.,-1.,0.)) ;
#103813=DIRECTION('ref_axis',(0.,0.,1.)) ;
#103814=DIRECTION('',(0.,1.,0.)) ;
#103815=DIRECTION('center_axis',(0.,0.,-1.)) ;
#103816=DIRECTION('ref_axis',(-1.,0.,0.)) ;
#103817=DIRECTION('',(1.,0.,0.)) ;
#103818=DIRECTION('',(0.,1.,0.)) ;
#103819=DIRECTION('center_axis',(0.,1.,0.)) ;
#103820=DIRECTION('ref_axis',(0.,0.,1.)) ;
#103821=DIRECTION('center_axis',(0.,-1.,0.)) ;
#103822=DIRECTION('ref_axis',(0.,0.,1.)) ;
#103823=DIRECTION('',(0.,1.,0.)) ;
#103824=DIRECTION('center_axis',(1.,0.,0.)) ;
#103825=DIRECTION('ref_axis',(0.,0.,-1.)) ;
#103826=DIRECTION('',(0.,0.,1.)) ;
#103827=DIRECTION('center_axis',(0.,1.,0.)) ;
#103828=DIRECTION('ref_axis',(0.,0.,1.)) ;
#103829=DIRECTION('',(1.,0.,0.)) ;
#103830=DIRECTION('',(0.,0.,-1.)) ;
#103831=DIRECTION('',(-1.,0.,0.)) ;
#103832=DIRECTION('',(0.,0.,1.)) ;
#103833=DIRECTION('center_axis',(0.,0.164398987305357,-0.986393923832144)) ;
#103834=DIRECTION('ref_axis',(0.,0.986393923832144,0.164398987305357)) ;
#103835=DIRECTION('',(-1.,-1.0450141421547E-16,-1.7416902369245E-17)) ;
#103836=DIRECTION('',(0.,-0.986393923832144,-0.164398987305357)) ;
#103837=DIRECTION('',(1.,0.,0.)) ;
#103838=DIRECTION('',(0.,0.986393923832144,0.164398987305357)) ;
#103839=DIRECTION('center_axis',(0.,-1.,0.)) ;
#103840=DIRECTION('ref_axis',(0.,0.,-1.)) ;
#103841=DIRECTION('',(0.,0.,1.)) ;
#103842=DIRECTION('',(0.,0.,-1.)) ;
#103843=DIRECTION('',(-1.,0.,0.)) ;
#103844=DIRECTION('center_axis',(0.,0.164398987305357,0.986393923832144)) ;
#103845=DIRECTION('ref_axis',(0.,-0.986393923832144,0.164398987305357)) ;
#103846=DIRECTION('',(0.,0.986393923832144,-0.164398987305357)) ;
#103847=DIRECTION('',(1.,1.0450141421547E-16,-1.7416902369245E-17)) ;
#103848=DIRECTION('',(0.,-0.986393923832144,0.164398987305357)) ;
#103849=DIRECTION('center_axis',(-1.,0.,0.)) ;
#103850=DIRECTION('ref_axis',(0.,0.,1.)) ;
#103851=DIRECTION('',(0.,0.,1.)) ;
#103852=DIRECTION('center_axis',(-1.,0.,0.)) ;
#103853=DIRECTION('ref_axis',(0.,0.,1.)) ;
#103854=DIRECTION('',(0.,-0.986393923832144,0.164398987305357)) ;
#103855=DIRECTION('',(0.,0.,-1.)) ;
#103856=DIRECTION('',(0.,0.986393923832144,0.164398987305357)) ;
#103857=DIRECTION('center_axis',(1.,0.,0.)) ;
#103858=DIRECTION('ref_axis',(0.,0.,-1.)) ;
#103859=DIRECTION('center_axis',(1.,0.,0.)) ;
#103860=DIRECTION('ref_axis',(0.,0.,-1.)) ;
#103861=DIRECTION('center_axis',(1.,0.,0.)) ;
#103862=DIRECTION('ref_axis',(0.,0.,1.)) ;
#103863=DIRECTION('center_axis',(1.,0.,0.)) ;
#103864=DIRECTION('ref_axis',(0.,0.,1.)) ;
#103865=DIRECTION('center_axis',(1.,0.,0.)) ;
#103866=DIRECTION('ref_axis',(0.,-8.88178419700125E-16,1.)) ;
#103867=DIRECTION('',(1.,0.,0.)) ;
#103868=DIRECTION('center_axis',(-1.,0.,0.)) ;
#103869=DIRECTION('ref_axis',(0.,0.,1.)) ;
#103870=DIRECTION('',(-1.,0.,0.)) ;
#103871=DIRECTION('center_axis',(0.,0.,-1.)) ;
#103872=DIRECTION('ref_axis',(1.,0.,0.)) ;
#103873=DIRECTION('center_axis',(0.,-1.,0.)) ;
#103874=DIRECTION('ref_axis',(0.,0.,1.)) ;
#103875=DIRECTION('center_axis',(0.971399006496778,0.,-0.23745309047699)) ;
#103876=DIRECTION('ref_axis',(-0.23745309047699,0.,-0.971399006496778)) ;
#103877=DIRECTION('center_axis',(0.971399006496778,0.,-0.237453090476989)) ;
#103878=DIRECTION('ref_axis',(-0.237453090476989,0.,-0.971399006496778)) ;
#103879=DIRECTION('center_axis',(0.655772517804501,-0.73774408253007,-0.160299948796655)) ;
#103880=DIRECTION('ref_axis',(-0.747409318683662,-0.664363838829917,2.67307565105543E-16)) ;
#103881=DIRECTION('center_axis',(-0.439210132175304,-4.70034527894889E-10,
-0.898384360835913)) ;
#103882=DIRECTION('ref_axis',(0.882040291645493,-0.189880214237367,-0.431219698245691)) ;
#103883=DIRECTION('center_axis',(0.655772517804504,-0.737744082530068,-0.160299948796656)) ;
#103884=DIRECTION('ref_axis',(0.74740931868366,0.664363838829919,-2.08334010827303E-16)) ;
#103885=DIRECTION('center_axis',(0.655772517804505,-0.737744082530068,-0.16029994879665)) ;
#103886=DIRECTION('ref_axis',(0.74740931868366,0.66436383882992,-5.75609428574487E-16)) ;
#103887=DIRECTION('center_axis',(0.664363838829919,-0.74740931868366,0.)) ;
#103888=DIRECTION('ref_axis',(0.74740931868366,0.664363838829919,0.)) ;
#103889=DIRECTION('center_axis',(-0.664363838829918,0.747409318683661,0.)) ;
#103890=DIRECTION('ref_axis',(-0.747409318683661,-0.664363838829918,0.)) ;
#103891=DIRECTION('center_axis',(0.,1.,0.)) ;
#103892=DIRECTION('ref_axis',(0.,0.,1.)) ;
#103893=DIRECTION('center_axis',(0.,-1.,0.)) ;
#103894=DIRECTION('ref_axis',(0.,0.,-1.)) ;
#103895=DIRECTION('center_axis',(0.,0.,1.)) ;
#103896=DIRECTION('ref_axis',(1.,0.,0.)) ;
#103897=DIRECTION('center_axis',(0.,0.,-1.)) ;
#103898=DIRECTION('ref_axis',(-1.,0.,0.)) ;
#103899=DIRECTION('center_axis',(0.,0.,-1.)) ;
#103900=DIRECTION('ref_axis',(-1.,0.,0.)) ;
#103901=DIRECTION('center_axis',(0.439210132175297,4.70023746982989E-10,
-0.898384360835917)) ;
#103902=DIRECTION('ref_axis',(0.882040291644911,-0.189880214240733,0.4312196982454)) ;
#103903=DIRECTION('center_axis',(-0.971399006496778,0.,-0.23745309047699)) ;
#103904=DIRECTION('ref_axis',(-0.23745309047699,0.,0.971399006496777)) ;
#103905=DIRECTION('center_axis',(0.971399006496778,0.,0.237453090476989)) ;
#103906=DIRECTION('ref_axis',(0.237453090476989,0.,-0.971399006496778)) ;
#103907=DIRECTION('center_axis',(0.,1.,0.)) ;
#103908=DIRECTION('ref_axis',(1.,0.,0.)) ;
#103909=DIRECTION('center_axis',(-3.54829801904343E-14,1.,8.67361737988405E-15)) ;
#103910=DIRECTION('ref_axis',(1.,3.54829801904343E-14,6.83923985932746E-30)) ;
#103911=DIRECTION('center_axis',(-0.948683298050516,0.316227766016832,4.6163005901636E-15)) ;
#103912=DIRECTION('ref_axis',(0.316227766016832,0.948683298050516,5.23037330488368E-13)) ;
#103913=DIRECTION('center_axis',(0.,0.,-1.)) ;
#103914=DIRECTION('ref_axis',(1.,0.,0.)) ;
#103915=DIRECTION('center_axis',(0.,-1.,0.)) ;
#103916=DIRECTION('ref_axis',(0.,0.,1.)) ;
#103917=DIRECTION('center_axis',(0.655772517804503,-0.737744082530069,0.160299948796655)) ;
#103918=DIRECTION('ref_axis',(-0.747409318683661,-0.664363838829918,1.99521945175207E-17)) ;
#103919=DIRECTION('center_axis',(0.,1.,0.)) ;
#103920=DIRECTION('ref_axis',(0.,0.,1.)) ;
#103921=DIRECTION('center_axis',(2.73957817177508E-14,1.,0.)) ;
#103922=DIRECTION('ref_axis',(-1.,2.73957817177508E-14,0.)) ;
#103923=DIRECTION('center_axis',(0.894427190999917,0.447213595499956,0.)) ;
#103924=DIRECTION('ref_axis',(-0.447213595499956,0.894427190999917,0.)) ;
#103925=DIRECTION('center_axis',(-0.894427190999916,-0.447213595499958,
0.)) ;
#103926=DIRECTION('ref_axis',(0.447213595499958,-0.894427190999916,0.)) ;
#103927=DIRECTION('center_axis',(0.,0.,1.)) ;
#103928=DIRECTION('ref_axis',(1.,0.,0.)) ;
#103929=DIRECTION('center_axis',(0.,0.,-1.)) ;
#103930=DIRECTION('ref_axis',(-1.,0.,0.)) ;
#103931=DIRECTION('center_axis',(0.,1.,0.)) ;
#103932=DIRECTION('ref_axis',(0.,0.,1.)) ;
#103933=DIRECTION('center_axis',(0.,-1.,0.)) ;
#103934=DIRECTION('ref_axis',(0.,0.,-1.)) ;
#103935=DIRECTION('center_axis',(-0.664363838829919,0.74740931868366,0.)) ;
#103936=DIRECTION('ref_axis',(-0.74740931868366,-0.664363838829919,0.)) ;
#103937=DIRECTION('center_axis',(-0.66436383882992,0.747409318683659,2.52106651083074E-15)) ;
#103938=DIRECTION('ref_axis',(-0.747409318683659,-0.66436383882992,7.82575143531171E-30)) ;
#103939=DIRECTION('center_axis',(-0.655772517804504,0.737744082530068,-0.160299948796656)) ;
#103940=DIRECTION('ref_axis',(-0.74740931868366,-0.664363838829919,2.31673158493852E-16)) ;
#103941=DIRECTION('center_axis',(0.655772517804496,-0.737744082530075,0.160299948796656)) ;
#103942=DIRECTION('ref_axis',(0.747409318683667,0.664363838829911,-2.10122272487167E-17)) ;
#103943=DIRECTION('center_axis',(0.,1.,0.)) ;
#103944=DIRECTION('ref_axis',(1.,0.,0.)) ;
#103945=DIRECTION('center_axis',(-0.873786407766988,-0.436893203883498,
0.213592233009711)) ;
#103946=DIRECTION('ref_axis',(-0.447213595499961,0.894427190999914,-1.41283224420644E-15)) ;
#103947=DIRECTION('center_axis',(-0.948683298050516,0.316227766016832,-3.71868658652068E-15)) ;
#103948=DIRECTION('ref_axis',(0.316227766016832,0.948683298050516,-5.15504951476798E-13)) ;
#103949=DIRECTION('center_axis',(0.,1.,0.)) ;
#103950=DIRECTION('ref_axis',(1.,0.,0.)) ;
#103951=DIRECTION('center_axis',(-5.47915634355017E-14,1.,0.)) ;
#103952=DIRECTION('ref_axis',(1.,5.47915634355017E-14,8.67361737988401E-15)) ;
#103953=DIRECTION('center_axis',(-0.971399006496778,0.,0.23745309047699)) ;
#103954=DIRECTION('ref_axis',(0.23745309047699,0.,0.971399006496778)) ;
#103955=DIRECTION('center_axis',(0.971399006496778,-3.69787733965917E-15,
-0.237453090476989)) ;
#103956=DIRECTION('ref_axis',(-0.237453090476989,1.76125929374961E-30,-0.971399006496778)) ;
#103957=DIRECTION('center_axis',(0.873786407766991,0.436893203883493,-0.213592233009709)) ;
#103958=DIRECTION('ref_axis',(-0.447213595499956,0.894427190999917,2.83414331365695E-16)) ;
#103959=DIRECTION('center_axis',(-0.873786407766992,-0.436893203883492,
0.21359223300971)) ;
#103960=DIRECTION('ref_axis',(0.447213595499955,-0.894427190999918,-1.48231119036019E-16)) ;
#103961=DIRECTION('center_axis',(-0.894427190999917,-0.447213595499956,
0.)) ;
#103962=DIRECTION('ref_axis',(0.447213595499956,-0.894427190999917,0.)) ;
#103963=DIRECTION('center_axis',(-0.894427190999917,-0.447213595499955,
0.)) ;
#103964=DIRECTION('ref_axis',(0.447213595499955,-0.894427190999917,0.)) ;
#103965=DIRECTION('center_axis',(0.,1.,0.)) ;
#103966=DIRECTION('ref_axis',(0.,0.,1.)) ;
#103967=DIRECTION('center_axis',(2.66122351428257E-14,1.,6.50521303491301E-15)) ;
#103968=DIRECTION('ref_axis',(-1.,2.66122351428257E-14,3.84707242087163E-30)) ;
#103969=DIRECTION('center_axis',(-0.439210132004928,-6.77418203687457E-14,
-0.898384360919208)) ;
#103970=DIRECTION('ref_axis',(0.898384360919208,9.23120187976291E-12,-0.439210132004928)) ;
#103971=DIRECTION('center_axis',(0.,1.,0.)) ;
#103972=DIRECTION('ref_axis',(1.,0.,0.)) ;
#103973=DIRECTION('center_axis',(-0.87378640776699,-0.436893203883495,-0.213592233009712)) ;
#103974=DIRECTION('ref_axis',(-0.447213595499958,0.894427190999916,-1.87666485977959E-15)) ;
#103975=DIRECTION('center_axis',(0.,0.,1.)) ;
#103976=DIRECTION('ref_axis',(1.,0.,0.)) ;
#103977=DIRECTION('center_axis',(0.439210132004928,6.77418203687389E-14,
-0.898384360919208)) ;
#103978=DIRECTION('ref_axis',(0.898384360919208,-4.19790080461511E-11,0.439210132004928)) ;
#103979=DIRECTION('center_axis',(-0.873786407766991,-0.436893203883493,
-0.213592233009709)) ;
#103980=DIRECTION('ref_axis',(0.447213595499956,-0.894427190999917,-1.06780556900622E-16)) ;
#103981=DIRECTION('center_axis',(-0.873786407766992,-0.436893203883492,
-0.213592233009707)) ;
#103982=DIRECTION('ref_axis',(0.447213595499955,-0.894427190999918,-7.04543255365314E-18)) ;
#103983=DIRECTION('center_axis',(-0.971399006496778,0.,-0.237453090476989)) ;
#103984=DIRECTION('ref_axis',(0.237453090476989,0.,-0.971399006496778)) ;
#103985=DIRECTION('center_axis',(0.971399006496778,0.,0.23745309047699)) ;
#103986=DIRECTION('ref_axis',(0.23745309047699,0.,-0.971399006496778)) ;
#103987=DIRECTION('center_axis',(0.,0.,-1.)) ;
#103988=DIRECTION('ref_axis',(-1.,0.,0.)) ;
#103989=DIRECTION('center_axis',(1.,1.0450141421547E-16,1.7416902369245E-17)) ;
#103990=DIRECTION('ref_axis',(-1.0450141421547E-16,1.,-1.82009092883888E-33)) ;
#103991=DIRECTION('center_axis',(0.672672795322926,0.739940072189931,-7.49337348295411E-10)) ;
#103992=DIRECTION('ref_axis',(0.738044870608594,-0.670949884715798,0.0715263669439543)) ;
#103993=DIRECTION('center_axis',(-1.,0.,0.)) ;
#103994=DIRECTION('ref_axis',(0.,-0.646374896130195,-0.763019982472726)) ;
#103995=DIRECTION('center_axis',(-1.,0.,0.)) ;
#103996=DIRECTION('ref_axis',(0.,0.,1.)) ;
#103997=DIRECTION('center_axis',(-1.,0.,0.)) ;
#103998=DIRECTION('ref_axis',(0.,0.,1.)) ;
#103999=DIRECTION('center_axis',(0.,0.986393923832144,0.164398987305357)) ;
#104000=DIRECTION('ref_axis',(0.,-0.164398987305357,0.986393923832144)) ;
#104001=DIRECTION('center_axis',(0.,-0.986393923832144,-0.164398987305358)) ;
#104002=DIRECTION('ref_axis',(0.,0.164398987305358,-0.986393923832144)) ;
#104003=DIRECTION('center_axis',(0.,0.,1.)) ;
#104004=DIRECTION('ref_axis',(1.,0.,0.)) ;
#104005=DIRECTION('center_axis',(0.,0.,1.)) ;
#104006=DIRECTION('ref_axis',(1.,0.,0.)) ;
#104007=DIRECTION('center_axis',(0.,0.,1.)) ;
#104008=DIRECTION('ref_axis',(1.,0.,0.)) ;
#104009=DIRECTION('center_axis',(0.,0.,-1.)) ;
#104010=DIRECTION('ref_axis',(1.,0.,0.)) ;
#104011=DIRECTION('center_axis',(-1.,0.,0.)) ;
#104012=DIRECTION('ref_axis',(0.,-0.646374896130195,-0.763019982472726)) ;
#104013=DIRECTION('center_axis',(0.,0.,1.)) ;
#104014=DIRECTION('ref_axis',(-1.,0.,0.)) ;
#104015=DIRECTION('center_axis',(0.,0.,-1.)) ;
#104016=DIRECTION('ref_axis',(-1.,0.,0.)) ;
#104017=DIRECTION('center_axis',(1.,1.0450141421547E-16,-1.7416902369245E-17)) ;
#104018=DIRECTION('ref_axis',(-1.0450141421547E-16,1.,1.82009092883888E-33)) ;
#104019=DIRECTION('center_axis',(0.672672795322883,0.73994007218997,7.49325583516064E-10)) ;
#104020=DIRECTION('ref_axis',(0.738044870607526,-0.67094988471475,-0.071526366964805)) ;
#104021=DIRECTION('center_axis',(1.,0.,0.)) ;
#104022=DIRECTION('ref_axis',(0.,0.,1.)) ;
#104023=DIRECTION('center_axis',(0.,0.,-1.)) ;
#104024=DIRECTION('ref_axis',(-1.,0.,0.)) ;
#104025=DIRECTION('center_axis',(0.,-0.986393923832144,0.164398987305357)) ;
#104026=DIRECTION('ref_axis',(0.,-0.164398987305357,-0.986393923832144)) ;
#104027=DIRECTION('center_axis',(1.,0.,0.)) ;
#104028=DIRECTION('ref_axis',(0.,0.,1.)) ;
#104029=DIRECTION('center_axis',(7.58941520739854E-15,0.,-1.)) ;
#104030=DIRECTION('ref_axis',(-1.,0.,-7.58941520739854E-15)) ;
#104031=DIRECTION('center_axis',(1.,0.,-8.67361737988404E-15)) ;
#104032=DIRECTION('ref_axis',(-8.67361737988404E-15,0.,-1.)) ;
#104033=DIRECTION('center_axis',(1.,0.,0.)) ;
#104034=DIRECTION('ref_axis',(0.,0.,-1.)) ;
#104035=DIRECTION('center_axis',(1.,0.,8.67361737988403E-15)) ;
#104036=DIRECTION('ref_axis',(8.67361737988403E-15,0.,-1.)) ;
#104037=DIRECTION('center_axis',(0.,0.,1.)) ;
#104038=DIRECTION('ref_axis',(1.,0.,0.)) ;
#104039=DIRECTION('center_axis',(0.,0.,-1.)) ;
#104040=DIRECTION('ref_axis',(-1.,0.,0.)) ;
#104041=DIRECTION('center_axis',(1.,0.,0.)) ;
#104042=DIRECTION('ref_axis',(0.,0.,1.)) ;
#104043=DIRECTION('center_axis',(-6.50521303491304E-15,0.,-1.)) ;
#104044=DIRECTION('ref_axis',(-1.,0.,6.50521303491304E-15)) ;
#104045=DIRECTION('center_axis',(1.,0.,0.)) ;
#104046=DIRECTION('ref_axis',(0.,0.,1.)) ;
#104047=DIRECTION('center_axis',(1.,9.40395480657835E-30,8.67361737988403E-15)) ;
#104048=DIRECTION('ref_axis',(8.67361737988403E-15,9.95682444457783E-60,
-1.)) ;
#104049=DIRECTION('center_axis',(0.,0.,-1.)) ;
#104050=DIRECTION('ref_axis',(-1.,0.,0.)) ;
#104051=DIRECTION('center_axis',(6.50521303491304E-15,0.,-1.)) ;
#104052=DIRECTION('ref_axis',(-1.,0.,-6.50521303491304E-15)) ;
#104053=DIRECTION('center_axis',(-1.,0.,0.)) ;
#104054=DIRECTION('ref_axis',(0.,0.,1.)) ;
#104055=DIRECTION('center_axis',(1.,-8.67361737988409E-15,0.)) ;
#104056=DIRECTION('ref_axis',(8.67361737988409E-15,1.,0.)) ;
#104057=DIRECTION('center_axis',(1.,0.,0.)) ;
#104058=DIRECTION('ref_axis',(0.,0.,1.)) ;
#104059=DIRECTION('center_axis',(-4.33680868994202E-16,0.,1.)) ;
#104060=DIRECTION('ref_axis',(1.,0.,4.33680868994202E-16)) ;
#104061=DIRECTION('center_axis',(0.,0.,-1.)) ;
#104062=DIRECTION('ref_axis',(-1.,0.,0.)) ;
#104063=DIRECTION('center_axis',(0.,0.,1.)) ;
#104064=DIRECTION('ref_axis',(1.,0.,0.)) ;
#104065=DIRECTION('center_axis',(0.,1.,0.)) ;
#104066=DIRECTION('ref_axis',(0.,0.,1.)) ;
#104067=DIRECTION('center_axis',(-1.,0.,0.)) ;
#104068=DIRECTION('ref_axis',(0.,0.,-1.)) ;
#104069=DIRECTION('center_axis',(0.,-1.,0.)) ;
#104070=DIRECTION('ref_axis',(0.,0.,1.)) ;
#104071=DIRECTION('center_axis',(0.,1.,0.)) ;
#104072=DIRECTION('ref_axis',(0.,0.,1.)) ;
#104073=DIRECTION('center_axis',(0.,-1.,0.)) ;
#104074=DIRECTION('ref_axis',(0.,0.,1.)) ;
#104075=DIRECTION('center_axis',(-1.,0.,0.)) ;
#104076=DIRECTION('ref_axis',(0.,0.,-1.)) ;
#104077=DIRECTION('center_axis',(-1.,0.,-1.73472347597681E-16)) ;
#104078=DIRECTION('ref_axis',(-1.73472347597681E-16,0.,1.)) ;
#104079=DIRECTION('center_axis',(-1.,0.,0.)) ;
#104080=DIRECTION('ref_axis',(0.,0.,1.)) ;
#104081=DIRECTION('center_axis',(0.,1.,0.)) ;
#104082=DIRECTION('ref_axis',(0.,0.,1.)) ;
#104083=DIRECTION('center_axis',(0.,-1.,0.)) ;
#104084=DIRECTION('ref_axis',(0.,0.,-1.)) ;
#104085=DIRECTION('center_axis',(-4.33680868994202E-16,0.,1.)) ;
#104086=DIRECTION('ref_axis',(1.,0.,4.33680868994202E-16)) ;
#104087=DIRECTION('center_axis',(0.,0.,1.)) ;
#104088=DIRECTION('ref_axis',(1.,0.,0.)) ;
#104089=DIRECTION('center_axis',(0.,0.,-1.)) ;
#104090=DIRECTION('ref_axis',(-1.,0.,0.)) ;
#104091=DIRECTION('center_axis',(0.,1.,0.)) ;
#104092=DIRECTION('ref_axis',(0.,0.,1.)) ;
#104093=DIRECTION('center_axis',(0.,-1.,0.)) ;
#104094=DIRECTION('ref_axis',(0.,0.,-1.)) ;
#104095=DIRECTION('center_axis',(1.,0.,-1.73472347597681E-16)) ;
#104096=DIRECTION('ref_axis',(-1.73472347597681E-16,0.,-1.)) ;
#104097=DIRECTION('center_axis',(-1.,0.,0.)) ;
#104098=DIRECTION('ref_axis',(0.,0.,1.)) ;
#104099=DIRECTION('center_axis',(0.,0.,-1.)) ;
#104100=DIRECTION('ref_axis',(-1.,0.,0.)) ;
#104101=DIRECTION('center_axis',(0.,0.,1.)) ;
#104102=DIRECTION('ref_axis',(1.,0.,0.)) ;
#104103=DIRECTION('center_axis',(0.,0.,-1.)) ;
#104104=DIRECTION('ref_axis',(-1.,0.,0.)) ;
#104105=DIRECTION('center_axis',(0.,1.,0.)) ;
#104106=DIRECTION('ref_axis',(0.,0.,1.)) ;
#104107=DIRECTION('center_axis',(0.,-1.,0.)) ;
#104108=DIRECTION('ref_axis',(0.,0.,1.)) ;
#104109=DIRECTION('center_axis',(0.,1.,0.)) ;
#104110=DIRECTION('ref_axis',(1.,0.,0.)) ;
#104111=DIRECTION('center_axis',(1.,0.,0.)) ;
#104112=DIRECTION('ref_axis',(0.,0.,1.)) ;
#104113=DIRECTION('center_axis',(0.,1.,0.)) ;
#104114=DIRECTION('ref_axis',(1.,0.,0.)) ;
#104115=DIRECTION('center_axis',(1.,0.,0.)) ;
#104116=DIRECTION('ref_axis',(0.,0.,1.)) ;
#104117=DIRECTION('center_axis',(0.,1.,0.)) ;
#104118=DIRECTION('ref_axis',(0.,0.,1.)) ;
#104119=DIRECTION('center_axis',(0.,-1.,0.)) ;
#104120=DIRECTION('ref_axis',(0.,0.,1.)) ;
#104121=DIRECTION('center_axis',(0.,1.,0.)) ;
#104122=DIRECTION('ref_axis',(0.,0.,1.)) ;
#104123=DIRECTION('center_axis',(0.,-1.,0.)) ;
#104124=DIRECTION('ref_axis',(0.,0.,-1.)) ;
#104125=DIRECTION('center_axis',(-1.,0.,-1.73472347597681E-16)) ;
#104126=DIRECTION('ref_axis',(-1.73472347597681E-16,0.,1.)) ;
#104127=DIRECTION('center_axis',(1.,0.,0.)) ;
#104128=DIRECTION('ref_axis',(0.,0.,-1.)) ;
#104129=DIRECTION('center_axis',(1.,0.,-1.73472347597681E-16)) ;
#104130=DIRECTION('ref_axis',(-1.73472347597681E-16,0.,-1.)) ;
#104131=DIRECTION('center_axis',(1.,0.,0.)) ;
#104132=DIRECTION('ref_axis',(0.,0.,-1.)) ;
#104133=DIRECTION('center_axis',(0.,1.,0.)) ;
#104134=DIRECTION('ref_axis',(0.,0.,1.)) ;
#104135=DIRECTION('center_axis',(0.,-1.,0.)) ;
#104136=DIRECTION('ref_axis',(0.,0.,-1.)) ;
#104137=DIRECTION('center_axis',(0.,1.,0.)) ;
#104138=DIRECTION('ref_axis',(1.,0.,0.)) ;
#104139=DIRECTION('center_axis',(0.,0.,1.)) ;
#104140=DIRECTION('ref_axis',(-1.,0.,0.)) ;
#104141=DIRECTION('center_axis',(0.,1.,0.)) ;
#104142=DIRECTION('ref_axis',(1.,0.,0.)) ;
#104143=DIRECTION('center_axis',(0.,0.,-1.)) ;
#104144=DIRECTION('ref_axis',(1.,0.,0.)) ;
#104145=DIRECTION('center_axis',(0.,0.,-1.)) ;
#104146=DIRECTION('ref_axis',(-1.,0.,0.)) ;
#104147=DIRECTION('center_axis',(2.16840434497101E-16,0.,1.)) ;
#104148=DIRECTION('ref_axis',(1.,0.,-2.16840434497101E-16)) ;
#104149=DIRECTION('center_axis',(0.,0.,-1.)) ;
#104150=DIRECTION('ref_axis',(-1.,0.,0.)) ;
#104151=DIRECTION('center_axis',(0.,0.,1.)) ;
#104152=DIRECTION('ref_axis',(1.,0.,0.)) ;
#104153=DIRECTION('center_axis',(0.,-1.,0.)) ;
#104154=DIRECTION('ref_axis',(0.,0.,-1.)) ;
#104155=DIRECTION('center_axis',(1.,0.,0.)) ;
#104156=DIRECTION('ref_axis',(0.,0.,1.)) ;
#104157=DIRECTION('center_axis',(0.,1.,0.)) ;
#104158=DIRECTION('ref_axis',(0.,0.,-1.)) ;
#104159=DIRECTION('center_axis',(0.,-1.,0.)) ;
#104160=DIRECTION('ref_axis',(0.,0.,-1.)) ;
#104161=DIRECTION('center_axis',(0.,1.,0.)) ;
#104162=DIRECTION('ref_axis',(0.,0.,-1.)) ;
#104163=DIRECTION('center_axis',(1.,0.,0.)) ;
#104164=DIRECTION('ref_axis',(0.,0.,1.)) ;
#104165=DIRECTION('center_axis',(1.,0.,-1.73472347597681E-16)) ;
#104166=DIRECTION('ref_axis',(-1.73472347597681E-16,0.,-1.)) ;
#104167=DIRECTION('center_axis',(1.,0.,0.)) ;
#104168=DIRECTION('ref_axis',(0.,0.,-1.)) ;
#104169=DIRECTION('center_axis',(0.,-1.,0.)) ;
#104170=DIRECTION('ref_axis',(0.,0.,-1.)) ;
#104171=DIRECTION('center_axis',(0.,1.,0.)) ;
#104172=DIRECTION('ref_axis',(0.,0.,1.)) ;
#104173=DIRECTION('center_axis',(2.16840434497101E-16,0.,1.)) ;
#104174=DIRECTION('ref_axis',(1.,0.,-2.16840434497101E-16)) ;
#104175=DIRECTION('center_axis',(0.,0.,1.)) ;
#104176=DIRECTION('ref_axis',(1.,0.,0.)) ;
#104177=DIRECTION('center_axis',(0.,0.,-1.)) ;
#104178=DIRECTION('ref_axis',(-1.,0.,0.)) ;
#104179=DIRECTION('center_axis',(0.,-1.,0.)) ;
#104180=DIRECTION('ref_axis',(0.,0.,-1.)) ;
#104181=DIRECTION('center_axis',(0.,1.,0.)) ;
#104182=DIRECTION('ref_axis',(0.,0.,1.)) ;
#104183=DIRECTION('center_axis',(-1.,0.,1.73472347597681E-16)) ;
#104184=DIRECTION('ref_axis',(1.73472347597681E-16,0.,1.)) ;
#104185=DIRECTION('center_axis',(1.,0.,0.)) ;
#104186=DIRECTION('ref_axis',(0.,0.,-1.)) ;
#104187=DIRECTION('center_axis',(-2.16840434497101E-16,0.,-1.)) ;
#104188=DIRECTION('ref_axis',(-1.,0.,2.16840434497101E-16)) ;
#104189=DIRECTION('center_axis',(0.,0.,1.)) ;
#104190=DIRECTION('ref_axis',(1.,0.,0.)) ;
#104191=DIRECTION('center_axis',(0.,0.,-1.)) ;
#104192=DIRECTION('ref_axis',(-1.,0.,0.)) ;
#104193=DIRECTION('center_axis',(0.,-1.,0.)) ;
#104194=DIRECTION('ref_axis',(0.,0.,-1.)) ;
#104195=DIRECTION('center_axis',(0.,1.,0.)) ;
#104196=DIRECTION('ref_axis',(0.,0.,-1.)) ;
#104197=DIRECTION('center_axis',(0.,1.,0.)) ;
#104198=DIRECTION('ref_axis',(1.,0.,0.)) ;
#104199=DIRECTION('center_axis',(-1.,0.,0.)) ;
#104200=DIRECTION('ref_axis',(0.,0.,-1.)) ;
#104201=DIRECTION('center_axis',(0.,1.,0.)) ;
#104202=DIRECTION('ref_axis',(1.,0.,0.)) ;
#104203=DIRECTION('center_axis',(-1.,0.,0.)) ;
#104204=DIRECTION('ref_axis',(0.,0.,-1.)) ;
#104205=DIRECTION('center_axis',(0.,-1.,0.)) ;
#104206=DIRECTION('ref_axis',(0.,0.,-1.)) ;
#104207=DIRECTION('center_axis',(0.,1.,0.)) ;
#104208=DIRECTION('ref_axis',(0.,0.,-1.)) ;
#104209=DIRECTION('center_axis',(0.,-1.,0.)) ;
#104210=DIRECTION('ref_axis',(0.,0.,-1.)) ;
#104211=DIRECTION('center_axis',(0.,1.,0.)) ;
#104212=DIRECTION('ref_axis',(0.,0.,1.)) ;
#104213=DIRECTION('center_axis',(1.,0.,-1.73472347597681E-16)) ;
#104214=DIRECTION('ref_axis',(-1.73472347597681E-16,0.,-1.)) ;
#104215=DIRECTION('center_axis',(-1.,0.,0.)) ;
#104216=DIRECTION('ref_axis',(0.,0.,1.)) ;
#104217=DIRECTION('center_axis',(-1.,0.,1.73472347597681E-16)) ;
#104218=DIRECTION('ref_axis',(1.73472347597681E-16,0.,1.)) ;
#104219=DIRECTION('center_axis',(-1.,0.,0.)) ;
#104220=DIRECTION('ref_axis',(0.,0.,1.)) ;
#104221=DIRECTION('center_axis',(0.,-1.,0.)) ;
#104222=DIRECTION('ref_axis',(0.,0.,-1.)) ;
#104223=DIRECTION('center_axis',(0.,1.,0.)) ;
#104224=DIRECTION('ref_axis',(0.,0.,1.)) ;
#104225=DIRECTION('center_axis',(0.,1.,0.)) ;
#104226=DIRECTION('ref_axis',(1.,0.,0.)) ;
#104227=DIRECTION('center_axis',(0.,0.,1.)) ;
#104228=DIRECTION('ref_axis',(-1.,0.,0.)) ;
#104229=DIRECTION('center_axis',(0.,1.,0.)) ;
#104230=DIRECTION('ref_axis',(1.,0.,0.)) ;
#104231=DIRECTION('center_axis',(0.,0.,-1.)) ;
#104232=DIRECTION('ref_axis',(1.,0.,0.)) ;
#104233=DIRECTION('center_axis',(-2.16840434497101E-16,0.,-1.)) ;
#104234=DIRECTION('ref_axis',(-1.,0.,2.16840434497101E-16)) ;
#104235=DIRECTION('center_axis',(-1.,0.,0.)) ;
#104236=DIRECTION('ref_axis',(0.,0.,1.)) ;
#104237=DIRECTION('center_axis',(0.,-0.632948931301575,-0.774193548387091)) ;
#104238=DIRECTION('ref_axis',(0.,0.774193548387091,-0.632948931301575)) ;
#104239=DIRECTION('center_axis',(0.,0.,1.)) ;
#104240=DIRECTION('ref_axis',(1.,0.,0.)) ;
#104241=DIRECTION('center_axis',(8.67361737988401E-15,0.,1.)) ;
#104242=DIRECTION('ref_axis',(1.,0.,-8.67361737988401E-15)) ;
#104243=DIRECTION('center_axis',(0.,1.,0.)) ;
#104244=DIRECTION('ref_axis',(1.,0.,0.)) ;
#104245=DIRECTION('center_axis',(-1.,0.,0.)) ;
#104246=DIRECTION('ref_axis',(0.,0.,-1.)) ;
#104247=DIRECTION('center_axis',(1.,0.,0.)) ;
#104248=DIRECTION('ref_axis',(0.,0.,-1.)) ;
#104249=DIRECTION('center_axis',(-1.,0.,0.)) ;
#104250=DIRECTION('ref_axis',(0.,0.,1.)) ;
#104251=DIRECTION('center_axis',(0.,0.,-1.)) ;
#104252=DIRECTION('ref_axis',(-1.,0.,0.)) ;
#104253=DIRECTION('center_axis',(0.,0.,-1.)) ;
#104254=DIRECTION('ref_axis',(-1.,0.,0.)) ;
#104255=DIRECTION('center_axis',(-1.,0.,0.)) ;
#104256=DIRECTION('ref_axis',(0.,0.,1.)) ;
#104257=DIRECTION('center_axis',(0.,-0.632948931301567,-0.774193548387097)) ;
#104258=DIRECTION('ref_axis',(0.,-0.774193548387097,0.632948931301567)) ;
#104259=DIRECTION('center_axis',(-1.,0.,0.)) ;
#104260=DIRECTION('ref_axis',(0.,0.,1.)) ;
#104261=DIRECTION('center_axis',(0.,0.632948931301567,-0.774193548387097)) ;
#104262=DIRECTION('ref_axis',(0.,0.774193548387097,0.632948931301567)) ;
#104263=DIRECTION('center_axis',(0.,0.,-1.)) ;
#104264=DIRECTION('ref_axis',(-1.,0.,0.)) ;
#104265=DIRECTION('center_axis',(0.,0.,-1.)) ;
#104266=DIRECTION('ref_axis',(-1.,0.,0.)) ;
#104267=DIRECTION('center_axis',(0.,0.,1.)) ;
#104268=DIRECTION('ref_axis',(1.,0.,0.)) ;
#104269=DIRECTION('center_axis',(-1.,0.,0.)) ;
#104270=DIRECTION('ref_axis',(0.,0.,1.)) ;
#104271=DIRECTION('center_axis',(1.,0.,0.)) ;
#104272=DIRECTION('ref_axis',(0.,-8.67361737988403E-15,1.)) ;
#104273=DIRECTION('center_axis',(1.,0.,0.)) ;
#104274=DIRECTION('ref_axis',(0.,0.,-1.)) ;
#104275=DIRECTION('center_axis',(1.,0.,0.)) ;
#104276=DIRECTION('ref_axis',(0.,0.,-1.)) ;
#104277=DIRECTION('center_axis',(0.,0.,1.)) ;
#104278=DIRECTION('ref_axis',(1.,0.,0.)) ;
#104279=DIRECTION('center_axis',(8.67361737988401E-15,0.,1.)) ;
#104280=DIRECTION('ref_axis',(1.,0.,-8.67361737988401E-15)) ;
#104281=DIRECTION('center_axis',(0.,8.67361737988405E-15,-1.)) ;
#104282=DIRECTION('ref_axis',(0.,1.,8.67361737988405E-15)) ;
#104283=DIRECTION('center_axis',(0.,1.,0.)) ;
#104284=DIRECTION('ref_axis',(1.,0.,0.)) ;
#104285=DIRECTION('center_axis',(1.22050154678007E-14,0.632948931301567,
-0.774193548387097)) ;
#104286=DIRECTION('ref_axis',(-2.03293076771647E-29,-0.774193548387097,
-0.632948931301567)) ;
#104287=DIRECTION('center_axis',(-1.,0.,0.)) ;
#104288=DIRECTION('ref_axis',(0.,0.,1.)) ;
#104289=DIRECTION('center_axis',(0.,0.,1.)) ;
#104290=DIRECTION('ref_axis',(1.,0.,0.)) ;
#104291=DIRECTION('center_axis',(0.,0.,1.)) ;
#104292=DIRECTION('ref_axis',(1.,0.,0.)) ;
#104293=DIRECTION('center_axis',(0.,0.,-1.)) ;
#104294=DIRECTION('ref_axis',(-1.,0.,0.)) ;
#104295=DIRECTION('center_axis',(0.,0.,-1.)) ;
#104296=DIRECTION('ref_axis',(1.,0.,0.)) ;
#104297=DIRECTION('center_axis',(0.,0.,-1.)) ;
#104298=DIRECTION('ref_axis',(-1.,0.,0.)) ;
#104299=DIRECTION('center_axis',(0.,0.,-1.)) ;
#104300=DIRECTION('ref_axis',(1.,0.,0.)) ;
#104301=DIRECTION('center_axis',(0.,0.,-1.)) ;
#104302=DIRECTION('ref_axis',(-1.,0.,0.)) ;
#104303=DIRECTION('center_axis',(0.,0.,-1.)) ;
#104304=DIRECTION('ref_axis',(1.,2.6020852139652E-14,0.)) ;
#104305=DIRECTION('center_axis',(0.,0.,-1.)) ;
#104306=DIRECTION('ref_axis',(-1.,0.,0.)) ;
#104307=DIRECTION('center_axis',(0.,0.,-1.)) ;
#104308=DIRECTION('ref_axis',(1.,0.,0.)) ;
#104309=DIRECTION('center_axis',(0.,0.,-1.)) ;
#104310=DIRECTION('ref_axis',(-1.,0.,0.)) ;
#104311=DIRECTION('center_axis',(0.,0.,-1.)) ;
#104312=DIRECTION('ref_axis',(1.,0.,0.)) ;
#104313=DIRECTION('center_axis',(-0.422618261740697,0.,0.906307787036651)) ;
#104314=DIRECTION('ref_axis',(0.906307787036651,0.,0.422618261740697)) ;
#104315=DIRECTION('center_axis',(0.422618261740697,0.,-0.906307787036651)) ;
#104316=DIRECTION('ref_axis',(-0.906307787036651,0.,-0.422618261740697)) ;
#104317=DIRECTION('center_axis',(0.422618261740697,0.,-0.906307787036651)) ;
#104318=DIRECTION('ref_axis',(-0.906307787036651,0.,-0.422618261740697)) ;
#104319=DIRECTION('center_axis',(-0.422618261740697,0.,0.906307787036651)) ;
#104320=DIRECTION('ref_axis',(0.906307787036651,0.,0.422618261740697)) ;
#104321=DIRECTION('center_axis',(0.,0.,-1.)) ;
#104322=DIRECTION('ref_axis',(-1.,0.,0.)) ;
#104323=DIRECTION('center_axis',(0.,0.,-1.)) ;
#104324=DIRECTION('ref_axis',(1.,0.,0.)) ;
#104325=DIRECTION('center_axis',(0.,0.,-1.)) ;
#104326=DIRECTION('ref_axis',(-1.,0.,0.)) ;
#104327=DIRECTION('center_axis',(0.,0.,-1.)) ;
#104328=DIRECTION('ref_axis',(1.,1.04083408558609E-13,0.)) ;
#104329=DIRECTION('center_axis',(0.,0.,1.)) ;
#104330=DIRECTION('ref_axis',(1.,0.,0.)) ;
#104331=DIRECTION('center_axis',(0.,0.,1.)) ;
#104332=DIRECTION('ref_axis',(1.,0.,0.)) ;
#104333=DIRECTION('center_axis',(0.,1.,0.)) ;
#104334=DIRECTION('ref_axis',(1.,0.,0.)) ;
#104335=DIRECTION('center_axis',(0.,-0.986393923832144,0.164398987305358)) ;
#104336=DIRECTION('ref_axis',(0.,-0.164398987305358,-0.986393923832144)) ;
#104337=DIRECTION('center_axis',(0.,0.986393923832144,-0.164398987305357)) ;
#104338=DIRECTION('ref_axis',(0.,0.164398987305357,0.986393923832144)) ;
#104339=DIRECTION('center_axis',(0.,-0.986393923832144,0.164398987305358)) ;
#104340=DIRECTION('ref_axis',(0.,-0.164398987305358,-0.986393923832144)) ;
#104341=DIRECTION('center_axis',(-1.,0.,0.)) ;
#104342=DIRECTION('ref_axis',(0.,0.107567764393763,-0.994197755008192)) ;
#104343=DIRECTION('center_axis',(4.02631181035923E-15,-0.928404294083138,
-0.371571617226061)) ;
#104344=DIRECTION('ref_axis',(-2.55493810320452E-31,0.371571617226061,-0.928404294083138)) ;
#104345=DIRECTION('center_axis',(0.275516865537137,-0.50093975551097,-0.820457078800105)) ;
#104346=DIRECTION('ref_axis',(-8.25573355829978E-17,0.853490367006418,-0.521108619605597)) ;
#104347=DIRECTION('center_axis',(0.,0.,-1.)) ;
#104348=DIRECTION('ref_axis',(-1.,0.,0.)) ;
#104349=DIRECTION('center_axis',(0.,0.,-1.)) ;
#104350=DIRECTION('ref_axis',(-1.,0.,0.)) ;
#104351=DIRECTION('center_axis',(0.,0.,-1.)) ;
#104352=DIRECTION('ref_axis',(-1.,0.,0.)) ;
#104353=DIRECTION('center_axis',(0.,0.,-1.)) ;
#104354=DIRECTION('ref_axis',(-1.,0.,0.)) ;
#104355=DIRECTION('center_axis',(0.,0.,-1.)) ;
#104356=DIRECTION('ref_axis',(-1.,0.,0.)) ;
#104357=DIRECTION('center_axis',(-0.275516865538071,0.500939755523742,-0.820457078791993)) ;
#104358=DIRECTION('ref_axis',(7.85941951813298E-17,0.853490366998217,0.521108619619028)) ;
#104359=DIRECTION('center_axis',(0.,-0.986393923832144,-0.164398987305357)) ;
#104360=DIRECTION('ref_axis',(0.,0.164398987305357,-0.986393923832144)) ;
#104361=DIRECTION('center_axis',(3.5648347838177E-16,0.986393923832144,
0.164398987305358)) ;
#104362=DIRECTION('ref_axis',(-2.28603566590726E-32,-0.164398987305358,
0.986393923832144)) ;
#104363=DIRECTION('center_axis',(0.,1.,0.)) ;
#104364=DIRECTION('ref_axis',(1.,0.,0.)) ;
#104365=DIRECTION('center_axis',(-1.,0.,0.)) ;
#104366=DIRECTION('ref_axis',(0.,0.,1.)) ;
#104367=DIRECTION('center_axis',(0.,0.,-1.)) ;
#104368=DIRECTION('ref_axis',(-1.,0.,0.)) ;
#104369=DIRECTION('center_axis',(0.,0.,-1.)) ;
#104370=DIRECTION('ref_axis',(-1.,0.,0.)) ;
#104371=DIRECTION('center_axis',(0.,0.,-1.)) ;
#104372=DIRECTION('ref_axis',(-1.,0.,0.)) ;
#104373=DIRECTION('center_axis',(0.,0.,-1.)) ;
#104374=DIRECTION('ref_axis',(-1.,0.,0.)) ;
#104375=DIRECTION('center_axis',(2.168404344971E-15,0.,1.)) ;
#104376=DIRECTION('ref_axis',(1.,0.,-2.168404344971E-15)) ;
#104377=DIRECTION('center_axis',(0.795723237447208,-7.53302716311723E-12,
0.605660407643206)) ;
#104378=DIRECTION('ref_axis',(0.605660407643206,-1.05709445921463E-26,-0.795723237447208)) ;
#104379=DIRECTION('center_axis',(1.57772181044204E-26,2.36658271566302E-26,
1.)) ;
#104380=DIRECTION('ref_axis',(-3.78339027370117E-66,-1.,2.36658271566302E-26)) ;
#104381=DIRECTION('center_axis',(-0.795723237415222,-2.11663082418553E-11,
0.605660407685229)) ;
#104382=DIRECTION('ref_axis',(0.605660407685229,9.32717726754359E-27,0.795723237415222)) ;
#104383=DIRECTION('center_axis',(0.,-3.94255335449274E-16,1.)) ;
#104384=DIRECTION('ref_axis',(0.,-1.,-3.94255335449274E-16)) ;
#104385=DIRECTION('center_axis',(0.147618562252691,0.989044367093028,0.)) ;
#104386=DIRECTION('ref_axis',(-0.989044367093028,0.147618562252691,0.)) ;
#104387=DIRECTION('',(0.,0.,1.)) ;
#104388=DIRECTION('',(0.989044367093028,-0.147618562252691,0.)) ;
#104389=DIRECTION('',(0.,0.,1.)) ;
#104390=DIRECTION('',(-0.989044367093028,0.147618562252691,0.)) ;
#104391=DIRECTION('center_axis',(0.,0.,1.)) ;
#104392=DIRECTION('ref_axis',(1.,0.,0.)) ;
#104393=DIRECTION('center_axis',(0.,0.,-1.)) ;
#104394=DIRECTION('ref_axis',(1.,0.,0.)) ;
#104395=DIRECTION('',(0.,0.,1.)) ;
#104396=DIRECTION('center_axis',(0.,0.,1.)) ;
#104397=DIRECTION('ref_axis',(1.,0.,0.)) ;
#104398=DIRECTION('center_axis',(0.697619267438899,0.716468671818953,0.)) ;
#104399=DIRECTION('ref_axis',(-0.716468671818953,0.697619267438899,0.)) ;
#104400=DIRECTION('',(0.716468671818953,-0.697619267438899,0.)) ;
#104401=DIRECTION('',(0.,0.,1.)) ;
#104402=DIRECTION('',(-0.716468671818953,0.697619267438899,0.)) ;
#104403=DIRECTION('center_axis',(0.,0.,1.)) ;
#104404=DIRECTION('ref_axis',(1.,0.,0.)) ;
#104405=DIRECTION('center_axis',(0.,0.,-1.)) ;
#104406=DIRECTION('ref_axis',(1.,0.,0.)) ;
#104407=DIRECTION('',(0.,0.,1.)) ;
#104408=DIRECTION('center_axis',(0.,0.,1.)) ;
#104409=DIRECTION('ref_axis',(1.,0.,0.)) ;
#104410=DIRECTION('center_axis',(1.,0.,0.)) ;
#104411=DIRECTION('ref_axis',(0.,0.,-1.)) ;
#104412=DIRECTION('',(0.,-1.,0.)) ;
#104413=DIRECTION('',(0.,0.,1.)) ;
#104414=DIRECTION('',(0.,1.,0.)) ;
#104415=DIRECTION('center_axis',(0.,0.,1.)) ;
#104416=DIRECTION('ref_axis',(1.,0.,0.)) ;
#104417=DIRECTION('center_axis',(0.,0.,-1.)) ;
#104418=DIRECTION('ref_axis',(1.,0.,0.)) ;
#104419=DIRECTION('',(0.,0.,1.)) ;
#104420=DIRECTION('center_axis',(0.,0.,1.)) ;
#104421=DIRECTION('ref_axis',(1.,0.,0.)) ;
#104422=DIRECTION('center_axis',(-0.453905661840943,-0.891049746169503,
0.)) ;
#104423=DIRECTION('ref_axis',(0.891049746169503,-0.453905661840943,0.)) ;
#104424=DIRECTION('',(-0.891049746169503,0.453905661840943,0.)) ;
#104425=DIRECTION('',(0.,0.,1.)) ;
#104426=DIRECTION('',(0.891049746169503,-0.453905661840943,0.)) ;
#104427=DIRECTION('center_axis',(0.,0.,1.)) ;
#104428=DIRECTION('ref_axis',(1.,0.,0.)) ;
#104429=DIRECTION('center_axis',(0.,0.,1.)) ;
#104430=DIRECTION('ref_axis',(1.,0.,0.)) ;
#104431=DIRECTION('',(0.,0.,1.)) ;
#104432=DIRECTION('center_axis',(0.,0.,-1.)) ;
#104433=DIRECTION('ref_axis',(1.,0.,0.)) ;
#104434=DIRECTION('center_axis',(-2.60782465076463E-16,-1.,0.)) ;
#104435=DIRECTION('ref_axis',(1.,-2.60782465076463E-16,0.)) ;
#104436=DIRECTION('',(-1.,2.60782465076463E-16,0.)) ;
#104437=DIRECTION('',(0.,0.,-1.)) ;
#104438=DIRECTION('',(1.,-2.60782465076463E-16,0.)) ;
#104439=DIRECTION('center_axis',(0.,0.,1.)) ;
#104440=DIRECTION('ref_axis',(1.,0.,0.)) ;
#104441=DIRECTION('center_axis',(0.,0.,1.)) ;
#104442=DIRECTION('ref_axis',(1.,0.,0.)) ;
#104443=DIRECTION('',(-1.,2.60782465076463E-16,0.)) ;
#104444=DIRECTION('',(0.,1.,0.)) ;
#104445=DIRECTION('',(0.989044367093028,-0.147618562252691,0.)) ;
#104446=DIRECTION('',(0.716468671818953,-0.697619267438899,0.)) ;
#104447=DIRECTION('',(0.,-1.,0.)) ;
#104448=DIRECTION('',(-0.891049746169503,0.453905661840943,0.)) ;
#104449=DIRECTION('center_axis',(0.,0.,1.)) ;
#104450=DIRECTION('ref_axis',(1.,0.,0.)) ;
#104451=DIRECTION('',(-0.716468671818953,0.697619267438899,0.)) ;
#104452=DIRECTION('',(-0.989044367093028,0.147618562252691,0.)) ;
#104453=DIRECTION('',(0.,-1.,0.)) ;
#104454=DIRECTION('',(1.,-2.60782465076463E-16,0.)) ;
#104455=DIRECTION('center_axis',(0.,0.,-1.)) ;
#104456=DIRECTION('ref_axis',(1.,0.,0.)) ;
#104457=DIRECTION('',(0.891049746169503,-0.453905661840943,0.)) ;
#104458=DIRECTION('',(0.,1.,0.)) ;
#104459=DIRECTION('center_axis',(-1.,0.,0.)) ;
#104460=DIRECTION('ref_axis',(0.,0.,1.)) ;
#104461=DIRECTION('center_axis',(-1.,0.,0.)) ;
#104462=DIRECTION('ref_axis',(0.,0.,1.)) ;
#104463=DIRECTION('',(0.,0.,-1.)) ;
#104464=DIRECTION('',(0.,1.,0.)) ;
#104465=DIRECTION('',(0.,0.,1.)) ;
#104466=DIRECTION('center_axis',(1.0450141421547E-16,-1.,0.)) ;
#104467=DIRECTION('ref_axis',(1.,1.0450141421547E-16,0.)) ;
#104468=DIRECTION('',(-1.,-1.0450141421547E-16,0.)) ;
#104469=DIRECTION('',(0.,0.,1.)) ;
#104470=DIRECTION('',(1.,1.0450141421547E-16,1.7416902369245E-17)) ;
#104471=DIRECTION('',(0.,0.,-1.)) ;
#104472=DIRECTION('center_axis',(0.,1.,0.)) ;
#104473=DIRECTION('ref_axis',(0.,0.,1.)) ;
#104474=DIRECTION('',(0.422618261740697,0.,-0.906307787036651)) ;
#104475=DIRECTION('center_axis',(-2.09002828430941E-16,1.,0.)) ;
#104476=DIRECTION('ref_axis',(-1.,-2.09002828430941E-16,0.)) ;
#104477=DIRECTION('',(-1.,-2.09002828430941E-16,0.)) ;
#104478=DIRECTION('',(0.,0.,-1.)) ;
#104479=DIRECTION('',(1.,2.09002828430941E-16,0.)) ;
#104480=DIRECTION('',(0.,0.,1.)) ;
#104481=DIRECTION('center_axis',(0.,0.,1.)) ;
#104482=DIRECTION('ref_axis',(1.,0.,0.)) ;
#104483=DIRECTION('center_axis',(0.,0.,-1.)) ;
#104484=DIRECTION('ref_axis',(1.,0.,0.)) ;
#104485=DIRECTION('center_axis',(0.,0.,1.)) ;
#104486=DIRECTION('ref_axis',(1.,0.,0.)) ;
#104487=DIRECTION('center_axis',(0.,0.,-1.)) ;
#104488=DIRECTION('ref_axis',(1.,1.30104260698261E-14,0.)) ;
#104489=DIRECTION('center_axis',(0.,0.,-1.)) ;
#104490=DIRECTION('ref_axis',(1.,0.,0.)) ;
#104491=DIRECTION('center_axis',(0.,0.,1.)) ;
#104492=DIRECTION('ref_axis',(1.,0.,0.)) ;
#104493=DIRECTION('center_axis',(0.,0.,1.)) ;
#104494=DIRECTION('ref_axis',(1.,0.,0.)) ;
#104495=DIRECTION('',(-0.664363838829919,0.74740931868366,0.)) ;
#104496=DIRECTION('',(0.,-1.,0.)) ;
#104497=DIRECTION('',(0.894427190999917,0.447213595499956,0.)) ;
#104498=DIRECTION('',(0.,1.,0.)) ;
#104499=DIRECTION('center_axis',(0.,0.,-1.)) ;
#104500=DIRECTION('ref_axis',(-1.,0.,0.)) ;
#104501=DIRECTION('',(-0.894427190999917,-0.447213595499956,0.)) ;
#104502=DIRECTION('',(0.,1.,0.)) ;
#104503=DIRECTION('',(0.664363838829919,-0.74740931868366,0.)) ;
#104504=DIRECTION('',(0.,-1.,0.)) ;
#104505=DIRECTION('center_axis',(-0.23745309047699,0.,-0.971399006496778)) ;
#104506=DIRECTION('ref_axis',(-0.971399006496778,0.,0.23745309047699)) ;
#104507=DIRECTION('center_axis',(-0.237453090476989,4.46069609701422E-15,
-0.971399006496778)) ;
#104508=DIRECTION('ref_axis',(0.921799787671161,-0.315455332292563,-0.225328836986284)) ;
#104509=DIRECTION('',(0.971399006496777,0.,-0.23745309047699)) ;
#104510=DIRECTION('',(0.,-1.,0.)) ;
#104511=DIRECTION('',(-0.971399006496777,0.,0.23745309047699)) ;
#104512=DIRECTION('center_axis',(-0.237453090476974,-7.91889358654166E-14,
-0.971399006496781)) ;
#104513=DIRECTION('ref_axis',(0.954559354254046,0.185392581172289,-0.233336731039876)) ;
#104514=DIRECTION('',(-0.873786407766991,-0.436893203883493,0.213592233009709)) ;
#104515=DIRECTION('',(0.,1.,0.)) ;
#104516=DIRECTION('',(0.655772517804503,-0.737744082530068,-0.160299948796656)) ;
#104517=DIRECTION('center_axis',(-1.,0.,0.)) ;
#104518=DIRECTION('ref_axis',(0.,0.,1.)) ;
#104519=DIRECTION('',(0.,-1.,0.)) ;
#104520=DIRECTION('center_axis',(-1.,-6.70078870827235E-15,-6.50913949396064E-15)) ;
#104521=DIRECTION('ref_axis',(6.50913949395814E-15,3.73530394823002E-13,
-1.)) ;
#104522=DIRECTION('',(0.,0.,-1.)) ;
#104523=DIRECTION('center_axis',(-1.,0.,0.)) ;
#104524=DIRECTION('ref_axis',(0.,1.52591140012917E-12,-1.)) ;
#104525=DIRECTION('center_axis',(-1.,6.70078870827225E-15,6.5091394939605E-15)) ;
#104526=DIRECTION('ref_axis',(-6.5091394939748E-15,-2.1338917236146E-12,
-1.)) ;
#104527=DIRECTION('',(0.,0.,-1.)) ;
#104528=DIRECTION('center_axis',(-1.,6.70078870827219E-15,-6.50913949396048E-15)) ;
#104529=DIRECTION('ref_axis',(6.50913949391343E-15,-7.02157667714827E-12,
-1.)) ;
#104530=DIRECTION('center_axis',(-0.23745309047699,0.,0.971399006496778)) ;
#104531=DIRECTION('ref_axis',(0.971399006496778,0.,0.23745309047699)) ;
#104532=DIRECTION('center_axis',(-0.237453090476981,-4.06097107001983E-14,
0.97139900649678)) ;
#104533=DIRECTION('ref_axis',(0.95455935425498,0.185392581167189,0.233336731040105)) ;
#104534=DIRECTION('',(0.971399006496777,0.,0.23745309047699)) ;
#104535=DIRECTION('',(-0.971399006496777,0.,-0.23745309047699)) ;
#104536=DIRECTION('center_axis',(-0.23745309047696,8.47532258432748E-14,
0.971399006496785)) ;
#104537=DIRECTION('ref_axis',(0.921799787670825,-0.315455332293604,0.225328836986199)) ;
#104538=DIRECTION('',(-0.655772517804503,0.737744082530068,-0.160299948796656)) ;
#104539=DIRECTION('',(0.,-1.,0.)) ;
#104540=DIRECTION('',(0.873786407766991,0.436893203883493,0.213592233009709)) ;
#104541=DIRECTION('center_axis',(0.,1.,0.)) ;
#104542=DIRECTION('ref_axis',(0.,0.,1.)) ;
#104543=DIRECTION('',(-0.971399006496777,0.,0.23745309047699)) ;
#104544=DIRECTION('',(0.,0.,-1.)) ;
#104545=DIRECTION('',(0.971399006496777,0.,0.23745309047699)) ;
#104546=DIRECTION('center_axis',(0.,1.,0.)) ;
#104547=DIRECTION('ref_axis',(0.,0.,1.)) ;
#104548=DIRECTION('',(-0.971399006496777,0.,-0.23745309047699)) ;
#104549=DIRECTION('',(0.,0.,1.)) ;
#104550=DIRECTION('',(0.971399006496777,0.,-0.23745309047699)) ;
#104551=DIRECTION('center_axis',(-0.447213595499956,0.894427190999917,0.)) ;
#104552=DIRECTION('ref_axis',(0.,0.,-1.)) ;
#104553=DIRECTION('',(0.,0.,-1.)) ;
#104554=DIRECTION('',(-0.873786407766991,-0.436893203883493,-0.213592233009709)) ;
#104555=DIRECTION('',(-0.894427190999917,-0.447213595499956,0.)) ;
#104556=DIRECTION('',(0.,0.,1.)) ;
#104557=DIRECTION('',(0.894427190999917,0.447213595499956,0.)) ;
#104558=DIRECTION('',(0.873786407766991,0.436893203883493,-0.213592233009709)) ;
#104559=DIRECTION('center_axis',(0.74740931868366,0.664363838829919,0.)) ;
#104560=DIRECTION('ref_axis',(0.,0.,1.)) ;
#104561=DIRECTION('',(0.,0.,-1.)) ;
#104562=DIRECTION('',(0.664363838829919,-0.74740931868366,0.)) ;
#104563=DIRECTION('',(0.655772517804503,-0.737744082530068,0.160299948796656)) ;
#104564=DIRECTION('',(0.,0.,1.)) ;
#104565=DIRECTION('',(-0.655772517804503,0.737744082530068,0.160299948796656)) ;
#104566=DIRECTION('',(-0.664363838829919,0.74740931868366,0.)) ;
#104567=DIRECTION('center_axis',(1.,0.,4.33680868994202E-16)) ;
#104568=DIRECTION('ref_axis',(4.33680868994202E-16,0.,-1.)) ;
#104569=DIRECTION('',(0.,1.,0.)) ;
#104570=DIRECTION('',(4.33680868994202E-16,0.,-1.)) ;
#104571=DIRECTION('',(0.,-1.,0.)) ;
#104572=DIRECTION('',(-4.33680868994202E-16,0.,1.)) ;
#104573=DIRECTION('center_axis',(-1.73472347597681E-16,0.,-1.)) ;
#104574=DIRECTION('ref_axis',(-1.,0.,1.73472347597681E-16)) ;
#104575=DIRECTION('',(-1.,0.,1.73472347597681E-16)) ;
#104576=DIRECTION('',(0.,-1.,0.)) ;
#104577=DIRECTION('',(1.,0.,-1.73472347597681E-16)) ;
#104578=DIRECTION('',(0.,1.,0.)) ;
#104579=DIRECTION('center_axis',(-1.,0.,0.)) ;
#104580=DIRECTION('ref_axis',(0.,0.,1.)) ;
#104581=DIRECTION('',(0.,0.,1.)) ;
#104582=DIRECTION('',(0.,-1.,0.)) ;
#104583=DIRECTION('',(0.,0.,-1.)) ;
#104584=DIRECTION('',(0.,1.,0.)) ;
#104585=DIRECTION('center_axis',(-1.73472347597681E-16,0.,1.)) ;
#104586=DIRECTION('ref_axis',(1.,0.,1.73472347597681E-16)) ;
#104587=DIRECTION('',(0.,1.,0.)) ;
#104588=DIRECTION('',(1.,0.,1.73472347597681E-16)) ;
#104589=DIRECTION('',(0.,-1.,0.)) ;
#104590=DIRECTION('',(-1.,0.,-1.73472347597681E-16)) ;
#104591=DIRECTION('center_axis',(0.,-1.,0.)) ;
#104592=DIRECTION('ref_axis',(0.,0.,-1.)) ;
#104593=DIRECTION('',(-1.,0.,-1.73472347597681E-16)) ;
#104594=DIRECTION('',(0.,0.,-1.)) ;
#104595=DIRECTION('',(1.,0.,-1.73472347597681E-16)) ;
#104596=DIRECTION('',(-4.33680868994202E-16,0.,1.)) ;
#104597=DIRECTION('',(1.,0.,0.)) ;
#104598=DIRECTION('center_axis',(0.,-1.,0.)) ;
#104599=DIRECTION('ref_axis',(0.,0.,-1.)) ;
#104600=DIRECTION('',(0.,0.,-1.)) ;
#104601=DIRECTION('center_axis',(0.,-1.,0.)) ;
#104602=DIRECTION('ref_axis',(0.,0.,-1.)) ;
#104603=DIRECTION('',(-1.,0.,0.)) ;
#104604=DIRECTION('center_axis',(0.,-1.,0.)) ;
#104605=DIRECTION('ref_axis',(0.,0.,1.)) ;
#104606=DIRECTION('',(0.,0.,1.)) ;
#104607=DIRECTION('center_axis',(0.,-1.,0.)) ;
#104608=DIRECTION('ref_axis',(0.,0.,-1.)) ;
#104609=DIRECTION('center_axis',(0.,-1.,0.)) ;
#104610=DIRECTION('ref_axis',(0.,0.,-1.)) ;
#104611=DIRECTION('center_axis',(0.,-1.,0.)) ;
#104612=DIRECTION('ref_axis',(0.,0.,-1.)) ;
#104613=DIRECTION('',(0.,-1.,0.)) ;
#104614=DIRECTION('',(0.,-1.,0.)) ;
#104615=DIRECTION('center_axis',(0.,0.,-1.)) ;
#104616=DIRECTION('ref_axis',(-1.,0.,0.)) ;
#104617=DIRECTION('',(1.,0.,0.)) ;
#104618=DIRECTION('',(0.,-1.,0.)) ;
#104619=DIRECTION('center_axis',(0.,-1.,0.)) ;
#104620=DIRECTION('ref_axis',(0.,0.,-1.)) ;
#104621=DIRECTION('center_axis',(0.,-1.,0.)) ;
#104622=DIRECTION('ref_axis',(0.,0.,-1.)) ;
#104623=DIRECTION('',(0.,-1.,0.)) ;
#104624=DIRECTION('center_axis',(-1.,0.,0.)) ;
#104625=DIRECTION('ref_axis',(0.,0.,1.)) ;
#104626=DIRECTION('',(0.,0.,-1.)) ;
#104627=DIRECTION('',(0.,-1.,0.)) ;
#104628=DIRECTION('center_axis',(0.,-1.,0.)) ;
#104629=DIRECTION('ref_axis',(0.,0.,-1.)) ;
#104630=DIRECTION('center_axis',(0.,-1.,0.)) ;
#104631=DIRECTION('ref_axis',(0.,0.,-1.)) ;
#104632=DIRECTION('',(0.,-1.,0.)) ;
#104633=DIRECTION('center_axis',(0.,0.,1.)) ;
#104634=DIRECTION('ref_axis',(1.,0.,0.)) ;
#104635=DIRECTION('',(-1.,0.,0.)) ;
#104636=DIRECTION('',(0.,-1.,0.)) ;
#104637=DIRECTION('center_axis',(0.,-1.,0.)) ;
#104638=DIRECTION('ref_axis',(0.,0.,-1.)) ;
#104639=DIRECTION('center_axis',(0.,-1.,0.)) ;
#104640=DIRECTION('ref_axis',(0.,0.,1.)) ;
#104641=DIRECTION('',(0.,-1.,0.)) ;
#104642=DIRECTION('center_axis',(1.,0.,0.)) ;
#104643=DIRECTION('ref_axis',(0.,0.,-1.)) ;
#104644=DIRECTION('',(0.,0.,1.)) ;
#104645=DIRECTION('center_axis',(0.,-1.,0.)) ;
#104646=DIRECTION('ref_axis',(0.,0.,-1.)) ;
#104647=DIRECTION('center_axis',(0.,1.,0.)) ;
#104648=DIRECTION('ref_axis',(0.,0.,1.)) ;
#104649=DIRECTION('',(-0.422618261740697,0.,0.906307787036651)) ;
#104650=DIRECTION('center_axis',(0.906307787036651,0.,0.422618261740697)) ;
#104651=DIRECTION('ref_axis',(0.422618261740697,0.,-0.906307787036651)) ;
#104652=DIRECTION('',(-0.422618261740697,0.,0.906307787036651)) ;
#104653=DIRECTION('',(0.422618261740697,0.,-0.906307787036651)) ;
#104654=DIRECTION('center_axis',(-0.906307787036651,0.,-0.422618261740697)) ;
#104655=DIRECTION('ref_axis',(-0.422618261740697,0.,0.906307787036651)) ;
#104656=DIRECTION('',(0.422618261740697,0.,-0.906307787036651)) ;
#104657=DIRECTION('',(-0.422618261740697,0.,0.906307787036651)) ;
#104658=DIRECTION('center_axis',(0.,1.,0.)) ;
#104659=DIRECTION('ref_axis',(0.,0.,1.)) ;
#104660=DIRECTION('',(-0.422618261740697,0.,0.906307787036651)) ;
#104661=DIRECTION('',(0.422618261740697,0.,-0.906307787036651)) ;
#104662=DIRECTION('center_axis',(1.,0.,-2.16840434497101E-16)) ;
#104663=DIRECTION('ref_axis',(-2.16840434497101E-16,0.,-1.)) ;
#104664=DIRECTION('',(2.16840434497101E-16,0.,1.)) ;
#104665=DIRECTION('',(0.,1.,0.)) ;
#104666=DIRECTION('',(-2.16840434497101E-16,0.,-1.)) ;
#104667=DIRECTION('',(0.,-1.,0.)) ;
#104668=DIRECTION('center_axis',(1.73472347597681E-16,0.,1.)) ;
#104669=DIRECTION('ref_axis',(1.,0.,-1.73472347597681E-16)) ;
#104670=DIRECTION('',(0.,-1.,0.)) ;
#104671=DIRECTION('',(-1.,0.,1.73472347597681E-16)) ;
#104672=DIRECTION('',(0.,1.,0.)) ;
#104673=DIRECTION('',(1.,0.,-1.73472347597681E-16)) ;
#104674=DIRECTION('center_axis',(-1.,0.,2.16840434497101E-16)) ;
#104675=DIRECTION('ref_axis',(2.16840434497101E-16,0.,1.)) ;
#104676=DIRECTION('',(0.,-1.,0.)) ;
#104677=DIRECTION('',(-2.16840434497101E-16,0.,-1.)) ;
#104678=DIRECTION('',(0.,1.,0.)) ;
#104679=DIRECTION('',(2.16840434497101E-16,0.,1.)) ;
#104680=DIRECTION('center_axis',(-1.73472347597681E-16,0.,-1.)) ;
#104681=DIRECTION('ref_axis',(-1.,0.,1.73472347597681E-16)) ;
#104682=DIRECTION('',(1.,0.,-1.73472347597681E-16)) ;
#104683=DIRECTION('',(0.,1.,0.)) ;
#104684=DIRECTION('',(-1.,0.,1.73472347597681E-16)) ;
#104685=DIRECTION('',(0.,-1.,0.)) ;
#104686=DIRECTION('center_axis',(0.,1.,0.)) ;
#104687=DIRECTION('ref_axis',(0.,0.,1.)) ;
#104688=DIRECTION('',(1.,0.,-1.73472347597681E-16)) ;
#104689=DIRECTION('',(-2.16840434497101E-16,0.,-1.)) ;
#104690=DIRECTION('',(-1.,0.,1.73472347597681E-16)) ;
#104691=DIRECTION('',(2.16840434497101E-16,0.,1.)) ;
#104692=DIRECTION('',(1.,0.,0.)) ;
#104693=DIRECTION('center_axis',(0.,1.,0.)) ;
#104694=DIRECTION('ref_axis',(0.,0.,1.)) ;
#104695=DIRECTION('',(0.,0.,1.)) ;
#104696=DIRECTION('center_axis',(0.,1.,0.)) ;
#104697=DIRECTION('ref_axis',(0.,0.,1.)) ;
#104698=DIRECTION('',(-1.,0.,0.)) ;
#104699=DIRECTION('center_axis',(0.,1.,0.)) ;
#104700=DIRECTION('ref_axis',(0.,0.,-1.)) ;
#104701=DIRECTION('',(0.,0.,-1.)) ;
#104702=DIRECTION('center_axis',(0.,1.,0.)) ;
#104703=DIRECTION('ref_axis',(0.,0.,1.)) ;
#104704=DIRECTION('center_axis',(0.,1.,0.)) ;
#104705=DIRECTION('ref_axis',(0.,0.,1.)) ;
#104706=DIRECTION('',(0.,1.,0.)) ;
#104707=DIRECTION('center_axis',(0.,-1.,0.)) ;
#104708=DIRECTION('ref_axis',(2.6020852139652E-14,0.,1.)) ;
#104709=DIRECTION('',(0.,1.,0.)) ;
#104710=DIRECTION('center_axis',(0.,0.,1.)) ;
#104711=DIRECTION('ref_axis',(1.,0.,0.)) ;
#104712=DIRECTION('',(-1.,0.,0.)) ;
#104713=DIRECTION('',(0.,1.,0.)) ;
#104714=DIRECTION('center_axis',(0.,1.,0.)) ;
#104715=DIRECTION('ref_axis',(0.,0.,1.)) ;
#104716=DIRECTION('center_axis',(0.,-1.,0.)) ;
#104717=DIRECTION('ref_axis',(0.,0.,1.)) ;
#104718=DIRECTION('',(0.,1.,0.)) ;
#104719=DIRECTION('center_axis',(-1.,0.,0.)) ;
#104720=DIRECTION('ref_axis',(0.,0.,1.)) ;
#104721=DIRECTION('',(0.,0.,-1.)) ;
#104722=DIRECTION('',(0.,1.,0.)) ;
#104723=DIRECTION('center_axis',(0.,1.,0.)) ;
#104724=DIRECTION('ref_axis',(0.,0.,1.)) ;
#104725=DIRECTION('center_axis',(0.,-1.,0.)) ;
#104726=DIRECTION('ref_axis',(0.,0.,1.)) ;
#104727=DIRECTION('',(0.,1.,0.)) ;
#104728=DIRECTION('center_axis',(0.,0.,-1.)) ;
#104729=DIRECTION('ref_axis',(-1.,0.,0.)) ;
#104730=DIRECTION('',(1.,0.,0.)) ;
#104731=DIRECTION('',(0.,1.,0.)) ;
#104732=DIRECTION('center_axis',(0.,1.,0.)) ;
#104733=DIRECTION('ref_axis',(0.,0.,1.)) ;
#104734=DIRECTION('center_axis',(0.,-1.,0.)) ;
#104735=DIRECTION('ref_axis',(0.,0.,1.)) ;
#104736=DIRECTION('',(0.,1.,0.)) ;
#104737=DIRECTION('center_axis',(1.,0.,0.)) ;
#104738=DIRECTION('ref_axis',(0.,0.,-1.)) ;
#104739=DIRECTION('',(0.,0.,1.)) ;
#104740=DIRECTION('center_axis',(0.,1.,0.)) ;
#104741=DIRECTION('ref_axis',(0.,0.,1.)) ;
#104742=DIRECTION('',(1.,0.,0.)) ;
#104743=DIRECTION('',(0.,0.,-1.)) ;
#104744=DIRECTION('',(-1.,0.,0.)) ;
#104745=DIRECTION('',(0.,0.,1.)) ;
#104746=DIRECTION('center_axis',(0.,0.164398987305357,-0.986393923832144)) ;
#104747=DIRECTION('ref_axis',(0.,0.986393923832144,0.164398987305357)) ;
#104748=DIRECTION('',(-1.,-1.0450141421547E-16,-1.7416902369245E-17)) ;
#104749=DIRECTION('',(0.,-0.986393923832144,-0.164398987305357)) ;
#104750=DIRECTION('',(1.,0.,0.)) ;
#104751=DIRECTION('',(0.,0.986393923832144,0.164398987305357)) ;
#104752=DIRECTION('center_axis',(0.,-1.,0.)) ;
#104753=DIRECTION('ref_axis',(0.,0.,-1.)) ;
#104754=DIRECTION('',(0.,0.,1.)) ;
#104755=DIRECTION('',(0.,0.,-1.)) ;
#104756=DIRECTION('',(-1.,0.,0.)) ;
#104757=DIRECTION('center_axis',(0.,0.164398987305357,0.986393923832144)) ;
#104758=DIRECTION('ref_axis',(0.,-0.986393923832144,0.164398987305357)) ;
#104759=DIRECTION('',(0.,0.986393923832144,-0.164398987305357)) ;
#104760=DIRECTION('',(1.,1.0450141421547E-16,-1.7416902369245E-17)) ;
#104761=DIRECTION('',(0.,-0.986393923832144,0.164398987305357)) ;
#104762=DIRECTION('center_axis',(-1.,0.,0.)) ;
#104763=DIRECTION('ref_axis',(0.,0.,1.)) ;
#104764=DIRECTION('',(0.,0.,1.)) ;
#104765=DIRECTION('center_axis',(-1.,0.,0.)) ;
#104766=DIRECTION('ref_axis',(0.,0.,1.)) ;
#104767=DIRECTION('',(0.,-0.986393923832144,0.164398987305357)) ;
#104768=DIRECTION('',(0.,0.,-1.)) ;
#104769=DIRECTION('',(0.,0.986393923832144,0.164398987305357)) ;
#104770=DIRECTION('center_axis',(1.,0.,0.)) ;
#104771=DIRECTION('ref_axis',(0.,0.,-1.)) ;
#104772=DIRECTION('center_axis',(1.,0.,0.)) ;
#104773=DIRECTION('ref_axis',(0.,0.,-1.)) ;
#104774=DIRECTION('center_axis',(1.,0.,0.)) ;
#104775=DIRECTION('ref_axis',(0.,0.,1.)) ;
#104776=DIRECTION('center_axis',(1.,0.,0.)) ;
#104777=DIRECTION('ref_axis',(0.,0.,1.)) ;
#104778=DIRECTION('center_axis',(1.,0.,0.)) ;
#104779=DIRECTION('ref_axis',(0.,-8.88178419700125E-16,1.)) ;
#104780=DIRECTION('',(1.,0.,0.)) ;
#104781=DIRECTION('center_axis',(-1.,0.,0.)) ;
#104782=DIRECTION('ref_axis',(0.,0.,1.)) ;
#104783=DIRECTION('',(-1.,0.,0.)) ;
#104784=DIRECTION('center_axis',(0.,0.,-1.)) ;
#104785=DIRECTION('ref_axis',(1.,0.,0.)) ;
#104786=DIRECTION('center_axis',(0.,-1.,0.)) ;
#104787=DIRECTION('ref_axis',(0.,0.,1.)) ;
#104788=DIRECTION('center_axis',(0.971399006496778,0.,-0.23745309047699)) ;
#104789=DIRECTION('ref_axis',(-0.23745309047699,0.,-0.971399006496778)) ;
#104790=DIRECTION('center_axis',(0.971399006496778,0.,-0.237453090476989)) ;
#104791=DIRECTION('ref_axis',(-0.237453090476989,0.,-0.971399006496778)) ;
#104792=DIRECTION('center_axis',(0.655772517804501,-0.73774408253007,-0.160299948796655)) ;
#104793=DIRECTION('ref_axis',(-0.747409318683662,-0.664363838829917,2.67307565105543E-16)) ;
#104794=DIRECTION('center_axis',(-0.439210132175389,-4.7027023783242E-10,
-0.898384360835871)) ;
#104795=DIRECTION('ref_axis',(0.882040291645213,-0.189880214238859,-0.431219698245608)) ;
#104796=DIRECTION('center_axis',(0.655772517804504,-0.737744082530068,-0.160299948796656)) ;
#104797=DIRECTION('ref_axis',(0.74740931868366,0.664363838829919,-2.08334010827303E-16)) ;
#104798=DIRECTION('center_axis',(0.655772517804505,-0.737744082530068,-0.16029994879665)) ;
#104799=DIRECTION('ref_axis',(0.74740931868366,0.66436383882992,-5.75609428574487E-16)) ;
#104800=DIRECTION('center_axis',(0.664363838829919,-0.74740931868366,0.)) ;
#104801=DIRECTION('ref_axis',(0.74740931868366,0.664363838829919,0.)) ;
#104802=DIRECTION('center_axis',(-0.664363838829918,0.747409318683661,0.)) ;
#104803=DIRECTION('ref_axis',(-0.747409318683661,-0.664363838829918,0.)) ;
#104804=DIRECTION('center_axis',(0.,1.,0.)) ;
#104805=DIRECTION('ref_axis',(0.,0.,1.)) ;
#104806=DIRECTION('center_axis',(0.,-1.,0.)) ;
#104807=DIRECTION('ref_axis',(0.,0.,-1.)) ;
#104808=DIRECTION('center_axis',(0.,0.,1.)) ;
#104809=DIRECTION('ref_axis',(1.,0.,0.)) ;
#104810=DIRECTION('center_axis',(0.,0.,-1.)) ;
#104811=DIRECTION('ref_axis',(-1.,0.,0.)) ;
#104812=DIRECTION('center_axis',(0.,0.,-1.)) ;
#104813=DIRECTION('ref_axis',(-1.,0.,0.)) ;
#104814=DIRECTION('center_axis',(0.439210132175242,4.69850272309497E-10,
-0.898384360835943)) ;
#104815=DIRECTION('ref_axis',(0.882040291645527,-0.189880214237253,0.431219698245671)) ;
#104816=DIRECTION('center_axis',(-0.971399006496778,0.,-0.23745309047699)) ;
#104817=DIRECTION('ref_axis',(-0.23745309047699,0.,0.971399006496777)) ;
#104818=DIRECTION('center_axis',(0.971399006496778,0.,0.237453090476989)) ;
#104819=DIRECTION('ref_axis',(0.237453090476989,0.,-0.971399006496778)) ;
#104820=DIRECTION('center_axis',(0.,1.,0.)) ;
#104821=DIRECTION('ref_axis',(1.,0.,0.)) ;
#104822=DIRECTION('center_axis',(-3.54829801904343E-14,1.,8.67361737988405E-15)) ;
#104823=DIRECTION('ref_axis',(1.,3.54829801904343E-14,6.83923985932746E-30)) ;
#104824=DIRECTION('center_axis',(-0.948683298050516,0.316227766016833,4.61630059016351E-15)) ;
#104825=DIRECTION('ref_axis',(0.316227766016833,0.948683298050516,-2.58893576341231E-13)) ;
#104826=DIRECTION('center_axis',(0.,0.,-1.)) ;
#104827=DIRECTION('ref_axis',(1.,0.,0.)) ;
#104828=DIRECTION('center_axis',(0.,-1.,0.)) ;
#104829=DIRECTION('ref_axis',(0.,0.,1.)) ;
#104830=DIRECTION('center_axis',(0.655772517804503,-0.737744082530069,0.160299948796655)) ;
#104831=DIRECTION('ref_axis',(-0.747409318683661,-0.664363838829918,1.99521945175207E-17)) ;
#104832=DIRECTION('center_axis',(0.,1.,0.)) ;
#104833=DIRECTION('ref_axis',(0.,0.,1.)) ;
#104834=DIRECTION('center_axis',(2.73957817177508E-14,1.,0.)) ;
#104835=DIRECTION('ref_axis',(-1.,2.73957817177508E-14,0.)) ;
#104836=DIRECTION('center_axis',(0.894427190999917,0.447213595499956,0.)) ;
#104837=DIRECTION('ref_axis',(-0.447213595499956,0.894427190999917,0.)) ;
#104838=DIRECTION('center_axis',(-0.894427190999916,-0.447213595499958,
0.)) ;
#104839=DIRECTION('ref_axis',(0.447213595499958,-0.894427190999916,0.)) ;
#104840=DIRECTION('center_axis',(0.,0.,1.)) ;
#104841=DIRECTION('ref_axis',(1.,0.,0.)) ;
#104842=DIRECTION('center_axis',(0.,0.,-1.)) ;
#104843=DIRECTION('ref_axis',(-1.,0.,0.)) ;
#104844=DIRECTION('center_axis',(0.,1.,0.)) ;
#104845=DIRECTION('ref_axis',(0.,0.,1.)) ;
#104846=DIRECTION('center_axis',(0.,-1.,0.)) ;
#104847=DIRECTION('ref_axis',(0.,0.,-1.)) ;
#104848=DIRECTION('center_axis',(-0.664363838829919,0.74740931868366,0.)) ;
#104849=DIRECTION('ref_axis',(-0.74740931868366,-0.664363838829919,0.)) ;
#104850=DIRECTION('center_axis',(-0.66436383882992,0.747409318683659,2.52106651083074E-15)) ;
#104851=DIRECTION('ref_axis',(-0.747409318683659,-0.66436383882992,7.82575143531171E-30)) ;
#104852=DIRECTION('center_axis',(-0.655772517804504,0.737744082530068,-0.160299948796656)) ;
#104853=DIRECTION('ref_axis',(-0.74740931868366,-0.664363838829919,2.31673158493852E-16)) ;
#104854=DIRECTION('center_axis',(0.655772517804496,-0.737744082530075,0.160299948796656)) ;
#104855=DIRECTION('ref_axis',(0.747409318683667,0.664363838829911,-2.10122272487167E-17)) ;
#104856=DIRECTION('center_axis',(0.,1.,0.)) ;
#104857=DIRECTION('ref_axis',(1.,0.,0.)) ;
#104858=DIRECTION('center_axis',(-0.873786407766988,-0.436893203883498,
0.213592233009711)) ;
#104859=DIRECTION('ref_axis',(-0.447213595499961,0.894427190999914,5.03515095507592E-16)) ;
#104860=DIRECTION('center_axis',(-0.948683298050516,0.316227766016832,-3.71868658652085E-15)) ;
#104861=DIRECTION('ref_axis',(0.316227766016832,0.948683298050516,-1.82909356595573E-12)) ;
#104862=DIRECTION('center_axis',(0.,1.,0.)) ;
#104863=DIRECTION('ref_axis',(1.,0.,0.)) ;
#104864=DIRECTION('center_axis',(-5.47915634355017E-14,1.,0.)) ;
#104865=DIRECTION('ref_axis',(1.,5.47915634355017E-14,0.)) ;
#104866=DIRECTION('center_axis',(-0.971399006496778,0.,0.23745309047699)) ;
#104867=DIRECTION('ref_axis',(0.23745309047699,0.,0.971399006496777)) ;
#104868=DIRECTION('center_axis',(0.971399006496778,-3.69787733965917E-15,
-0.237453090476989)) ;
#104869=DIRECTION('ref_axis',(-0.237453090476989,3.58403898099287E-30,-0.971399006496778)) ;
#104870=DIRECTION('center_axis',(0.873786407766991,0.436893203883493,-0.213592233009709)) ;
#104871=DIRECTION('ref_axis',(-0.447213595499956,0.894427190999917,2.83414331365695E-16)) ;
#104872=DIRECTION('center_axis',(-0.873786407766992,-0.436893203883492,
0.21359223300971)) ;
#104873=DIRECTION('ref_axis',(0.447213595499955,-0.894427190999918,-1.48231119036019E-16)) ;
#104874=DIRECTION('center_axis',(-0.894427190999917,-0.447213595499956,
0.)) ;
#104875=DIRECTION('ref_axis',(0.447213595499956,-0.894427190999917,0.)) ;
#104876=DIRECTION('center_axis',(-0.894427190999917,-0.447213595499955,
0.)) ;
#104877=DIRECTION('ref_axis',(0.447213595499955,-0.894427190999917,0.)) ;
#104878=DIRECTION('center_axis',(0.,1.,0.)) ;
#104879=DIRECTION('ref_axis',(0.,0.,1.)) ;
#104880=DIRECTION('center_axis',(2.66122351428257E-14,1.,6.50521303491301E-15)) ;
#104881=DIRECTION('ref_axis',(-1.,2.66122351428257E-14,3.84707242087163E-30)) ;
#104882=DIRECTION('center_axis',(-0.439210132004996,2.91128537537112E-13,
-0.898384360919175)) ;
#104883=DIRECTION('ref_axis',(0.898384360919175,-2.87197520732744E-11,-0.439210132004996)) ;
#104884=DIRECTION('center_axis',(0.,1.,0.)) ;
#104885=DIRECTION('ref_axis',(1.,0.,0.)) ;
#104886=DIRECTION('center_axis',(-0.87378640776699,-0.436893203883495,-0.213592233009712)) ;
#104887=DIRECTION('ref_axis',(-0.447213595499958,0.894427190999916,1.8708344946598E-16)) ;
#104888=DIRECTION('center_axis',(0.,0.,1.)) ;
#104889=DIRECTION('ref_axis',(1.,0.,0.)) ;
#104890=DIRECTION('center_axis',(0.439210132004893,2.5322537614034E-13,
-0.898384360919225)) ;
#104891=DIRECTION('ref_axis',(0.898384360919225,-2.39002175271898E-11,0.439210132004893)) ;
#104892=DIRECTION('center_axis',(-0.873786407766991,-0.436893203883493,
-0.213592233009709)) ;
#104893=DIRECTION('ref_axis',(0.447213595499956,-0.894427190999917,-1.06780556900622E-16)) ;
#104894=DIRECTION('center_axis',(-0.873786407766992,-0.436893203883492,
-0.213592233009707)) ;
#104895=DIRECTION('ref_axis',(0.447213595499955,-0.894427190999918,-7.04543255365314E-18)) ;
#104896=DIRECTION('center_axis',(-0.971399006496778,0.,-0.237453090476989)) ;
#104897=DIRECTION('ref_axis',(0.237453090476989,0.,-0.971399006496778)) ;
#104898=DIRECTION('center_axis',(0.971399006496778,0.,0.23745309047699)) ;
#104899=DIRECTION('ref_axis',(0.23745309047699,0.,-0.971399006496777)) ;
#104900=DIRECTION('center_axis',(0.,0.,-1.)) ;
#104901=DIRECTION('ref_axis',(-1.,0.,0.)) ;
#104902=DIRECTION('center_axis',(1.,1.0450141421547E-16,1.7416902369245E-17)) ;
#104903=DIRECTION('ref_axis',(-1.0450141421547E-16,1.,-1.82009092883888E-33)) ;
#104904=DIRECTION('center_axis',(0.672672795322785,0.73994007219006,-7.49271823359204E-10)) ;
#104905=DIRECTION('ref_axis',(0.738044870607466,-0.670949884714521,0.0715263669675738)) ;
#104906=DIRECTION('center_axis',(-1.,0.,0.)) ;
#104907=DIRECTION('ref_axis',(0.,-0.646374896130196,-0.763019982472726)) ;
#104908=DIRECTION('center_axis',(-1.,0.,0.)) ;
#104909=DIRECTION('ref_axis',(0.,0.,1.)) ;
#104910=DIRECTION('center_axis',(-1.,0.,0.)) ;
#104911=DIRECTION('ref_axis',(0.,0.,1.)) ;
#104912=DIRECTION('center_axis',(0.,0.986393923832144,0.164398987305357)) ;
#104913=DIRECTION('ref_axis',(0.,-0.164398987305357,0.986393923832144)) ;
#104914=DIRECTION('center_axis',(0.,-0.986393923832144,-0.164398987305358)) ;
#104915=DIRECTION('ref_axis',(0.,0.164398987305358,-0.986393923832144)) ;
#104916=DIRECTION('center_axis',(0.,0.,1.)) ;
#104917=DIRECTION('ref_axis',(1.,0.,0.)) ;
#104918=DIRECTION('center_axis',(0.,0.,1.)) ;
#104919=DIRECTION('ref_axis',(1.,0.,0.)) ;
#104920=DIRECTION('center_axis',(0.,0.,1.)) ;
#104921=DIRECTION('ref_axis',(1.,0.,0.)) ;
#104922=DIRECTION('center_axis',(0.,0.,-1.)) ;
#104923=DIRECTION('ref_axis',(1.,0.,0.)) ;
#104924=DIRECTION('center_axis',(-1.,0.,0.)) ;
#104925=DIRECTION('ref_axis',(0.,-0.646374896130195,-0.763019982472726)) ;
#104926=DIRECTION('center_axis',(0.,0.,1.)) ;
#104927=DIRECTION('ref_axis',(-1.,0.,0.)) ;
#104928=DIRECTION('center_axis',(1.,1.0450141421547E-16,-1.7416902369245E-17)) ;
#104929=DIRECTION('ref_axis',(-1.0450141421547E-16,1.,1.82009092883888E-33)) ;
#104930=DIRECTION('center_axis',(0.67267279532264,0.739940072190192,7.49194226733993E-10)) ;
#104931=DIRECTION('ref_axis',(0.738044870608016,-0.670949884714764,-0.0715263669596091)) ;
#104932=DIRECTION('center_axis',(1.,0.,0.)) ;
#104933=DIRECTION('ref_axis',(0.,-4.33680868994203E-15,1.)) ;
#104934=DIRECTION('center_axis',(0.,0.,-1.)) ;
#104935=DIRECTION('ref_axis',(-1.,0.,0.)) ;
#104936=DIRECTION('center_axis',(0.,-0.986393923832144,0.164398987305357)) ;
#104937=DIRECTION('ref_axis',(0.,-0.164398987305357,-0.986393923832144)) ;
#104938=DIRECTION('center_axis',(1.,0.,0.)) ;
#104939=DIRECTION('ref_axis',(0.,0.,1.)) ;
#104940=DIRECTION('center_axis',(7.58941520739854E-15,0.,-1.)) ;
#104941=DIRECTION('ref_axis',(-1.,0.,-7.58941520739854E-15)) ;
#104942=DIRECTION('center_axis',(1.,0.,-8.67361737988404E-15)) ;
#104943=DIRECTION('ref_axis',(-8.67361737988404E-15,0.,-1.)) ;
#104944=DIRECTION('center_axis',(1.,0.,0.)) ;
#104945=DIRECTION('ref_axis',(0.,0.,-1.)) ;
#104946=DIRECTION('center_axis',(1.,0.,8.67361737988403E-15)) ;
#104947=DIRECTION('ref_axis',(8.67361737988403E-15,0.,-1.)) ;
#104948=DIRECTION('center_axis',(0.,0.,1.)) ;
#104949=DIRECTION('ref_axis',(1.,0.,0.)) ;
#104950=DIRECTION('center_axis',(0.,0.,-1.)) ;
#104951=DIRECTION('ref_axis',(-1.,0.,0.)) ;
#104952=DIRECTION('center_axis',(1.,0.,0.)) ;
#104953=DIRECTION('ref_axis',(0.,0.,1.)) ;
#104954=DIRECTION('center_axis',(-6.50521303491304E-15,0.,-1.)) ;
#104955=DIRECTION('ref_axis',(-1.,0.,6.50521303491304E-15)) ;
#104956=DIRECTION('center_axis',(1.,0.,0.)) ;
#104957=DIRECTION('ref_axis',(0.,0.,1.)) ;
#104958=DIRECTION('center_axis',(1.,9.40395480657835E-30,8.67361737988403E-15)) ;
#104959=DIRECTION('ref_axis',(8.67361737988403E-15,1.69266015557823E-58,
-1.)) ;
#104960=DIRECTION('center_axis',(0.,0.,-1.)) ;
#104961=DIRECTION('ref_axis',(-1.,0.,0.)) ;
#104962=DIRECTION('center_axis',(6.50521303491304E-15,0.,-1.)) ;
#104963=DIRECTION('ref_axis',(-1.,0.,-6.50521303491304E-15)) ;
#104964=DIRECTION('center_axis',(-1.,0.,0.)) ;
#104965=DIRECTION('ref_axis',(0.,0.,1.)) ;
#104966=DIRECTION('center_axis',(1.,-8.67361737988409E-15,0.)) ;
#104967=DIRECTION('ref_axis',(8.67361737988409E-15,1.,0.)) ;
#104968=DIRECTION('center_axis',(1.,0.,0.)) ;
#104969=DIRECTION('ref_axis',(0.,0.,1.)) ;
#104970=DIRECTION('center_axis',(-4.33680868994202E-16,0.,1.)) ;
#104971=DIRECTION('ref_axis',(1.,0.,4.33680868994202E-16)) ;
#104972=DIRECTION('center_axis',(0.,0.,-1.)) ;
#104973=DIRECTION('ref_axis',(-1.,0.,0.)) ;
#104974=DIRECTION('center_axis',(0.,0.,1.)) ;
#104975=DIRECTION('ref_axis',(1.,0.,0.)) ;
#104976=DIRECTION('center_axis',(0.,1.,0.)) ;
#104977=DIRECTION('ref_axis',(0.,0.,1.)) ;
#104978=DIRECTION('center_axis',(-1.,0.,0.)) ;
#104979=DIRECTION('ref_axis',(0.,0.,-1.)) ;
#104980=DIRECTION('center_axis',(0.,-1.,0.)) ;
#104981=DIRECTION('ref_axis',(0.,0.,1.)) ;
#104982=DIRECTION('center_axis',(0.,1.,0.)) ;
#104983=DIRECTION('ref_axis',(0.,0.,1.)) ;
#104984=DIRECTION('center_axis',(0.,-1.,0.)) ;
#104985=DIRECTION('ref_axis',(0.,0.,1.)) ;
#104986=DIRECTION('center_axis',(-1.,0.,0.)) ;
#104987=DIRECTION('ref_axis',(0.,0.,-1.)) ;
#104988=DIRECTION('center_axis',(-1.,0.,-1.73472347597681E-16)) ;
#104989=DIRECTION('ref_axis',(-1.73472347597681E-16,0.,1.)) ;
#104990=DIRECTION('center_axis',(-1.,0.,0.)) ;
#104991=DIRECTION('ref_axis',(0.,0.,1.)) ;
#104992=DIRECTION('center_axis',(0.,1.,0.)) ;
#104993=DIRECTION('ref_axis',(0.,0.,1.)) ;
#104994=DIRECTION('center_axis',(0.,-1.,0.)) ;
#104995=DIRECTION('ref_axis',(0.,0.,-1.)) ;
#104996=DIRECTION('center_axis',(-4.33680868994202E-16,0.,1.)) ;
#104997=DIRECTION('ref_axis',(1.,0.,4.33680868994202E-16)) ;
#104998=DIRECTION('center_axis',(0.,0.,1.)) ;
#104999=DIRECTION('ref_axis',(1.,0.,0.)) ;
#105000=DIRECTION('center_axis',(0.,0.,-1.)) ;
#105001=DIRECTION('ref_axis',(-1.,0.,0.)) ;
#105002=DIRECTION('center_axis',(0.,1.,0.)) ;
#105003=DIRECTION('ref_axis',(0.,0.,1.)) ;
#105004=DIRECTION('center_axis',(0.,-1.,0.)) ;
#105005=DIRECTION('ref_axis',(0.,0.,-1.)) ;
#105006=DIRECTION('center_axis',(1.,0.,-1.73472347597681E-16)) ;
#105007=DIRECTION('ref_axis',(-1.73472347597681E-16,0.,-1.)) ;
#105008=DIRECTION('center_axis',(-1.,0.,0.)) ;
#105009=DIRECTION('ref_axis',(0.,0.,1.)) ;
#105010=DIRECTION('center_axis',(0.,0.,-1.)) ;
#105011=DIRECTION('ref_axis',(-1.,0.,0.)) ;
#105012=DIRECTION('center_axis',(0.,0.,1.)) ;
#105013=DIRECTION('ref_axis',(1.,0.,0.)) ;
#105014=DIRECTION('center_axis',(0.,0.,-1.)) ;
#105015=DIRECTION('ref_axis',(-1.,0.,0.)) ;
#105016=DIRECTION('center_axis',(0.,1.,0.)) ;
#105017=DIRECTION('ref_axis',(0.,0.,1.)) ;
#105018=DIRECTION('center_axis',(0.,-1.,0.)) ;
#105019=DIRECTION('ref_axis',(0.,0.,1.)) ;
#105020=DIRECTION('center_axis',(0.,1.,0.)) ;
#105021=DIRECTION('ref_axis',(1.,0.,0.)) ;
#105022=DIRECTION('center_axis',(1.,0.,0.)) ;
#105023=DIRECTION('ref_axis',(0.,0.,1.)) ;
#105024=DIRECTION('center_axis',(0.,1.,0.)) ;
#105025=DIRECTION('ref_axis',(1.,0.,0.)) ;
#105026=DIRECTION('center_axis',(1.,0.,0.)) ;
#105027=DIRECTION('ref_axis',(0.,0.,1.)) ;
#105028=DIRECTION('center_axis',(0.,1.,0.)) ;
#105029=DIRECTION('ref_axis',(0.,0.,1.)) ;
#105030=DIRECTION('center_axis',(0.,-1.,0.)) ;
#105031=DIRECTION('ref_axis',(0.,0.,1.)) ;
#105032=DIRECTION('center_axis',(0.,1.,0.)) ;
#105033=DIRECTION('ref_axis',(0.,0.,1.)) ;
#105034=DIRECTION('center_axis',(0.,-1.,0.)) ;
#105035=DIRECTION('ref_axis',(0.,0.,-1.)) ;
#105036=DIRECTION('center_axis',(-1.,0.,-1.73472347597681E-16)) ;
#105037=DIRECTION('ref_axis',(-1.73472347597681E-16,0.,1.)) ;
#105038=DIRECTION('center_axis',(1.,0.,0.)) ;
#105039=DIRECTION('ref_axis',(0.,0.,-1.)) ;
#105040=DIRECTION('center_axis',(1.,0.,-1.73472347597681E-16)) ;
#105041=DIRECTION('ref_axis',(-1.73472347597681E-16,0.,-1.)) ;
#105042=DIRECTION('center_axis',(1.,0.,0.)) ;
#105043=DIRECTION('ref_axis',(0.,0.,-1.)) ;
#105044=DIRECTION('center_axis',(0.,1.,0.)) ;
#105045=DIRECTION('ref_axis',(0.,0.,1.)) ;
#105046=DIRECTION('center_axis',(0.,-1.,0.)) ;
#105047=DIRECTION('ref_axis',(0.,0.,-1.)) ;
#105048=DIRECTION('center_axis',(0.,1.,0.)) ;
#105049=DIRECTION('ref_axis',(1.,0.,0.)) ;
#105050=DIRECTION('center_axis',(0.,0.,1.)) ;
#105051=DIRECTION('ref_axis',(-1.,0.,0.)) ;
#105052=DIRECTION('center_axis',(0.,1.,0.)) ;
#105053=DIRECTION('ref_axis',(1.,0.,0.)) ;
#105054=DIRECTION('center_axis',(0.,0.,-1.)) ;
#105055=DIRECTION('ref_axis',(1.,0.,0.)) ;
#105056=DIRECTION('center_axis',(0.,0.,-1.)) ;
#105057=DIRECTION('ref_axis',(-1.,0.,0.)) ;
#105058=DIRECTION('center_axis',(2.16840434497101E-16,0.,1.)) ;
#105059=DIRECTION('ref_axis',(1.,0.,-2.16840434497101E-16)) ;
#105060=DIRECTION('center_axis',(0.,0.,-1.)) ;
#105061=DIRECTION('ref_axis',(-1.,0.,0.)) ;
#105062=DIRECTION('center_axis',(0.,0.,1.)) ;
#105063=DIRECTION('ref_axis',(1.,0.,0.)) ;
#105064=DIRECTION('center_axis',(0.,-1.,0.)) ;
#105065=DIRECTION('ref_axis',(0.,0.,-1.)) ;
#105066=DIRECTION('center_axis',(1.,0.,0.)) ;
#105067=DIRECTION('ref_axis',(0.,0.,1.)) ;
#105068=DIRECTION('center_axis',(0.,1.,0.)) ;
#105069=DIRECTION('ref_axis',(0.,0.,-1.)) ;
#105070=DIRECTION('center_axis',(0.,-1.,0.)) ;
#105071=DIRECTION('ref_axis',(0.,0.,-1.)) ;
#105072=DIRECTION('center_axis',(0.,1.,0.)) ;
#105073=DIRECTION('ref_axis',(0.,0.,-1.)) ;
#105074=DIRECTION('center_axis',(1.,0.,0.)) ;
#105075=DIRECTION('ref_axis',(0.,0.,1.)) ;
#105076=DIRECTION('center_axis',(1.,0.,-1.73472347597681E-16)) ;
#105077=DIRECTION('ref_axis',(-1.73472347597681E-16,0.,-1.)) ;
#105078=DIRECTION('center_axis',(1.,0.,0.)) ;
#105079=DIRECTION('ref_axis',(0.,0.,-1.)) ;
#105080=DIRECTION('center_axis',(0.,-1.,0.)) ;
#105081=DIRECTION('ref_axis',(0.,0.,-1.)) ;
#105082=DIRECTION('center_axis',(0.,1.,0.)) ;
#105083=DIRECTION('ref_axis',(0.,0.,1.)) ;
#105084=DIRECTION('center_axis',(2.16840434497101E-16,0.,1.)) ;
#105085=DIRECTION('ref_axis',(1.,0.,-2.16840434497101E-16)) ;
#105086=DIRECTION('center_axis',(0.,0.,1.)) ;
#105087=DIRECTION('ref_axis',(1.,0.,0.)) ;
#105088=DIRECTION('center_axis',(0.,0.,-1.)) ;
#105089=DIRECTION('ref_axis',(-1.,0.,0.)) ;
#105090=DIRECTION('center_axis',(0.,-1.,0.)) ;
#105091=DIRECTION('ref_axis',(0.,0.,-1.)) ;
#105092=DIRECTION('center_axis',(0.,1.,0.)) ;
#105093=DIRECTION('ref_axis',(0.,0.,1.)) ;
#105094=DIRECTION('center_axis',(-1.,0.,1.73472347597681E-16)) ;
#105095=DIRECTION('ref_axis',(1.73472347597681E-16,0.,1.)) ;
#105096=DIRECTION('center_axis',(1.,0.,0.)) ;
#105097=DIRECTION('ref_axis',(0.,0.,-1.)) ;
#105098=DIRECTION('center_axis',(-2.16840434497101E-16,0.,-1.)) ;
#105099=DIRECTION('ref_axis',(-1.,0.,2.16840434497101E-16)) ;
#105100=DIRECTION('center_axis',(0.,0.,1.)) ;
#105101=DIRECTION('ref_axis',(1.,0.,0.)) ;
#105102=DIRECTION('center_axis',(0.,0.,-1.)) ;
#105103=DIRECTION('ref_axis',(-1.,0.,0.)) ;
#105104=DIRECTION('center_axis',(0.,-1.,0.)) ;
#105105=DIRECTION('ref_axis',(0.,0.,-1.)) ;
#105106=DIRECTION('center_axis',(0.,1.,0.)) ;
#105107=DIRECTION('ref_axis',(0.,0.,-1.)) ;
#105108=DIRECTION('center_axis',(0.,1.,0.)) ;
#105109=DIRECTION('ref_axis',(1.,0.,0.)) ;
#105110=DIRECTION('center_axis',(-1.,0.,0.)) ;
#105111=DIRECTION('ref_axis',(0.,0.,-1.)) ;
#105112=DIRECTION('center_axis',(0.,1.,0.)) ;
#105113=DIRECTION('ref_axis',(1.,0.,0.)) ;
#105114=DIRECTION('center_axis',(-1.,0.,0.)) ;
#105115=DIRECTION('ref_axis',(0.,0.,-1.)) ;
#105116=DIRECTION('center_axis',(0.,-1.,0.)) ;
#105117=DIRECTION('ref_axis',(0.,0.,-1.)) ;
#105118=DIRECTION('center_axis',(0.,1.,0.)) ;
#105119=DIRECTION('ref_axis',(0.,0.,-1.)) ;
#105120=DIRECTION('center_axis',(0.,-1.,0.)) ;
#105121=DIRECTION('ref_axis',(0.,0.,-1.)) ;
#105122=DIRECTION('center_axis',(0.,1.,0.)) ;
#105123=DIRECTION('ref_axis',(0.,0.,1.)) ;
#105124=DIRECTION('center_axis',(1.,0.,-1.73472347597681E-16)) ;
#105125=DIRECTION('ref_axis',(-1.73472347597681E-16,0.,-1.)) ;
#105126=DIRECTION('center_axis',(-1.,0.,0.)) ;
#105127=DIRECTION('ref_axis',(0.,0.,1.)) ;
#105128=DIRECTION('center_axis',(-1.,0.,1.73472347597681E-16)) ;
#105129=DIRECTION('ref_axis',(1.73472347597681E-16,0.,1.)) ;
#105130=DIRECTION('center_axis',(-1.,0.,0.)) ;
#105131=DIRECTION('ref_axis',(0.,0.,1.)) ;
#105132=DIRECTION('center_axis',(0.,-1.,0.)) ;
#105133=DIRECTION('ref_axis',(0.,0.,-1.)) ;
#105134=DIRECTION('center_axis',(0.,1.,0.)) ;
#105135=DIRECTION('ref_axis',(0.,0.,1.)) ;
#105136=DIRECTION('center_axis',(0.,1.,0.)) ;
#105137=DIRECTION('ref_axis',(1.,0.,0.)) ;
#105138=DIRECTION('center_axis',(0.,0.,1.)) ;
#105139=DIRECTION('ref_axis',(-1.,0.,0.)) ;
#105140=DIRECTION('center_axis',(0.,1.,0.)) ;
#105141=DIRECTION('ref_axis',(1.,0.,0.)) ;
#105142=DIRECTION('center_axis',(0.,0.,-1.)) ;
#105143=DIRECTION('ref_axis',(1.,0.,0.)) ;
#105144=DIRECTION('center_axis',(-2.16840434497101E-16,0.,-1.)) ;
#105145=DIRECTION('ref_axis',(-1.,0.,2.16840434497101E-16)) ;
#105146=DIRECTION('center_axis',(-1.,0.,0.)) ;
#105147=DIRECTION('ref_axis',(0.,0.,1.)) ;
#105148=DIRECTION('center_axis',(0.,-0.632948931301575,-0.774193548387091)) ;
#105149=DIRECTION('ref_axis',(0.,0.774193548387091,-0.632948931301575)) ;
#105150=DIRECTION('center_axis',(0.,1.,0.)) ;
#105151=DIRECTION('ref_axis',(1.,0.,0.)) ;
#105152=DIRECTION('center_axis',(-1.,0.,0.)) ;
#105153=DIRECTION('ref_axis',(0.,0.,-1.)) ;
#105154=DIRECTION('center_axis',(1.,0.,0.)) ;
#105155=DIRECTION('ref_axis',(0.,0.,-1.)) ;
#105156=DIRECTION('center_axis',(-1.,0.,0.)) ;
#105157=DIRECTION('ref_axis',(0.,0.,1.)) ;
#105158=DIRECTION('center_axis',(-1.,0.,0.)) ;
#105159=DIRECTION('ref_axis',(0.,0.,1.)) ;
#105160=DIRECTION('center_axis',(0.,-0.632948931301567,-0.774193548387097)) ;
#105161=DIRECTION('ref_axis',(0.,-0.774193548387097,0.632948931301567)) ;
#105162=DIRECTION('center_axis',(-1.,0.,0.)) ;
#105163=DIRECTION('ref_axis',(0.,0.,1.)) ;
#105164=DIRECTION('center_axis',(0.,0.632948931301567,-0.774193548387097)) ;
#105165=DIRECTION('ref_axis',(0.,0.774193548387097,0.632948931301567)) ;
#105166=DIRECTION('center_axis',(0.,0.,-1.)) ;
#105167=DIRECTION('ref_axis',(-1.,0.,0.)) ;
#105168=DIRECTION('center_axis',(0.,0.,1.)) ;
#105169=DIRECTION('ref_axis',(1.,0.,0.)) ;
#105170=DIRECTION('center_axis',(-1.,0.,0.)) ;
#105171=DIRECTION('ref_axis',(0.,0.,1.)) ;
#105172=DIRECTION('center_axis',(1.,0.,0.)) ;
#105173=DIRECTION('ref_axis',(0.,0.,1.)) ;
#105174=DIRECTION('center_axis',(1.,0.,0.)) ;
#105175=DIRECTION('ref_axis',(0.,0.,-1.)) ;
#105176=DIRECTION('center_axis',(1.,0.,0.)) ;
#105177=DIRECTION('ref_axis',(0.,0.,-1.)) ;
#105178=DIRECTION('center_axis',(0.,0.,1.)) ;
#105179=DIRECTION('ref_axis',(1.,0.,0.)) ;
#105180=DIRECTION('center_axis',(0.,8.67361737988405E-15,-1.)) ;
#105181=DIRECTION('ref_axis',(0.,1.,8.67361737988405E-15)) ;
#105182=DIRECTION('center_axis',(0.,1.,0.)) ;
#105183=DIRECTION('ref_axis',(1.,0.,0.)) ;
#105184=DIRECTION('center_axis',(1.22050154678007E-14,0.632948931301567,
-0.774193548387097)) ;
#105185=DIRECTION('ref_axis',(-2.03293076771647E-29,-0.774193548387097,
-0.632948931301567)) ;
#105186=DIRECTION('center_axis',(-1.,0.,0.)) ;
#105187=DIRECTION('ref_axis',(0.,0.,1.)) ;
#105188=DIRECTION('center_axis',(-0.422618261740697,0.,0.906307787036651)) ;
#105189=DIRECTION('ref_axis',(0.906307787036651,0.,0.422618261740697)) ;
#105190=DIRECTION('center_axis',(0.422618261740697,0.,-0.906307787036651)) ;
#105191=DIRECTION('ref_axis',(-0.906307787036651,0.,-0.422618261740697)) ;
#105192=DIRECTION('center_axis',(0.422618261740697,0.,-0.906307787036651)) ;
#105193=DIRECTION('ref_axis',(-0.906307787036651,0.,-0.422618261740697)) ;
#105194=DIRECTION('center_axis',(-0.422618261740697,0.,0.906307787036651)) ;
#105195=DIRECTION('ref_axis',(0.906307787036651,0.,0.422618261740697)) ;
#105196=DIRECTION('center_axis',(0.,1.,0.)) ;
#105197=DIRECTION('ref_axis',(1.,0.,0.)) ;
#105198=DIRECTION('center_axis',(0.,-0.986393923832144,0.164398987305358)) ;
#105199=DIRECTION('ref_axis',(0.,-0.164398987305358,-0.986393923832144)) ;
#105200=DIRECTION('center_axis',(0.,0.986393923832144,-0.164398987305357)) ;
#105201=DIRECTION('ref_axis',(0.,0.164398987305357,0.986393923832144)) ;
#105202=DIRECTION('center_axis',(0.,-0.986393923832144,0.164398987305358)) ;
#105203=DIRECTION('ref_axis',(0.,-0.164398987305358,-0.986393923832144)) ;
#105204=DIRECTION('center_axis',(-1.,0.,0.)) ;
#105205=DIRECTION('ref_axis',(0.,0.107567764393761,-0.994197755008192)) ;
#105206=DIRECTION('center_axis',(4.02631181035923E-15,-0.928404294083138,
-0.371571617226061)) ;
#105207=DIRECTION('ref_axis',(-2.55493810320452E-31,0.371571617226061,-0.928404294083138)) ;
#105208=DIRECTION('center_axis',(0.275516865537137,-0.50093975551097,-0.820457078800105)) ;
#105209=DIRECTION('ref_axis',(3.47276585739718E-16,0.853490367006418,-0.521108619605597)) ;
#105210=DIRECTION('center_axis',(0.,0.,-1.)) ;
#105211=DIRECTION('ref_axis',(-1.,0.,0.)) ;
#105212=DIRECTION('center_axis',(0.,0.,-1.)) ;
#105213=DIRECTION('ref_axis',(-1.,0.,0.)) ;
#105214=DIRECTION('center_axis',(-0.275516865538071,0.500939755523742,-0.820457078791993)) ;
#105215=DIRECTION('ref_axis',(-3.28467467648445E-16,0.853490366998217,0.521108619619028)) ;
#105216=DIRECTION('center_axis',(0.,-0.986393923832144,-0.164398987305357)) ;
#105217=DIRECTION('ref_axis',(0.,0.164398987305357,-0.986393923832144)) ;
#105218=DIRECTION('center_axis',(3.5648347838177E-16,0.986393923832144,
0.164398987305358)) ;
#105219=DIRECTION('ref_axis',(-1.58445824743934E-31,-0.164398987305358,
0.986393923832144)) ;
#105220=DIRECTION('center_axis',(0.,1.,0.)) ;
#105221=DIRECTION('ref_axis',(1.,0.,0.)) ;
#105222=DIRECTION('center_axis',(-1.,0.,0.)) ;
#105223=DIRECTION('ref_axis',(0.,0.,1.)) ;
#105224=DIRECTION('center_axis',(0.,0.,-1.)) ;
#105225=DIRECTION('ref_axis',(-1.,0.,0.)) ;
#105226=DIRECTION('center_axis',(2.168404344971E-15,0.,1.)) ;
#105227=DIRECTION('ref_axis',(1.,0.,-2.168404344971E-15)) ;
#105228=DIRECTION('center_axis',(0.795723237447208,-7.53302716311723E-12,
0.605660407643206)) ;
#105229=DIRECTION('ref_axis',(0.605660407643206,-1.95871398704475E-26,-0.795723237447208)) ;
#105230=DIRECTION('center_axis',(1.57772181044204E-26,2.36658271566302E-26,
1.)) ;
#105231=DIRECTION('ref_axis',(3.73380916671669E-52,-1.,2.36658271566302E-26)) ;
#105232=DIRECTION('center_axis',(-0.795723237415222,-2.11663082418553E-11,
0.605660407685229)) ;
#105233=DIRECTION('ref_axis',(0.605660407685229,9.32717726754359E-27,0.795723237415222)) ;
#105234=DIRECTION('center_axis',(0.,1.,0.)) ;
#105235=DIRECTION('ref_axis',(1.,0.,0.)) ;
#105236=DIRECTION('center_axis',(-0.716468671818951,0.697619267438901,0.)) ;
#105237=DIRECTION('ref_axis',(-0.697619267438901,-0.716468671818951,0.)) ;
#105238=DIRECTION('center_axis',(0.,-1.,0.)) ;
#105239=DIRECTION('ref_axis',(0.,0.,-1.)) ;
#105240=DIRECTION('center_axis',(0.,1.,0.)) ;
#105241=DIRECTION('ref_axis',(1.,0.,0.)) ;
#105242=DIRECTION('center_axis',(0.,-1.,0.)) ;
#105243=DIRECTION('ref_axis',(0.,0.,-1.)) ;
#105244=DIRECTION('center_axis',(-0.716468671818951,0.697619267438901,0.)) ;
#105245=DIRECTION('ref_axis',(-0.697619267438901,-0.716468671818951,0.)) ;
#105246=DIRECTION('center_axis',(0.,-1.,0.)) ;
#105247=DIRECTION('ref_axis',(0.,0.,-1.)) ;
#105248=DIRECTION('center_axis',(0.,-1.,0.)) ;
#105249=DIRECTION('ref_axis',(0.,0.,-1.)) ;
#105250=DIRECTION('center_axis',(0.716468671818953,-0.697619267438899,0.)) ;
#105251=DIRECTION('ref_axis',(0.697619267438899,0.716468671818953,0.)) ;
#105252=DIRECTION('center_axis',(-0.716468671818955,0.697619267438896,0.)) ;
#105253=DIRECTION('ref_axis',(-0.697619267438896,-0.716468671818955,0.)) ;
#105254=DIRECTION('center_axis',(-0.716468671818953,0.697619267438899,0.)) ;
#105255=DIRECTION('ref_axis',(-0.697619267438899,-0.716468671818953,0.)) ;
#105256=DIRECTION('center_axis',(-0.716468671818955,0.697619267438897,0.)) ;
#105257=DIRECTION('ref_axis',(-0.697619267438897,-0.716468671818955,0.)) ;
#105258=DIRECTION('center_axis',(0.,1.,0.)) ;
#105259=DIRECTION('ref_axis',(0.,0.,1.)) ;
#105260=DIRECTION('center_axis',(0.,-1.,0.)) ;
#105261=DIRECTION('ref_axis',(0.,0.,-1.)) ;
#105262=DIRECTION('center_axis',(0.,0.,1.)) ;
#105263=DIRECTION('ref_axis',(1.,0.,0.)) ;
#105264=DIRECTION('center_axis',(-0.891049746169499,0.453905661840951,0.)) ;
#105265=DIRECTION('ref_axis',(-0.453905661840951,-0.891049746169499,0.)) ;
#105266=DIRECTION('center_axis',(0.,1.,0.)) ;
#105267=DIRECTION('ref_axis',(1.,0.,0.)) ;
#105268=DIRECTION('center_axis',(-0.989044367093028,0.147618562252689,-1.28038692714842E-15)) ;
#105269=DIRECTION('ref_axis',(-0.147618562252689,-0.989044367093028,-5.00003579437924E-32)) ;
#105270=DIRECTION('center_axis',(0.,1.,0.)) ;
#105271=DIRECTION('ref_axis',(1.,0.,0.)) ;
#105272=DIRECTION('center_axis',(-0.989044367093028,0.147618562252688,0.)) ;
#105273=DIRECTION('ref_axis',(-0.147618562252688,-0.989044367093028,0.)) ;
#105274=DIRECTION('center_axis',(0.,0.,1.)) ;
#105275=DIRECTION('ref_axis',(1.,0.,0.)) ;
#105276=DIRECTION('center_axis',(-0.891049746169497,0.453905661840955,-3.93700403737147E-15)) ;
#105277=DIRECTION('ref_axis',(-0.453905661840955,-0.891049746169497,3.34787224203447E-31)) ;
#105278=DIRECTION('center_axis',(-0.891049746169503,0.453905661840943,0.)) ;
#105279=DIRECTION('ref_axis',(-0.453905661840943,-0.891049746169503,0.)) ;
#105280=DIRECTION('center_axis',(-0.891049746169501,0.453905661840946,0.)) ;
#105281=DIRECTION('ref_axis',(-0.453905661840946,-0.891049746169501,0.)) ;
#105282=DIRECTION('center_axis',(0.989044367093028,-0.147618562252691,0.)) ;
#105283=DIRECTION('ref_axis',(0.147618562252691,0.989044367093028,0.)) ;
#105284=DIRECTION('center_axis',(0.,0.,1.)) ;
#105285=DIRECTION('ref_axis',(1.,0.,0.)) ;
#105286=DIRECTION('center_axis',(0.,0.,-1.)) ;
#105287=DIRECTION('ref_axis',(-1.,0.,0.)) ;
#105288=DIRECTION('center_axis',(0.,0.,1.)) ;
#105289=DIRECTION('ref_axis',(1.,0.,0.)) ;
#105290=DIRECTION('center_axis',(-0.989044367093028,0.147618562252691,0.)) ;
#105291=DIRECTION('ref_axis',(-0.147618562252691,-0.989044367093028,0.)) ;
#105292=DIRECTION('center_axis',(0.891049746169503,-0.453905661840943,0.)) ;
#105293=DIRECTION('ref_axis',(0.453905661840943,0.891049746169503,0.)) ;
#105294=DIRECTION('center_axis',(-0.891049746169501,0.453905661840946,0.)) ;
#105295=DIRECTION('ref_axis',(-0.453905661840946,-0.891049746169501,0.)) ;
#105296=DIRECTION('center_axis',(0.,0.,1.)) ;
#105297=DIRECTION('ref_axis',(1.,0.,0.)) ;
#105298=DIRECTION('center_axis',(-1.,0.,0.)) ;
#105299=DIRECTION('ref_axis',(0.,0.,1.)) ;
#105300=DIRECTION('center_axis',(0.,1.,0.)) ;
#105301=DIRECTION('ref_axis',(0.,0.,-1.)) ;
#105302=DIRECTION('center_axis',(0.,1.,0.)) ;
#105303=DIRECTION('ref_axis',(0.,0.,-1.)) ;
#105304=DIRECTION('center_axis',(0.,0.,1.)) ;
#105305=DIRECTION('ref_axis',(1.,0.,0.)) ;
#105306=DIRECTION('center_axis',(-1.,0.,0.)) ;
#105307=DIRECTION('ref_axis',(0.,0.,1.)) ;
#105308=DIRECTION('center_axis',(-1.,2.60782465076463E-16,0.)) ;
#105309=DIRECTION('ref_axis',(-2.60782465076463E-16,-1.,0.)) ;
#105310=DIRECTION('center_axis',(-1.,0.,0.)) ;
#105311=DIRECTION('ref_axis',(0.,0.,1.)) ;
#105312=DIRECTION('center_axis',(0.,1.,0.)) ;
#105313=DIRECTION('ref_axis',(0.,0.,1.)) ;
#105314=DIRECTION('center_axis',(0.,1.,0.)) ;
#105315=DIRECTION('ref_axis',(0.,0.,1.)) ;
#105316=DIRECTION('center_axis',(0.,-1.,0.)) ;
#105317=DIRECTION('ref_axis',(0.,0.,-1.)) ;
#105318=DIRECTION('center_axis',(0.,1.,0.)) ;
#105319=DIRECTION('ref_axis',(0.,0.,1.)) ;
#105320=DIRECTION('center_axis',(1.,-2.60782465076463E-16,0.)) ;
#105321=DIRECTION('ref_axis',(2.60782465076463E-16,1.,0.)) ;
#105322=DIRECTION('center_axis',(-1.,0.,0.)) ;
#105323=DIRECTION('ref_axis',(0.,0.,1.)) ;
#105324=DIRECTION('center_axis',(-1.,0.,0.)) ;
#105325=DIRECTION('ref_axis',(0.,0.,1.)) ;
#105326=DIRECTION('center_axis',(0.,0.,-1.)) ;
#105327=DIRECTION('ref_axis',(1.,0.,0.)) ;
#105328=DIRECTION('center_axis',(-1.,0.,0.)) ;
#105329=DIRECTION('ref_axis',(0.,0.,1.)) ;
#105330=DIRECTION('center_axis',(0.,0.,1.)) ;
#105331=DIRECTION('ref_axis',(-1.,0.,0.)) ;
#105332=DIRECTION('center_axis',(0.,0.,1.)) ;
#105333=DIRECTION('ref_axis',(1.,0.,0.)) ;
#105334=DIRECTION('center_axis',(-1.,0.,0.)) ;
#105335=DIRECTION('ref_axis',(0.,0.,1.)) ;
#105336=DIRECTION('center_axis',(-1.,0.,0.)) ;
#105337=DIRECTION('ref_axis',(0.,0.,1.)) ;
#105338=DIRECTION('center_axis',(-3.56483478381767E-16,0.986393923832144,
0.164398987305358)) ;
#105339=DIRECTION('ref_axis',(-3.72967278346455E-31,-0.164398987305358,
0.986393923832144)) ;
#105340=DIRECTION('center_axis',(1.,0.,0.)) ;
#105341=DIRECTION('ref_axis',(0.,1.43114686768087E-13,1.)) ;
#105342=DIRECTION('center_axis',(-4.02631181035926E-15,0.928404294083138,
-0.371571617226061)) ;
#105343=DIRECTION('ref_axis',(-1.2864990704331E-29,0.371571617226061,0.928404294083138)) ;
#105344=DIRECTION('center_axis',(0.,-1.,0.)) ;
#105345=DIRECTION('ref_axis',(0.,0.,-1.)) ;
#105346=DIRECTION('center_axis',(0.,-1.,0.)) ;
#105347=DIRECTION('ref_axis',(0.,0.,-1.)) ;
#105348=DIRECTION('center_axis',(-1.,0.,-1.22464679914735E-16)) ;
#105349=DIRECTION('ref_axis',(-1.22464679914735E-16,0.,1.)) ;
#105350=DIRECTION('center_axis',(0.,1.,0.)) ;
#105351=DIRECTION('ref_axis',(0.,0.,-1.)) ;
#105352=DIRECTION('center_axis',(0.,1.,0.)) ;
#105353=DIRECTION('ref_axis',(0.,0.,-1.)) ;
#105354=DIRECTION('center_axis',(1.,0.,0.)) ;
#105355=DIRECTION('ref_axis',(0.,0.,-1.)) ;
#105356=DIRECTION('center_axis',(1.,0.,0.)) ;
#105357=DIRECTION('ref_axis',(0.,0.,-1.)) ;
#105358=DIRECTION('center_axis',(0.,1.,1.22464679914735E-16)) ;
#105359=DIRECTION('ref_axis',(0.,-1.22464679914735E-16,1.)) ;
#105360=DIRECTION('center_axis',(-1.,0.,0.)) ;
#105361=DIRECTION('ref_axis',(0.,0.,-1.)) ;
#105362=DIRECTION('center_axis',(-1.,0.,0.)) ;
#105363=DIRECTION('ref_axis',(0.,0.,1.)) ;
#105364=DIRECTION('center_axis',(-1.,0.,0.)) ;
#105365=DIRECTION('ref_axis',(0.,0.,1.)) ;
#105366=DIRECTION('center_axis',(0.,-1.,1.22464679914735E-16)) ;
#105367=DIRECTION('ref_axis',(0.,-1.22464679914735E-16,-1.)) ;
#105368=DIRECTION('center_axis',(1.,0.,0.)) ;
#105369=DIRECTION('ref_axis',(0.,0.,1.)) ;
#105370=DIRECTION('center_axis',(1.,0.,0.)) ;
#105371=DIRECTION('ref_axis',(0.,0.,1.)) ;
#105372=DIRECTION('center_axis',(-1.,0.,0.)) ;
#105373=DIRECTION('ref_axis',(0.,0.,1.)) ;
#105374=DIRECTION('center_axis',(-1.,0.,0.)) ;
#105375=DIRECTION('ref_axis',(0.,0.,1.)) ;
#105376=DIRECTION('center_axis',(0.,0.986393923832144,-0.164398987305358)) ;
#105377=DIRECTION('ref_axis',(0.,-0.164398987305358,-0.986393923832144)) ;
#105378=DIRECTION('center_axis',(1.,0.,0.)) ;
#105379=DIRECTION('ref_axis',(0.,0.,1.)) ;
#105380=DIRECTION('center_axis',(0.,0.,1.)) ;
#105381=DIRECTION('ref_axis',(1.,0.,0.)) ;
#105382=DIRECTION('center_axis',(0.,1.,0.)) ;
#105383=DIRECTION('ref_axis',(1.,0.,0.)) ;
#105384=DIRECTION('center_axis',(1.,0.,0.)) ;
#105385=DIRECTION('ref_axis',(0.,0.,-1.)) ;
#105386=DIRECTION('center_axis',(0.,0.,-1.)) ;
#105387=DIRECTION('ref_axis',(-1.,0.,0.)) ;
#105388=DIRECTION('center_axis',(0.,-0.986393923832144,0.164398987305358)) ;
#105389=DIRECTION('ref_axis',(0.,0.164398987305358,0.986393923832144)) ;
#105390=DIRECTION('center_axis',(-1.,0.,0.)) ;
#105391=DIRECTION('ref_axis',(0.,0.,1.)) ;
#105392=DIRECTION('',(1.,0.,0.)) ;
#105393=DIRECTION('center_axis',(-1.,0.,0.)) ;
#105394=DIRECTION('ref_axis',(0.,0.,1.)) ;
#105395=DIRECTION('',(-1.,0.,0.)) ;
#105396=DIRECTION('center_axis',(0.,1.,0.)) ;
#105397=DIRECTION('ref_axis',(1.,0.,0.)) ;
#105398=DIRECTION('center_axis',(0.,-0.986393923832144,-0.164398987305358)) ;
#105399=DIRECTION('ref_axis',(0.,-0.164398987305358,0.986393923832144)) ;
#105400=DIRECTION('center_axis',(0.,0.,1.)) ;
#105401=DIRECTION('ref_axis',(1.,0.,0.)) ;
#105402=DIRECTION('center_axis',(-1.,0.,0.)) ;
#105403=DIRECTION('ref_axis',(0.,0.,-1.)) ;
#105404=DIRECTION('center_axis',(1.,0.,0.)) ;
#105405=DIRECTION('ref_axis',(0.,0.,-1.)) ;
#105406=DIRECTION('center_axis',(1.,0.,0.)) ;
#105407=DIRECTION('ref_axis',(0.,0.,-1.)) ;
#105408=DIRECTION('',(0.707106781186546,-8.65956056235495E-17,0.707106781186549)) ;
#105409=DIRECTION('center_axis',(1.,0.,0.)) ;
#105410=DIRECTION('ref_axis',(0.,0.,-1.)) ;
#105411=DIRECTION('',(1.,0.,0.)) ;
#105412=DIRECTION('center_axis',(0.,1.,0.)) ;
#105413=DIRECTION('ref_axis',(0.,0.,1.)) ;
#105414=DIRECTION('center_axis',(0.,1.,0.)) ;
#105415=DIRECTION('ref_axis',(0.,0.,1.)) ;
#105416=DIRECTION('',(0.,1.,0.)) ;
#105417=DIRECTION('center_axis',(0.,1.,0.)) ;
#105418=DIRECTION('ref_axis',(0.,0.,1.)) ;
#105419=DIRECTION('',(0.,1.,0.)) ;
#105420=DIRECTION('center_axis',(0.,1.,0.)) ;
#105421=DIRECTION('ref_axis',(0.,0.,1.)) ;
#105422=DIRECTION('',(0.,1.,0.)) ;
#105423=DIRECTION('center_axis',(0.,1.,0.)) ;
#105424=DIRECTION('ref_axis',(0.,0.,1.)) ;
#105425=DIRECTION('',(0.,1.,0.)) ;
#105426=DIRECTION('center_axis',(0.,1.,0.)) ;
#105427=DIRECTION('ref_axis',(0.,0.,1.)) ;
#105428=DIRECTION('',(0.,1.,0.)) ;
#105429=DIRECTION('center_axis',(-1.,0.,0.)) ;
#105430=DIRECTION('ref_axis',(0.,0.,1.)) ;
#105431=DIRECTION('center_axis',(-1.,0.,0.)) ;
#105432=DIRECTION('ref_axis',(0.,0.,1.)) ;
#105433=DIRECTION('center_axis',(-3.56483478381767E-16,0.986393923832144,
0.164398987305358)) ;
#105434=DIRECTION('ref_axis',(-3.72967278346455E-31,-0.164398987305358,
0.986393923832144)) ;
#105435=DIRECTION('center_axis',(1.,0.,0.)) ;
#105436=DIRECTION('ref_axis',(0.,1.43114686768087E-13,1.)) ;
#105437=DIRECTION('center_axis',(-4.02631181035926E-15,0.928404294083138,
-0.371571617226061)) ;
#105438=DIRECTION('ref_axis',(-1.2864990704331E-29,0.371571617226061,0.928404294083138)) ;
#105439=DIRECTION('center_axis',(0.,0.,1.)) ;
#105440=DIRECTION('ref_axis',(1.,0.,0.)) ;
#105441=DIRECTION('center_axis',(0.,0.,1.)) ;
#105442=DIRECTION('ref_axis',(1.,0.,0.)) ;
#105443=DIRECTION('',(0.,0.,-1.)) ;
#105444=DIRECTION('center_axis',(0.,0.,-1.)) ;
#105445=DIRECTION('ref_axis',(1.,0.,0.)) ;
#105446=DIRECTION('',(0.,0.,1.)) ;
#105447=DIRECTION('center_axis',(0.,-1.,0.)) ;
#105448=DIRECTION('ref_axis',(0.,0.,-1.)) ;
#105449=DIRECTION('center_axis',(0.,-1.,0.)) ;
#105450=DIRECTION('ref_axis',(0.,0.,-1.)) ;
#105451=DIRECTION('center_axis',(-1.,0.,-1.22464679914735E-16)) ;
#105452=DIRECTION('ref_axis',(-1.22464679914735E-16,0.,1.)) ;
#105453=DIRECTION('center_axis',(0.,1.,0.)) ;
#105454=DIRECTION('ref_axis',(0.,0.,-1.)) ;
#105455=DIRECTION('center_axis',(0.,1.,0.)) ;
#105456=DIRECTION('ref_axis',(0.,0.,-1.)) ;
#105457=DIRECTION('center_axis',(1.,0.,0.)) ;
#105458=DIRECTION('ref_axis',(0.,0.,-1.)) ;
#105459=DIRECTION('center_axis',(1.,0.,0.)) ;
#105460=DIRECTION('ref_axis',(0.,0.,-1.)) ;
#105461=DIRECTION('center_axis',(0.,1.,1.22464679914735E-16)) ;
#105462=DIRECTION('ref_axis',(0.,-1.22464679914735E-16,1.)) ;
#105463=DIRECTION('center_axis',(-1.,0.,0.)) ;
#105464=DIRECTION('ref_axis',(0.,0.,-1.)) ;
#105465=DIRECTION('center_axis',(-1.,0.,0.)) ;
#105466=DIRECTION('ref_axis',(0.,0.,1.)) ;
#105467=DIRECTION('center_axis',(-1.,0.,0.)) ;
#105468=DIRECTION('ref_axis',(0.,0.,1.)) ;
#105469=DIRECTION('center_axis',(0.,-1.,1.22464679914735E-16)) ;
#105470=DIRECTION('ref_axis',(0.,-1.22464679914735E-16,-1.)) ;
#105471=DIRECTION('center_axis',(1.,0.,0.)) ;
#105472=DIRECTION('ref_axis',(0.,0.,1.)) ;
#105473=DIRECTION('center_axis',(1.,0.,0.)) ;
#105474=DIRECTION('ref_axis',(0.,0.,1.)) ;
#105475=DIRECTION('center_axis',(-1.,0.,0.)) ;
#105476=DIRECTION('ref_axis',(0.,0.,1.)) ;
#105477=DIRECTION('center_axis',(-1.,0.,0.)) ;
#105478=DIRECTION('ref_axis',(0.,0.,1.)) ;
#105479=DIRECTION('center_axis',(0.,0.986393923832144,-0.164398987305358)) ;
#105480=DIRECTION('ref_axis',(0.,-0.164398987305358,-0.986393923832144)) ;
#105481=DIRECTION('center_axis',(1.,0.,0.)) ;
#105482=DIRECTION('ref_axis',(0.,0.,1.)) ;
#105483=DIRECTION('center_axis',(0.,0.,1.)) ;
#105484=DIRECTION('ref_axis',(1.,0.,0.)) ;
#105485=DIRECTION('center_axis',(0.,1.,0.)) ;
#105486=DIRECTION('ref_axis',(1.,0.,0.)) ;
#105487=DIRECTION('center_axis',(1.,0.,0.)) ;
#105488=DIRECTION('ref_axis',(0.,0.,-1.)) ;
#105489=DIRECTION('center_axis',(0.,0.,-1.)) ;
#105490=DIRECTION('ref_axis',(-1.,0.,0.)) ;
#105491=DIRECTION('center_axis',(0.,-0.986393923832144,0.164398987305358)) ;
#105492=DIRECTION('ref_axis',(0.,0.164398987305358,0.986393923832144)) ;
#105493=DIRECTION('center_axis',(-1.,0.,0.)) ;
#105494=DIRECTION('ref_axis',(0.,0.,1.)) ;
#105495=DIRECTION('',(1.,0.,0.)) ;
#105496=DIRECTION('center_axis',(-1.,0.,0.)) ;
#105497=DIRECTION('ref_axis',(0.,0.,1.)) ;
#105498=DIRECTION('',(-1.,0.,0.)) ;
#105499=DIRECTION('center_axis',(0.,1.,0.)) ;
#105500=DIRECTION('ref_axis',(1.,0.,0.)) ;
#105501=DIRECTION('center_axis',(0.,-0.986393923832144,-0.164398987305358)) ;
#105502=DIRECTION('ref_axis',(0.,-0.164398987305358,0.986393923832144)) ;
#105503=DIRECTION('center_axis',(0.,0.,1.)) ;
#105504=DIRECTION('ref_axis',(1.,0.,0.)) ;
#105505=DIRECTION('center_axis',(-1.,0.,0.)) ;
#105506=DIRECTION('ref_axis',(0.,0.,-1.)) ;
#105507=DIRECTION('center_axis',(1.,0.,0.)) ;
#105508=DIRECTION('ref_axis',(0.,0.,-1.)) ;
#105509=DIRECTION('center_axis',(1.,0.,0.)) ;
#105510=DIRECTION('ref_axis',(0.,0.,-1.)) ;
#105511=DIRECTION('',(0.707106781186546,-8.65956056235495E-17,0.707106781186549)) ;
#105512=DIRECTION('center_axis',(1.,0.,0.)) ;
#105513=DIRECTION('ref_axis',(0.,0.,-1.)) ;
#105514=DIRECTION('',(1.,0.,0.)) ;
#105515=DIRECTION('center_axis',(0.,1.,0.)) ;
#105516=DIRECTION('ref_axis',(0.,0.,1.)) ;
#105517=DIRECTION('center_axis',(0.,1.,0.)) ;
#105518=DIRECTION('ref_axis',(0.,0.,1.)) ;
#105519=DIRECTION('',(0.,1.,0.)) ;
#105520=DIRECTION('center_axis',(0.,1.,0.)) ;
#105521=DIRECTION('ref_axis',(0.,0.,1.)) ;
#105522=DIRECTION('',(0.,1.,0.)) ;
#105523=DIRECTION('center_axis',(0.,1.,0.)) ;
#105524=DIRECTION('ref_axis',(0.,0.,1.)) ;
#105525=DIRECTION('',(0.,1.,0.)) ;
#105526=DIRECTION('center_axis',(0.,1.,0.)) ;
#105527=DIRECTION('ref_axis',(0.,0.,1.)) ;
#105528=DIRECTION('',(0.,1.,0.)) ;
#105529=DIRECTION('center_axis',(0.,1.,0.)) ;
#105530=DIRECTION('ref_axis',(0.,0.,1.)) ;
#105531=DIRECTION('',(0.,1.,0.)) ;
#105532=DIRECTION('center_axis',(-1.,0.,0.)) ;
#105533=DIRECTION('ref_axis',(0.,0.,1.)) ;
#105534=DIRECTION('',(0.,0.,1.)) ;
#105535=DIRECTION('',(0.,1.,0.)) ;
#105536=DIRECTION('',(0.,0.,-1.)) ;
#105537=DIRECTION('',(0.,1.,0.)) ;
#105538=DIRECTION('center_axis',(1.,0.,0.)) ;
#105539=DIRECTION('ref_axis',(0.,0.,1.)) ;
#105540=DIRECTION('',(0.,1.,0.)) ;
#105541=DIRECTION('',(0.,0.,-1.)) ;
#105542=DIRECTION('',(0.,-1.,0.)) ;
#105543=DIRECTION('center_axis',(1.,0.,0.)) ;
#105544=DIRECTION('ref_axis',(0.,0.,1.)) ;
#105545=DIRECTION('',(0.,0.,1.)) ;
#105546=DIRECTION('center_axis',(-3.46944695195361E-15,-1.,0.)) ;
#105547=DIRECTION('ref_axis',(1.,-3.46944695195361E-15,0.)) ;
#105548=DIRECTION('',(1.,-3.46944695195361E-15,0.)) ;
#105549=DIRECTION('',(0.,0.,1.)) ;
#105550=DIRECTION('',(-1.,3.46944695195361E-15,0.)) ;
#105551=DIRECTION('',(0.,0.,-1.)) ;
#105552=DIRECTION('center_axis',(-1.,0.,0.)) ;
#105553=DIRECTION('ref_axis',(0.,0.,1.)) ;
#105554=DIRECTION('',(0.,-1.,0.)) ;
#105555=DIRECTION('',(0.,0.,1.)) ;
#105556=DIRECTION('',(0.,1.,0.)) ;
#105557=DIRECTION('',(0.,0.,-1.)) ;
#105558=DIRECTION('center_axis',(0.,1.,0.)) ;
#105559=DIRECTION('ref_axis',(0.,0.,1.)) ;
#105560=DIRECTION('',(-1.,0.,0.)) ;
#105561=DIRECTION('',(0.,0.,1.)) ;
#105562=DIRECTION('',(1.,0.,0.)) ;
#105563=DIRECTION('',(0.,0.,-1.)) ;
#105564=DIRECTION('center_axis',(0.,0.,-1.)) ;
#105565=DIRECTION('ref_axis',(-1.,0.,0.)) ;
#105566=DIRECTION('center_axis',(0.,0.,1.)) ;
#105567=DIRECTION('ref_axis',(-1.,0.,0.)) ;
#105568=DIRECTION('',(0.,0.,-1.)) ;
#105569=DIRECTION('center_axis',(0.,0.,1.)) ;
#105570=DIRECTION('ref_axis',(1.,0.,0.)) ;
#105571=DIRECTION('center_axis',(0.,0.,1.)) ;
#105572=DIRECTION('ref_axis',(1.,0.,0.)) ;
#105573=DIRECTION('center_axis',(0.,0.,1.)) ;
#105574=DIRECTION('ref_axis',(-1.,0.,0.)) ;
#105575=DIRECTION('center_axis',(0.,0.,-1.)) ;
#105576=DIRECTION('ref_axis',(1.,0.,0.)) ;
#105577=DIRECTION('center_axis',(0.,0.,1.)) ;
#105578=DIRECTION('ref_axis',(1.,0.,0.)) ;
#105579=DIRECTION('center_axis',(0.,0.,1.)) ;
#105580=DIRECTION('ref_axis',(-1.,0.,0.)) ;
#105581=DIRECTION('center_axis',(0.,0.,-1.)) ;
#105582=DIRECTION('ref_axis',(1.,0.,0.)) ;
#105583=DIRECTION('center_axis',(0.,0.,-1.)) ;
#105584=DIRECTION('ref_axis',(-1.,0.,0.)) ;
#105585=DIRECTION('center_axis',(0.,0.,-1.)) ;
#105586=DIRECTION('ref_axis',(1.,0.,0.)) ;
#105587=DIRECTION('',(0.,0.,1.)) ;
#105588=DIRECTION('center_axis',(0.,0.,1.)) ;
#105589=DIRECTION('ref_axis',(-1.,3.46944695195362E-14,0.)) ;
#105590=DIRECTION('center_axis',(0.,0.,1.)) ;
#105591=DIRECTION('ref_axis',(1.,0.,0.)) ;
#105592=DIRECTION('',(0.,0.,1.)) ;
#105593=DIRECTION('center_axis',(-1.,0.,0.)) ;
#105594=DIRECTION('ref_axis',(0.,0.,1.)) ;
#105595=DIRECTION('center_axis',(-1.,0.,0.)) ;
#105596=DIRECTION('ref_axis',(0.,0.,1.)) ;
#105597=DIRECTION('',(0.,0.,-1.)) ;
#105598=DIRECTION('',(0.,1.,0.)) ;
#105599=DIRECTION('',(0.,0.,1.)) ;
#105600=DIRECTION('center_axis',(-2.09002828430941E-16,1.,0.)) ;
#105601=DIRECTION('ref_axis',(-1.,-2.09002828430941E-16,0.)) ;
#105602=DIRECTION('',(0.,0.,1.)) ;
#105603=DIRECTION('',(-1.,-2.09002828430941E-16,0.)) ;
#105604=DIRECTION('',(0.,0.,-1.)) ;
#105605=DIRECTION('',(1.,2.09002828430941E-16,0.)) ;
#105606=DIRECTION('center_axis',(1.0450141421547E-16,-1.,0.)) ;
#105607=DIRECTION('ref_axis',(1.,1.0450141421547E-16,0.)) ;
#105608=DIRECTION('',(-1.,-1.0450141421547E-16,0.)) ;
#105609=DIRECTION('',(0.,0.,1.)) ;
#105610=DIRECTION('',(1.,1.0450141421547E-16,1.7416902369245E-17)) ;
#105611=DIRECTION('',(0.,0.,-1.)) ;
#105612=DIRECTION('center_axis',(0.,1.,0.)) ;
#105613=DIRECTION('ref_axis',(0.,0.,1.)) ;
#105614=DIRECTION('',(0.422618261740697,0.,-0.906307787036651)) ;
#105615=DIRECTION('center_axis',(-1.,0.,0.)) ;
#105616=DIRECTION('ref_axis',(0.,0.,1.)) ;
#105617=DIRECTION('',(0.,0.986393923832144,-0.164398987305357)) ;
#105618=DIRECTION('',(0.,0.,1.)) ;
#105619=DIRECTION('',(0.,-0.986393923832144,-0.164398987305357)) ;
#105620=DIRECTION('center_axis',(1.,0.,0.)) ;
#105621=DIRECTION('ref_axis',(0.,0.,1.)) ;
#105622=DIRECTION('',(0.,0.,1.)) ;
#105623=DIRECTION('',(0.,0.986393923832144,-0.164398987305357)) ;
#105624=DIRECTION('',(0.,0.,1.)) ;
#105625=DIRECTION('',(0.,1.,0.)) ;
#105626=DIRECTION('',(0.,0.,-1.)) ;
#105627=DIRECTION('center_axis',(1.,0.,0.)) ;
#105628=DIRECTION('ref_axis',(0.,2.6020852139652E-14,1.)) ;
#105629=DIRECTION('center_axis',(1.,0.,0.)) ;
#105630=DIRECTION('ref_axis',(0.,8.88178419700125E-16,1.)) ;
#105631=DIRECTION('center_axis',(1.,0.,0.)) ;
#105632=DIRECTION('ref_axis',(0.,0.,1.)) ;
#105633=DIRECTION('',(0.,0.,-1.)) ;
#105634=DIRECTION('center_axis',(1.,0.,0.)) ;
#105635=DIRECTION('ref_axis',(0.,0.,1.)) ;
#105636=DIRECTION('center_axis',(1.,0.,0.)) ;
#105637=DIRECTION('ref_axis',(0.,0.,1.)) ;
#105638=DIRECTION('center_axis',(1.,0.,0.)) ;
#105639=DIRECTION('ref_axis',(0.,0.,1.)) ;
#105640=DIRECTION('',(0.,0.,-1.)) ;
#105641=DIRECTION('',(0.,1.,0.)) ;
#105642=DIRECTION('',(0.,0.,1.)) ;
#105643=DIRECTION('',(0.,-0.986393923832144,-0.164398987305357)) ;
#105644=DIRECTION('center_axis',(1.,0.,0.)) ;
#105645=DIRECTION('ref_axis',(0.,0.,1.)) ;
#105646=DIRECTION('',(0.,0.,1.)) ;
#105647=DIRECTION('center_axis',(1.0450141421547E-16,-1.,0.)) ;
#105648=DIRECTION('ref_axis',(1.,1.0450141421547E-16,0.)) ;
#105649=DIRECTION('',(-1.,-1.0450141421547E-16,1.7416902369245E-17)) ;
#105650=DIRECTION('',(0.,0.,1.)) ;
#105651=DIRECTION('',(1.,1.0450141421547E-16,1.7416902369245E-17)) ;
#105652=DIRECTION('',(0.,0.,-1.)) ;
#105653=DIRECTION('center_axis',(-0.876215908676647,-0.481918749772156,
0.)) ;
#105654=DIRECTION('ref_axis',(0.481918749772156,-0.876215908676647,0.)) ;
#105655=DIRECTION('',(0.,0.,1.)) ;
#105656=DIRECTION('',(-0.481918749772156,0.876215908676647,0.)) ;
#105657=DIRECTION('',(0.,0.,-1.)) ;
#105658=DIRECTION('center_axis',(-0.87621590867669,-0.481918749772079,-2.87461714907713E-14)) ;
#105659=DIRECTION('ref_axis',(0.436954455884537,-0.794462647062935,-0.421781822633934)) ;
#105660=DIRECTION('',(0.,0.,-1.)) ;
#105661=DIRECTION('center_axis',(-0.876215908676657,-0.481918749772137,
4.26347712001692E-15)) ;
#105662=DIRECTION('ref_axis',(0.436954455989552,-0.794462647253768,0.421781822165689)) ;
#105663=DIRECTION('',(0.,0.,-1.)) ;
#105664=DIRECTION('center_axis',(-0.876215908676638,-0.481918749772173,
5.32934639996306E-15)) ;
#105665=DIRECTION('ref_axis',(0.436954455831528,-0.794462646966382,-0.421781822870715)) ;
#105666=DIRECTION('',(0.,0.,-1.)) ;
#105667=DIRECTION('center_axis',(-0.876215908676651,-0.481918749772149,
9.43132817458479E-15)) ;
#105668=DIRECTION('ref_axis',(0.436954455977753,-0.794462647232284,0.42178182221838)) ;
#105669=DIRECTION('',(0.,0.,-1.)) ;
#105670=DIRECTION('',(-0.481918749772156,0.876215908676647,0.)) ;
#105671=DIRECTION('center_axis',(-0.876215908676647,-0.481918749772156,
0.)) ;
#105672=DIRECTION('ref_axis',(0.481918749772156,-0.876215908676647,0.)) ;
#105673=DIRECTION('',(-0.481918749772156,0.876215908676647,0.)) ;
#105674=DIRECTION('',(-0.481918749772156,0.876215908676647,0.)) ;
#105675=DIRECTION('',(0.,0.,-1.)) ;
#105676=DIRECTION('center_axis',(-1.,0.,0.)) ;
#105677=DIRECTION('ref_axis',(0.,0.,1.)) ;
#105678=DIRECTION('',(0.,1.,0.)) ;
#105679=DIRECTION('',(0.,0.,1.)) ;
#105680=DIRECTION('',(0.,1.,0.)) ;
#105681=DIRECTION('',(0.,1.,0.)) ;
#105682=DIRECTION('center_axis',(0.,-1.,0.)) ;
#105683=DIRECTION('ref_axis',(0.,0.,-1.)) ;
#105684=DIRECTION('',(-1.,0.,0.)) ;
#105685=DIRECTION('',(0.,0.,1.)) ;
#105686=DIRECTION('',(-1.,0.,0.)) ;
#105687=DIRECTION('',(0.,0.,-1.)) ;
#105688=DIRECTION('center_axis',(0.,1.,0.)) ;
#105689=DIRECTION('ref_axis',(0.,0.,-1.)) ;
#105690=DIRECTION('',(2.16840434497101E-16,0.,1.)) ;
#105691=DIRECTION('center_axis',(0.,1.,0.)) ;
#105692=DIRECTION('ref_axis',(0.,0.,-1.)) ;
#105693=DIRECTION('',(-1.,0.,1.73472347597681E-16)) ;
#105694=DIRECTION('center_axis',(0.,1.,0.)) ;
#105695=DIRECTION('ref_axis',(0.,0.,-1.)) ;
#105696=DIRECTION('',(-2.16840434497101E-16,0.,-1.)) ;
#105697=DIRECTION('center_axis',(0.,1.,0.)) ;
#105698=DIRECTION('ref_axis',(0.,0.,-1.)) ;
#105699=DIRECTION('',(1.,0.,-1.73472347597681E-16)) ;
#105700=DIRECTION('center_axis',(0.,1.,0.)) ;
#105701=DIRECTION('ref_axis',(0.,0.,-1.)) ;
#105702=DIRECTION('',(2.16840434497101E-16,0.,1.)) ;
#105703=DIRECTION('center_axis',(0.,1.,0.)) ;
#105704=DIRECTION('ref_axis',(0.,0.,-1.)) ;
#105705=DIRECTION('',(-1.,0.,1.73472347597681E-16)) ;
#105706=DIRECTION('center_axis',(0.,1.,0.)) ;
#105707=DIRECTION('ref_axis',(0.,0.,-1.)) ;
#105708=DIRECTION('',(-2.16840434497101E-16,0.,-1.)) ;
#105709=DIRECTION('center_axis',(0.,1.,0.)) ;
#105710=DIRECTION('ref_axis',(0.,0.,-1.)) ;
#105711=DIRECTION('',(1.,0.,-1.73472347597681E-16)) ;
#105712=DIRECTION('center_axis',(1.,0.,0.)) ;
#105713=DIRECTION('ref_axis',(0.,0.,-1.)) ;
#105714=DIRECTION('',(0.,-1.,0.)) ;
#105715=DIRECTION('',(0.,0.,1.)) ;
#105716=DIRECTION('',(0.,-1.,0.)) ;
#105717=DIRECTION('',(0.,0.,-1.)) ;
#105718=DIRECTION('center_axis',(0.,1.,0.)) ;
#105719=DIRECTION('ref_axis',(0.,0.,1.)) ;
#105720=DIRECTION('',(1.,0.,0.)) ;
#105721=DIRECTION('',(1.,0.,0.)) ;
#105722=DIRECTION('',(0.,0.,-1.)) ;
#105723=DIRECTION('center_axis',(0.98058067569092,-0.196116135138184,0.)) ;
#105724=DIRECTION('ref_axis',(0.196116135138184,0.98058067569092,0.)) ;
#105725=DIRECTION('',(-0.196116135138184,-0.98058067569092,0.)) ;
#105726=DIRECTION('',(0.,0.,1.)) ;
#105727=DIRECTION('',(-0.196116135138184,-0.98058067569092,0.)) ;
#105728=DIRECTION('center_axis',(1.,0.,0.)) ;
#105729=DIRECTION('ref_axis',(0.,0.,-1.)) ;
#105730=DIRECTION('',(0.,-1.,0.)) ;
#105731=DIRECTION('',(0.,0.,1.)) ;
#105732=DIRECTION('',(0.,-1.,0.)) ;
#105733=DIRECTION('',(0.,0.,-1.)) ;
#105734=DIRECTION('',(0.,0.,1.)) ;
#105735=DIRECTION('',(0.,-1.,0.)) ;
#105736=DIRECTION('',(0.,0.,-1.)) ;
#105737=DIRECTION('',(0.,1.,0.)) ;
#105738=DIRECTION('',(0.,0.,1.)) ;
#105739=DIRECTION('',(0.,-1.,0.)) ;
#105740=DIRECTION('',(0.,0.,-1.)) ;
#105741=DIRECTION('',(0.,1.,0.)) ;
#105742=DIRECTION('center_axis',(0.,1.,0.)) ;
#105743=DIRECTION('ref_axis',(0.,0.,1.)) ;
#105744=DIRECTION('',(1.,0.,0.)) ;
#105745=DIRECTION('',(0.,0.,1.)) ;
#105746=DIRECTION('',(1.,0.,0.)) ;
#105747=DIRECTION('',(0.,0.,-1.)) ;
#105748=DIRECTION('center_axis',(0.,-1.,0.)) ;
#105749=DIRECTION('ref_axis',(0.,0.,1.)) ;
#105750=DIRECTION('',(0.,0.,1.)) ;
#105751=DIRECTION('center_axis',(0.,-1.,0.)) ;
#105752=DIRECTION('ref_axis',(0.,0.,1.)) ;
#105753=DIRECTION('',(1.,0.,1.73472347597681E-16)) ;
#105754=DIRECTION('center_axis',(0.,-1.,0.)) ;
#105755=DIRECTION('ref_axis',(0.,0.,1.)) ;
#105756=DIRECTION('',(4.33680868994202E-16,0.,-1.)) ;
#105757=DIRECTION('center_axis',(0.,-1.,0.)) ;
#105758=DIRECTION('ref_axis',(0.,0.,1.)) ;
#105759=DIRECTION('',(-1.,0.,1.73472347597681E-16)) ;
#105760=DIRECTION('center_axis',(0.,-1.,0.)) ;
#105761=DIRECTION('ref_axis',(0.,0.,1.)) ;
#105762=DIRECTION('',(0.,0.,1.)) ;
#105763=DIRECTION('center_axis',(0.,-1.,0.)) ;
#105764=DIRECTION('ref_axis',(0.,0.,1.)) ;
#105765=DIRECTION('',(1.,0.,1.73472347597681E-16)) ;
#105766=DIRECTION('center_axis',(0.,-1.,0.)) ;
#105767=DIRECTION('ref_axis',(0.,0.,1.)) ;
#105768=DIRECTION('',(4.33680868994202E-16,0.,-1.)) ;
#105769=DIRECTION('center_axis',(0.,-1.,0.)) ;
#105770=DIRECTION('ref_axis',(0.,0.,1.)) ;
#105771=DIRECTION('',(-1.,0.,1.73472347597681E-16)) ;
#105772=DIRECTION('center_axis',(-1.,6.93889390390723E-16,0.)) ;
#105773=DIRECTION('ref_axis',(-6.93889390390723E-16,-1.,0.)) ;
#105774=DIRECTION('',(6.93889390390723E-16,1.,0.)) ;
#105775=DIRECTION('',(0.,0.,1.)) ;
#105776=DIRECTION('',(6.93889390390723E-16,1.,0.)) ;
#105777=DIRECTION('',(0.,0.,-1.)) ;
#105778=DIRECTION('center_axis',(0.,1.,0.)) ;
#105779=DIRECTION('ref_axis',(0.,0.,1.)) ;
#105780=DIRECTION('',(0.,0.,1.)) ;
#105781=DIRECTION('',(0.,0.,1.)) ;
#105782=DIRECTION('',(1.,0.,0.)) ;
#105783=DIRECTION('',(0.,0.,-1.)) ;
#105784=DIRECTION('',(1.,0.,0.)) ;
#105785=DIRECTION('',(0.,0.,1.)) ;
#105786=DIRECTION('center_axis',(-1.,0.,0.)) ;
#105787=DIRECTION('ref_axis',(0.,0.,1.)) ;
#105788=DIRECTION('',(0.,0.,1.)) ;
#105789=DIRECTION('center_axis',(-1.,0.,0.)) ;
#105790=DIRECTION('ref_axis',(0.,0.,1.)) ;
#105791=DIRECTION('',(0.,0.,-1.)) ;
#105792=DIRECTION('center_axis',(-1.,0.,0.)) ;
#105793=DIRECTION('ref_axis',(0.,0.,1.)) ;
#105794=DIRECTION('center_axis',(-2.09002828430941E-16,1.,0.)) ;
#105795=DIRECTION('ref_axis',(-1.,-2.09002828430941E-16,0.)) ;
#105796=DIRECTION('',(-1.,-2.09002828430941E-16,0.)) ;
#105797=DIRECTION('',(0.,0.,-1.)) ;
#105798=DIRECTION('',(1.,2.09002828430941E-16,0.)) ;
#105799=DIRECTION('',(0.,0.,1.)) ;
#105800=DIRECTION('center_axis',(0.,0.,1.)) ;
#105801=DIRECTION('ref_axis',(1.,0.,0.)) ;
#105802=DIRECTION('center_axis',(0.,0.,-1.)) ;
#105803=DIRECTION('ref_axis',(1.,0.,0.)) ;
#105804=DIRECTION('center_axis',(0.,0.,-1.)) ;
#105805=DIRECTION('ref_axis',(1.,1.04083408558609E-13,0.)) ;
#105806=DIRECTION('center_axis',(0.,0.,1.)) ;
#105807=DIRECTION('ref_axis',(1.,0.,0.)) ;
#105808=DIRECTION('center_axis',(0.,0.,1.)) ;
#105809=DIRECTION('ref_axis',(1.,0.,0.)) ;
#105810=DIRECTION('center_axis',(0.,0.,-1.)) ;
#105811=DIRECTION('ref_axis',(1.,1.30104260698261E-14,0.)) ;
#105812=DIRECTION('center_axis',(0.,0.,-1.)) ;
#105813=DIRECTION('ref_axis',(1.,0.,0.)) ;
#105814=DIRECTION('center_axis',(0.,0.,1.)) ;
#105815=DIRECTION('ref_axis',(1.,0.,0.)) ;
#105816=DIRECTION('center_axis',(0.,0.,-1.)) ;
#105817=DIRECTION('ref_axis',(1.,0.,0.)) ;
#105818=DIRECTION('center_axis',(0.,0.,1.)) ;
#105819=DIRECTION('ref_axis',(1.,0.,0.)) ;
#105820=DIRECTION('center_axis',(0.,0.,-1.)) ;
#105821=DIRECTION('ref_axis',(1.,0.,0.)) ;
#105822=DIRECTION('center_axis',(0.,0.,-1.)) ;
#105823=DIRECTION('ref_axis',(1.,0.,0.)) ;
#105824=DIRECTION('center_axis',(0.,0.,-1.)) ;
#105825=DIRECTION('ref_axis',(1.,2.6020852139652E-14,0.)) ;
#105826=DIRECTION('center_axis',(0.,0.,-1.)) ;
#105827=DIRECTION('ref_axis',(1.,0.,0.)) ;
#105828=DIRECTION('center_axis',(0.,0.,-1.)) ;
#105829=DIRECTION('ref_axis',(1.,0.,0.)) ;
#105830=DIRECTION('center_axis',(0.,0.,1.)) ;
#105831=DIRECTION('ref_axis',(1.,0.,0.)) ;
#105832=DIRECTION('',(-0.664363838829919,0.74740931868366,0.)) ;
#105833=DIRECTION('',(0.,-1.,0.)) ;
#105834=DIRECTION('',(0.894427190999917,0.447213595499956,0.)) ;
#105835=DIRECTION('',(0.,1.,0.)) ;
#105836=DIRECTION('center_axis',(0.,0.,-1.)) ;
#105837=DIRECTION('ref_axis',(-1.,0.,0.)) ;
#105838=DIRECTION('',(-0.894427190999917,-0.447213595499956,0.)) ;
#105839=DIRECTION('',(0.,1.,0.)) ;
#105840=DIRECTION('',(0.664363838829919,-0.74740931868366,0.)) ;
#105841=DIRECTION('',(0.,-1.,0.)) ;
#105842=DIRECTION('center_axis',(-0.23745309047699,0.,-0.971399006496778)) ;
#105843=DIRECTION('ref_axis',(-0.971399006496778,0.,0.23745309047699)) ;
#105844=DIRECTION('center_axis',(-0.237453090476988,5.12980051156625E-14,
-0.971399006496778)) ;
#105845=DIRECTION('ref_axis',(0.921799787670952,-0.315455332293199,-0.225328836986247)) ;
#105846=DIRECTION('',(0.971399006496777,0.,-0.23745309047699)) ;
#105847=DIRECTION('',(0.,-1.,0.)) ;
#105848=DIRECTION('',(-0.971399006496777,0.,0.23745309047699)) ;
#105849=DIRECTION('center_axis',(-0.23745309047692,-4.15843437570133E-13,
-0.971399006496795)) ;
#105850=DIRECTION('ref_axis',(0.9545593542551,0.185392581166527,-0.233336731040142)) ;
#105851=DIRECTION('',(-0.873786407766991,-0.436893203883493,0.213592233009709)) ;
#105852=DIRECTION('',(0.,1.,0.)) ;
#105853=DIRECTION('',(0.655772517804503,-0.737744082530068,-0.160299948796656)) ;
#105854=DIRECTION('center_axis',(-1.,0.,0.)) ;
#105855=DIRECTION('ref_axis',(0.,0.,1.)) ;
#105856=DIRECTION('',(0.,-1.,0.)) ;
#105857=DIRECTION('center_axis',(-1.,-6.70078870827245E-15,-6.50913949396088E-15)) ;
#105858=DIRECTION('ref_axis',(6.50913949389232E-15,1.02323485816278E-11,
-1.)) ;
#105859=DIRECTION('',(0.,0.,-1.)) ;
#105860=DIRECTION('center_axis',(-1.,-6.70078870827188E-15,6.50913949396004E-15)) ;
#105861=DIRECTION('ref_axis',(-6.5091394941529E-15,2.87817090394427E-11,
-1.)) ;
#105862=DIRECTION('center_axis',(-1.,6.70078870827192E-15,6.50913949396007E-15)) ;
#105863=DIRECTION('ref_axis',(-6.50913949414225E-15,-2.71882442700375E-11,
-1.)) ;
#105864=DIRECTION('',(0.,0.,-1.)) ;
#105865=DIRECTION('center_axis',(-1.,6.70078870827247E-15,-6.50913949396088E-15)) ;
#105866=DIRECTION('ref_axis',(6.50913949373767E-15,-3.33117585083476E-11,
-1.)) ;
#105867=DIRECTION('center_axis',(-0.23745309047699,0.,0.971399006496778)) ;
#105868=DIRECTION('ref_axis',(0.971399006496778,0.,0.23745309047699)) ;
#105869=DIRECTION('center_axis',(-0.237453090476876,-4.17061728891309E-13,
0.971399006496805)) ;
#105870=DIRECTION('ref_axis',(0.954559354253017,0.185392581177947,0.233336731039587)) ;
#105871=DIRECTION('',(0.971399006496777,0.,0.23745309047699)) ;
#105872=DIRECTION('',(-0.971399006496777,0.,-0.23745309047699)) ;
#105873=DIRECTION('center_axis',(-0.237453090476943,1.57363445644675E-13,
0.971399006496789)) ;
#105874=DIRECTION('ref_axis',(0.921799787671554,-0.315455332291342,0.225328836986384)) ;
#105875=DIRECTION('',(-0.655772517804503,0.737744082530068,-0.160299948796656)) ;
#105876=DIRECTION('',(0.,-1.,0.)) ;
#105877=DIRECTION('',(0.873786407766991,0.436893203883493,0.213592233009709)) ;
#105878=DIRECTION('center_axis',(0.,1.,0.)) ;
#105879=DIRECTION('ref_axis',(0.,0.,1.)) ;
#105880=DIRECTION('',(-0.971399006496777,0.,0.23745309047699)) ;
#105881=DIRECTION('',(0.,0.,-1.)) ;
#105882=DIRECTION('',(0.971399006496777,0.,0.23745309047699)) ;
#105883=DIRECTION('center_axis',(0.,1.,0.)) ;
#105884=DIRECTION('ref_axis',(0.,0.,1.)) ;
#105885=DIRECTION('',(-0.971399006496777,0.,-0.23745309047699)) ;
#105886=DIRECTION('',(0.,0.,1.)) ;
#105887=DIRECTION('',(0.971399006496777,0.,-0.23745309047699)) ;
#105888=DIRECTION('center_axis',(-0.447213595499956,0.894427190999917,0.)) ;
#105889=DIRECTION('ref_axis',(0.,0.,-1.)) ;
#105890=DIRECTION('',(0.,0.,-1.)) ;
#105891=DIRECTION('',(-0.873786407766991,-0.436893203883493,-0.213592233009709)) ;
#105892=DIRECTION('',(-0.894427190999917,-0.447213595499956,0.)) ;
#105893=DIRECTION('',(0.,0.,1.)) ;
#105894=DIRECTION('',(0.894427190999917,0.447213595499956,0.)) ;
#105895=DIRECTION('',(0.873786407766991,0.436893203883493,-0.213592233009709)) ;
#105896=DIRECTION('center_axis',(0.74740931868366,0.664363838829919,0.)) ;
#105897=DIRECTION('ref_axis',(0.,0.,1.)) ;
#105898=DIRECTION('',(0.,0.,-1.)) ;
#105899=DIRECTION('',(0.664363838829919,-0.74740931868366,0.)) ;
#105900=DIRECTION('',(0.655772517804503,-0.737744082530068,0.160299948796656)) ;
#105901=DIRECTION('',(0.,0.,1.)) ;
#105902=DIRECTION('',(-0.655772517804503,0.737744082530068,0.160299948796656)) ;
#105903=DIRECTION('',(-0.664363838829919,0.74740931868366,0.)) ;
#105904=DIRECTION('center_axis',(1.,0.,4.33680868994202E-16)) ;
#105905=DIRECTION('ref_axis',(4.33680868994202E-16,0.,-1.)) ;
#105906=DIRECTION('',(0.,1.,0.)) ;
#105907=DIRECTION('',(4.33680868994202E-16,0.,-1.)) ;
#105908=DIRECTION('',(0.,-1.,0.)) ;
#105909=DIRECTION('',(-4.33680868994202E-16,0.,1.)) ;
#105910=DIRECTION('center_axis',(-1.73472347597681E-16,0.,-1.)) ;
#105911=DIRECTION('ref_axis',(-1.,0.,1.73472347597681E-16)) ;
#105912=DIRECTION('',(-1.,0.,1.73472347597681E-16)) ;
#105913=DIRECTION('',(0.,-1.,0.)) ;
#105914=DIRECTION('',(1.,0.,-1.73472347597681E-16)) ;
#105915=DIRECTION('',(0.,1.,0.)) ;
#105916=DIRECTION('center_axis',(-1.,0.,0.)) ;
#105917=DIRECTION('ref_axis',(0.,0.,1.)) ;
#105918=DIRECTION('',(0.,0.,1.)) ;
#105919=DIRECTION('',(0.,-1.,0.)) ;
#105920=DIRECTION('',(0.,0.,-1.)) ;
#105921=DIRECTION('',(0.,1.,0.)) ;
#105922=DIRECTION('center_axis',(-1.73472347597681E-16,0.,1.)) ;
#105923=DIRECTION('ref_axis',(1.,0.,1.73472347597681E-16)) ;
#105924=DIRECTION('',(0.,1.,0.)) ;
#105925=DIRECTION('',(1.,0.,1.73472347597681E-16)) ;
#105926=DIRECTION('',(0.,-1.,0.)) ;
#105927=DIRECTION('',(-1.,0.,-1.73472347597681E-16)) ;
#105928=DIRECTION('center_axis',(0.,-1.,0.)) ;
#105929=DIRECTION('ref_axis',(0.,0.,-1.)) ;
#105930=DIRECTION('',(-1.,0.,-1.73472347597681E-16)) ;
#105931=DIRECTION('',(0.,0.,-1.)) ;
#105932=DIRECTION('',(1.,0.,-1.73472347597681E-16)) ;
#105933=DIRECTION('',(-4.33680868994202E-16,0.,1.)) ;
#105934=DIRECTION('',(1.,0.,0.)) ;
#105935=DIRECTION('center_axis',(0.,-1.,0.)) ;
#105936=DIRECTION('ref_axis',(0.,0.,-1.)) ;
#105937=DIRECTION('',(0.,0.,-1.)) ;
#105938=DIRECTION('center_axis',(0.,-1.,0.)) ;
#105939=DIRECTION('ref_axis',(0.,0.,-1.)) ;
#105940=DIRECTION('',(-1.,0.,0.)) ;
#105941=DIRECTION('center_axis',(0.,-1.,0.)) ;
#105942=DIRECTION('ref_axis',(0.,0.,1.)) ;
#105943=DIRECTION('',(0.,0.,1.)) ;
#105944=DIRECTION('center_axis',(0.,-1.,0.)) ;
#105945=DIRECTION('ref_axis',(0.,0.,-1.)) ;
#105946=DIRECTION('center_axis',(0.,-1.,0.)) ;
#105947=DIRECTION('ref_axis',(0.,0.,-1.)) ;
#105948=DIRECTION('center_axis',(0.,-1.,0.)) ;
#105949=DIRECTION('ref_axis',(0.,0.,-1.)) ;
#105950=DIRECTION('',(0.,-1.,0.)) ;
#105951=DIRECTION('',(0.,-1.,0.)) ;
#105952=DIRECTION('center_axis',(0.,0.,-1.)) ;
#105953=DIRECTION('ref_axis',(-1.,0.,0.)) ;
#105954=DIRECTION('',(1.,0.,0.)) ;
#105955=DIRECTION('',(0.,-1.,0.)) ;
#105956=DIRECTION('center_axis',(0.,-1.,0.)) ;
#105957=DIRECTION('ref_axis',(0.,0.,-1.)) ;
#105958=DIRECTION('center_axis',(0.,-1.,0.)) ;
#105959=DIRECTION('ref_axis',(0.,0.,-1.)) ;
#105960=DIRECTION('',(0.,-1.,0.)) ;
#105961=DIRECTION('center_axis',(-1.,0.,0.)) ;
#105962=DIRECTION('ref_axis',(0.,0.,1.)) ;
#105963=DIRECTION('',(0.,0.,-1.)) ;
#105964=DIRECTION('',(0.,-1.,0.)) ;
#105965=DIRECTION('center_axis',(0.,-1.,0.)) ;
#105966=DIRECTION('ref_axis',(0.,0.,-1.)) ;
#105967=DIRECTION('center_axis',(0.,-1.,0.)) ;
#105968=DIRECTION('ref_axis',(0.,0.,-1.)) ;
#105969=DIRECTION('',(0.,-1.,0.)) ;
#105970=DIRECTION('center_axis',(0.,0.,1.)) ;
#105971=DIRECTION('ref_axis',(1.,0.,0.)) ;
#105972=DIRECTION('',(-1.,0.,0.)) ;
#105973=DIRECTION('',(0.,-1.,0.)) ;
#105974=DIRECTION('center_axis',(0.,-1.,0.)) ;
#105975=DIRECTION('ref_axis',(0.,0.,-1.)) ;
#105976=DIRECTION('center_axis',(0.,-1.,0.)) ;
#105977=DIRECTION('ref_axis',(0.,0.,1.)) ;
#105978=DIRECTION('',(0.,-1.,0.)) ;
#105979=DIRECTION('center_axis',(1.,0.,0.)) ;
#105980=DIRECTION('ref_axis',(0.,0.,-1.)) ;
#105981=DIRECTION('',(0.,0.,1.)) ;
#105982=DIRECTION('center_axis',(0.,-1.,0.)) ;
#105983=DIRECTION('ref_axis',(0.,0.,-1.)) ;
#105984=DIRECTION('center_axis',(0.,1.,0.)) ;
#105985=DIRECTION('ref_axis',(0.,0.,1.)) ;
#105986=DIRECTION('',(-0.422618261740697,0.,0.906307787036651)) ;
#105987=DIRECTION('center_axis',(0.906307787036651,0.,0.422618261740697)) ;
#105988=DIRECTION('ref_axis',(0.422618261740697,0.,-0.906307787036651)) ;
#105989=DIRECTION('',(-0.422618261740697,0.,0.906307787036651)) ;
#105990=DIRECTION('',(0.422618261740697,0.,-0.906307787036651)) ;
#105991=DIRECTION('center_axis',(-0.906307787036651,0.,-0.422618261740697)) ;
#105992=DIRECTION('ref_axis',(-0.422618261740697,0.,0.906307787036651)) ;
#105993=DIRECTION('',(0.422618261740697,0.,-0.906307787036651)) ;
#105994=DIRECTION('',(-0.422618261740697,0.,0.906307787036651)) ;
#105995=DIRECTION('center_axis',(0.,1.,0.)) ;
#105996=DIRECTION('ref_axis',(0.,0.,1.)) ;
#105997=DIRECTION('',(-0.422618261740697,0.,0.906307787036651)) ;
#105998=DIRECTION('',(0.422618261740697,0.,-0.906307787036651)) ;
#105999=DIRECTION('center_axis',(1.,0.,-2.16840434497101E-16)) ;
#106000=DIRECTION('ref_axis',(-2.16840434497101E-16,0.,-1.)) ;
#106001=DIRECTION('',(2.16840434497101E-16,0.,1.)) ;
#106002=DIRECTION('',(0.,1.,0.)) ;
#106003=DIRECTION('',(-2.16840434497101E-16,0.,-1.)) ;
#106004=DIRECTION('',(0.,-1.,0.)) ;
#106005=DIRECTION('center_axis',(1.73472347597681E-16,0.,1.)) ;
#106006=DIRECTION('ref_axis',(1.,0.,-1.73472347597681E-16)) ;
#106007=DIRECTION('',(0.,-1.,0.)) ;
#106008=DIRECTION('',(-1.,0.,1.73472347597681E-16)) ;
#106009=DIRECTION('',(0.,1.,0.)) ;
#106010=DIRECTION('',(1.,0.,-1.73472347597681E-16)) ;
#106011=DIRECTION('center_axis',(-1.,0.,2.16840434497101E-16)) ;
#106012=DIRECTION('ref_axis',(2.16840434497101E-16,0.,1.)) ;
#106013=DIRECTION('',(0.,-1.,0.)) ;
#106014=DIRECTION('',(-2.16840434497101E-16,0.,-1.)) ;
#106015=DIRECTION('',(0.,1.,0.)) ;
#106016=DIRECTION('',(2.16840434497101E-16,0.,1.)) ;
#106017=DIRECTION('center_axis',(-1.73472347597681E-16,0.,-1.)) ;
#106018=DIRECTION('ref_axis',(-1.,0.,1.73472347597681E-16)) ;
#106019=DIRECTION('',(1.,0.,-1.73472347597681E-16)) ;
#106020=DIRECTION('',(0.,1.,0.)) ;
#106021=DIRECTION('',(-1.,0.,1.73472347597681E-16)) ;
#106022=DIRECTION('',(0.,-1.,0.)) ;
#106023=DIRECTION('center_axis',(0.,1.,0.)) ;
#106024=DIRECTION('ref_axis',(0.,0.,1.)) ;
#106025=DIRECTION('',(1.,0.,-1.73472347597681E-16)) ;
#106026=DIRECTION('',(-2.16840434497101E-16,0.,-1.)) ;
#106027=DIRECTION('',(-1.,0.,1.73472347597681E-16)) ;
#106028=DIRECTION('',(2.16840434497101E-16,0.,1.)) ;
#106029=DIRECTION('',(1.,0.,0.)) ;
#106030=DIRECTION('center_axis',(0.,1.,0.)) ;
#106031=DIRECTION('ref_axis',(0.,0.,1.)) ;
#106032=DIRECTION('',(0.,0.,1.)) ;
#106033=DIRECTION('center_axis',(0.,1.,0.)) ;
#106034=DIRECTION('ref_axis',(0.,0.,1.)) ;
#106035=DIRECTION('',(-1.,0.,0.)) ;
#106036=DIRECTION('center_axis',(0.,1.,0.)) ;
#106037=DIRECTION('ref_axis',(0.,0.,-1.)) ;
#106038=DIRECTION('',(0.,0.,-1.)) ;
#106039=DIRECTION('center_axis',(0.,1.,0.)) ;
#106040=DIRECTION('ref_axis',(0.,0.,1.)) ;
#106041=DIRECTION('center_axis',(0.,1.,0.)) ;
#106042=DIRECTION('ref_axis',(0.,0.,1.)) ;
#106043=DIRECTION('',(0.,1.,0.)) ;
#106044=DIRECTION('center_axis',(0.,-1.,0.)) ;
#106045=DIRECTION('ref_axis',(2.60208521396523E-14,0.,1.)) ;
#106046=DIRECTION('',(0.,1.,0.)) ;
#106047=DIRECTION('center_axis',(0.,0.,1.)) ;
#106048=DIRECTION('ref_axis',(1.,0.,0.)) ;
#106049=DIRECTION('',(-1.,0.,0.)) ;
#106050=DIRECTION('',(0.,1.,0.)) ;
#106051=DIRECTION('center_axis',(0.,1.,0.)) ;
#106052=DIRECTION('ref_axis',(0.,0.,1.)) ;
#106053=DIRECTION('center_axis',(0.,-1.,0.)) ;
#106054=DIRECTION('ref_axis',(0.,0.,1.)) ;
#106055=DIRECTION('',(0.,1.,0.)) ;
#106056=DIRECTION('center_axis',(-1.,0.,0.)) ;
#106057=DIRECTION('ref_axis',(0.,0.,1.)) ;
#106058=DIRECTION('',(0.,0.,-1.)) ;
#106059=DIRECTION('',(0.,1.,0.)) ;
#106060=DIRECTION('center_axis',(0.,1.,0.)) ;
#106061=DIRECTION('ref_axis',(0.,0.,1.)) ;
#106062=DIRECTION('center_axis',(0.,-1.,0.)) ;
#106063=DIRECTION('ref_axis',(0.,0.,1.)) ;
#106064=DIRECTION('',(0.,1.,0.)) ;
#106065=DIRECTION('center_axis',(0.,0.,-1.)) ;
#106066=DIRECTION('ref_axis',(-1.,0.,0.)) ;
#106067=DIRECTION('',(1.,0.,0.)) ;
#106068=DIRECTION('',(0.,1.,0.)) ;
#106069=DIRECTION('center_axis',(0.,1.,0.)) ;
#106070=DIRECTION('ref_axis',(0.,0.,1.)) ;
#106071=DIRECTION('center_axis',(0.,-1.,0.)) ;
#106072=DIRECTION('ref_axis',(0.,0.,1.)) ;
#106073=DIRECTION('',(0.,1.,0.)) ;
#106074=DIRECTION('center_axis',(1.,0.,0.)) ;
#106075=DIRECTION('ref_axis',(0.,0.,-1.)) ;
#106076=DIRECTION('',(0.,0.,1.)) ;
#106077=DIRECTION('center_axis',(0.,1.,0.)) ;
#106078=DIRECTION('ref_axis',(0.,0.,1.)) ;
#106079=DIRECTION('',(1.,0.,0.)) ;
#106080=DIRECTION('',(0.,0.,-1.)) ;
#106081=DIRECTION('',(-1.,0.,0.)) ;
#106082=DIRECTION('',(0.,0.,1.)) ;
#106083=DIRECTION('center_axis',(0.,0.164398987305357,-0.986393923832144)) ;
#106084=DIRECTION('ref_axis',(0.,0.986393923832144,0.164398987305357)) ;
#106085=DIRECTION('',(-1.,-1.0450141421547E-16,-1.7416902369245E-17)) ;
#106086=DIRECTION('',(0.,-0.986393923832144,-0.164398987305357)) ;
#106087=DIRECTION('',(1.,0.,0.)) ;
#106088=DIRECTION('',(0.,0.986393923832144,0.164398987305357)) ;
#106089=DIRECTION('center_axis',(0.,-1.,0.)) ;
#106090=DIRECTION('ref_axis',(0.,0.,-1.)) ;
#106091=DIRECTION('',(0.,0.,1.)) ;
#106092=DIRECTION('',(0.,0.,-1.)) ;
#106093=DIRECTION('',(-1.,0.,0.)) ;
#106094=DIRECTION('center_axis',(0.,0.164398987305357,0.986393923832144)) ;
#106095=DIRECTION('ref_axis',(0.,-0.986393923832144,0.164398987305357)) ;
#106096=DIRECTION('',(0.,0.986393923832144,-0.164398987305357)) ;
#106097=DIRECTION('',(1.,1.0450141421547E-16,-1.7416902369245E-17)) ;
#106098=DIRECTION('',(0.,-0.986393923832144,0.164398987305357)) ;
#106099=DIRECTION('center_axis',(-1.,0.,0.)) ;
#106100=DIRECTION('ref_axis',(0.,0.,1.)) ;
#106101=DIRECTION('',(0.,0.,1.)) ;
#106102=DIRECTION('center_axis',(-1.,0.,0.)) ;
#106103=DIRECTION('ref_axis',(0.,0.,1.)) ;
#106104=DIRECTION('',(0.,-0.986393923832144,0.164398987305357)) ;
#106105=DIRECTION('',(0.,0.,-1.)) ;
#106106=DIRECTION('',(0.,0.986393923832144,0.164398987305357)) ;
#106107=DIRECTION('center_axis',(1.,0.,0.)) ;
#106108=DIRECTION('ref_axis',(0.,0.,-1.)) ;
#106109=DIRECTION('center_axis',(1.,0.,0.)) ;
#106110=DIRECTION('ref_axis',(0.,0.,-1.)) ;
#106111=DIRECTION('center_axis',(1.,0.,0.)) ;
#106112=DIRECTION('ref_axis',(0.,0.,1.)) ;
#106113=DIRECTION('center_axis',(1.,0.,0.)) ;
#106114=DIRECTION('ref_axis',(0.,1.77635683940025E-15,1.)) ;
#106115=DIRECTION('center_axis',(1.,0.,0.)) ;
#106116=DIRECTION('ref_axis',(0.,-3.5527136788005E-15,1.)) ;
#106117=DIRECTION('',(1.,0.,0.)) ;
#106118=DIRECTION('center_axis',(-1.,0.,0.)) ;
#106119=DIRECTION('ref_axis',(0.,0.,1.)) ;
#106120=DIRECTION('',(-1.,0.,0.)) ;
#106121=DIRECTION('center_axis',(0.,0.,-1.)) ;
#106122=DIRECTION('ref_axis',(1.,0.,0.)) ;
#106123=DIRECTION('center_axis',(0.,-1.,0.)) ;
#106124=DIRECTION('ref_axis',(0.,0.,1.)) ;
#106125=DIRECTION('center_axis',(0.971399006496778,0.,-0.23745309047699)) ;
#106126=DIRECTION('ref_axis',(-0.23745309047699,0.,-0.971399006496778)) ;
#106127=DIRECTION('center_axis',(0.971399006496778,0.,-0.237453090476989)) ;
#106128=DIRECTION('ref_axis',(-0.237453090476989,0.,-0.971399006496778)) ;
#106129=DIRECTION('center_axis',(0.655772517804501,-0.73774408253007,-0.160299948796655)) ;
#106130=DIRECTION('ref_axis',(-0.747409318683663,-0.664363838829916,-3.82464933042368E-16)) ;
#106131=DIRECTION('center_axis',(-0.439210132175037,-4.69342344346061E-10,
-0.898384360836044)) ;
#106132=DIRECTION('ref_axis',(0.882040291646593,-0.189880214231443,-0.43121969824605)) ;
#106133=DIRECTION('center_axis',(0.655772517804504,-0.737744082530068,-0.160299948796656)) ;
#106134=DIRECTION('ref_axis',(0.74740931868366,0.664363838829919,-2.08334010827303E-16)) ;
#106135=DIRECTION('center_axis',(0.655772517804505,-0.737744082530068,-0.16029994879665)) ;
#106136=DIRECTION('ref_axis',(0.74740931868366,0.66436383882992,-5.75609428574487E-16)) ;
#106137=DIRECTION('center_axis',(0.664363838829919,-0.74740931868366,0.)) ;
#106138=DIRECTION('ref_axis',(0.74740931868366,0.664363838829919,0.)) ;
#106139=DIRECTION('center_axis',(-0.664363838829918,0.747409318683661,0.)) ;
#106140=DIRECTION('ref_axis',(-0.747409318683661,-0.664363838829918,0.)) ;
#106141=DIRECTION('center_axis',(0.,1.,0.)) ;
#106142=DIRECTION('ref_axis',(0.,0.,1.)) ;
#106143=DIRECTION('center_axis',(0.,-1.,0.)) ;
#106144=DIRECTION('ref_axis',(0.,0.,-1.)) ;
#106145=DIRECTION('center_axis',(0.,0.,1.)) ;
#106146=DIRECTION('ref_axis',(1.,0.,0.)) ;
#106147=DIRECTION('center_axis',(0.,0.,-1.)) ;
#106148=DIRECTION('ref_axis',(-1.,0.,0.)) ;
#106149=DIRECTION('center_axis',(0.,0.,-1.)) ;
#106150=DIRECTION('ref_axis',(-1.,0.,0.)) ;
#106151=DIRECTION('center_axis',(0.439210132174959,4.69119130465546E-10,
-0.898384360836082)) ;
#106152=DIRECTION('ref_axis',(0.882040291646776,-0.189880214230495,0.431219698246092)) ;
#106153=DIRECTION('center_axis',(-0.971399006496778,0.,-0.23745309047699)) ;
#106154=DIRECTION('ref_axis',(-0.23745309047699,0.,0.971399006496778)) ;
#106155=DIRECTION('center_axis',(0.971399006496778,0.,0.237453090476989)) ;
#106156=DIRECTION('ref_axis',(0.237453090476989,0.,-0.971399006496778)) ;
#106157=DIRECTION('center_axis',(0.,1.,0.)) ;
#106158=DIRECTION('ref_axis',(1.,0.,0.)) ;
#106159=DIRECTION('center_axis',(-3.54829801904343E-14,1.,8.67361737988405E-15)) ;
#106160=DIRECTION('ref_axis',(1.,3.54829801904343E-14,6.83923985932746E-30)) ;
#106161=DIRECTION('center_axis',(-0.948683298050516,0.316227766016833,4.68041587613745E-15)) ;
#106162=DIRECTION('ref_axis',(0.316227766016833,0.948683298050516,-2.29441790171558E-12)) ;
#106163=DIRECTION('center_axis',(0.,0.,-1.)) ;
#106164=DIRECTION('ref_axis',(1.,0.,0.)) ;
#106165=DIRECTION('center_axis',(0.,-1.,0.)) ;
#106166=DIRECTION('ref_axis',(0.,0.,1.)) ;
#106167=DIRECTION('center_axis',(0.655772517804503,-0.737744082530069,0.160299948796655)) ;
#106168=DIRECTION('ref_axis',(-0.747409318683661,-0.664363838829918,2.39955779178099E-16)) ;
#106169=DIRECTION('center_axis',(0.,1.,0.)) ;
#106170=DIRECTION('ref_axis',(0.,0.,1.)) ;
#106171=DIRECTION('center_axis',(2.73957817177508E-14,1.,0.)) ;
#106172=DIRECTION('ref_axis',(-1.,2.73957817177508E-14,0.)) ;
#106173=DIRECTION('center_axis',(0.894427190999917,0.447213595499956,0.)) ;
#106174=DIRECTION('ref_axis',(-0.447213595499956,0.894427190999917,0.)) ;
#106175=DIRECTION('center_axis',(-0.894427190999916,-0.447213595499958,
0.)) ;
#106176=DIRECTION('ref_axis',(0.447213595499958,-0.894427190999916,0.)) ;
#106177=DIRECTION('center_axis',(0.,0.,1.)) ;
#106178=DIRECTION('ref_axis',(1.,0.,0.)) ;
#106179=DIRECTION('center_axis',(0.,0.,-1.)) ;
#106180=DIRECTION('ref_axis',(-1.,0.,0.)) ;
#106181=DIRECTION('center_axis',(0.,1.,0.)) ;
#106182=DIRECTION('ref_axis',(0.,0.,1.)) ;
#106183=DIRECTION('center_axis',(0.,-1.,0.)) ;
#106184=DIRECTION('ref_axis',(0.,0.,-1.)) ;
#106185=DIRECTION('center_axis',(-0.664363838829919,0.74740931868366,0.)) ;
#106186=DIRECTION('ref_axis',(-0.74740931868366,-0.664363838829919,0.)) ;
#106187=DIRECTION('center_axis',(-0.66436383882992,0.747409318683659,2.52106651083074E-15)) ;
#106188=DIRECTION('ref_axis',(-0.747409318683659,-0.66436383882992,7.82575143531171E-30)) ;
#106189=DIRECTION('center_axis',(-0.655772517804504,0.737744082530068,-0.160299948796656)) ;
#106190=DIRECTION('ref_axis',(-0.74740931868366,-0.664363838829919,2.31673158493852E-16)) ;
#106191=DIRECTION('center_axis',(0.655772517804496,-0.737744082530075,0.160299948796656)) ;
#106192=DIRECTION('ref_axis',(0.747409318683667,0.664363838829911,-2.10122272487167E-17)) ;
#106193=DIRECTION('center_axis',(0.,1.,0.)) ;
#106194=DIRECTION('ref_axis',(1.,0.,0.)) ;
#106195=DIRECTION('center_axis',(-0.873786407766988,-0.436893203883498,
0.213592233009711)) ;
#106196=DIRECTION('ref_axis',(-0.447213595499961,0.894427190999914,3.0060297474479E-16)) ;
#106197=DIRECTION('center_axis',(-0.948683298050516,0.316227766016832,-3.84691715846994E-15)) ;
#106198=DIRECTION('ref_axis',(0.316227766016832,0.948683298050516,-1.68048965429074E-12)) ;
#106199=DIRECTION('center_axis',(0.,1.,0.)) ;
#106200=DIRECTION('ref_axis',(1.,0.,0.)) ;
#106201=DIRECTION('center_axis',(-5.47915634355017E-14,1.,0.)) ;
#106202=DIRECTION('ref_axis',(1.,5.47915634355017E-14,6.93889390390721E-14)) ;
#106203=DIRECTION('center_axis',(-0.971399006496778,0.,0.23745309047699)) ;
#106204=DIRECTION('ref_axis',(0.23745309047699,0.,0.971399006496778)) ;
#106205=DIRECTION('center_axis',(0.971399006496778,-3.69787733965917E-15,
-0.237453090476989)) ;
#106206=DIRECTION('ref_axis',(-0.237453090476989,1.87410005036359E-29,-0.971399006496778)) ;
#106207=DIRECTION('center_axis',(0.873786407766991,0.436893203883493,-0.213592233009709)) ;
#106208=DIRECTION('ref_axis',(-0.447213595499956,0.894427190999917,2.83414331365695E-16)) ;
#106209=DIRECTION('center_axis',(-0.873786407766992,-0.436893203883492,
0.21359223300971)) ;
#106210=DIRECTION('ref_axis',(0.447213595499955,-0.894427190999918,-1.48231119036019E-16)) ;
#106211=DIRECTION('center_axis',(-0.894427190999917,-0.447213595499956,
0.)) ;
#106212=DIRECTION('ref_axis',(0.447213595499956,-0.894427190999917,0.)) ;
#106213=DIRECTION('center_axis',(-0.894427190999917,-0.447213595499955,
0.)) ;
#106214=DIRECTION('ref_axis',(0.447213595499955,-0.894427190999917,0.)) ;
#106215=DIRECTION('center_axis',(0.,1.,0.)) ;
#106216=DIRECTION('ref_axis',(0.,0.,1.)) ;
#106217=DIRECTION('center_axis',(2.66122351428257E-14,1.,6.50521303491301E-15)) ;
#106218=DIRECTION('ref_axis',(-1.,2.66122351428257E-14,3.84707242087163E-30)) ;
#106219=DIRECTION('center_axis',(-0.439210132005065,2.74999532687384E-13,
-0.898384360919141)) ;
#106220=DIRECTION('ref_axis',(0.898384360919141,-1.32695180921442E-11,-0.439210132005065)) ;
#106221=DIRECTION('center_axis',(0.,1.,0.)) ;
#106222=DIRECTION('ref_axis',(1.,0.,0.)) ;
#106223=DIRECTION('center_axis',(-0.87378640776699,-0.436893203883495,-0.213592233009712)) ;
#106224=DIRECTION('ref_axis',(-0.447213595499958,0.894427190999916,-1.950883489007E-18)) ;
#106225=DIRECTION('center_axis',(0.,0.,1.)) ;
#106226=DIRECTION('ref_axis',(1.,0.,0.)) ;
#106227=DIRECTION('center_axis',(0.4392101320051,-6.47579544715494E-13,
-0.898384360919124)) ;
#106228=DIRECTION('ref_axis',(0.898384360919124,-3.722424582079E-12,0.4392101320051)) ;
#106229=DIRECTION('center_axis',(-0.873786407766991,-0.436893203883493,
-0.213592233009709)) ;
#106230=DIRECTION('ref_axis',(0.447213595499956,-0.894427190999917,-1.06780556900622E-16)) ;
#106231=DIRECTION('center_axis',(-0.873786407766992,-0.436893203883492,
-0.213592233009707)) ;
#106232=DIRECTION('ref_axis',(0.447213595499955,-0.894427190999918,-7.04543255365314E-18)) ;
#106233=DIRECTION('center_axis',(-0.971399006496778,0.,-0.237453090476989)) ;
#106234=DIRECTION('ref_axis',(0.237453090476989,0.,-0.971399006496778)) ;
#106235=DIRECTION('center_axis',(0.971399006496778,0.,0.23745309047699)) ;
#106236=DIRECTION('ref_axis',(0.23745309047699,0.,-0.971399006496778)) ;
#106237=DIRECTION('center_axis',(0.,0.,-1.)) ;
#106238=DIRECTION('ref_axis',(-1.,0.,0.)) ;
#106239=DIRECTION('center_axis',(1.,1.0450141421547E-16,1.7416902369245E-17)) ;
#106240=DIRECTION('ref_axis',(-1.0450141421547E-16,1.,-1.82009092883888E-33)) ;
#106241=DIRECTION('center_axis',(0.672672795323067,0.739940072189803,-7.49424791604764E-10)) ;
#106242=DIRECTION('ref_axis',(0.738044870610434,-0.670949884717718,0.0715263669069537)) ;
#106243=DIRECTION('center_axis',(-1.,0.,0.)) ;
#106244=DIRECTION('ref_axis',(0.,-0.646374896130193,-0.763019982472728)) ;
#106245=DIRECTION('center_axis',(-1.,0.,0.)) ;
#106246=DIRECTION('ref_axis',(0.,0.,1.)) ;
#106247=DIRECTION('center_axis',(-1.,0.,0.)) ;
#106248=DIRECTION('ref_axis',(0.,0.,1.)) ;
#106249=DIRECTION('center_axis',(0.,0.986393923832144,0.164398987305357)) ;
#106250=DIRECTION('ref_axis',(0.,-0.164398987305357,0.986393923832144)) ;
#106251=DIRECTION('center_axis',(0.,-0.986393923832144,-0.164398987305358)) ;
#106252=DIRECTION('ref_axis',(0.,0.164398987305358,-0.986393923832144)) ;
#106253=DIRECTION('center_axis',(0.,0.,1.)) ;
#106254=DIRECTION('ref_axis',(1.,0.,0.)) ;
#106255=DIRECTION('center_axis',(0.,0.,1.)) ;
#106256=DIRECTION('ref_axis',(1.,0.,0.)) ;
#106257=DIRECTION('center_axis',(0.,0.,1.)) ;
#106258=DIRECTION('ref_axis',(1.,0.,0.)) ;
#106259=DIRECTION('center_axis',(0.,0.,-1.)) ;
#106260=DIRECTION('ref_axis',(1.,0.,0.)) ;
#106261=DIRECTION('center_axis',(-1.,0.,0.)) ;
#106262=DIRECTION('ref_axis',(0.,-0.646374896130191,-0.76301998247273)) ;
#106263=DIRECTION('center_axis',(0.,0.,1.)) ;
#106264=DIRECTION('ref_axis',(-1.,0.,0.)) ;
#106265=DIRECTION('center_axis',(0.,0.,-1.)) ;
#106266=DIRECTION('ref_axis',(-1.,0.,0.)) ;
#106267=DIRECTION('center_axis',(1.,1.0450141421547E-16,-1.7416902369245E-17)) ;
#106268=DIRECTION('ref_axis',(-1.0450141421547E-16,1.,1.82009092883888E-33)) ;
#106269=DIRECTION('center_axis',(0.672672795322483,0.739940072190334,7.49091207824656E-10)) ;
#106270=DIRECTION('ref_axis',(0.738044870606418,-0.670949884713036,-0.0715263669923128)) ;
#106271=DIRECTION('center_axis',(1.,0.,0.)) ;
#106272=DIRECTION('ref_axis',(0.,4.77048955893625E-14,1.)) ;
#106273=DIRECTION('center_axis',(0.,0.,-1.)) ;
#106274=DIRECTION('ref_axis',(-1.,0.,0.)) ;
#106275=DIRECTION('center_axis',(0.,-0.986393923832144,0.164398987305357)) ;
#106276=DIRECTION('ref_axis',(0.,-0.164398987305357,-0.986393923832144)) ;
#106277=DIRECTION('center_axis',(1.,0.,0.)) ;
#106278=DIRECTION('ref_axis',(0.,0.,1.)) ;
#106279=DIRECTION('center_axis',(7.58941520739854E-15,0.,-1.)) ;
#106280=DIRECTION('ref_axis',(-1.,0.,-7.58941520739854E-15)) ;
#106281=DIRECTION('center_axis',(1.,0.,-8.67361737988404E-15)) ;
#106282=DIRECTION('ref_axis',(-8.67361737988404E-15,0.,-1.)) ;
#106283=DIRECTION('center_axis',(1.,0.,0.)) ;
#106284=DIRECTION('ref_axis',(0.,0.,-1.)) ;
#106285=DIRECTION('center_axis',(1.,0.,8.67361737988403E-15)) ;
#106286=DIRECTION('ref_axis',(8.67361737988403E-15,0.,-1.)) ;
#106287=DIRECTION('center_axis',(0.,0.,1.)) ;
#106288=DIRECTION('ref_axis',(1.,0.,0.)) ;
#106289=DIRECTION('center_axis',(0.,0.,-1.)) ;
#106290=DIRECTION('ref_axis',(-1.,0.,0.)) ;
#106291=DIRECTION('center_axis',(1.,0.,0.)) ;
#106292=DIRECTION('ref_axis',(0.,0.,1.)) ;
#106293=DIRECTION('center_axis',(-6.50521303491304E-15,0.,-1.)) ;
#106294=DIRECTION('ref_axis',(-1.,0.,6.50521303491304E-15)) ;
#106295=DIRECTION('center_axis',(1.,0.,0.)) ;
#106296=DIRECTION('ref_axis',(0.,0.,1.)) ;
#106297=DIRECTION('center_axis',(1.,9.40395480657835E-30,8.67361737988403E-15)) ;
#106298=DIRECTION('ref_axis',(8.67361737988403E-15,-5.27711695562625E-58,
-1.)) ;
#106299=DIRECTION('center_axis',(0.,0.,-1.)) ;
#106300=DIRECTION('ref_axis',(-1.,0.,0.)) ;
#106301=DIRECTION('center_axis',(6.50521303491304E-15,0.,-1.)) ;
#106302=DIRECTION('ref_axis',(-1.,0.,-6.50521303491304E-15)) ;
#106303=DIRECTION('center_axis',(-1.,0.,0.)) ;
#106304=DIRECTION('ref_axis',(0.,0.,1.)) ;
#106305=DIRECTION('center_axis',(1.,-8.67361737988409E-15,0.)) ;
#106306=DIRECTION('ref_axis',(8.67361737988409E-15,1.,0.)) ;
#106307=DIRECTION('center_axis',(1.,0.,0.)) ;
#106308=DIRECTION('ref_axis',(0.,0.,1.)) ;
#106309=DIRECTION('center_axis',(-4.33680868994202E-16,0.,1.)) ;
#106310=DIRECTION('ref_axis',(1.,0.,4.33680868994202E-16)) ;
#106311=DIRECTION('center_axis',(0.,0.,-1.)) ;
#106312=DIRECTION('ref_axis',(-1.,0.,0.)) ;
#106313=DIRECTION('center_axis',(0.,0.,1.)) ;
#106314=DIRECTION('ref_axis',(1.,0.,0.)) ;
#106315=DIRECTION('center_axis',(0.,1.,0.)) ;
#106316=DIRECTION('ref_axis',(0.,0.,1.)) ;
#106317=DIRECTION('center_axis',(-1.,0.,0.)) ;
#106318=DIRECTION('ref_axis',(0.,0.,-1.)) ;
#106319=DIRECTION('center_axis',(0.,-1.,0.)) ;
#106320=DIRECTION('ref_axis',(0.,0.,1.)) ;
#106321=DIRECTION('center_axis',(0.,1.,0.)) ;
#106322=DIRECTION('ref_axis',(0.,0.,1.)) ;
#106323=DIRECTION('center_axis',(0.,-1.,0.)) ;
#106324=DIRECTION('ref_axis',(0.,0.,1.)) ;
#106325=DIRECTION('center_axis',(-1.,0.,0.)) ;
#106326=DIRECTION('ref_axis',(0.,0.,-1.)) ;
#106327=DIRECTION('center_axis',(-1.,0.,-1.73472347597681E-16)) ;
#106328=DIRECTION('ref_axis',(-1.73472347597681E-16,0.,1.)) ;
#106329=DIRECTION('center_axis',(-1.,0.,0.)) ;
#106330=DIRECTION('ref_axis',(0.,0.,1.)) ;
#106331=DIRECTION('center_axis',(0.,1.,0.)) ;
#106332=DIRECTION('ref_axis',(0.,0.,1.)) ;
#106333=DIRECTION('center_axis',(0.,-1.,0.)) ;
#106334=DIRECTION('ref_axis',(0.,0.,-1.)) ;
#106335=DIRECTION('center_axis',(-4.33680868994202E-16,0.,1.)) ;
#106336=DIRECTION('ref_axis',(1.,0.,4.33680868994202E-16)) ;
#106337=DIRECTION('center_axis',(0.,0.,1.)) ;
#106338=DIRECTION('ref_axis',(1.,0.,0.)) ;
#106339=DIRECTION('center_axis',(0.,0.,-1.)) ;
#106340=DIRECTION('ref_axis',(-1.,0.,0.)) ;
#106341=DIRECTION('center_axis',(0.,1.,0.)) ;
#106342=DIRECTION('ref_axis',(0.,0.,1.)) ;
#106343=DIRECTION('center_axis',(0.,-1.,0.)) ;
#106344=DIRECTION('ref_axis',(0.,0.,-1.)) ;
#106345=DIRECTION('center_axis',(1.,0.,-1.73472347597681E-16)) ;
#106346=DIRECTION('ref_axis',(-1.73472347597681E-16,0.,-1.)) ;
#106347=DIRECTION('center_axis',(-1.,0.,0.)) ;
#106348=DIRECTION('ref_axis',(0.,0.,1.)) ;
#106349=DIRECTION('center_axis',(0.,0.,-1.)) ;
#106350=DIRECTION('ref_axis',(-1.,0.,0.)) ;
#106351=DIRECTION('center_axis',(0.,0.,1.)) ;
#106352=DIRECTION('ref_axis',(1.,0.,0.)) ;
#106353=DIRECTION('center_axis',(0.,0.,-1.)) ;
#106354=DIRECTION('ref_axis',(-1.,0.,0.)) ;
#106355=DIRECTION('center_axis',(0.,1.,0.)) ;
#106356=DIRECTION('ref_axis',(0.,0.,1.)) ;
#106357=DIRECTION('center_axis',(0.,-1.,0.)) ;
#106358=DIRECTION('ref_axis',(0.,0.,1.)) ;
#106359=DIRECTION('center_axis',(0.,1.,0.)) ;
#106360=DIRECTION('ref_axis',(1.,0.,0.)) ;
#106361=DIRECTION('center_axis',(1.,0.,0.)) ;
#106362=DIRECTION('ref_axis',(0.,0.,1.)) ;
#106363=DIRECTION('center_axis',(0.,1.,0.)) ;
#106364=DIRECTION('ref_axis',(1.,0.,0.)) ;
#106365=DIRECTION('center_axis',(1.,0.,0.)) ;
#106366=DIRECTION('ref_axis',(0.,0.,1.)) ;
#106367=DIRECTION('center_axis',(0.,1.,0.)) ;
#106368=DIRECTION('ref_axis',(0.,0.,1.)) ;
#106369=DIRECTION('center_axis',(0.,-1.,0.)) ;
#106370=DIRECTION('ref_axis',(0.,0.,1.)) ;
#106371=DIRECTION('center_axis',(0.,1.,0.)) ;
#106372=DIRECTION('ref_axis',(0.,0.,1.)) ;
#106373=DIRECTION('center_axis',(0.,-1.,0.)) ;
#106374=DIRECTION('ref_axis',(0.,0.,-1.)) ;
#106375=DIRECTION('center_axis',(-1.,0.,-1.73472347597681E-16)) ;
#106376=DIRECTION('ref_axis',(-1.73472347597681E-16,0.,1.)) ;
#106377=DIRECTION('center_axis',(1.,0.,0.)) ;
#106378=DIRECTION('ref_axis',(0.,0.,-1.)) ;
#106379=DIRECTION('center_axis',(1.,0.,-1.73472347597681E-16)) ;
#106380=DIRECTION('ref_axis',(-1.73472347597681E-16,0.,-1.)) ;
#106381=DIRECTION('center_axis',(1.,0.,0.)) ;
#106382=DIRECTION('ref_axis',(0.,0.,-1.)) ;
#106383=DIRECTION('center_axis',(0.,1.,0.)) ;
#106384=DIRECTION('ref_axis',(0.,0.,1.)) ;
#106385=DIRECTION('center_axis',(0.,-1.,0.)) ;
#106386=DIRECTION('ref_axis',(0.,0.,-1.)) ;
#106387=DIRECTION('center_axis',(0.,1.,0.)) ;
#106388=DIRECTION('ref_axis',(1.,0.,0.)) ;
#106389=DIRECTION('center_axis',(0.,0.,1.)) ;
#106390=DIRECTION('ref_axis',(-1.,0.,0.)) ;
#106391=DIRECTION('center_axis',(0.,1.,0.)) ;
#106392=DIRECTION('ref_axis',(1.,0.,0.)) ;
#106393=DIRECTION('center_axis',(0.,0.,-1.)) ;
#106394=DIRECTION('ref_axis',(1.,0.,0.)) ;
#106395=DIRECTION('center_axis',(0.,0.,-1.)) ;
#106396=DIRECTION('ref_axis',(-1.,0.,0.)) ;
#106397=DIRECTION('center_axis',(2.16840434497101E-16,0.,1.)) ;
#106398=DIRECTION('ref_axis',(1.,0.,-2.16840434497101E-16)) ;
#106399=DIRECTION('center_axis',(0.,0.,-1.)) ;
#106400=DIRECTION('ref_axis',(-1.,0.,0.)) ;
#106401=DIRECTION('center_axis',(0.,0.,1.)) ;
#106402=DIRECTION('ref_axis',(1.,0.,0.)) ;
#106403=DIRECTION('center_axis',(0.,-1.,0.)) ;
#106404=DIRECTION('ref_axis',(0.,0.,-1.)) ;
#106405=DIRECTION('center_axis',(1.,0.,0.)) ;
#106406=DIRECTION('ref_axis',(0.,0.,1.)) ;
#106407=DIRECTION('center_axis',(0.,1.,0.)) ;
#106408=DIRECTION('ref_axis',(0.,0.,-1.)) ;
#106409=DIRECTION('center_axis',(0.,-1.,0.)) ;
#106410=DIRECTION('ref_axis',(0.,0.,-1.)) ;
#106411=DIRECTION('center_axis',(0.,1.,0.)) ;
#106412=DIRECTION('ref_axis',(0.,0.,-1.)) ;
#106413=DIRECTION('center_axis',(1.,0.,0.)) ;
#106414=DIRECTION('ref_axis',(0.,0.,1.)) ;
#106415=DIRECTION('center_axis',(1.,0.,-1.73472347597681E-16)) ;
#106416=DIRECTION('ref_axis',(-1.73472347597681E-16,0.,-1.)) ;
#106417=DIRECTION('center_axis',(1.,0.,0.)) ;
#106418=DIRECTION('ref_axis',(0.,0.,-1.)) ;
#106419=DIRECTION('center_axis',(0.,-1.,0.)) ;
#106420=DIRECTION('ref_axis',(0.,0.,-1.)) ;
#106421=DIRECTION('center_axis',(0.,1.,0.)) ;
#106422=DIRECTION('ref_axis',(0.,0.,1.)) ;
#106423=DIRECTION('center_axis',(2.16840434497101E-16,0.,1.)) ;
#106424=DIRECTION('ref_axis',(1.,0.,-2.16840434497101E-16)) ;
#106425=DIRECTION('center_axis',(0.,0.,1.)) ;
#106426=DIRECTION('ref_axis',(1.,0.,0.)) ;
#106427=DIRECTION('center_axis',(0.,0.,-1.)) ;
#106428=DIRECTION('ref_axis',(-1.,0.,0.)) ;
#106429=DIRECTION('center_axis',(0.,-1.,0.)) ;
#106430=DIRECTION('ref_axis',(0.,0.,-1.)) ;
#106431=DIRECTION('center_axis',(0.,1.,0.)) ;
#106432=DIRECTION('ref_axis',(0.,0.,1.)) ;
#106433=DIRECTION('center_axis',(-1.,0.,1.73472347597681E-16)) ;
#106434=DIRECTION('ref_axis',(1.73472347597681E-16,0.,1.)) ;
#106435=DIRECTION('center_axis',(1.,0.,0.)) ;
#106436=DIRECTION('ref_axis',(0.,0.,-1.)) ;
#106437=DIRECTION('center_axis',(-2.16840434497101E-16,0.,-1.)) ;
#106438=DIRECTION('ref_axis',(-1.,0.,2.16840434497101E-16)) ;
#106439=DIRECTION('center_axis',(0.,0.,1.)) ;
#106440=DIRECTION('ref_axis',(1.,0.,0.)) ;
#106441=DIRECTION('center_axis',(0.,0.,-1.)) ;
#106442=DIRECTION('ref_axis',(-1.,0.,0.)) ;
#106443=DIRECTION('center_axis',(0.,-1.,0.)) ;
#106444=DIRECTION('ref_axis',(0.,0.,-1.)) ;
#106445=DIRECTION('center_axis',(0.,1.,0.)) ;
#106446=DIRECTION('ref_axis',(0.,0.,-1.)) ;
#106447=DIRECTION('center_axis',(0.,1.,0.)) ;
#106448=DIRECTION('ref_axis',(1.,0.,0.)) ;
#106449=DIRECTION('center_axis',(-1.,0.,0.)) ;
#106450=DIRECTION('ref_axis',(0.,0.,-1.)) ;
#106451=DIRECTION('center_axis',(0.,1.,0.)) ;
#106452=DIRECTION('ref_axis',(1.,0.,0.)) ;
#106453=DIRECTION('center_axis',(-1.,0.,0.)) ;
#106454=DIRECTION('ref_axis',(0.,0.,-1.)) ;
#106455=DIRECTION('center_axis',(0.,-1.,0.)) ;
#106456=DIRECTION('ref_axis',(0.,0.,-1.)) ;
#106457=DIRECTION('center_axis',(0.,1.,0.)) ;
#106458=DIRECTION('ref_axis',(0.,0.,-1.)) ;
#106459=DIRECTION('center_axis',(0.,-1.,0.)) ;
#106460=DIRECTION('ref_axis',(0.,0.,-1.)) ;
#106461=DIRECTION('center_axis',(0.,1.,0.)) ;
#106462=DIRECTION('ref_axis',(0.,0.,1.)) ;
#106463=DIRECTION('center_axis',(1.,0.,-1.73472347597681E-16)) ;
#106464=DIRECTION('ref_axis',(-1.73472347597681E-16,0.,-1.)) ;
#106465=DIRECTION('center_axis',(-1.,0.,0.)) ;
#106466=DIRECTION('ref_axis',(0.,0.,1.)) ;
#106467=DIRECTION('center_axis',(-1.,0.,1.73472347597681E-16)) ;
#106468=DIRECTION('ref_axis',(1.73472347597681E-16,0.,1.)) ;
#106469=DIRECTION('center_axis',(-1.,0.,0.)) ;
#106470=DIRECTION('ref_axis',(0.,0.,1.)) ;
#106471=DIRECTION('center_axis',(0.,-1.,0.)) ;
#106472=DIRECTION('ref_axis',(0.,0.,-1.)) ;
#106473=DIRECTION('center_axis',(0.,1.,0.)) ;
#106474=DIRECTION('ref_axis',(0.,0.,1.)) ;
#106475=DIRECTION('center_axis',(0.,1.,0.)) ;
#106476=DIRECTION('ref_axis',(1.,0.,0.)) ;
#106477=DIRECTION('center_axis',(0.,0.,1.)) ;
#106478=DIRECTION('ref_axis',(-1.,0.,0.)) ;
#106479=DIRECTION('center_axis',(0.,1.,0.)) ;
#106480=DIRECTION('ref_axis',(1.,0.,0.)) ;
#106481=DIRECTION('center_axis',(0.,0.,-1.)) ;
#106482=DIRECTION('ref_axis',(1.,0.,0.)) ;
#106483=DIRECTION('center_axis',(-2.16840434497101E-16,0.,-1.)) ;
#106484=DIRECTION('ref_axis',(-1.,0.,2.16840434497101E-16)) ;
#106485=DIRECTION('center_axis',(-1.,0.,0.)) ;
#106486=DIRECTION('ref_axis',(0.,0.,1.)) ;
#106487=DIRECTION('center_axis',(0.,-0.632948931301575,-0.774193548387091)) ;
#106488=DIRECTION('ref_axis',(0.,0.774193548387091,-0.632948931301575)) ;
#106489=DIRECTION('center_axis',(0.,0.,1.)) ;
#106490=DIRECTION('ref_axis',(1.,0.,0.)) ;
#106491=DIRECTION('center_axis',(0.,8.67361737988405E-15,-1.)) ;
#106492=DIRECTION('ref_axis',(0.,1.,8.67361737988405E-15)) ;
#106493=DIRECTION('center_axis',(8.67361737988401E-15,0.,1.)) ;
#106494=DIRECTION('ref_axis',(1.,0.,-8.67361737988401E-15)) ;
#106495=DIRECTION('center_axis',(0.,1.,0.)) ;
#106496=DIRECTION('ref_axis',(1.,0.,0.)) ;
#106497=DIRECTION('center_axis',(-1.,0.,0.)) ;
#106498=DIRECTION('ref_axis',(0.,5.20417042793045E-14,-1.)) ;
#106499=DIRECTION('center_axis',(1.,0.,0.)) ;
#106500=DIRECTION('ref_axis',(0.,0.,-1.)) ;
#106501=DIRECTION('center_axis',(-1.,0.,0.)) ;
#106502=DIRECTION('ref_axis',(0.,0.,1.)) ;
#106503=DIRECTION('center_axis',(0.,0.,-1.)) ;
#106504=DIRECTION('ref_axis',(-1.,0.,0.)) ;
#106505=DIRECTION('center_axis',(0.,0.,1.)) ;
#106506=DIRECTION('ref_axis',(1.,0.,0.)) ;
#106507=DIRECTION('center_axis',(0.,0.,-1.)) ;
#106508=DIRECTION('ref_axis',(-1.,0.,0.)) ;
#106509=DIRECTION('center_axis',(-1.,0.,0.)) ;
#106510=DIRECTION('ref_axis',(0.,0.,1.)) ;
#106511=DIRECTION('center_axis',(0.,-0.632948931301567,-0.774193548387097)) ;
#106512=DIRECTION('ref_axis',(0.,-0.774193548387097,0.632948931301567)) ;
#106513=DIRECTION('center_axis',(-1.,0.,0.)) ;
#106514=DIRECTION('ref_axis',(0.,0.,1.)) ;
#106515=DIRECTION('center_axis',(0.,0.632948931301567,-0.774193548387097)) ;
#106516=DIRECTION('ref_axis',(0.,0.774193548387097,0.632948931301567)) ;
#106517=DIRECTION('center_axis',(0.,0.,-1.)) ;
#106518=DIRECTION('ref_axis',(-1.,0.,0.)) ;
#106519=DIRECTION('center_axis',(0.,0.,1.)) ;
#106520=DIRECTION('ref_axis',(1.,0.,0.)) ;
#106521=DIRECTION('center_axis',(-1.,0.,0.)) ;
#106522=DIRECTION('ref_axis',(0.,0.,1.)) ;
#106523=DIRECTION('center_axis',(1.,0.,0.)) ;
#106524=DIRECTION('ref_axis',(0.,5.20417042793045E-14,1.)) ;
#106525=DIRECTION('center_axis',(1.,0.,0.)) ;
#106526=DIRECTION('ref_axis',(0.,0.,-1.)) ;
#106527=DIRECTION('center_axis',(1.,0.,0.)) ;
#106528=DIRECTION('ref_axis',(0.,0.,-1.)) ;
#106529=DIRECTION('center_axis',(0.,0.,1.)) ;
#106530=DIRECTION('ref_axis',(1.,0.,0.)) ;
#106531=DIRECTION('center_axis',(0.,8.67361737988405E-15,-1.)) ;
#106532=DIRECTION('ref_axis',(0.,1.,8.67361737988405E-15)) ;
#106533=DIRECTION('center_axis',(0.,1.,0.)) ;
#106534=DIRECTION('ref_axis',(1.,0.,0.)) ;
#106535=DIRECTION('center_axis',(1.22050154678007E-14,0.632948931301567,
-0.774193548387097)) ;
#106536=DIRECTION('ref_axis',(1.73472347597684E-14,-0.774193548387097,-0.632948931301567)) ;
#106537=DIRECTION('center_axis',(-1.,0.,0.)) ;
#106538=DIRECTION('ref_axis',(0.,0.,1.)) ;
#106539=DIRECTION('center_axis',(0.,0.,1.)) ;
#106540=DIRECTION('ref_axis',(1.,0.,0.)) ;
#106541=DIRECTION('center_axis',(0.,0.,-1.)) ;
#106542=DIRECTION('ref_axis',(1.,0.,0.)) ;
#106543=DIRECTION('center_axis',(0.,0.,-1.)) ;
#106544=DIRECTION('ref_axis',(-1.,0.,0.)) ;
#106545=DIRECTION('center_axis',(0.,0.,1.)) ;
#106546=DIRECTION('ref_axis',(1.,0.,0.)) ;
#106547=DIRECTION('center_axis',(0.,0.,-1.)) ;
#106548=DIRECTION('ref_axis',(-1.,0.,0.)) ;
#106549=DIRECTION('center_axis',(0.,0.,1.)) ;
#106550=DIRECTION('ref_axis',(1.,0.,0.)) ;
#106551=DIRECTION('center_axis',(0.,0.,-1.)) ;
#106552=DIRECTION('ref_axis',(-1.,0.,0.)) ;
#106553=DIRECTION('center_axis',(0.,0.,1.)) ;
#106554=DIRECTION('ref_axis',(1.,0.,0.)) ;
#106555=DIRECTION('center_axis',(0.,0.,-1.)) ;
#106556=DIRECTION('ref_axis',(-1.,0.,0.)) ;
#106557=DIRECTION('center_axis',(0.,0.,1.)) ;
#106558=DIRECTION('ref_axis',(1.,0.,0.)) ;
#106559=DIRECTION('center_axis',(0.,0.,-1.)) ;
#106560=DIRECTION('ref_axis',(-1.,0.,0.)) ;
#106561=DIRECTION('center_axis',(0.,0.,1.)) ;
#106562=DIRECTION('ref_axis',(1.,0.,0.)) ;
#106563=DIRECTION('center_axis',(-0.422618261740697,0.,0.906307787036651)) ;
#106564=DIRECTION('ref_axis',(0.906307787036651,0.,0.422618261740697)) ;
#106565=DIRECTION('center_axis',(0.422618261740697,0.,-0.906307787036651)) ;
#106566=DIRECTION('ref_axis',(-0.906307787036651,0.,-0.422618261740697)) ;
#106567=DIRECTION('center_axis',(0.422618261740697,0.,-0.906307787036651)) ;
#106568=DIRECTION('ref_axis',(-0.906307787036651,0.,-0.422618261740697)) ;
#106569=DIRECTION('center_axis',(-0.422618261740697,0.,0.906307787036651)) ;
#106570=DIRECTION('ref_axis',(0.906307787036651,0.,0.422618261740697)) ;
#106571=DIRECTION('center_axis',(0.,0.,-1.)) ;
#106572=DIRECTION('ref_axis',(-1.,0.,0.)) ;
#106573=DIRECTION('center_axis',(0.,0.,1.)) ;
#106574=DIRECTION('ref_axis',(1.,0.,0.)) ;
#106575=DIRECTION('center_axis',(0.,0.,-1.)) ;
#106576=DIRECTION('ref_axis',(-1.,0.,0.)) ;
#106577=DIRECTION('center_axis',(0.,0.,1.)) ;
#106578=DIRECTION('ref_axis',(1.,0.,0.)) ;
#106579=DIRECTION('center_axis',(0.,0.,1.)) ;
#106580=DIRECTION('ref_axis',(1.,0.,0.)) ;
#106581=DIRECTION('center_axis',(0.,0.,-1.)) ;
#106582=DIRECTION('ref_axis',(1.,0.,0.)) ;
#106583=DIRECTION('center_axis',(0.,1.,0.)) ;
#106584=DIRECTION('ref_axis',(1.,0.,0.)) ;
#106585=DIRECTION('center_axis',(0.,-0.986393923832144,0.164398987305358)) ;
#106586=DIRECTION('ref_axis',(0.,-0.164398987305358,-0.986393923832144)) ;
#106587=DIRECTION('center_axis',(0.,0.986393923832144,-0.164398987305357)) ;
#106588=DIRECTION('ref_axis',(0.,0.164398987305357,0.986393923832144)) ;
#106589=DIRECTION('center_axis',(0.,-0.986393923832144,0.164398987305358)) ;
#106590=DIRECTION('ref_axis',(0.,-0.164398987305358,-0.986393923832144)) ;
#106591=DIRECTION('center_axis',(-1.,0.,0.)) ;
#106592=DIRECTION('ref_axis',(0.,0.107567764393767,-0.994197755008191)) ;
#106593=DIRECTION('center_axis',(4.02631181035923E-15,-0.928404294083138,
-0.371571617226061)) ;
#106594=DIRECTION('ref_axis',(-1.28610411910257E-29,0.371571617226061,-0.928404294083138)) ;
#106595=DIRECTION('center_axis',(0.275516865537137,-0.50093975551097,-0.820457078800105)) ;
#106596=DIRECTION('ref_axis',(3.47276585739718E-16,0.853490367006418,-0.521108619605597)) ;
#106597=DIRECTION('center_axis',(0.,0.,-1.)) ;
#106598=DIRECTION('ref_axis',(-1.,0.,0.)) ;
#106599=DIRECTION('center_axis',(0.,0.,-1.)) ;
#106600=DIRECTION('ref_axis',(-1.,0.,0.)) ;
#106601=DIRECTION('center_axis',(0.,0.,-1.)) ;
#106602=DIRECTION('ref_axis',(-1.,0.,0.)) ;
#106603=DIRECTION('center_axis',(0.,0.,-1.)) ;
#106604=DIRECTION('ref_axis',(-1.,0.,0.)) ;
#106605=DIRECTION('center_axis',(0.,0.,-1.)) ;
#106606=DIRECTION('ref_axis',(-1.,0.,0.)) ;
#106607=DIRECTION('center_axis',(-0.275516865538071,0.500939755523742,-0.820457078791993)) ;
#106608=DIRECTION('ref_axis',(1.34532370065023E-15,0.853490366998217,0.521108619619028)) ;
#106609=DIRECTION('center_axis',(0.,-0.986393923832144,-0.164398987305357)) ;
#106610=DIRECTION('ref_axis',(0.,0.164398987305357,-0.986393923832144)) ;
#106611=DIRECTION('center_axis',(3.5648347838177E-16,0.986393923832144,
0.164398987305358)) ;
#106612=DIRECTION('ref_axis',(3.79675591822878E-31,-0.164398987305358,0.986393923832144)) ;
#106613=DIRECTION('center_axis',(0.,1.,0.)) ;
#106614=DIRECTION('ref_axis',(1.,0.,0.)) ;
#106615=DIRECTION('center_axis',(-1.,0.,0.)) ;
#106616=DIRECTION('ref_axis',(0.,0.,1.)) ;
#106617=DIRECTION('center_axis',(0.,0.,-1.)) ;
#106618=DIRECTION('ref_axis',(-1.,0.,0.)) ;
#106619=DIRECTION('center_axis',(2.168404344971E-15,0.,1.)) ;
#106620=DIRECTION('ref_axis',(1.,0.,-2.168404344971E-15)) ;
#106621=DIRECTION('center_axis',(0.,0.,-1.)) ;
#106622=DIRECTION('ref_axis',(-1.,0.,0.)) ;
#106623=DIRECTION('center_axis',(0.,0.,-1.)) ;
#106624=DIRECTION('ref_axis',(-1.,0.,0.)) ;
#106625=DIRECTION('center_axis',(2.168404344971E-15,0.,1.)) ;
#106626=DIRECTION('ref_axis',(1.,0.,-2.168404344971E-15)) ;
#106627=DIRECTION('center_axis',(0.795723237447208,-7.53302716311723E-12,
0.605660407643206)) ;
#106628=DIRECTION('ref_axis',(0.605660407643206,-5.87919516709105E-26,-0.795723237447208)) ;
#106629=DIRECTION('center_axis',(1.57772181044204E-26,2.36658271566302E-26,
1.)) ;
#106630=DIRECTION('ref_axis',(3.73380916671669E-52,-1.,2.36658271566302E-26)) ;
#106631=DIRECTION('center_axis',(-0.795723237415222,-2.11663082418553E-11,
0.605660407685229)) ;
#106632=DIRECTION('ref_axis',(0.605660407685229,1.1913710773826E-25,0.795723237415222)) ;
#106633=DIRECTION('center_axis',(0.,0.,-1.)) ;
#106634=DIRECTION('ref_axis',(-1.,0.,0.)) ;
#106635=DIRECTION('center_axis',(0.147618562252691,0.989044367093028,0.)) ;
#106636=DIRECTION('ref_axis',(-0.989044367093028,0.147618562252691,0.)) ;
#106637=DIRECTION('',(0.,0.,1.)) ;
#106638=DIRECTION('',(0.989044367093028,-0.147618562252691,0.)) ;
#106639=DIRECTION('',(0.,0.,1.)) ;
#106640=DIRECTION('',(-0.989044367093028,0.147618562252691,0.)) ;
#106641=DIRECTION('center_axis',(0.,0.,1.)) ;
#106642=DIRECTION('ref_axis',(1.,0.,0.)) ;
#106643=DIRECTION('center_axis',(0.,0.,-1.)) ;
#106644=DIRECTION('ref_axis',(1.,0.,0.)) ;
#106645=DIRECTION('',(0.,0.,1.)) ;
#106646=DIRECTION('center_axis',(0.,0.,1.)) ;
#106647=DIRECTION('ref_axis',(1.,0.,0.)) ;
#106648=DIRECTION('center_axis',(0.697619267438899,0.716468671818953,0.)) ;
#106649=DIRECTION('ref_axis',(-0.716468671818953,0.697619267438899,0.)) ;
#106650=DIRECTION('',(0.716468671818953,-0.697619267438899,0.)) ;
#106651=DIRECTION('',(0.,0.,1.)) ;
#106652=DIRECTION('',(-0.716468671818953,0.697619267438899,0.)) ;
#106653=DIRECTION('center_axis',(0.,0.,1.)) ;
#106654=DIRECTION('ref_axis',(1.,0.,0.)) ;
#106655=DIRECTION('center_axis',(0.,0.,-1.)) ;
#106656=DIRECTION('ref_axis',(1.,0.,0.)) ;
#106657=DIRECTION('',(0.,0.,1.)) ;
#106658=DIRECTION('center_axis',(0.,0.,1.)) ;
#106659=DIRECTION('ref_axis',(1.,0.,0.)) ;
#106660=DIRECTION('center_axis',(1.,0.,0.)) ;
#106661=DIRECTION('ref_axis',(0.,0.,-1.)) ;
#106662=DIRECTION('',(0.,-1.,0.)) ;
#106663=DIRECTION('',(0.,0.,1.)) ;
#106664=DIRECTION('',(0.,1.,0.)) ;
#106665=DIRECTION('center_axis',(0.,0.,1.)) ;
#106666=DIRECTION('ref_axis',(1.,0.,0.)) ;
#106667=DIRECTION('center_axis',(0.,0.,-1.)) ;
#106668=DIRECTION('ref_axis',(1.,0.,0.)) ;
#106669=DIRECTION('',(0.,0.,1.)) ;
#106670=DIRECTION('center_axis',(0.,0.,1.)) ;
#106671=DIRECTION('ref_axis',(1.,0.,0.)) ;
#106672=DIRECTION('center_axis',(-0.453905661840943,-0.891049746169503,
0.)) ;
#106673=DIRECTION('ref_axis',(0.891049746169503,-0.453905661840943,0.)) ;
#106674=DIRECTION('',(-0.891049746169503,0.453905661840943,0.)) ;
#106675=DIRECTION('',(0.,0.,1.)) ;
#106676=DIRECTION('',(0.891049746169503,-0.453905661840943,0.)) ;
#106677=DIRECTION('center_axis',(0.,0.,1.)) ;
#106678=DIRECTION('ref_axis',(1.,0.,0.)) ;
#106679=DIRECTION('center_axis',(0.,0.,1.)) ;
#106680=DIRECTION('ref_axis',(1.,0.,0.)) ;
#106681=DIRECTION('',(0.,0.,1.)) ;
#106682=DIRECTION('center_axis',(0.,0.,-1.)) ;
#106683=DIRECTION('ref_axis',(1.,0.,0.)) ;
#106684=DIRECTION('center_axis',(-2.60782465076463E-16,-1.,0.)) ;
#106685=DIRECTION('ref_axis',(1.,-2.60782465076463E-16,0.)) ;
#106686=DIRECTION('',(-1.,2.60782465076463E-16,0.)) ;
#106687=DIRECTION('',(0.,0.,-1.)) ;
#106688=DIRECTION('',(1.,-2.60782465076463E-16,0.)) ;
#106689=DIRECTION('center_axis',(0.,0.,1.)) ;
#106690=DIRECTION('ref_axis',(1.,0.,0.)) ;
#106691=DIRECTION('center_axis',(0.,0.,1.)) ;
#106692=DIRECTION('ref_axis',(1.,0.,0.)) ;
#106693=DIRECTION('',(-1.,2.60782465076463E-16,0.)) ;
#106694=DIRECTION('',(0.,1.,0.)) ;
#106695=DIRECTION('',(0.989044367093028,-0.147618562252691,0.)) ;
#106696=DIRECTION('',(0.716468671818953,-0.697619267438899,0.)) ;
#106697=DIRECTION('',(0.,-1.,0.)) ;
#106698=DIRECTION('',(-0.891049746169503,0.453905661840943,0.)) ;
#106699=DIRECTION('center_axis',(0.,0.,1.)) ;
#106700=DIRECTION('ref_axis',(1.,0.,0.)) ;
#106701=DIRECTION('',(-0.716468671818953,0.697619267438899,0.)) ;
#106702=DIRECTION('',(-0.989044367093028,0.147618562252691,0.)) ;
#106703=DIRECTION('',(0.,-1.,0.)) ;
#106704=DIRECTION('',(1.,-2.60782465076463E-16,0.)) ;
#106705=DIRECTION('center_axis',(0.,0.,-1.)) ;
#106706=DIRECTION('ref_axis',(1.,0.,0.)) ;
#106707=DIRECTION('',(0.891049746169503,-0.453905661840943,0.)) ;
#106708=DIRECTION('',(0.,1.,0.)) ;
#106709=DIRECTION('center_axis',(-2.09002828430941E-16,1.,0.)) ;
#106710=DIRECTION('ref_axis',(-1.,-2.09002828430941E-16,0.)) ;
#106711=DIRECTION('',(1.,2.09002828430941E-16,0.)) ;
#106712=DIRECTION('',(0.,0.,-1.)) ;
#106713=DIRECTION('',(1.,2.09002828430941E-16,0.)) ;
#106714=DIRECTION('',(0.,0.,1.)) ;
#106715=DIRECTION('center_axis',(0.,1.,0.)) ;
#106716=DIRECTION('ref_axis',(0.,0.,1.)) ;
#106717=DIRECTION('',(0.422618261740697,0.,-0.906307787036651)) ;
#106718=DIRECTION('center_axis',(1.0450141421547E-16,-1.,0.)) ;
#106719=DIRECTION('ref_axis',(1.,1.0450141421547E-16,0.)) ;
#106720=DIRECTION('',(-1.,-1.0450141421547E-16,1.7416902369245E-17)) ;
#106721=DIRECTION('',(0.,0.,1.)) ;
#106722=DIRECTION('',(-1.,-1.0450141421547E-16,0.)) ;
#106723=DIRECTION('',(0.,0.,-1.)) ;
#106724=DIRECTION('center_axis',(-1.,0.,0.)) ;
#106725=DIRECTION('ref_axis',(0.,0.,1.)) ;
#106726=DIRECTION('',(0.,1.,0.)) ;
#106727=DIRECTION('',(0.,0.,-1.)) ;
#106728=DIRECTION('center_axis',(-1.,0.,0.)) ;
#106729=DIRECTION('ref_axis',(0.,0.,1.)) ;
#106730=DIRECTION('',(0.,0.,1.)) ;
#106731=DIRECTION('center_axis',(0.,0.,1.)) ;
#106732=DIRECTION('ref_axis',(1.,0.,0.)) ;
#106733=DIRECTION('center_axis',(0.,0.,1.)) ;
#106734=DIRECTION('ref_axis',(1.,0.,0.)) ;
#106735=DIRECTION('center_axis',(0.,0.,-1.)) ;
#106736=DIRECTION('ref_axis',(1.,0.,0.)) ;
#106737=DIRECTION('center_axis',(0.,0.,1.)) ;
#106738=DIRECTION('ref_axis',(1.,0.,0.)) ;
#106739=DIRECTION('center_axis',(0.,0.,1.)) ;
#106740=DIRECTION('ref_axis',(1.,0.,0.)) ;
#106741=DIRECTION('center_axis',(0.,0.,-1.)) ;
#106742=DIRECTION('ref_axis',(1.,0.,0.)) ;
#106743=DIRECTION('center_axis',(0.,0.,1.)) ;
#106744=DIRECTION('ref_axis',(1.,0.,0.)) ;
#106745=DIRECTION('',(-0.664363838829919,0.74740931868366,0.)) ;
#106746=DIRECTION('',(0.,-1.,0.)) ;
#106747=DIRECTION('',(0.894427190999917,0.447213595499956,0.)) ;
#106748=DIRECTION('',(0.,1.,0.)) ;
#106749=DIRECTION('center_axis',(0.,0.,-1.)) ;
#106750=DIRECTION('ref_axis',(-1.,0.,0.)) ;
#106751=DIRECTION('',(-0.894427190999917,-0.447213595499956,0.)) ;
#106752=DIRECTION('',(0.,1.,0.)) ;
#106753=DIRECTION('',(0.664363838829919,-0.74740931868366,0.)) ;
#106754=DIRECTION('',(0.,-1.,0.)) ;
#106755=DIRECTION('center_axis',(-0.23745309047699,0.,-0.971399006496778)) ;
#106756=DIRECTION('ref_axis',(-0.971399006496778,0.,0.23745309047699)) ;
#106757=DIRECTION('center_axis',(-0.237453090476986,2.27991133847471E-14,
-0.971399006496778)) ;
#106758=DIRECTION('ref_axis',(0.921799787669962,-0.315455332296274,-0.225328836985994)) ;
#106759=DIRECTION('',(0.971399006496777,0.,-0.23745309047699)) ;
#106760=DIRECTION('',(0.,-1.,0.)) ;
#106761=DIRECTION('',(-0.971399006496777,0.,0.23745309047699)) ;
#106762=DIRECTION('center_axis',(-0.237453090477116,4.55640954056451E-13,
-0.971399006496747)) ;
#106763=DIRECTION('ref_axis',(0.954559354253584,0.18539258117475,-0.233336731039809)) ;
#106764=DIRECTION('',(-0.873786407766991,-0.436893203883493,0.213592233009709)) ;
#106765=DIRECTION('',(0.,1.,0.)) ;
#106766=DIRECTION('',(0.655772517804503,-0.737744082530068,-0.160299948796656)) ;
#106767=DIRECTION('center_axis',(-1.,0.,0.)) ;
#106768=DIRECTION('ref_axis',(0.,0.,1.)) ;
#106769=DIRECTION('',(0.,-1.,0.)) ;
#106770=DIRECTION('center_axis',(-1.,-6.7007887082719E-15,-6.50913949396006E-15)) ;
#106771=DIRECTION('ref_axis',(6.50913949401742E-15,-8.55940926010333E-12,
-1.)) ;
#106772=DIRECTION('',(0.,0.,-1.)) ;
#106773=DIRECTION('center_axis',(-1.,-6.70078870827233E-15,6.50913949396061E-15)) ;
#106774=DIRECTION('ref_axis',(-6.50913949402726E-15,9.94624019410426E-12,
-1.)) ;
#106775=DIRECTION('center_axis',(-1.,6.70078870827237E-15,6.50913949396064E-15)) ;
#106776=DIRECTION('ref_axis',(-6.50913949394999E-15,1.589491041799E-12,
-1.)) ;
#106777=DIRECTION('',(0.,0.,-1.)) ;
#106778=DIRECTION('center_axis',(-1.,6.70078870827261E-15,-6.50913949396074E-15)) ;
#106779=DIRECTION('ref_axis',(6.50913949379813E-15,-2.42675544807721E-11,
-1.)) ;
#106780=DIRECTION('center_axis',(-0.23745309047699,0.,0.971399006496778)) ;
#106781=DIRECTION('ref_axis',(0.971399006496778,0.,0.23745309047699)) ;
#106782=DIRECTION('center_axis',(-0.237453090476854,-6.19298088178216E-13,
0.971399006496811)) ;
#106783=DIRECTION('ref_axis',(0.954559354253699,0.185392581174206,0.23333673103977)) ;
#106784=DIRECTION('',(0.971399006496777,0.,0.23745309047699)) ;
#106785=DIRECTION('',(-0.971399006496777,0.,-0.23745309047699)) ;
#106786=DIRECTION('center_axis',(-0.237453090477054,-1.72356340859612E-13,
0.971399006496762)) ;
#106787=DIRECTION('ref_axis',(0.9217997876717,-0.315455332290889,0.225328836986424)) ;
#106788=DIRECTION('',(-0.655772517804503,0.737744082530068,-0.160299948796656)) ;
#106789=DIRECTION('',(0.,-1.,0.)) ;
#106790=DIRECTION('',(0.873786407766991,0.436893203883493,0.213592233009709)) ;
#106791=DIRECTION('center_axis',(0.,1.,0.)) ;
#106792=DIRECTION('ref_axis',(0.,0.,1.)) ;
#106793=DIRECTION('',(-0.971399006496777,0.,0.23745309047699)) ;
#106794=DIRECTION('',(0.,0.,-1.)) ;
#106795=DIRECTION('',(0.971399006496777,0.,0.23745309047699)) ;
#106796=DIRECTION('center_axis',(0.,1.,0.)) ;
#106797=DIRECTION('ref_axis',(0.,0.,1.)) ;
#106798=DIRECTION('',(-0.971399006496777,0.,-0.23745309047699)) ;
#106799=DIRECTION('',(0.,0.,1.)) ;
#106800=DIRECTION('',(0.971399006496777,0.,-0.23745309047699)) ;
#106801=DIRECTION('center_axis',(-0.447213595499956,0.894427190999917,0.)) ;
#106802=DIRECTION('ref_axis',(0.,0.,-1.)) ;
#106803=DIRECTION('',(0.,0.,-1.)) ;
#106804=DIRECTION('',(-0.873786407766991,-0.436893203883493,-0.213592233009709)) ;
#106805=DIRECTION('',(-0.894427190999917,-0.447213595499956,0.)) ;
#106806=DIRECTION('',(0.,0.,1.)) ;
#106807=DIRECTION('',(0.894427190999917,0.447213595499956,0.)) ;
#106808=DIRECTION('',(0.873786407766991,0.436893203883493,-0.213592233009709)) ;
#106809=DIRECTION('center_axis',(0.74740931868366,0.664363838829919,0.)) ;
#106810=DIRECTION('ref_axis',(0.,0.,1.)) ;
#106811=DIRECTION('',(0.,0.,-1.)) ;
#106812=DIRECTION('',(0.664363838829919,-0.74740931868366,0.)) ;
#106813=DIRECTION('',(0.655772517804503,-0.737744082530068,0.160299948796656)) ;
#106814=DIRECTION('',(0.,0.,1.)) ;
#106815=DIRECTION('',(-0.655772517804503,0.737744082530068,0.160299948796656)) ;
#106816=DIRECTION('',(-0.664363838829919,0.74740931868366,0.)) ;
#106817=DIRECTION('center_axis',(1.,0.,4.33680868994202E-16)) ;
#106818=DIRECTION('ref_axis',(4.33680868994202E-16,0.,-1.)) ;
#106819=DIRECTION('',(0.,1.,0.)) ;
#106820=DIRECTION('',(4.33680868994202E-16,0.,-1.)) ;
#106821=DIRECTION('',(0.,-1.,0.)) ;
#106822=DIRECTION('',(-4.33680868994202E-16,0.,1.)) ;
#106823=DIRECTION('center_axis',(-1.73472347597681E-16,0.,-1.)) ;
#106824=DIRECTION('ref_axis',(-1.,0.,1.73472347597681E-16)) ;
#106825=DIRECTION('',(-1.,0.,1.73472347597681E-16)) ;
#106826=DIRECTION('',(0.,-1.,0.)) ;
#106827=DIRECTION('',(1.,0.,-1.73472347597681E-16)) ;
#106828=DIRECTION('',(0.,1.,0.)) ;
#106829=DIRECTION('center_axis',(-1.,0.,0.)) ;
#106830=DIRECTION('ref_axis',(0.,0.,1.)) ;
#106831=DIRECTION('',(0.,0.,1.)) ;
#106832=DIRECTION('',(0.,-1.,0.)) ;
#106833=DIRECTION('',(0.,0.,-1.)) ;
#106834=DIRECTION('',(0.,1.,0.)) ;
#106835=DIRECTION('center_axis',(-1.73472347597681E-16,0.,1.)) ;
#106836=DIRECTION('ref_axis',(1.,0.,1.73472347597681E-16)) ;
#106837=DIRECTION('',(0.,1.,0.)) ;
#106838=DIRECTION('',(1.,0.,1.73472347597681E-16)) ;
#106839=DIRECTION('',(0.,-1.,0.)) ;
#106840=DIRECTION('',(-1.,0.,-1.73472347597681E-16)) ;
#106841=DIRECTION('center_axis',(0.,-1.,0.)) ;
#106842=DIRECTION('ref_axis',(0.,0.,-1.)) ;
#106843=DIRECTION('',(-1.,0.,-1.73472347597681E-16)) ;
#106844=DIRECTION('',(0.,0.,-1.)) ;
#106845=DIRECTION('',(1.,0.,-1.73472347597681E-16)) ;
#106846=DIRECTION('',(-4.33680868994202E-16,0.,1.)) ;
#106847=DIRECTION('',(1.,0.,0.)) ;
#106848=DIRECTION('center_axis',(0.,-1.,0.)) ;
#106849=DIRECTION('ref_axis',(0.,0.,-1.)) ;
#106850=DIRECTION('',(0.,0.,-1.)) ;
#106851=DIRECTION('center_axis',(0.,-1.,0.)) ;
#106852=DIRECTION('ref_axis',(0.,0.,-1.)) ;
#106853=DIRECTION('',(-1.,0.,0.)) ;
#106854=DIRECTION('center_axis',(0.,-1.,0.)) ;
#106855=DIRECTION('ref_axis',(0.,0.,1.)) ;
#106856=DIRECTION('',(0.,0.,1.)) ;
#106857=DIRECTION('center_axis',(0.,-1.,0.)) ;
#106858=DIRECTION('ref_axis',(0.,0.,-1.)) ;
#106859=DIRECTION('center_axis',(0.,-1.,0.)) ;
#106860=DIRECTION('ref_axis',(0.,0.,-1.)) ;
#106861=DIRECTION('center_axis',(0.,-1.,0.)) ;
#106862=DIRECTION('ref_axis',(0.,0.,-1.)) ;
#106863=DIRECTION('',(0.,-1.,0.)) ;
#106864=DIRECTION('',(0.,-1.,0.)) ;
#106865=DIRECTION('center_axis',(0.,0.,-1.)) ;
#106866=DIRECTION('ref_axis',(-1.,0.,0.)) ;
#106867=DIRECTION('',(1.,0.,0.)) ;
#106868=DIRECTION('',(0.,-1.,0.)) ;
#106869=DIRECTION('center_axis',(0.,-1.,0.)) ;
#106870=DIRECTION('ref_axis',(0.,0.,-1.)) ;
#106871=DIRECTION('center_axis',(0.,-1.,0.)) ;
#106872=DIRECTION('ref_axis',(0.,0.,-1.)) ;
#106873=DIRECTION('',(0.,-1.,0.)) ;
#106874=DIRECTION('center_axis',(-1.,0.,0.)) ;
#106875=DIRECTION('ref_axis',(0.,0.,1.)) ;
#106876=DIRECTION('',(0.,0.,-1.)) ;
#106877=DIRECTION('',(0.,-1.,0.)) ;
#106878=DIRECTION('center_axis',(0.,-1.,0.)) ;
#106879=DIRECTION('ref_axis',(0.,0.,-1.)) ;
#106880=DIRECTION('center_axis',(0.,-1.,0.)) ;
#106881=DIRECTION('ref_axis',(0.,0.,-1.)) ;
#106882=DIRECTION('',(0.,-1.,0.)) ;
#106883=DIRECTION('center_axis',(0.,0.,1.)) ;
#106884=DIRECTION('ref_axis',(1.,0.,0.)) ;
#106885=DIRECTION('',(-1.,0.,0.)) ;
#106886=DIRECTION('',(0.,-1.,0.)) ;
#106887=DIRECTION('center_axis',(0.,-1.,0.)) ;
#106888=DIRECTION('ref_axis',(0.,0.,-1.)) ;
#106889=DIRECTION('center_axis',(0.,-1.,0.)) ;
#106890=DIRECTION('ref_axis',(0.,0.,1.)) ;
#106891=DIRECTION('',(0.,-1.,0.)) ;
#106892=DIRECTION('center_axis',(1.,0.,0.)) ;
#106893=DIRECTION('ref_axis',(0.,0.,-1.)) ;
#106894=DIRECTION('',(0.,0.,1.)) ;
#106895=DIRECTION('center_axis',(0.,-1.,0.)) ;
#106896=DIRECTION('ref_axis',(0.,0.,-1.)) ;
#106897=DIRECTION('center_axis',(0.,1.,0.)) ;
#106898=DIRECTION('ref_axis',(0.,0.,1.)) ;
#106899=DIRECTION('',(-0.422618261740697,0.,0.906307787036651)) ;
#106900=DIRECTION('center_axis',(0.906307787036651,0.,0.422618261740697)) ;
#106901=DIRECTION('ref_axis',(0.422618261740697,0.,-0.906307787036651)) ;
#106902=DIRECTION('',(-0.422618261740697,0.,0.906307787036651)) ;
#106903=DIRECTION('',(0.422618261740697,0.,-0.906307787036651)) ;
#106904=DIRECTION('center_axis',(-0.906307787036651,0.,-0.422618261740697)) ;
#106905=DIRECTION('ref_axis',(-0.422618261740697,0.,0.906307787036651)) ;
#106906=DIRECTION('',(0.422618261740697,0.,-0.906307787036651)) ;
#106907=DIRECTION('',(-0.422618261740697,0.,0.906307787036651)) ;
#106908=DIRECTION('center_axis',(0.,1.,0.)) ;
#106909=DIRECTION('ref_axis',(0.,0.,1.)) ;
#106910=DIRECTION('',(-0.422618261740697,0.,0.906307787036651)) ;
#106911=DIRECTION('',(0.422618261740697,0.,-0.906307787036651)) ;
#106912=DIRECTION('center_axis',(1.,0.,-2.16840434497101E-16)) ;
#106913=DIRECTION('ref_axis',(-2.16840434497101E-16,0.,-1.)) ;
#106914=DIRECTION('',(2.16840434497101E-16,0.,1.)) ;
#106915=DIRECTION('',(0.,1.,0.)) ;
#106916=DIRECTION('',(-2.16840434497101E-16,0.,-1.)) ;
#106917=DIRECTION('',(0.,-1.,0.)) ;
#106918=DIRECTION('center_axis',(1.73472347597681E-16,0.,1.)) ;
#106919=DIRECTION('ref_axis',(1.,0.,-1.73472347597681E-16)) ;
#106920=DIRECTION('',(0.,-1.,0.)) ;
#106921=DIRECTION('',(-1.,0.,1.73472347597681E-16)) ;
#106922=DIRECTION('',(0.,1.,0.)) ;
#106923=DIRECTION('',(1.,0.,-1.73472347597681E-16)) ;
#106924=DIRECTION('center_axis',(-1.,0.,2.16840434497101E-16)) ;
#106925=DIRECTION('ref_axis',(2.16840434497101E-16,0.,1.)) ;
#106926=DIRECTION('',(0.,-1.,0.)) ;
#106927=DIRECTION('',(-2.16840434497101E-16,0.,-1.)) ;
#106928=DIRECTION('',(0.,1.,0.)) ;
#106929=DIRECTION('',(2.16840434497101E-16,0.,1.)) ;
#106930=DIRECTION('center_axis',(-1.73472347597681E-16,0.,-1.)) ;
#106931=DIRECTION('ref_axis',(-1.,0.,1.73472347597681E-16)) ;
#106932=DIRECTION('',(1.,0.,-1.73472347597681E-16)) ;
#106933=DIRECTION('',(0.,1.,0.)) ;
#106934=DIRECTION('',(-1.,0.,1.73472347597681E-16)) ;
#106935=DIRECTION('',(0.,-1.,0.)) ;
#106936=DIRECTION('center_axis',(0.,1.,0.)) ;
#106937=DIRECTION('ref_axis',(0.,0.,1.)) ;
#106938=DIRECTION('',(1.,0.,-1.73472347597681E-16)) ;
#106939=DIRECTION('',(-2.16840434497101E-16,0.,-1.)) ;
#106940=DIRECTION('',(-1.,0.,1.73472347597681E-16)) ;
#106941=DIRECTION('',(2.16840434497101E-16,0.,1.)) ;
#106942=DIRECTION('',(1.,0.,0.)) ;
#106943=DIRECTION('center_axis',(0.,1.,0.)) ;
#106944=DIRECTION('ref_axis',(0.,0.,1.)) ;
#106945=DIRECTION('',(0.,0.,1.)) ;
#106946=DIRECTION('center_axis',(0.,1.,0.)) ;
#106947=DIRECTION('ref_axis',(0.,0.,1.)) ;
#106948=DIRECTION('',(-1.,0.,0.)) ;
#106949=DIRECTION('center_axis',(0.,1.,0.)) ;
#106950=DIRECTION('ref_axis',(0.,0.,-1.)) ;
#106951=DIRECTION('',(0.,0.,-1.)) ;
#106952=DIRECTION('center_axis',(0.,1.,0.)) ;
#106953=DIRECTION('ref_axis',(0.,0.,1.)) ;
#106954=DIRECTION('center_axis',(0.,1.,0.)) ;
#106955=DIRECTION('ref_axis',(0.,0.,1.)) ;
#106956=DIRECTION('',(0.,1.,0.)) ;
#106957=DIRECTION('center_axis',(0.,-1.,0.)) ;
#106958=DIRECTION('ref_axis',(2.60208521396523E-14,0.,1.)) ;
#106959=DIRECTION('',(0.,1.,0.)) ;
#106960=DIRECTION('center_axis',(0.,0.,1.)) ;
#106961=DIRECTION('ref_axis',(1.,0.,0.)) ;
#106962=DIRECTION('',(-1.,0.,0.)) ;
#106963=DIRECTION('',(0.,1.,0.)) ;
#106964=DIRECTION('center_axis',(0.,1.,0.)) ;
#106965=DIRECTION('ref_axis',(0.,0.,1.)) ;
#106966=DIRECTION('center_axis',(0.,-1.,0.)) ;
#106967=DIRECTION('ref_axis',(0.,0.,1.)) ;
#106968=DIRECTION('',(0.,1.,0.)) ;
#106969=DIRECTION('center_axis',(-1.,0.,0.)) ;
#106970=DIRECTION('ref_axis',(0.,0.,1.)) ;
#106971=DIRECTION('',(0.,0.,-1.)) ;
#106972=DIRECTION('',(0.,1.,0.)) ;
#106973=DIRECTION('center_axis',(0.,1.,0.)) ;
#106974=DIRECTION('ref_axis',(0.,0.,1.)) ;
#106975=DIRECTION('center_axis',(0.,-1.,0.)) ;
#106976=DIRECTION('ref_axis',(0.,0.,1.)) ;
#106977=DIRECTION('',(0.,1.,0.)) ;
#106978=DIRECTION('center_axis',(0.,0.,-1.)) ;
#106979=DIRECTION('ref_axis',(-1.,0.,0.)) ;
#106980=DIRECTION('',(1.,0.,0.)) ;
#106981=DIRECTION('',(0.,1.,0.)) ;
#106982=DIRECTION('center_axis',(0.,1.,0.)) ;
#106983=DIRECTION('ref_axis',(0.,0.,1.)) ;
#106984=DIRECTION('center_axis',(0.,-1.,0.)) ;
#106985=DIRECTION('ref_axis',(0.,0.,1.)) ;
#106986=DIRECTION('',(0.,1.,0.)) ;
#106987=DIRECTION('center_axis',(1.,0.,0.)) ;
#106988=DIRECTION('ref_axis',(0.,0.,-1.)) ;
#106989=DIRECTION('',(0.,0.,1.)) ;
#106990=DIRECTION('center_axis',(0.,1.,0.)) ;
#106991=DIRECTION('ref_axis',(0.,0.,1.)) ;
#106992=DIRECTION('',(1.,0.,0.)) ;
#106993=DIRECTION('',(0.,0.,-1.)) ;
#106994=DIRECTION('',(-1.,0.,0.)) ;
#106995=DIRECTION('',(0.,0.,1.)) ;
#106996=DIRECTION('center_axis',(0.,0.164398987305357,-0.986393923832144)) ;
#106997=DIRECTION('ref_axis',(0.,0.986393923832144,0.164398987305357)) ;
#106998=DIRECTION('',(-1.,-1.0450141421547E-16,-1.7416902369245E-17)) ;
#106999=DIRECTION('',(0.,-0.986393923832144,-0.164398987305357)) ;
#107000=DIRECTION('',(1.,0.,0.)) ;
#107001=DIRECTION('',(0.,0.986393923832144,0.164398987305357)) ;
#107002=DIRECTION('center_axis',(0.,-1.,0.)) ;
#107003=DIRECTION('ref_axis',(0.,0.,-1.)) ;
#107004=DIRECTION('',(0.,0.,1.)) ;
#107005=DIRECTION('',(0.,0.,-1.)) ;
#107006=DIRECTION('',(-1.,0.,0.)) ;
#107007=DIRECTION('center_axis',(0.,0.164398987305357,0.986393923832144)) ;
#107008=DIRECTION('ref_axis',(0.,-0.986393923832144,0.164398987305357)) ;
#107009=DIRECTION('',(0.,0.986393923832144,-0.164398987305357)) ;
#107010=DIRECTION('',(1.,1.0450141421547E-16,-1.7416902369245E-17)) ;
#107011=DIRECTION('',(0.,-0.986393923832144,0.164398987305357)) ;
#107012=DIRECTION('center_axis',(-1.,0.,0.)) ;
#107013=DIRECTION('ref_axis',(0.,0.,1.)) ;
#107014=DIRECTION('',(0.,0.,1.)) ;
#107015=DIRECTION('center_axis',(-1.,0.,0.)) ;
#107016=DIRECTION('ref_axis',(0.,0.,1.)) ;
#107017=DIRECTION('',(0.,-0.986393923832144,0.164398987305357)) ;
#107018=DIRECTION('',(0.,0.,-1.)) ;
#107019=DIRECTION('',(0.,0.986393923832144,0.164398987305357)) ;
#107020=DIRECTION('center_axis',(1.,0.,0.)) ;
#107021=DIRECTION('ref_axis',(0.,0.,-1.)) ;
#107022=DIRECTION('center_axis',(1.,0.,0.)) ;
#107023=DIRECTION('ref_axis',(0.,0.,-1.)) ;
#107024=DIRECTION('center_axis',(1.,0.,0.)) ;
#107025=DIRECTION('ref_axis',(0.,0.,1.)) ;
#107026=DIRECTION('center_axis',(1.,0.,0.)) ;
#107027=DIRECTION('ref_axis',(0.,1.77635683940025E-15,1.)) ;
#107028=DIRECTION('center_axis',(1.,0.,0.)) ;
#107029=DIRECTION('ref_axis',(0.,-3.5527136788005E-15,1.)) ;
#107030=DIRECTION('',(1.,0.,0.)) ;
#107031=DIRECTION('center_axis',(-1.,0.,0.)) ;
#107032=DIRECTION('ref_axis',(0.,0.,1.)) ;
#107033=DIRECTION('',(-1.,0.,0.)) ;
#107034=DIRECTION('center_axis',(0.,0.,-1.)) ;
#107035=DIRECTION('ref_axis',(1.,0.,0.)) ;
#107036=DIRECTION('center_axis',(0.,-1.,0.)) ;
#107037=DIRECTION('ref_axis',(0.,0.,1.)) ;
#107038=DIRECTION('center_axis',(0.971399006496778,0.,-0.23745309047699)) ;
#107039=DIRECTION('ref_axis',(-0.23745309047699,0.,-0.971399006496778)) ;
#107040=DIRECTION('center_axis',(0.971399006496778,0.,-0.237453090476989)) ;
#107041=DIRECTION('ref_axis',(-0.237453090476989,0.,-0.971399006496778)) ;
#107042=DIRECTION('center_axis',(0.655772517804501,-0.73774408253007,-0.160299948796655)) ;
#107043=DIRECTION('ref_axis',(-0.747409318683662,-0.664363838829917,2.67307565105543E-16)) ;
#107044=DIRECTION('center_axis',(-0.439210132176044,-4.72063789540106E-10,
-0.898384360835551)) ;
#107045=DIRECTION('ref_axis',(0.882040291644445,-0.18988021424233,-0.43121969824565)) ;
#107046=DIRECTION('center_axis',(0.655772517804504,-0.737744082530068,-0.160299948796656)) ;
#107047=DIRECTION('ref_axis',(0.74740931868366,0.664363838829919,-2.08334010827303E-16)) ;
#107048=DIRECTION('center_axis',(0.655772517804505,-0.737744082530068,-0.16029994879665)) ;
#107049=DIRECTION('ref_axis',(0.74740931868366,0.66436383882992,-5.75609428574487E-16)) ;
#107050=DIRECTION('center_axis',(0.664363838829919,-0.74740931868366,0.)) ;
#107051=DIRECTION('ref_axis',(0.74740931868366,0.664363838829919,0.)) ;
#107052=DIRECTION('center_axis',(-0.664363838829918,0.747409318683661,0.)) ;
#107053=DIRECTION('ref_axis',(-0.747409318683661,-0.664363838829918,0.)) ;
#107054=DIRECTION('center_axis',(0.,1.,0.)) ;
#107055=DIRECTION('ref_axis',(0.,0.,1.)) ;
#107056=DIRECTION('center_axis',(0.,-1.,0.)) ;
#107057=DIRECTION('ref_axis',(0.,0.,-1.)) ;
#107058=DIRECTION('center_axis',(0.,0.,1.)) ;
#107059=DIRECTION('ref_axis',(1.,0.,0.)) ;
#107060=DIRECTION('center_axis',(0.,0.,-1.)) ;
#107061=DIRECTION('ref_axis',(-1.,0.,0.)) ;
#107062=DIRECTION('center_axis',(0.,0.,-1.)) ;
#107063=DIRECTION('ref_axis',(-1.,0.,0.)) ;
#107064=DIRECTION('center_axis',(0.439210132175102,4.69462404501499E-10,
-0.898384360836012)) ;
#107065=DIRECTION('ref_axis',(0.882040291646306,-0.189880214232972,0.431219698245964)) ;
#107066=DIRECTION('center_axis',(-0.971399006496778,0.,-0.23745309047699)) ;
#107067=DIRECTION('ref_axis',(-0.23745309047699,0.,0.971399006496778)) ;
#107068=DIRECTION('center_axis',(0.971399006496778,0.,0.237453090476989)) ;
#107069=DIRECTION('ref_axis',(0.237453090476989,0.,-0.971399006496778)) ;
#107070=DIRECTION('center_axis',(0.,1.,0.)) ;
#107071=DIRECTION('ref_axis',(1.,0.,0.)) ;
#107072=DIRECTION('center_axis',(-3.54829801904343E-14,1.,8.67361737988405E-15)) ;
#107073=DIRECTION('ref_axis',(1.,3.54829801904343E-14,6.83923985932746E-30)) ;
#107074=DIRECTION('center_axis',(-0.948683298050516,0.316227766016833,4.61630059016332E-15)) ;
#107075=DIRECTION('ref_axis',(0.316227766016833,0.948683298050516,2.49257808733912E-13)) ;
#107076=DIRECTION('center_axis',(0.,0.,-1.)) ;
#107077=DIRECTION('ref_axis',(1.,0.,0.)) ;
#107078=DIRECTION('center_axis',(0.,-1.,0.)) ;
#107079=DIRECTION('ref_axis',(0.,0.,1.)) ;
#107080=DIRECTION('center_axis',(0.655772517804503,-0.737744082530069,0.160299948796655)) ;
#107081=DIRECTION('ref_axis',(-0.747409318683661,-0.664363838829918,2.39955779178099E-16)) ;
#107082=DIRECTION('center_axis',(0.,1.,0.)) ;
#107083=DIRECTION('ref_axis',(0.,0.,1.)) ;
#107084=DIRECTION('center_axis',(2.73957817177508E-14,1.,0.)) ;
#107085=DIRECTION('ref_axis',(-1.,2.73957817177508E-14,0.)) ;
#107086=DIRECTION('center_axis',(0.894427190999917,0.447213595499956,0.)) ;
#107087=DIRECTION('ref_axis',(-0.447213595499956,0.894427190999917,0.)) ;
#107088=DIRECTION('center_axis',(-0.894427190999916,-0.447213595499958,
0.)) ;
#107089=DIRECTION('ref_axis',(0.447213595499958,-0.894427190999916,0.)) ;
#107090=DIRECTION('center_axis',(0.,0.,1.)) ;
#107091=DIRECTION('ref_axis',(1.,0.,0.)) ;
#107092=DIRECTION('center_axis',(0.,0.,-1.)) ;
#107093=DIRECTION('ref_axis',(-1.,0.,0.)) ;
#107094=DIRECTION('center_axis',(0.,1.,0.)) ;
#107095=DIRECTION('ref_axis',(0.,0.,1.)) ;
#107096=DIRECTION('center_axis',(0.,-1.,0.)) ;
#107097=DIRECTION('ref_axis',(0.,0.,-1.)) ;
#107098=DIRECTION('center_axis',(-0.664363838829919,0.74740931868366,0.)) ;
#107099=DIRECTION('ref_axis',(-0.74740931868366,-0.664363838829919,0.)) ;
#107100=DIRECTION('center_axis',(-0.66436383882992,0.747409318683659,2.52106651083074E-15)) ;
#107101=DIRECTION('ref_axis',(-0.747409318683659,-0.66436383882992,7.82575143531171E-30)) ;
#107102=DIRECTION('center_axis',(-0.655772517804504,0.737744082530068,-0.160299948796656)) ;
#107103=DIRECTION('ref_axis',(-0.74740931868366,-0.664363838829919,2.31673158493852E-16)) ;
#107104=DIRECTION('center_axis',(0.655772517804496,-0.737744082530075,0.160299948796656)) ;
#107105=DIRECTION('ref_axis',(0.747409318683667,0.664363838829911,-2.10122272487167E-17)) ;
#107106=DIRECTION('center_axis',(0.,1.,0.)) ;
#107107=DIRECTION('ref_axis',(1.,0.,0.)) ;
#107108=DIRECTION('center_axis',(-0.873786407766988,-0.436893203883498,
0.213592233009711)) ;
#107109=DIRECTION('ref_axis',(-0.447213595499961,0.894427190999914,5.03515095507592E-16)) ;
#107110=DIRECTION('center_axis',(-0.948683298050516,0.316227766016832,-3.59045601457216E-15)) ;
#107111=DIRECTION('ref_axis',(0.316227766016832,0.948683298050516,-1.73053540936819E-12)) ;
#107112=DIRECTION('center_axis',(0.,1.,0.)) ;
#107113=DIRECTION('ref_axis',(1.,0.,0.)) ;
#107114=DIRECTION('center_axis',(-5.47915634355017E-14,1.,0.)) ;
#107115=DIRECTION('ref_axis',(1.,5.47915634355017E-14,6.93889390390721E-14)) ;
#107116=DIRECTION('center_axis',(-0.971399006496778,0.,0.23745309047699)) ;
#107117=DIRECTION('ref_axis',(0.23745309047699,0.,0.971399006496777)) ;
#107118=DIRECTION('center_axis',(0.971399006496778,-3.69787733965917E-15,
-0.237453090476989)) ;
#107119=DIRECTION('ref_axis',(-0.237453090476989,3.58403898099287E-30,-0.971399006496778)) ;
#107120=DIRECTION('center_axis',(0.873786407766991,0.436893203883493,-0.213592233009709)) ;
#107121=DIRECTION('ref_axis',(-0.447213595499956,0.894427190999917,2.83414331365695E-16)) ;
#107122=DIRECTION('center_axis',(-0.873786407766992,-0.436893203883492,
0.21359223300971)) ;
#107123=DIRECTION('ref_axis',(0.447213595499955,-0.894427190999918,-1.48231119036019E-16)) ;
#107124=DIRECTION('center_axis',(-0.894427190999917,-0.447213595499956,
0.)) ;
#107125=DIRECTION('ref_axis',(0.447213595499956,-0.894427190999917,0.)) ;
#107126=DIRECTION('center_axis',(-0.894427190999917,-0.447213595499955,
0.)) ;
#107127=DIRECTION('ref_axis',(0.447213595499955,-0.894427190999917,0.)) ;
#107128=DIRECTION('center_axis',(0.,1.,0.)) ;
#107129=DIRECTION('ref_axis',(0.,0.,1.)) ;
#107130=DIRECTION('center_axis',(2.66122351428257E-14,1.,6.50521303491301E-15)) ;
#107131=DIRECTION('ref_axis',(-1.,2.66122351428257E-14,3.84707242087163E-30)) ;
#107132=DIRECTION('center_axis',(-0.439210132004893,-2.53225376140315E-13,
-0.898384360919225)) ;
#107133=DIRECTION('ref_axis',(0.898384360919225,-2.84946438885355E-11,-0.439210132004893)) ;
#107134=DIRECTION('center_axis',(0.,1.,0.)) ;
#107135=DIRECTION('ref_axis',(1.,0.,0.)) ;
#107136=DIRECTION('center_axis',(-0.87378640776699,-0.436893203883495,-0.213592233009712)) ;
#107137=DIRECTION('ref_axis',(-0.447213595499958,0.894427190999916,-1.950883489007E-18)) ;
#107138=DIRECTION('center_axis',(0.,0.,1.)) ;
#107139=DIRECTION('ref_axis',(1.,0.,0.)) ;
#107140=DIRECTION('center_axis',(0.439210132005014,-3.83870315422912E-13,
-0.898384360919166)) ;
#107141=DIRECTION('ref_axis',(0.898384360919166,1.69706610442857E-11,0.439210132005014)) ;
#107142=DIRECTION('center_axis',(-0.873786407766991,-0.436893203883493,
-0.213592233009709)) ;
#107143=DIRECTION('ref_axis',(0.447213595499956,-0.894427190999917,-1.06780556900622E-16)) ;
#107144=DIRECTION('center_axis',(-0.873786407766992,-0.436893203883492,
-0.213592233009707)) ;
#107145=DIRECTION('ref_axis',(0.447213595499955,-0.894427190999918,-7.04543255365314E-18)) ;
#107146=DIRECTION('center_axis',(-0.971399006496778,0.,-0.237453090476989)) ;
#107147=DIRECTION('ref_axis',(0.237453090476989,0.,-0.971399006496778)) ;
#107148=DIRECTION('center_axis',(0.971399006496778,0.,0.23745309047699)) ;
#107149=DIRECTION('ref_axis',(0.23745309047699,0.,-0.971399006496778)) ;
#107150=DIRECTION('center_axis',(1.,1.0450141421547E-16,1.7416902369245E-17)) ;
#107151=DIRECTION('ref_axis',(-1.0450141421547E-16,1.,-1.82009092883888E-33)) ;
#107152=DIRECTION('center_axis',(0.672672795323245,0.739940072189642,-7.49525355246789E-10)) ;
#107153=DIRECTION('ref_axis',(0.7380448706102,-0.670949884717819,0.0715263669084184)) ;
#107154=DIRECTION('center_axis',(-1.,0.,0.)) ;
#107155=DIRECTION('ref_axis',(0.,-0.646374896130194,-0.763019982472727)) ;
#107156=DIRECTION('center_axis',(-1.,0.,0.)) ;
#107157=DIRECTION('ref_axis',(0.,0.,1.)) ;
#107158=DIRECTION('center_axis',(-1.,0.,0.)) ;
#107159=DIRECTION('ref_axis',(0.,0.,1.)) ;
#107160=DIRECTION('center_axis',(0.,0.986393923832144,0.164398987305357)) ;
#107161=DIRECTION('ref_axis',(0.,-0.164398987305357,0.986393923832144)) ;
#107162=DIRECTION('center_axis',(0.,-0.986393923832144,-0.164398987305358)) ;
#107163=DIRECTION('ref_axis',(0.,0.164398987305358,-0.986393923832144)) ;
#107164=DIRECTION('center_axis',(0.,0.,1.)) ;
#107165=DIRECTION('ref_axis',(1.,0.,0.)) ;
#107166=DIRECTION('center_axis',(0.,0.,1.)) ;
#107167=DIRECTION('ref_axis',(1.,0.,0.)) ;
#107168=DIRECTION('center_axis',(0.,0.,1.)) ;
#107169=DIRECTION('ref_axis',(1.,0.,0.)) ;
#107170=DIRECTION('center_axis',(0.,0.,-1.)) ;
#107171=DIRECTION('ref_axis',(1.,0.,0.)) ;
#107172=DIRECTION('center_axis',(-1.,0.,0.)) ;
#107173=DIRECTION('ref_axis',(0.,-0.646374896130192,-0.763019982472729)) ;
#107174=DIRECTION('center_axis',(0.,0.,1.)) ;
#107175=DIRECTION('ref_axis',(-1.,0.,0.)) ;
#107176=DIRECTION('center_axis',(0.,0.,-1.)) ;
#107177=DIRECTION('ref_axis',(-1.,0.,0.)) ;
#107178=DIRECTION('center_axis',(1.,1.0450141421547E-16,-1.7416902369245E-17)) ;
#107179=DIRECTION('ref_axis',(-1.0450141421547E-16,1.,1.82009092883888E-33)) ;
#107180=DIRECTION('center_axis',(0.672672795323166,0.739940072189713,7.49492439365374E-10)) ;
#107181=DIRECTION('ref_axis',(0.738044870611677,-0.670949884719022,-0.0715263668818917)) ;
#107182=DIRECTION('center_axis',(1.,0.,0.)) ;
#107183=DIRECTION('ref_axis',(0.,5.20417042793045E-14,1.)) ;
#107184=DIRECTION('center_axis',(0.,0.,-1.)) ;
#107185=DIRECTION('ref_axis',(-1.,0.,0.)) ;
#107186=DIRECTION('center_axis',(0.,-0.986393923832144,0.164398987305357)) ;
#107187=DIRECTION('ref_axis',(0.,-0.164398987305357,-0.986393923832144)) ;
#107188=DIRECTION('center_axis',(1.,0.,0.)) ;
#107189=DIRECTION('ref_axis',(0.,0.,1.)) ;
#107190=DIRECTION('center_axis',(7.58941520739854E-15,0.,-1.)) ;
#107191=DIRECTION('ref_axis',(-1.,0.,-7.58941520739854E-15)) ;
#107192=DIRECTION('center_axis',(1.,0.,-8.67361737988404E-15)) ;
#107193=DIRECTION('ref_axis',(-8.67361737988404E-15,0.,-1.)) ;
#107194=DIRECTION('center_axis',(1.,0.,0.)) ;
#107195=DIRECTION('ref_axis',(0.,0.,-1.)) ;
#107196=DIRECTION('center_axis',(1.,0.,8.67361737988403E-15)) ;
#107197=DIRECTION('ref_axis',(8.67361737988403E-15,0.,-1.)) ;
#107198=DIRECTION('center_axis',(0.,0.,1.)) ;
#107199=DIRECTION('ref_axis',(1.,0.,0.)) ;
#107200=DIRECTION('center_axis',(0.,0.,-1.)) ;
#107201=DIRECTION('ref_axis',(-1.,0.,0.)) ;
#107202=DIRECTION('center_axis',(1.,0.,0.)) ;
#107203=DIRECTION('ref_axis',(0.,0.,1.)) ;
#107204=DIRECTION('center_axis',(-6.50521303491304E-15,0.,-1.)) ;
#107205=DIRECTION('ref_axis',(-1.,0.,6.50521303491304E-15)) ;
#107206=DIRECTION('center_axis',(1.,0.,0.)) ;
#107207=DIRECTION('ref_axis',(0.,0.,1.)) ;
#107208=DIRECTION('center_axis',(1.,9.40395480657835E-30,8.67361737988403E-15)) ;
#107209=DIRECTION('ref_axis',(8.67361737988403E-15,-5.27711695562625E-58,
-1.)) ;
#107210=DIRECTION('center_axis',(0.,0.,-1.)) ;
#107211=DIRECTION('ref_axis',(-1.,0.,0.)) ;
#107212=DIRECTION('center_axis',(6.50521303491304E-15,0.,-1.)) ;
#107213=DIRECTION('ref_axis',(-1.,0.,-6.50521303491304E-15)) ;
#107214=DIRECTION('center_axis',(-1.,0.,0.)) ;
#107215=DIRECTION('ref_axis',(0.,0.,1.)) ;
#107216=DIRECTION('center_axis',(1.,-8.67361737988409E-15,0.)) ;
#107217=DIRECTION('ref_axis',(8.67361737988409E-15,1.,0.)) ;
#107218=DIRECTION('center_axis',(1.,0.,0.)) ;
#107219=DIRECTION('ref_axis',(0.,0.,1.)) ;
#107220=DIRECTION('center_axis',(-4.33680868994202E-16,0.,1.)) ;
#107221=DIRECTION('ref_axis',(1.,0.,4.33680868994202E-16)) ;
#107222=DIRECTION('center_axis',(0.,0.,-1.)) ;
#107223=DIRECTION('ref_axis',(-1.,0.,0.)) ;
#107224=DIRECTION('center_axis',(0.,0.,1.)) ;
#107225=DIRECTION('ref_axis',(1.,0.,0.)) ;
#107226=DIRECTION('center_axis',(0.,1.,0.)) ;
#107227=DIRECTION('ref_axis',(0.,0.,1.)) ;
#107228=DIRECTION('center_axis',(-1.,0.,0.)) ;
#107229=DIRECTION('ref_axis',(0.,0.,-1.)) ;
#107230=DIRECTION('center_axis',(0.,-1.,0.)) ;
#107231=DIRECTION('ref_axis',(0.,0.,1.)) ;
#107232=DIRECTION('center_axis',(0.,1.,0.)) ;
#107233=DIRECTION('ref_axis',(0.,0.,1.)) ;
#107234=DIRECTION('center_axis',(0.,-1.,0.)) ;
#107235=DIRECTION('ref_axis',(0.,0.,1.)) ;
#107236=DIRECTION('center_axis',(-1.,0.,0.)) ;
#107237=DIRECTION('ref_axis',(0.,0.,-1.)) ;
#107238=DIRECTION('center_axis',(-1.,0.,-1.73472347597681E-16)) ;
#107239=DIRECTION('ref_axis',(-1.73472347597681E-16,0.,1.)) ;
#107240=DIRECTION('center_axis',(-1.,0.,0.)) ;
#107241=DIRECTION('ref_axis',(0.,0.,1.)) ;
#107242=DIRECTION('center_axis',(0.,1.,0.)) ;
#107243=DIRECTION('ref_axis',(0.,0.,1.)) ;
#107244=DIRECTION('center_axis',(0.,-1.,0.)) ;
#107245=DIRECTION('ref_axis',(0.,0.,-1.)) ;
#107246=DIRECTION('center_axis',(-4.33680868994202E-16,0.,1.)) ;
#107247=DIRECTION('ref_axis',(1.,0.,4.33680868994202E-16)) ;
#107248=DIRECTION('center_axis',(0.,0.,1.)) ;
#107249=DIRECTION('ref_axis',(1.,0.,0.)) ;
#107250=DIRECTION('center_axis',(0.,0.,-1.)) ;
#107251=DIRECTION('ref_axis',(-1.,0.,0.)) ;
#107252=DIRECTION('center_axis',(0.,1.,0.)) ;
#107253=DIRECTION('ref_axis',(0.,0.,1.)) ;
#107254=DIRECTION('center_axis',(0.,-1.,0.)) ;
#107255=DIRECTION('ref_axis',(0.,0.,-1.)) ;
#107256=DIRECTION('center_axis',(1.,0.,-1.73472347597681E-16)) ;
#107257=DIRECTION('ref_axis',(-1.73472347597681E-16,0.,-1.)) ;
#107258=DIRECTION('center_axis',(-1.,0.,0.)) ;
#107259=DIRECTION('ref_axis',(0.,0.,1.)) ;
#107260=DIRECTION('center_axis',(0.,0.,-1.)) ;
#107261=DIRECTION('ref_axis',(-1.,0.,0.)) ;
#107262=DIRECTION('center_axis',(0.,0.,1.)) ;
#107263=DIRECTION('ref_axis',(1.,0.,0.)) ;
#107264=DIRECTION('center_axis',(0.,0.,-1.)) ;
#107265=DIRECTION('ref_axis',(-1.,0.,0.)) ;
#107266=DIRECTION('center_axis',(0.,1.,0.)) ;
#107267=DIRECTION('ref_axis',(0.,0.,1.)) ;
#107268=DIRECTION('center_axis',(0.,-1.,0.)) ;
#107269=DIRECTION('ref_axis',(0.,0.,1.)) ;
#107270=DIRECTION('center_axis',(0.,1.,0.)) ;
#107271=DIRECTION('ref_axis',(1.,0.,0.)) ;
#107272=DIRECTION('center_axis',(1.,0.,0.)) ;
#107273=DIRECTION('ref_axis',(0.,0.,1.)) ;
#107274=DIRECTION('center_axis',(0.,1.,0.)) ;
#107275=DIRECTION('ref_axis',(1.,0.,0.)) ;
#107276=DIRECTION('center_axis',(1.,0.,0.)) ;
#107277=DIRECTION('ref_axis',(0.,0.,1.)) ;
#107278=DIRECTION('center_axis',(0.,1.,0.)) ;
#107279=DIRECTION('ref_axis',(0.,0.,1.)) ;
#107280=DIRECTION('center_axis',(0.,-1.,0.)) ;
#107281=DIRECTION('ref_axis',(0.,0.,1.)) ;
#107282=DIRECTION('center_axis',(0.,1.,0.)) ;
#107283=DIRECTION('ref_axis',(0.,0.,1.)) ;
#107284=DIRECTION('center_axis',(0.,-1.,0.)) ;
#107285=DIRECTION('ref_axis',(0.,0.,-1.)) ;
#107286=DIRECTION('center_axis',(-1.,0.,-1.73472347597681E-16)) ;
#107287=DIRECTION('ref_axis',(-1.73472347597681E-16,0.,1.)) ;
#107288=DIRECTION('center_axis',(1.,0.,0.)) ;
#107289=DIRECTION('ref_axis',(0.,0.,-1.)) ;
#107290=DIRECTION('center_axis',(1.,0.,-1.73472347597681E-16)) ;
#107291=DIRECTION('ref_axis',(-1.73472347597681E-16,0.,-1.)) ;
#107292=DIRECTION('center_axis',(1.,0.,0.)) ;
#107293=DIRECTION('ref_axis',(0.,0.,-1.)) ;
#107294=DIRECTION('center_axis',(0.,1.,0.)) ;
#107295=DIRECTION('ref_axis',(0.,0.,1.)) ;
#107296=DIRECTION('center_axis',(0.,-1.,0.)) ;
#107297=DIRECTION('ref_axis',(0.,0.,-1.)) ;
#107298=DIRECTION('center_axis',(0.,1.,0.)) ;
#107299=DIRECTION('ref_axis',(1.,0.,0.)) ;
#107300=DIRECTION('center_axis',(0.,0.,1.)) ;
#107301=DIRECTION('ref_axis',(-1.,0.,0.)) ;
#107302=DIRECTION('center_axis',(0.,1.,0.)) ;
#107303=DIRECTION('ref_axis',(1.,0.,0.)) ;
#107304=DIRECTION('center_axis',(0.,0.,-1.)) ;
#107305=DIRECTION('ref_axis',(1.,0.,0.)) ;
#107306=DIRECTION('center_axis',(0.,0.,-1.)) ;
#107307=DIRECTION('ref_axis',(-1.,0.,0.)) ;
#107308=DIRECTION('center_axis',(2.16840434497101E-16,0.,1.)) ;
#107309=DIRECTION('ref_axis',(1.,0.,-2.16840434497101E-16)) ;
#107310=DIRECTION('center_axis',(0.,0.,-1.)) ;
#107311=DIRECTION('ref_axis',(-1.,0.,0.)) ;
#107312=DIRECTION('center_axis',(0.,0.,1.)) ;
#107313=DIRECTION('ref_axis',(1.,0.,0.)) ;
#107314=DIRECTION('center_axis',(0.,-1.,0.)) ;
#107315=DIRECTION('ref_axis',(0.,0.,-1.)) ;
#107316=DIRECTION('center_axis',(1.,0.,0.)) ;
#107317=DIRECTION('ref_axis',(0.,0.,1.)) ;
#107318=DIRECTION('center_axis',(0.,1.,0.)) ;
#107319=DIRECTION('ref_axis',(0.,0.,-1.)) ;
#107320=DIRECTION('center_axis',(0.,-1.,0.)) ;
#107321=DIRECTION('ref_axis',(0.,0.,-1.)) ;
#107322=DIRECTION('center_axis',(0.,1.,0.)) ;
#107323=DIRECTION('ref_axis',(0.,0.,-1.)) ;
#107324=DIRECTION('center_axis',(1.,0.,0.)) ;
#107325=DIRECTION('ref_axis',(0.,0.,1.)) ;
#107326=DIRECTION('center_axis',(1.,0.,-1.73472347597681E-16)) ;
#107327=DIRECTION('ref_axis',(-1.73472347597681E-16,0.,-1.)) ;
#107328=DIRECTION('center_axis',(1.,0.,0.)) ;
#107329=DIRECTION('ref_axis',(0.,0.,-1.)) ;
#107330=DIRECTION('center_axis',(0.,-1.,0.)) ;
#107331=DIRECTION('ref_axis',(0.,0.,-1.)) ;
#107332=DIRECTION('center_axis',(0.,1.,0.)) ;
#107333=DIRECTION('ref_axis',(0.,0.,1.)) ;
#107334=DIRECTION('center_axis',(2.16840434497101E-16,0.,1.)) ;
#107335=DIRECTION('ref_axis',(1.,0.,-2.16840434497101E-16)) ;
#107336=DIRECTION('center_axis',(0.,0.,1.)) ;
#107337=DIRECTION('ref_axis',(1.,0.,0.)) ;
#107338=DIRECTION('center_axis',(0.,0.,-1.)) ;
#107339=DIRECTION('ref_axis',(-1.,0.,0.)) ;
#107340=DIRECTION('center_axis',(0.,-1.,0.)) ;
#107341=DIRECTION('ref_axis',(0.,0.,-1.)) ;
#107342=DIRECTION('center_axis',(0.,1.,0.)) ;
#107343=DIRECTION('ref_axis',(0.,0.,1.)) ;
#107344=DIRECTION('center_axis',(-1.,0.,1.73472347597681E-16)) ;
#107345=DIRECTION('ref_axis',(1.73472347597681E-16,0.,1.)) ;
#107346=DIRECTION('center_axis',(1.,0.,0.)) ;
#107347=DIRECTION('ref_axis',(0.,0.,-1.)) ;
#107348=DIRECTION('center_axis',(-2.16840434497101E-16,0.,-1.)) ;
#107349=DIRECTION('ref_axis',(-1.,0.,2.16840434497101E-16)) ;
#107350=DIRECTION('center_axis',(0.,0.,1.)) ;
#107351=DIRECTION('ref_axis',(1.,0.,0.)) ;
#107352=DIRECTION('center_axis',(0.,0.,-1.)) ;
#107353=DIRECTION('ref_axis',(-1.,0.,0.)) ;
#107354=DIRECTION('center_axis',(0.,-1.,0.)) ;
#107355=DIRECTION('ref_axis',(0.,0.,-1.)) ;
#107356=DIRECTION('center_axis',(0.,1.,0.)) ;
#107357=DIRECTION('ref_axis',(0.,0.,-1.)) ;
#107358=DIRECTION('center_axis',(0.,1.,0.)) ;
#107359=DIRECTION('ref_axis',(1.,0.,0.)) ;
#107360=DIRECTION('center_axis',(-1.,0.,0.)) ;
#107361=DIRECTION('ref_axis',(0.,0.,-1.)) ;
#107362=DIRECTION('center_axis',(0.,1.,0.)) ;
#107363=DIRECTION('ref_axis',(1.,0.,0.)) ;
#107364=DIRECTION('center_axis',(-1.,0.,0.)) ;
#107365=DIRECTION('ref_axis',(0.,0.,-1.)) ;
#107366=DIRECTION('center_axis',(0.,-1.,0.)) ;
#107367=DIRECTION('ref_axis',(0.,0.,-1.)) ;
#107368=DIRECTION('center_axis',(0.,1.,0.)) ;
#107369=DIRECTION('ref_axis',(0.,0.,-1.)) ;
#107370=DIRECTION('center_axis',(0.,-1.,0.)) ;
#107371=DIRECTION('ref_axis',(0.,0.,-1.)) ;
#107372=DIRECTION('center_axis',(0.,1.,0.)) ;
#107373=DIRECTION('ref_axis',(0.,0.,1.)) ;
#107374=DIRECTION('center_axis',(1.,0.,-1.73472347597681E-16)) ;
#107375=DIRECTION('ref_axis',(-1.73472347597681E-16,0.,-1.)) ;
#107376=DIRECTION('center_axis',(-1.,0.,0.)) ;
#107377=DIRECTION('ref_axis',(0.,0.,1.)) ;
#107378=DIRECTION('center_axis',(-1.,0.,1.73472347597681E-16)) ;
#107379=DIRECTION('ref_axis',(1.73472347597681E-16,0.,1.)) ;
#107380=DIRECTION('center_axis',(-1.,0.,0.)) ;
#107381=DIRECTION('ref_axis',(0.,0.,1.)) ;
#107382=DIRECTION('center_axis',(0.,-1.,0.)) ;
#107383=DIRECTION('ref_axis',(0.,0.,-1.)) ;
#107384=DIRECTION('center_axis',(0.,1.,0.)) ;
#107385=DIRECTION('ref_axis',(0.,0.,1.)) ;
#107386=DIRECTION('center_axis',(0.,1.,0.)) ;
#107387=DIRECTION('ref_axis',(1.,0.,0.)) ;
#107388=DIRECTION('center_axis',(0.,0.,1.)) ;
#107389=DIRECTION('ref_axis',(-1.,0.,0.)) ;
#107390=DIRECTION('center_axis',(0.,1.,0.)) ;
#107391=DIRECTION('ref_axis',(1.,0.,0.)) ;
#107392=DIRECTION('center_axis',(0.,0.,-1.)) ;
#107393=DIRECTION('ref_axis',(1.,0.,0.)) ;
#107394=DIRECTION('center_axis',(-2.16840434497101E-16,0.,-1.)) ;
#107395=DIRECTION('ref_axis',(-1.,0.,2.16840434497101E-16)) ;
#107396=DIRECTION('center_axis',(-1.,0.,0.)) ;
#107397=DIRECTION('ref_axis',(0.,0.,1.)) ;
#107398=DIRECTION('center_axis',(0.,-0.632948931301575,-0.774193548387091)) ;
#107399=DIRECTION('ref_axis',(0.,0.774193548387091,-0.632948931301575)) ;
#107400=DIRECTION('center_axis',(0.,0.,1.)) ;
#107401=DIRECTION('ref_axis',(1.,0.,0.)) ;
#107402=DIRECTION('center_axis',(8.67361737988401E-15,0.,1.)) ;
#107403=DIRECTION('ref_axis',(1.,0.,-8.67361737988401E-15)) ;
#107404=DIRECTION('center_axis',(0.,1.,0.)) ;
#107405=DIRECTION('ref_axis',(1.,0.,0.)) ;
#107406=DIRECTION('center_axis',(-1.,0.,0.)) ;
#107407=DIRECTION('ref_axis',(0.,4.33680868994204E-15,-1.)) ;
#107408=DIRECTION('center_axis',(1.,0.,0.)) ;
#107409=DIRECTION('ref_axis',(0.,0.,-1.)) ;
#107410=DIRECTION('center_axis',(-1.,0.,0.)) ;
#107411=DIRECTION('ref_axis',(0.,0.,1.)) ;
#107412=DIRECTION('center_axis',(0.,0.,-1.)) ;
#107413=DIRECTION('ref_axis',(-1.,0.,0.)) ;
#107414=DIRECTION('center_axis',(0.,0.,-1.)) ;
#107415=DIRECTION('ref_axis',(-1.,0.,0.)) ;
#107416=DIRECTION('center_axis',(-1.,0.,0.)) ;
#107417=DIRECTION('ref_axis',(0.,0.,1.)) ;
#107418=DIRECTION('center_axis',(0.,-0.632948931301567,-0.774193548387097)) ;
#107419=DIRECTION('ref_axis',(0.,-0.774193548387097,0.632948931301567)) ;
#107420=DIRECTION('center_axis',(-1.,0.,0.)) ;
#107421=DIRECTION('ref_axis',(0.,0.,1.)) ;
#107422=DIRECTION('center_axis',(0.,0.632948931301567,-0.774193548387097)) ;
#107423=DIRECTION('ref_axis',(0.,0.774193548387097,0.632948931301567)) ;
#107424=DIRECTION('center_axis',(-1.,0.,0.)) ;
#107425=DIRECTION('ref_axis',(0.,0.,1.)) ;
#107426=DIRECTION('center_axis',(1.,0.,0.)) ;
#107427=DIRECTION('ref_axis',(0.,5.20417042793045E-14,1.)) ;
#107428=DIRECTION('center_axis',(1.,0.,0.)) ;
#107429=DIRECTION('ref_axis',(0.,0.,-1.)) ;
#107430=DIRECTION('center_axis',(1.,0.,0.)) ;
#107431=DIRECTION('ref_axis',(0.,0.,-1.)) ;
#107432=DIRECTION('center_axis',(0.,1.,0.)) ;
#107433=DIRECTION('ref_axis',(1.,0.,0.)) ;
#107434=DIRECTION('center_axis',(1.22050154678007E-14,0.632948931301567,
-0.774193548387097)) ;
#107435=DIRECTION('ref_axis',(1.73472347597684E-14,-0.774193548387097,-0.632948931301567)) ;
#107436=DIRECTION('center_axis',(-1.,0.,0.)) ;
#107437=DIRECTION('ref_axis',(0.,0.,1.)) ;
#107438=DIRECTION('center_axis',(-0.422618261740697,0.,0.906307787036651)) ;
#107439=DIRECTION('ref_axis',(0.906307787036651,0.,0.422618261740697)) ;
#107440=DIRECTION('center_axis',(0.422618261740697,0.,-0.906307787036651)) ;
#107441=DIRECTION('ref_axis',(-0.906307787036651,0.,-0.422618261740697)) ;
#107442=DIRECTION('center_axis',(0.422618261740697,0.,-0.906307787036651)) ;
#107443=DIRECTION('ref_axis',(-0.906307787036651,0.,-0.422618261740697)) ;
#107444=DIRECTION('center_axis',(-0.422618261740697,0.,0.906307787036651)) ;
#107445=DIRECTION('ref_axis',(0.906307787036651,0.,0.422618261740697)) ;
#107446=DIRECTION('center_axis',(0.,1.,0.)) ;
#107447=DIRECTION('ref_axis',(1.,0.,0.)) ;
#107448=DIRECTION('center_axis',(0.,-0.986393923832144,0.164398987305358)) ;
#107449=DIRECTION('ref_axis',(0.,-0.164398987305358,-0.986393923832144)) ;
#107450=DIRECTION('center_axis',(0.,0.986393923832144,-0.164398987305357)) ;
#107451=DIRECTION('ref_axis',(0.,0.164398987305357,0.986393923832144)) ;
#107452=DIRECTION('center_axis',(0.,-0.986393923832144,0.164398987305358)) ;
#107453=DIRECTION('ref_axis',(0.,-0.164398987305358,-0.986393923832144)) ;
#107454=DIRECTION('center_axis',(-1.,0.,0.)) ;
#107455=DIRECTION('ref_axis',(0.,0.107567764393758,-0.994197755008192)) ;
#107456=DIRECTION('center_axis',(4.02631181035923E-15,-0.928404294083138,
-0.371571617226061)) ;
#107457=DIRECTION('ref_axis',(1.27444840229953E-29,0.371571617226061,-0.928404294083138)) ;
#107458=DIRECTION('center_axis',(0.275516865537137,-0.50093975551097,-0.820457078800105)) ;
#107459=DIRECTION('ref_axis',(3.47276585739718E-16,0.853490367006418,-0.521108619605597)) ;
#107460=DIRECTION('center_axis',(0.,0.,-1.)) ;
#107461=DIRECTION('ref_axis',(-1.,0.,0.)) ;
#107462=DIRECTION('center_axis',(0.,0.,-1.)) ;
#107463=DIRECTION('ref_axis',(-1.,0.,0.)) ;
#107464=DIRECTION('center_axis',(-0.275516865538071,0.500939755523742,-0.820457078791993)) ;
#107465=DIRECTION('ref_axis',(1.34532370065023E-15,0.853490366998217,0.521108619619028)) ;
#107466=DIRECTION('center_axis',(0.,-0.986393923832144,-0.164398987305357)) ;
#107467=DIRECTION('ref_axis',(0.,0.164398987305357,-0.986393923832144)) ;
#107468=DIRECTION('center_axis',(3.5648347838177E-16,0.986393923832144,
0.164398987305358)) ;
#107469=DIRECTION('ref_axis',(3.79675591822878E-31,-0.164398987305358,0.986393923832144)) ;
#107470=DIRECTION('center_axis',(0.,1.,0.)) ;
#107471=DIRECTION('ref_axis',(1.,0.,0.)) ;
#107472=DIRECTION('center_axis',(-1.,0.,0.)) ;
#107473=DIRECTION('ref_axis',(0.,0.,1.)) ;
#107474=DIRECTION('center_axis',(0.,0.,-1.)) ;
#107475=DIRECTION('ref_axis',(-1.,0.,0.)) ;
#107476=DIRECTION('center_axis',(0.,0.,-1.)) ;
#107477=DIRECTION('ref_axis',(-1.,0.,0.)) ;
#107478=DIRECTION('center_axis',(0.795723237447208,-7.53302716311723E-12,
0.605660407643206)) ;
#107479=DIRECTION('ref_axis',(0.605660407643206,2.00215687134887E-26,-0.795723237447208)) ;
#107480=DIRECTION('center_axis',(1.57772181044204E-26,2.36658271566302E-26,
1.)) ;
#107481=DIRECTION('ref_axis',(3.73380916671669E-52,-1.,2.36658271566302E-26)) ;
#107482=DIRECTION('center_axis',(-0.795723237415222,-2.11663082418553E-11,
0.605660407685229)) ;
#107483=DIRECTION('ref_axis',(0.605660407685229,1.1913710773826E-25,0.795723237415222)) ;
#107484=DIRECTION('center_axis',(0.,1.,0.)) ;
#107485=DIRECTION('ref_axis',(1.,0.,0.)) ;
#107486=DIRECTION('center_axis',(-0.716468671818951,0.697619267438901,0.)) ;
#107487=DIRECTION('ref_axis',(-0.697619267438901,-0.716468671818951,0.)) ;
#107488=DIRECTION('center_axis',(0.,-1.,0.)) ;
#107489=DIRECTION('ref_axis',(0.,0.,-1.)) ;
#107490=DIRECTION('center_axis',(0.,1.,0.)) ;
#107491=DIRECTION('ref_axis',(1.,0.,0.)) ;
#107492=DIRECTION('center_axis',(0.,-1.,0.)) ;
#107493=DIRECTION('ref_axis',(0.,0.,-1.)) ;
#107494=DIRECTION('center_axis',(-0.716468671818951,0.697619267438901,0.)) ;
#107495=DIRECTION('ref_axis',(-0.697619267438901,-0.716468671818951,0.)) ;
#107496=DIRECTION('center_axis',(0.,-1.,0.)) ;
#107497=DIRECTION('ref_axis',(0.,0.,-1.)) ;
#107498=DIRECTION('center_axis',(0.,-1.,0.)) ;
#107499=DIRECTION('ref_axis',(0.,0.,-1.)) ;
#107500=DIRECTION('center_axis',(0.716468671818953,-0.697619267438899,0.)) ;
#107501=DIRECTION('ref_axis',(0.697619267438899,0.716468671818953,0.)) ;
#107502=DIRECTION('center_axis',(-0.716468671818955,0.697619267438896,0.)) ;
#107503=DIRECTION('ref_axis',(-0.697619267438896,-0.716468671818955,0.)) ;
#107504=DIRECTION('center_axis',(-0.716468671818953,0.697619267438899,0.)) ;
#107505=DIRECTION('ref_axis',(-0.697619267438899,-0.716468671818953,0.)) ;
#107506=DIRECTION('center_axis',(-0.716468671818955,0.697619267438896,0.)) ;
#107507=DIRECTION('ref_axis',(-0.697619267438896,-0.716468671818955,0.)) ;
#107508=DIRECTION('center_axis',(0.,1.,0.)) ;
#107509=DIRECTION('ref_axis',(0.,0.,1.)) ;
#107510=DIRECTION('center_axis',(0.,-1.,0.)) ;
#107511=DIRECTION('ref_axis',(0.,0.,-1.)) ;
#107512=DIRECTION('center_axis',(0.,0.,1.)) ;
#107513=DIRECTION('ref_axis',(1.,0.,0.)) ;
#107514=DIRECTION('center_axis',(-0.891049746169499,0.453905661840951,0.)) ;
#107515=DIRECTION('ref_axis',(-0.453905661840951,-0.891049746169499,0.)) ;
#107516=DIRECTION('center_axis',(0.,1.,0.)) ;
#107517=DIRECTION('ref_axis',(1.,0.,0.)) ;
#107518=DIRECTION('center_axis',(-0.989044367093028,0.147618562252689,-1.28038692714843E-15)) ;
#107519=DIRECTION('ref_axis',(-0.147618562252689,-0.989044367093028,4.74381411340675E-32)) ;
#107520=DIRECTION('center_axis',(0.,1.,0.)) ;
#107521=DIRECTION('ref_axis',(1.,0.,0.)) ;
#107522=DIRECTION('center_axis',(-0.989044367093028,0.147618562252688,0.)) ;
#107523=DIRECTION('ref_axis',(-0.147618562252688,-0.989044367093028,0.)) ;
#107524=DIRECTION('center_axis',(0.,0.,1.)) ;
#107525=DIRECTION('ref_axis',(1.,0.,0.)) ;
#107526=DIRECTION('center_axis',(-0.891049746169497,0.453905661840955,-3.93700403737149E-15)) ;
#107527=DIRECTION('ref_axis',(-0.453905661840955,-0.891049746169497,6.00336752605965E-33)) ;
#107528=DIRECTION('center_axis',(-0.891049746169503,0.453905661840943,0.)) ;
#107529=DIRECTION('ref_axis',(-0.453905661840943,-0.891049746169503,0.)) ;
#107530=DIRECTION('center_axis',(-0.891049746169501,0.453905661840946,0.)) ;
#107531=DIRECTION('ref_axis',(-0.453905661840946,-0.891049746169501,0.)) ;
#107532=DIRECTION('center_axis',(0.989044367093028,-0.147618562252691,0.)) ;
#107533=DIRECTION('ref_axis',(0.147618562252691,0.989044367093028,0.)) ;
#107534=DIRECTION('center_axis',(0.,0.,1.)) ;
#107535=DIRECTION('ref_axis',(1.,0.,0.)) ;
#107536=DIRECTION('center_axis',(0.,0.,-1.)) ;
#107537=DIRECTION('ref_axis',(-1.,0.,0.)) ;
#107538=DIRECTION('center_axis',(0.,0.,1.)) ;
#107539=DIRECTION('ref_axis',(1.,0.,0.)) ;
#107540=DIRECTION('center_axis',(-0.989044367093028,0.147618562252691,0.)) ;
#107541=DIRECTION('ref_axis',(-0.147618562252691,-0.989044367093028,0.)) ;
#107542=DIRECTION('center_axis',(0.891049746169503,-0.453905661840943,0.)) ;
#107543=DIRECTION('ref_axis',(0.453905661840943,0.891049746169503,0.)) ;
#107544=DIRECTION('center_axis',(-0.891049746169501,0.453905661840946,0.)) ;
#107545=DIRECTION('ref_axis',(-0.453905661840946,-0.891049746169501,0.)) ;
#107546=DIRECTION('center_axis',(0.,0.,1.)) ;
#107547=DIRECTION('ref_axis',(1.,0.,0.)) ;
#107548=DIRECTION('center_axis',(-1.,0.,0.)) ;
#107549=DIRECTION('ref_axis',(0.,0.,1.)) ;
#107550=DIRECTION('center_axis',(0.,1.,0.)) ;
#107551=DIRECTION('ref_axis',(0.,0.,-1.)) ;
#107552=DIRECTION('center_axis',(0.,1.,0.)) ;
#107553=DIRECTION('ref_axis',(0.,0.,-1.)) ;
#107554=DIRECTION('center_axis',(0.,0.,1.)) ;
#107555=DIRECTION('ref_axis',(1.,0.,0.)) ;
#107556=DIRECTION('center_axis',(-1.,0.,0.)) ;
#107557=DIRECTION('ref_axis',(0.,0.,1.)) ;
#107558=DIRECTION('center_axis',(-1.,2.60782465076463E-16,0.)) ;
#107559=DIRECTION('ref_axis',(-2.60782465076463E-16,-1.,0.)) ;
#107560=DIRECTION('center_axis',(-1.,0.,0.)) ;
#107561=DIRECTION('ref_axis',(0.,0.,1.)) ;
#107562=DIRECTION('center_axis',(0.,1.,0.)) ;
#107563=DIRECTION('ref_axis',(0.,0.,1.)) ;
#107564=DIRECTION('center_axis',(0.,1.,0.)) ;
#107565=DIRECTION('ref_axis',(0.,0.,1.)) ;
#107566=DIRECTION('center_axis',(0.,-1.,0.)) ;
#107567=DIRECTION('ref_axis',(0.,0.,-1.)) ;
#107568=DIRECTION('center_axis',(0.,1.,0.)) ;
#107569=DIRECTION('ref_axis',(0.,0.,1.)) ;
#107570=DIRECTION('center_axis',(1.,-2.60782465076463E-16,0.)) ;
#107571=DIRECTION('ref_axis',(2.60782465076463E-16,1.,0.)) ;
#107572=DIRECTION('center_axis',(-1.,0.,0.)) ;
#107573=DIRECTION('ref_axis',(0.,0.,1.)) ;
#107574=DIRECTION('center_axis',(-1.,0.,0.)) ;
#107575=DIRECTION('ref_axis',(0.,0.,1.)) ;
#107576=DIRECTION('center_axis',(0.,0.,-1.)) ;
#107577=DIRECTION('ref_axis',(1.,0.,0.)) ;
#107578=DIRECTION('center_axis',(-1.,0.,0.)) ;
#107579=DIRECTION('ref_axis',(0.,0.,1.)) ;
#107580=DIRECTION('center_axis',(0.,0.,1.)) ;
#107581=DIRECTION('ref_axis',(-1.,0.,0.)) ;
#107582=DIRECTION('center_axis',(0.,0.,1.)) ;
#107583=DIRECTION('ref_axis',(1.,0.,0.)) ;
#107584=DIRECTION('center_axis',(-1.,0.,0.)) ;
#107585=DIRECTION('ref_axis',(0.,0.,1.)) ;
#107586=DIRECTION('center_axis',(-1.,0.,0.)) ;
#107587=DIRECTION('ref_axis',(0.,0.,1.)) ;
#107588=DIRECTION('center_axis',(-3.56483478381767E-16,0.986393923832144,
0.164398987305358)) ;
#107589=DIRECTION('ref_axis',(-3.72967278346455E-31,-0.164398987305358,
0.986393923832144)) ;
#107590=DIRECTION('center_axis',(1.,0.,0.)) ;
#107591=DIRECTION('ref_axis',(0.,1.38777878078145E-13,1.)) ;
#107592=DIRECTION('center_axis',(-4.02631181035926E-15,0.928404294083138,
-0.371571617226061)) ;
#107593=DIRECTION('ref_axis',(1.27405345096899E-29,0.371571617226061,0.928404294083138)) ;
#107594=DIRECTION('center_axis',(0.,0.,1.)) ;
#107595=DIRECTION('ref_axis',(1.,0.,0.)) ;
#107596=DIRECTION('center_axis',(0.,0.,1.)) ;
#107597=DIRECTION('ref_axis',(1.,0.,0.)) ;
#107598=DIRECTION('',(0.,0.,-1.)) ;
#107599=DIRECTION('center_axis',(0.,0.,-1.)) ;
#107600=DIRECTION('ref_axis',(1.,0.,0.)) ;
#107601=DIRECTION('',(0.,0.,1.)) ;
#107602=DIRECTION('center_axis',(0.,-1.,0.)) ;
#107603=DIRECTION('ref_axis',(0.,0.,-1.)) ;
#107604=DIRECTION('center_axis',(0.,-1.,0.)) ;
#107605=DIRECTION('ref_axis',(0.,0.,-1.)) ;
#107606=DIRECTION('center_axis',(-1.,0.,-1.22464679914735E-16)) ;
#107607=DIRECTION('ref_axis',(-1.22464679914735E-16,0.,1.)) ;
#107608=DIRECTION('center_axis',(0.,1.,0.)) ;
#107609=DIRECTION('ref_axis',(0.,0.,-1.)) ;
#107610=DIRECTION('center_axis',(0.,1.,0.)) ;
#107611=DIRECTION('ref_axis',(0.,0.,-1.)) ;
#107612=DIRECTION('center_axis',(1.,0.,0.)) ;
#107613=DIRECTION('ref_axis',(0.,0.,-1.)) ;
#107614=DIRECTION('center_axis',(1.,0.,0.)) ;
#107615=DIRECTION('ref_axis',(0.,0.,-1.)) ;
#107616=DIRECTION('center_axis',(0.,1.,1.22464679914735E-16)) ;
#107617=DIRECTION('ref_axis',(0.,-1.22464679914735E-16,1.)) ;
#107618=DIRECTION('center_axis',(-1.,0.,0.)) ;
#107619=DIRECTION('ref_axis',(0.,0.,-1.)) ;
#107620=DIRECTION('center_axis',(-1.,0.,0.)) ;
#107621=DIRECTION('ref_axis',(0.,0.,1.)) ;
#107622=DIRECTION('center_axis',(-1.,0.,0.)) ;
#107623=DIRECTION('ref_axis',(0.,0.,1.)) ;
#107624=DIRECTION('center_axis',(0.,-1.,1.22464679914735E-16)) ;
#107625=DIRECTION('ref_axis',(0.,-1.22464679914735E-16,-1.)) ;
#107626=DIRECTION('center_axis',(1.,0.,0.)) ;
#107627=DIRECTION('ref_axis',(0.,0.,1.)) ;
#107628=DIRECTION('center_axis',(1.,0.,0.)) ;
#107629=DIRECTION('ref_axis',(0.,0.,1.)) ;
#107630=DIRECTION('center_axis',(-1.,0.,0.)) ;
#107631=DIRECTION('ref_axis',(0.,0.,1.)) ;
#107632=DIRECTION('center_axis',(-1.,0.,0.)) ;
#107633=DIRECTION('ref_axis',(0.,0.,1.)) ;
#107634=DIRECTION('center_axis',(0.,0.986393923832144,-0.164398987305358)) ;
#107635=DIRECTION('ref_axis',(0.,-0.164398987305358,-0.986393923832144)) ;
#107636=DIRECTION('center_axis',(1.,0.,0.)) ;
#107637=DIRECTION('ref_axis',(0.,0.,1.)) ;
#107638=DIRECTION('center_axis',(0.,0.,1.)) ;
#107639=DIRECTION('ref_axis',(1.,0.,0.)) ;
#107640=DIRECTION('center_axis',(0.,1.,0.)) ;
#107641=DIRECTION('ref_axis',(1.,0.,0.)) ;
#107642=DIRECTION('center_axis',(1.,0.,0.)) ;
#107643=DIRECTION('ref_axis',(0.,0.,-1.)) ;
#107644=DIRECTION('center_axis',(0.,0.,-1.)) ;
#107645=DIRECTION('ref_axis',(-1.,0.,0.)) ;
#107646=DIRECTION('center_axis',(0.,-0.986393923832144,0.164398987305358)) ;
#107647=DIRECTION('ref_axis',(0.,0.164398987305358,0.986393923832144)) ;
#107648=DIRECTION('center_axis',(-1.,0.,0.)) ;
#107649=DIRECTION('ref_axis',(0.,0.,1.)) ;
#107650=DIRECTION('',(1.,0.,0.)) ;
#107651=DIRECTION('center_axis',(-1.,0.,0.)) ;
#107652=DIRECTION('ref_axis',(0.,0.,1.)) ;
#107653=DIRECTION('',(-1.,0.,0.)) ;
#107654=DIRECTION('center_axis',(0.,1.,0.)) ;
#107655=DIRECTION('ref_axis',(1.,0.,0.)) ;
#107656=DIRECTION('center_axis',(0.,-0.986393923832144,-0.164398987305358)) ;
#107657=DIRECTION('ref_axis',(0.,-0.164398987305358,0.986393923832144)) ;
#107658=DIRECTION('center_axis',(0.,0.,1.)) ;
#107659=DIRECTION('ref_axis',(1.,0.,0.)) ;
#107660=DIRECTION('center_axis',(-1.,0.,0.)) ;
#107661=DIRECTION('ref_axis',(0.,2.60208521396523E-14,-1.)) ;
#107662=DIRECTION('center_axis',(1.,0.,0.)) ;
#107663=DIRECTION('ref_axis',(0.,0.,-1.)) ;
#107664=DIRECTION('center_axis',(1.,0.,0.)) ;
#107665=DIRECTION('ref_axis',(0.,0.,-1.)) ;
#107666=DIRECTION('',(0.707106781186546,-8.65956056235495E-17,0.707106781186549)) ;
#107667=DIRECTION('center_axis',(1.,0.,0.)) ;
#107668=DIRECTION('ref_axis',(0.,0.,-1.)) ;
#107669=DIRECTION('',(1.,0.,0.)) ;
#107670=DIRECTION('center_axis',(0.,1.,0.)) ;
#107671=DIRECTION('ref_axis',(0.,0.,1.)) ;
#107672=DIRECTION('center_axis',(0.,1.,0.)) ;
#107673=DIRECTION('ref_axis',(0.,0.,1.)) ;
#107674=DIRECTION('',(0.,1.,0.)) ;
#107675=DIRECTION('center_axis',(0.,1.,0.)) ;
#107676=DIRECTION('ref_axis',(0.,0.,1.)) ;
#107677=DIRECTION('',(0.,1.,0.)) ;
#107678=DIRECTION('center_axis',(0.,1.,0.)) ;
#107679=DIRECTION('ref_axis',(0.,0.,1.)) ;
#107680=DIRECTION('',(0.,1.,0.)) ;
#107681=DIRECTION('center_axis',(0.,1.,0.)) ;
#107682=DIRECTION('ref_axis',(0.,0.,1.)) ;
#107683=DIRECTION('',(0.,1.,0.)) ;
#107684=DIRECTION('center_axis',(0.,1.,0.)) ;
#107685=DIRECTION('ref_axis',(0.,0.,1.)) ;
#107686=DIRECTION('',(0.,1.,0.)) ;
#107687=DIRECTION('center_axis',(-1.,0.,0.)) ;
#107688=DIRECTION('ref_axis',(0.,0.,1.)) ;
#107689=DIRECTION('center_axis',(-1.,0.,0.)) ;
#107690=DIRECTION('ref_axis',(0.,0.,1.)) ;
#107691=DIRECTION('',(0.,0.,-1.)) ;
#107692=DIRECTION('',(0.,1.,0.)) ;
#107693=DIRECTION('',(0.,0.,1.)) ;
#107694=DIRECTION('center_axis',(-2.09002828430941E-16,1.,0.)) ;
#107695=DIRECTION('ref_axis',(-1.,-2.09002828430941E-16,0.)) ;
#107696=DIRECTION('',(1.,2.09002828430941E-16,0.)) ;
#107697=DIRECTION('',(0.,0.,-1.)) ;
#107698=DIRECTION('',(1.,2.09002828430941E-16,0.)) ;
#107699=DIRECTION('',(0.,0.,1.)) ;
#107700=DIRECTION('center_axis',(1.0450141421547E-16,-1.,0.)) ;
#107701=DIRECTION('ref_axis',(1.,1.0450141421547E-16,0.)) ;
#107702=DIRECTION('',(-1.,-1.0450141421547E-16,0.)) ;
#107703=DIRECTION('',(0.,0.,1.)) ;
#107704=DIRECTION('',(1.,1.0450141421547E-16,1.7416902369245E-17)) ;
#107705=DIRECTION('',(0.,0.,-1.)) ;
#107706=DIRECTION('center_axis',(0.,1.,0.)) ;
#107707=DIRECTION('ref_axis',(0.,0.,1.)) ;
#107708=DIRECTION('',(0.422618261740697,0.,-0.906307787036651)) ;
#107709=DIRECTION('center_axis',(-1.,0.,0.)) ;
#107710=DIRECTION('ref_axis',(0.,0.,1.)) ;
#107711=DIRECTION('',(0.,0.986393923832144,-0.164398987305357)) ;
#107712=DIRECTION('',(0.,0.,1.)) ;
#107713=DIRECTION('',(0.,1.,0.)) ;
#107714=DIRECTION('',(0.,0.,-1.)) ;
#107715=DIRECTION('center_axis',(1.,0.,0.)) ;
#107716=DIRECTION('ref_axis',(0.,0.,1.)) ;
#107717=DIRECTION('center_axis',(1.,0.,0.)) ;
#107718=DIRECTION('ref_axis',(0.,0.,1.)) ;
#107719=DIRECTION('center_axis',(1.,0.,0.)) ;
#107720=DIRECTION('ref_axis',(0.,0.,1.)) ;
#107721=DIRECTION('',(0.,0.,-1.)) ;
#107722=DIRECTION('',(0.,1.,0.)) ;
#107723=DIRECTION('',(0.,0.,1.)) ;
#107724=DIRECTION('',(0.,-0.986393923832144,-0.164398987305357)) ;
#107725=DIRECTION('center_axis',(1.,0.,0.)) ;
#107726=DIRECTION('ref_axis',(0.,0.,1.)) ;
#107727=DIRECTION('',(0.,0.,1.)) ;
#107728=DIRECTION('center_axis',(1.0450141421547E-16,-1.,0.)) ;
#107729=DIRECTION('ref_axis',(1.,1.0450141421547E-16,0.)) ;
#107730=DIRECTION('',(-1.,-1.0450141421547E-16,1.7416902369245E-17)) ;
#107731=DIRECTION('',(0.,0.,1.)) ;
#107732=DIRECTION('',(-1.,-1.0450141421547E-16,0.)) ;
#107733=DIRECTION('',(0.,0.,-1.)) ;
#107734=DIRECTION('center_axis',(-0.876215908676647,-0.481918749772156,
0.)) ;
#107735=DIRECTION('ref_axis',(0.481918749772156,-0.876215908676647,0.)) ;
#107736=DIRECTION('',(-0.481918749772156,0.876215908676647,0.)) ;
#107737=DIRECTION('',(0.,0.,-1.)) ;
#107738=DIRECTION('center_axis',(-0.876215908676613,-0.481918749772218,
1.02549544363153E-14)) ;
#107739=DIRECTION('ref_axis',(0.43695445588893,-0.794462647070658,-0.421781822614834)) ;
#107740=DIRECTION('',(0.,0.,-1.)) ;
#107741=DIRECTION('center_axis',(-0.876215908676637,-0.481918749772175,
-7.94557099638636E-15)) ;
#107742=DIRECTION('ref_axis',(0.436954455952196,-0.794462647185776,0.421781822332458)) ;
#107743=DIRECTION('',(0.,0.,-1.)) ;
#107744=DIRECTION('',(-0.481918749772156,0.876215908676647,0.)) ;
#107745=DIRECTION('',(0.,0.,1.)) ;
#107746=DIRECTION('center_axis',(-1.,0.,0.)) ;
#107747=DIRECTION('ref_axis',(0.,0.,1.)) ;
#107748=DIRECTION('',(0.,1.,0.)) ;
#107749=DIRECTION('',(0.,0.,1.)) ;
#107750=DIRECTION('',(0.,1.,0.)) ;
#107751=DIRECTION('',(0.,0.,-1.)) ;
#107752=DIRECTION('center_axis',(-0.876215908676647,-0.481918749772156,
0.)) ;
#107753=DIRECTION('ref_axis',(0.481918749772156,-0.876215908676647,0.)) ;
#107754=DIRECTION('',(-0.481918749772156,0.876215908676647,0.)) ;
#107755=DIRECTION('',(0.,0.,1.)) ;
#107756=DIRECTION('',(-0.481918749772156,0.876215908676647,0.)) ;
#107757=DIRECTION('',(0.,0.,-1.)) ;
#107758=DIRECTION('center_axis',(-3.46944695195361E-15,-1.,0.)) ;
#107759=DIRECTION('ref_axis',(1.,-3.46944695195361E-15,0.)) ;
#107760=DIRECTION('',(-1.,3.46944695195361E-15,0.)) ;
#107761=DIRECTION('',(0.,0.,1.)) ;
#107762=DIRECTION('',(-1.,3.46944695195361E-15,0.)) ;
#107763=DIRECTION('',(0.,0.,-1.)) ;
#107764=DIRECTION('center_axis',(-1.,0.,0.)) ;
#107765=DIRECTION('ref_axis',(0.,0.,1.)) ;
#107766=DIRECTION('',(0.,1.,0.)) ;
#107767=DIRECTION('',(0.,0.,1.)) ;
#107768=DIRECTION('',(0.,1.,0.)) ;
#107769=DIRECTION('',(0.,0.,-1.)) ;
#107770=DIRECTION('center_axis',(0.,1.,0.)) ;
#107771=DIRECTION('ref_axis',(0.,0.,1.)) ;
#107772=DIRECTION('',(1.,0.,0.)) ;
#107773=DIRECTION('',(0.,0.,1.)) ;
#107774=DIRECTION('',(1.,0.,0.)) ;
#107775=DIRECTION('',(0.,0.,-1.)) ;
#107776=DIRECTION('center_axis',(-1.,0.,0.)) ;
#107777=DIRECTION('ref_axis',(0.,0.,1.)) ;
#107778=DIRECTION('',(0.,1.,0.)) ;
#107779=DIRECTION('',(0.,0.,1.)) ;
#107780=DIRECTION('',(0.,1.,0.)) ;
#107781=DIRECTION('',(0.,0.,-1.)) ;
#107782=DIRECTION('center_axis',(0.,-1.,0.)) ;
#107783=DIRECTION('ref_axis',(0.,0.,-1.)) ;
#107784=DIRECTION('',(-1.,0.,0.)) ;
#107785=DIRECTION('',(0.,0.,1.)) ;
#107786=DIRECTION('',(-1.,0.,0.)) ;
#107787=DIRECTION('',(0.,0.,-1.)) ;
#107788=DIRECTION('center_axis',(0.,1.,0.)) ;
#107789=DIRECTION('ref_axis',(0.,0.,-1.)) ;
#107790=DIRECTION('',(2.16840434497101E-16,0.,1.)) ;
#107791=DIRECTION('center_axis',(0.,1.,0.)) ;
#107792=DIRECTION('ref_axis',(0.,0.,-1.)) ;
#107793=DIRECTION('',(-1.,0.,1.73472347597681E-16)) ;
#107794=DIRECTION('center_axis',(0.,1.,0.)) ;
#107795=DIRECTION('ref_axis',(0.,0.,-1.)) ;
#107796=DIRECTION('',(-2.16840434497101E-16,0.,-1.)) ;
#107797=DIRECTION('center_axis',(0.,1.,0.)) ;
#107798=DIRECTION('ref_axis',(0.,0.,-1.)) ;
#107799=DIRECTION('',(1.,0.,-1.73472347597681E-16)) ;
#107800=DIRECTION('center_axis',(1.,0.,0.)) ;
#107801=DIRECTION('ref_axis',(0.,0.,-1.)) ;
#107802=DIRECTION('',(0.,-1.,0.)) ;
#107803=DIRECTION('',(0.,0.,1.)) ;
#107804=DIRECTION('',(0.,-1.,0.)) ;
#107805=DIRECTION('',(0.,0.,-1.)) ;
#107806=DIRECTION('center_axis',(0.,1.,0.)) ;
#107807=DIRECTION('ref_axis',(0.,0.,1.)) ;
#107808=DIRECTION('',(1.,0.,0.)) ;
#107809=DIRECTION('',(1.,0.,0.)) ;
#107810=DIRECTION('',(0.,0.,-1.)) ;
#107811=DIRECTION('center_axis',(0.98058067569092,-0.196116135138184,0.)) ;
#107812=DIRECTION('ref_axis',(0.196116135138184,0.98058067569092,0.)) ;
#107813=DIRECTION('',(-0.196116135138184,-0.98058067569092,0.)) ;
#107814=DIRECTION('',(0.,0.,1.)) ;
#107815=DIRECTION('',(-0.196116135138184,-0.98058067569092,0.)) ;
#107816=DIRECTION('center_axis',(1.,0.,0.)) ;
#107817=DIRECTION('ref_axis',(0.,0.,-1.)) ;
#107818=DIRECTION('',(0.,-1.,0.)) ;
#107819=DIRECTION('',(0.,0.,1.)) ;
#107820=DIRECTION('',(0.,-1.,0.)) ;
#107821=DIRECTION('',(0.,0.,-1.)) ;
#107822=DIRECTION('',(0.,0.,1.)) ;
#107823=DIRECTION('',(0.,-1.,0.)) ;
#107824=DIRECTION('',(0.,0.,-1.)) ;
#107825=DIRECTION('',(0.,1.,0.)) ;
#107826=DIRECTION('center_axis',(0.,1.,0.)) ;
#107827=DIRECTION('ref_axis',(0.,0.,1.)) ;
#107828=DIRECTION('',(1.,0.,0.)) ;
#107829=DIRECTION('',(0.,0.,1.)) ;
#107830=DIRECTION('',(1.,0.,0.)) ;
#107831=DIRECTION('',(0.,0.,-1.)) ;
#107832=DIRECTION('center_axis',(0.,-1.,0.)) ;
#107833=DIRECTION('ref_axis',(0.,0.,1.)) ;
#107834=DIRECTION('',(0.,0.,1.)) ;
#107835=DIRECTION('center_axis',(0.,-1.,0.)) ;
#107836=DIRECTION('ref_axis',(0.,0.,1.)) ;
#107837=DIRECTION('',(1.,0.,1.73472347597681E-16)) ;
#107838=DIRECTION('center_axis',(0.,-1.,0.)) ;
#107839=DIRECTION('ref_axis',(0.,0.,1.)) ;
#107840=DIRECTION('',(4.33680868994202E-16,0.,-1.)) ;
#107841=DIRECTION('center_axis',(0.,-1.,0.)) ;
#107842=DIRECTION('ref_axis',(0.,0.,1.)) ;
#107843=DIRECTION('',(-1.,0.,1.73472347597681E-16)) ;
#107844=DIRECTION('center_axis',(-1.,6.93889390390723E-16,0.)) ;
#107845=DIRECTION('ref_axis',(-6.93889390390723E-16,-1.,0.)) ;
#107846=DIRECTION('',(6.93889390390723E-16,1.,0.)) ;
#107847=DIRECTION('',(0.,0.,1.)) ;
#107848=DIRECTION('',(6.93889390390723E-16,1.,0.)) ;
#107849=DIRECTION('',(0.,0.,-1.)) ;
#107850=DIRECTION('center_axis',(0.,1.,0.)) ;
#107851=DIRECTION('ref_axis',(0.,0.,1.)) ;
#107852=DIRECTION('',(0.,0.,1.)) ;
#107853=DIRECTION('',(1.,0.,0.)) ;
#107854=DIRECTION('',(0.,0.,-1.)) ;
#107855=DIRECTION('',(1.,0.,0.)) ;
#107856=DIRECTION('',(0.,0.,1.)) ;
#107857=DIRECTION('center_axis',(-1.,0.,0.)) ;
#107858=DIRECTION('ref_axis',(0.,0.,1.)) ;
#107859=DIRECTION('',(0.,1.,0.)) ;
#107860=DIRECTION('',(0.,0.,-1.)) ;
#107861=DIRECTION('center_axis',(-1.,0.,0.)) ;
#107862=DIRECTION('ref_axis',(0.,0.,1.)) ;
#107863=DIRECTION('',(0.,0.,1.)) ;
#107864=DIRECTION('center_axis',(-2.09002828430941E-16,1.,0.)) ;
#107865=DIRECTION('ref_axis',(-1.,-2.09002828430941E-16,0.)) ;
#107866=DIRECTION('',(-1.,-2.09002828430941E-16,0.)) ;
#107867=DIRECTION('',(0.,0.,-1.)) ;
#107868=DIRECTION('',(1.,2.09002828430941E-16,0.)) ;
#107869=DIRECTION('',(0.,0.,1.)) ;
#107870=DIRECTION('center_axis',(0.,0.,1.)) ;
#107871=DIRECTION('ref_axis',(1.,0.,0.)) ;
#107872=DIRECTION('center_axis',(0.,0.,1.)) ;
#107873=DIRECTION('ref_axis',(1.,0.,0.)) ;
#107874=DIRECTION('center_axis',(0.,0.,-1.)) ;
#107875=DIRECTION('ref_axis',(1.,0.,0.)) ;
#107876=DIRECTION('center_axis',(0.,0.,1.)) ;
#107877=DIRECTION('ref_axis',(1.,0.,0.)) ;
#107878=DIRECTION('center_axis',(0.,0.,1.)) ;
#107879=DIRECTION('ref_axis',(1.,0.,0.)) ;
#107880=DIRECTION('center_axis',(0.,0.,-1.)) ;
#107881=DIRECTION('ref_axis',(1.,0.,0.)) ;
#107882=DIRECTION('center_axis',(0.,0.,-1.)) ;
#107883=DIRECTION('ref_axis',(1.,0.,0.)) ;
#107884=DIRECTION('center_axis',(0.,0.,1.)) ;
#107885=DIRECTION('ref_axis',(1.,0.,0.)) ;
#107886=DIRECTION('center_axis',(0.,0.,1.)) ;
#107887=DIRECTION('ref_axis',(1.,0.,0.)) ;
#107888=DIRECTION('center_axis',(0.,0.,-1.)) ;
#107889=DIRECTION('ref_axis',(1.,0.,0.)) ;
#107890=DIRECTION('center_axis',(0.,0.,-1.)) ;
#107891=DIRECTION('ref_axis',(1.,0.,0.)) ;
#107892=DIRECTION('center_axis',(0.,0.,1.)) ;
#107893=DIRECTION('ref_axis',(1.,0.,0.)) ;
#107894=DIRECTION('center_axis',(0.,0.,1.)) ;
#107895=DIRECTION('ref_axis',(1.,0.,0.)) ;
#107896=DIRECTION('center_axis',(0.,0.,1.)) ;
#107897=DIRECTION('ref_axis',(1.,0.,0.)) ;
#107898=DIRECTION('center_axis',(0.,0.,1.)) ;
#107899=DIRECTION('ref_axis',(1.,0.,0.)) ;
#107900=DIRECTION('center_axis',(0.,0.,1.)) ;
#107901=DIRECTION('ref_axis',(1.,0.,0.)) ;
#107902=DIRECTION('center_axis',(0.,0.,1.)) ;
#107903=DIRECTION('ref_axis',(1.,0.,0.)) ;
#107904=DIRECTION('center_axis',(0.,0.,1.)) ;
#107905=DIRECTION('ref_axis',(1.,0.,0.)) ;
#107906=DIRECTION('center_axis',(0.,0.,-1.)) ;
#107907=DIRECTION('ref_axis',(1.,0.,0.)) ;
#107908=DIRECTION('center_axis',(0.,0.,1.)) ;
#107909=DIRECTION('ref_axis',(1.,0.,0.)) ;
#107910=DIRECTION('center_axis',(0.,0.,-1.)) ;
#107911=DIRECTION('ref_axis',(1.,0.,0.)) ;
#107912=DIRECTION('center_axis',(0.,0.,1.)) ;
#107913=DIRECTION('ref_axis',(1.,0.,0.)) ;
#107914=DIRECTION('center_axis',(0.,0.,-1.)) ;
#107915=DIRECTION('ref_axis',(1.,0.,0.)) ;
#107916=DIRECTION('center_axis',(0.,0.,-1.)) ;
#107917=DIRECTION('ref_axis',(1.,0.,0.)) ;
#107918=DIRECTION('center_axis',(0.,0.,-1.)) ;
#107919=DIRECTION('ref_axis',(1.,2.6020852139652E-14,0.)) ;
#107920=DIRECTION('center_axis',(0.,0.,-1.)) ;
#107921=DIRECTION('ref_axis',(1.,0.,0.)) ;
#107922=DIRECTION('center_axis',(0.,0.,-1.)) ;
#107923=DIRECTION('ref_axis',(1.,0.,0.)) ;
#107924=DIRECTION('center_axis',(0.,0.,-1.)) ;
#107925=DIRECTION('ref_axis',(1.,0.,0.)) ;
#107926=DIRECTION('center_axis',(0.,0.,-1.)) ;
#107927=DIRECTION('ref_axis',(1.,0.,0.)) ;
#107928=DIRECTION('center_axis',(0.,0.,1.)) ;
#107929=DIRECTION('ref_axis',(1.,0.,0.)) ;
#107930=DIRECTION('center_axis',(0.,0.,1.)) ;
#107931=DIRECTION('ref_axis',(1.,0.,0.)) ;
#107932=DIRECTION('center_axis',(0.,0.,-1.)) ;
#107933=DIRECTION('ref_axis',(1.,0.,0.)) ;
#107934=DIRECTION('center_axis',(0.,0.,-1.)) ;
#107935=DIRECTION('ref_axis',(1.,1.04083408558609E-13,0.)) ;
#107936=DIRECTION('center_axis',(0.,0.,1.)) ;
#107937=DIRECTION('ref_axis',(1.,0.,0.)) ;
#107938=DIRECTION('center_axis',(0.,0.,1.)) ;
#107939=DIRECTION('ref_axis',(1.,0.,0.)) ;
#107940=DIRECTION('center_axis',(0.,0.,-1.)) ;
#107941=DIRECTION('ref_axis',(1.,1.30104260698261E-14,0.)) ;
#107942=DIRECTION('center_axis',(0.,0.,-1.)) ;
#107943=DIRECTION('ref_axis',(1.,0.,0.)) ;
#107944=DIRECTION('center_axis',(0.,0.,1.)) ;
#107945=DIRECTION('ref_axis',(1.,0.,0.)) ;
#107946=DIRECTION('center_axis',(0.,0.,1.)) ;
#107947=DIRECTION('ref_axis',(1.,0.,0.)) ;
#107948=DIRECTION('',(-0.664363838829919,0.74740931868366,0.)) ;
#107949=DIRECTION('',(0.,-1.,0.)) ;
#107950=DIRECTION('',(0.894427190999917,0.447213595499956,0.)) ;
#107951=DIRECTION('',(0.,1.,0.)) ;
#107952=DIRECTION('center_axis',(0.,0.,-1.)) ;
#107953=DIRECTION('ref_axis',(-1.,0.,0.)) ;
#107954=DIRECTION('',(-0.894427190999917,-0.447213595499956,0.)) ;
#107955=DIRECTION('',(0.,1.,0.)) ;
#107956=DIRECTION('',(0.664363838829919,-0.74740931868366,0.)) ;
#107957=DIRECTION('',(0.,-1.,0.)) ;
#107958=DIRECTION('center_axis',(-0.23745309047699,0.,-0.971399006496778)) ;
#107959=DIRECTION('ref_axis',(-0.971399006496778,0.,0.23745309047699)) ;
#107960=DIRECTION('center_axis',(-0.237453090477004,-2.97379739801035E-15,
-0.971399006496774)) ;
#107961=DIRECTION('ref_axis',(0.921799787670054,-0.315455332295983,-0.225328836986026)) ;
#107962=DIRECTION('',(0.971399006496777,0.,-0.23745309047699)) ;
#107963=DIRECTION('',(0.,-1.,0.)) ;
#107964=DIRECTION('',(-0.971399006496777,0.,0.23745309047699)) ;
#107965=DIRECTION('center_axis',(-0.237453090477001,4.30462933422326E-14,
-0.971399006496775)) ;
#107966=DIRECTION('ref_axis',(0.954559354253683,0.185392581174263,-0.233336731039792)) ;
#107967=DIRECTION('',(-0.873786407766991,-0.436893203883493,0.213592233009709)) ;
#107968=DIRECTION('',(0.,1.,0.)) ;
#107969=DIRECTION('',(0.655772517804503,-0.737744082530068,-0.160299948796656)) ;
#107970=DIRECTION('center_axis',(-1.,0.,0.)) ;
#107971=DIRECTION('ref_axis',(0.,0.,1.)) ;
#107972=DIRECTION('',(0.,-1.,0.)) ;
#107973=DIRECTION('center_axis',(-1.,-6.7007887082726E-15,-6.50913949396074E-15)) ;
#107974=DIRECTION('ref_axis',(6.5091394940182E-15,-8.57530417051636E-12,
-1.)) ;
#107975=DIRECTION('',(0.,0.,-1.)) ;
#107976=DIRECTION('center_axis',(-1.,-6.70078870827228E-15,6.50913949396049E-15)) ;
#107977=DIRECTION('ref_axis',(-6.50913949405411E-15,1.3971626257459E-11,
-1.)) ;
#107978=DIRECTION('center_axis',(-1.,6.70078870827231E-15,6.50913949396052E-15)) ;
#107979=DIRECTION('ref_axis',(-6.50913949404309E-15,-1.23225293015881E-11,
-1.)) ;
#107980=DIRECTION('',(0.,0.,-1.)) ;
#107981=DIRECTION('center_axis',(-1.,6.70078870827261E-15,-6.50913949396074E-15)) ;
#107982=DIRECTION('ref_axis',(6.50913949382473E-15,-2.02978006038297E-11,
-1.)) ;
#107983=DIRECTION('center_axis',(-0.23745309047699,0.,0.971399006496778)) ;
#107984=DIRECTION('ref_axis',(0.971399006496778,0.,0.23745309047699)) ;
#107985=DIRECTION('center_axis',(-0.237453090476854,-7.13106519896081E-13,
0.971399006496811)) ;
#107986=DIRECTION('ref_axis',(0.954559354253092,0.185392581177496,0.233336731039639)) ;
#107987=DIRECTION('',(0.971399006496777,0.,0.23745309047699)) ;
#107988=DIRECTION('',(-0.971399006496777,0.,-0.23745309047699)) ;
#107989=DIRECTION('center_axis',(-0.237453090476972,2.29230216096572E-14,
0.971399006496782)) ;
#107990=DIRECTION('ref_axis',(0.921799787671121,-0.315455332292693,0.225328836986263)) ;
#107991=DIRECTION('',(-0.655772517804503,0.737744082530068,-0.160299948796656)) ;
#107992=DIRECTION('',(0.,-1.,0.)) ;
#107993=DIRECTION('',(0.873786407766991,0.436893203883493,0.213592233009709)) ;
#107994=DIRECTION('center_axis',(0.,1.,0.)) ;
#107995=DIRECTION('ref_axis',(0.,0.,1.)) ;
#107996=DIRECTION('',(-0.971399006496777,0.,0.23745309047699)) ;
#107997=DIRECTION('',(0.,0.,-1.)) ;
#107998=DIRECTION('',(0.971399006496777,0.,0.23745309047699)) ;
#107999=DIRECTION('center_axis',(0.,1.,0.)) ;
#108000=DIRECTION('ref_axis',(0.,0.,1.)) ;
#108001=DIRECTION('',(-0.971399006496777,0.,-0.23745309047699)) ;
#108002=DIRECTION('',(0.,0.,1.)) ;
#108003=DIRECTION('',(0.971399006496777,0.,-0.23745309047699)) ;
#108004=DIRECTION('center_axis',(-0.447213595499956,0.894427190999917,0.)) ;
#108005=DIRECTION('ref_axis',(0.,0.,-1.)) ;
#108006=DIRECTION('',(0.,0.,-1.)) ;
#108007=DIRECTION('',(-0.873786407766991,-0.436893203883493,-0.213592233009709)) ;
#108008=DIRECTION('',(-0.894427190999917,-0.447213595499956,0.)) ;
#108009=DIRECTION('',(0.,0.,1.)) ;
#108010=DIRECTION('',(0.894427190999917,0.447213595499956,0.)) ;
#108011=DIRECTION('',(0.873786407766991,0.436893203883493,-0.213592233009709)) ;
#108012=DIRECTION('center_axis',(0.74740931868366,0.664363838829919,0.)) ;
#108013=DIRECTION('ref_axis',(0.,0.,1.)) ;
#108014=DIRECTION('',(0.,0.,-1.)) ;
#108015=DIRECTION('',(0.664363838829919,-0.74740931868366,0.)) ;
#108016=DIRECTION('',(0.655772517804503,-0.737744082530068,0.160299948796656)) ;
#108017=DIRECTION('',(0.,0.,1.)) ;
#108018=DIRECTION('',(-0.655772517804503,0.737744082530068,0.160299948796656)) ;
#108019=DIRECTION('',(-0.664363838829919,0.74740931868366,0.)) ;
#108020=DIRECTION('center_axis',(1.,0.,4.33680868994202E-16)) ;
#108021=DIRECTION('ref_axis',(4.33680868994202E-16,0.,-1.)) ;
#108022=DIRECTION('',(0.,1.,0.)) ;
#108023=DIRECTION('',(4.33680868994202E-16,0.,-1.)) ;
#108024=DIRECTION('',(0.,-1.,0.)) ;
#108025=DIRECTION('',(-4.33680868994202E-16,0.,1.)) ;
#108026=DIRECTION('center_axis',(-1.73472347597681E-16,0.,-1.)) ;
#108027=DIRECTION('ref_axis',(-1.,0.,1.73472347597681E-16)) ;
#108028=DIRECTION('',(-1.,0.,1.73472347597681E-16)) ;
#108029=DIRECTION('',(0.,-1.,0.)) ;
#108030=DIRECTION('',(1.,0.,-1.73472347597681E-16)) ;
#108031=DIRECTION('',(0.,1.,0.)) ;
#108032=DIRECTION('center_axis',(-1.,0.,0.)) ;
#108033=DIRECTION('ref_axis',(0.,0.,1.)) ;
#108034=DIRECTION('',(0.,0.,1.)) ;
#108035=DIRECTION('',(0.,-1.,0.)) ;
#108036=DIRECTION('',(0.,0.,-1.)) ;
#108037=DIRECTION('',(0.,1.,0.)) ;
#108038=DIRECTION('center_axis',(-1.73472347597681E-16,0.,1.)) ;
#108039=DIRECTION('ref_axis',(1.,0.,1.73472347597681E-16)) ;
#108040=DIRECTION('',(0.,1.,0.)) ;
#108041=DIRECTION('',(1.,0.,1.73472347597681E-16)) ;
#108042=DIRECTION('',(0.,-1.,0.)) ;
#108043=DIRECTION('',(-1.,0.,-1.73472347597681E-16)) ;
#108044=DIRECTION('center_axis',(0.,-1.,0.)) ;
#108045=DIRECTION('ref_axis',(0.,0.,-1.)) ;
#108046=DIRECTION('',(-1.,0.,-1.73472347597681E-16)) ;
#108047=DIRECTION('',(0.,0.,-1.)) ;
#108048=DIRECTION('',(1.,0.,-1.73472347597681E-16)) ;
#108049=DIRECTION('',(-4.33680868994202E-16,0.,1.)) ;
#108050=DIRECTION('',(1.,0.,0.)) ;
#108051=DIRECTION('center_axis',(0.,-1.,0.)) ;
#108052=DIRECTION('ref_axis',(0.,0.,-1.)) ;
#108053=DIRECTION('',(0.,0.,-1.)) ;
#108054=DIRECTION('center_axis',(0.,-1.,0.)) ;
#108055=DIRECTION('ref_axis',(0.,0.,-1.)) ;
#108056=DIRECTION('',(-1.,0.,0.)) ;
#108057=DIRECTION('center_axis',(0.,-1.,0.)) ;
#108058=DIRECTION('ref_axis',(0.,0.,1.)) ;
#108059=DIRECTION('',(0.,0.,1.)) ;
#108060=DIRECTION('center_axis',(0.,-1.,0.)) ;
#108061=DIRECTION('ref_axis',(0.,0.,-1.)) ;
#108062=DIRECTION('center_axis',(0.,-1.,0.)) ;
#108063=DIRECTION('ref_axis',(0.,0.,-1.)) ;
#108064=DIRECTION('center_axis',(0.,-1.,0.)) ;
#108065=DIRECTION('ref_axis',(0.,0.,-1.)) ;
#108066=DIRECTION('',(0.,-1.,0.)) ;
#108067=DIRECTION('',(0.,-1.,0.)) ;
#108068=DIRECTION('center_axis',(0.,0.,-1.)) ;
#108069=DIRECTION('ref_axis',(-1.,0.,0.)) ;
#108070=DIRECTION('',(1.,0.,0.)) ;
#108071=DIRECTION('',(0.,-1.,0.)) ;
#108072=DIRECTION('center_axis',(0.,-1.,0.)) ;
#108073=DIRECTION('ref_axis',(0.,0.,-1.)) ;
#108074=DIRECTION('center_axis',(0.,-1.,0.)) ;
#108075=DIRECTION('ref_axis',(0.,0.,-1.)) ;
#108076=DIRECTION('',(0.,-1.,0.)) ;
#108077=DIRECTION('center_axis',(-1.,0.,0.)) ;
#108078=DIRECTION('ref_axis',(0.,0.,1.)) ;
#108079=DIRECTION('',(0.,0.,-1.)) ;
#108080=DIRECTION('',(0.,-1.,0.)) ;
#108081=DIRECTION('center_axis',(0.,-1.,0.)) ;
#108082=DIRECTION('ref_axis',(0.,0.,-1.)) ;
#108083=DIRECTION('center_axis',(0.,-1.,0.)) ;
#108084=DIRECTION('ref_axis',(0.,0.,-1.)) ;
#108085=DIRECTION('',(0.,-1.,0.)) ;
#108086=DIRECTION('center_axis',(0.,0.,1.)) ;
#108087=DIRECTION('ref_axis',(1.,0.,0.)) ;
#108088=DIRECTION('',(-1.,0.,0.)) ;
#108089=DIRECTION('',(0.,-1.,0.)) ;
#108090=DIRECTION('center_axis',(0.,-1.,0.)) ;
#108091=DIRECTION('ref_axis',(0.,0.,-1.)) ;
#108092=DIRECTION('center_axis',(0.,-1.,0.)) ;
#108093=DIRECTION('ref_axis',(0.,0.,1.)) ;
#108094=DIRECTION('',(0.,-1.,0.)) ;
#108095=DIRECTION('center_axis',(1.,0.,0.)) ;
#108096=DIRECTION('ref_axis',(0.,0.,-1.)) ;
#108097=DIRECTION('',(0.,0.,1.)) ;
#108098=DIRECTION('center_axis',(0.,-1.,0.)) ;
#108099=DIRECTION('ref_axis',(0.,0.,-1.)) ;
#108100=DIRECTION('center_axis',(0.,1.,0.)) ;
#108101=DIRECTION('ref_axis',(0.,0.,1.)) ;
#108102=DIRECTION('',(-0.422618261740697,0.,0.906307787036651)) ;
#108103=DIRECTION('center_axis',(0.906307787036651,0.,0.422618261740697)) ;
#108104=DIRECTION('ref_axis',(0.422618261740697,0.,-0.906307787036651)) ;
#108105=DIRECTION('',(-0.422618261740697,0.,0.906307787036651)) ;
#108106=DIRECTION('',(0.422618261740697,0.,-0.906307787036651)) ;
#108107=DIRECTION('center_axis',(-0.906307787036651,0.,-0.422618261740697)) ;
#108108=DIRECTION('ref_axis',(-0.422618261740697,0.,0.906307787036651)) ;
#108109=DIRECTION('',(0.422618261740697,0.,-0.906307787036651)) ;
#108110=DIRECTION('',(-0.422618261740697,0.,0.906307787036651)) ;
#108111=DIRECTION('center_axis',(0.,1.,0.)) ;
#108112=DIRECTION('ref_axis',(0.,0.,1.)) ;
#108113=DIRECTION('',(-0.422618261740697,0.,0.906307787036651)) ;
#108114=DIRECTION('',(0.422618261740697,0.,-0.906307787036651)) ;
#108115=DIRECTION('center_axis',(1.,0.,-2.16840434497101E-16)) ;
#108116=DIRECTION('ref_axis',(-2.16840434497101E-16,0.,-1.)) ;
#108117=DIRECTION('',(2.16840434497101E-16,0.,1.)) ;
#108118=DIRECTION('',(0.,1.,0.)) ;
#108119=DIRECTION('',(-2.16840434497101E-16,0.,-1.)) ;
#108120=DIRECTION('',(0.,-1.,0.)) ;
#108121=DIRECTION('center_axis',(1.73472347597681E-16,0.,1.)) ;
#108122=DIRECTION('ref_axis',(1.,0.,-1.73472347597681E-16)) ;
#108123=DIRECTION('',(0.,-1.,0.)) ;
#108124=DIRECTION('',(-1.,0.,1.73472347597681E-16)) ;
#108125=DIRECTION('',(0.,1.,0.)) ;
#108126=DIRECTION('',(1.,0.,-1.73472347597681E-16)) ;
#108127=DIRECTION('center_axis',(-1.,0.,2.16840434497101E-16)) ;
#108128=DIRECTION('ref_axis',(2.16840434497101E-16,0.,1.)) ;
#108129=DIRECTION('',(0.,-1.,0.)) ;
#108130=DIRECTION('',(-2.16840434497101E-16,0.,-1.)) ;
#108131=DIRECTION('',(0.,1.,0.)) ;
#108132=DIRECTION('',(2.16840434497101E-16,0.,1.)) ;
#108133=DIRECTION('center_axis',(-1.73472347597681E-16,0.,-1.)) ;
#108134=DIRECTION('ref_axis',(-1.,0.,1.73472347597681E-16)) ;
#108135=DIRECTION('',(1.,0.,-1.73472347597681E-16)) ;
#108136=DIRECTION('',(0.,1.,0.)) ;
#108137=DIRECTION('',(-1.,0.,1.73472347597681E-16)) ;
#108138=DIRECTION('',(0.,-1.,0.)) ;
#108139=DIRECTION('center_axis',(0.,1.,0.)) ;
#108140=DIRECTION('ref_axis',(0.,0.,1.)) ;
#108141=DIRECTION('',(1.,0.,-1.73472347597681E-16)) ;
#108142=DIRECTION('',(-2.16840434497101E-16,0.,-1.)) ;
#108143=DIRECTION('',(-1.,0.,1.73472347597681E-16)) ;
#108144=DIRECTION('',(2.16840434497101E-16,0.,1.)) ;
#108145=DIRECTION('',(1.,0.,0.)) ;
#108146=DIRECTION('center_axis',(0.,1.,0.)) ;
#108147=DIRECTION('ref_axis',(0.,0.,1.)) ;
#108148=DIRECTION('',(0.,0.,1.)) ;
#108149=DIRECTION('center_axis',(0.,1.,0.)) ;
#108150=DIRECTION('ref_axis',(0.,0.,1.)) ;
#108151=DIRECTION('',(-1.,0.,0.)) ;
#108152=DIRECTION('center_axis',(0.,1.,0.)) ;
#108153=DIRECTION('ref_axis',(0.,0.,-1.)) ;
#108154=DIRECTION('',(0.,0.,-1.)) ;
#108155=DIRECTION('center_axis',(0.,1.,0.)) ;
#108156=DIRECTION('ref_axis',(0.,0.,1.)) ;
#108157=DIRECTION('center_axis',(0.,1.,0.)) ;
#108158=DIRECTION('ref_axis',(0.,0.,1.)) ;
#108159=DIRECTION('',(0.,1.,0.)) ;
#108160=DIRECTION('center_axis',(0.,-1.,0.)) ;
#108161=DIRECTION('ref_axis',(2.60208521396523E-14,0.,1.)) ;
#108162=DIRECTION('',(0.,1.,0.)) ;
#108163=DIRECTION('center_axis',(0.,0.,1.)) ;
#108164=DIRECTION('ref_axis',(1.,0.,0.)) ;
#108165=DIRECTION('',(-1.,0.,0.)) ;
#108166=DIRECTION('',(0.,1.,0.)) ;
#108167=DIRECTION('center_axis',(0.,1.,0.)) ;
#108168=DIRECTION('ref_axis',(0.,0.,1.)) ;
#108169=DIRECTION('center_axis',(0.,-1.,0.)) ;
#108170=DIRECTION('ref_axis',(0.,0.,1.)) ;
#108171=DIRECTION('',(0.,1.,0.)) ;
#108172=DIRECTION('center_axis',(-1.,0.,0.)) ;
#108173=DIRECTION('ref_axis',(0.,0.,1.)) ;
#108174=DIRECTION('',(0.,0.,-1.)) ;
#108175=DIRECTION('',(0.,1.,0.)) ;
#108176=DIRECTION('center_axis',(0.,1.,0.)) ;
#108177=DIRECTION('ref_axis',(0.,0.,1.)) ;
#108178=DIRECTION('center_axis',(0.,-1.,0.)) ;
#108179=DIRECTION('ref_axis',(0.,0.,1.)) ;
#108180=DIRECTION('',(0.,1.,0.)) ;
#108181=DIRECTION('center_axis',(0.,0.,-1.)) ;
#108182=DIRECTION('ref_axis',(-1.,0.,0.)) ;
#108183=DIRECTION('',(1.,0.,0.)) ;
#108184=DIRECTION('',(0.,1.,0.)) ;
#108185=DIRECTION('center_axis',(0.,1.,0.)) ;
#108186=DIRECTION('ref_axis',(0.,0.,1.)) ;
#108187=DIRECTION('center_axis',(0.,-1.,0.)) ;
#108188=DIRECTION('ref_axis',(0.,0.,1.)) ;
#108189=DIRECTION('',(0.,1.,0.)) ;
#108190=DIRECTION('center_axis',(1.,0.,0.)) ;
#108191=DIRECTION('ref_axis',(0.,0.,-1.)) ;
#108192=DIRECTION('',(0.,0.,1.)) ;
#108193=DIRECTION('center_axis',(0.,1.,0.)) ;
#108194=DIRECTION('ref_axis',(0.,0.,1.)) ;
#108195=DIRECTION('',(1.,0.,0.)) ;
#108196=DIRECTION('',(0.,0.,-1.)) ;
#108197=DIRECTION('',(-1.,0.,0.)) ;
#108198=DIRECTION('',(0.,0.,1.)) ;
#108199=DIRECTION('center_axis',(0.,0.164398987305357,-0.986393923832144)) ;
#108200=DIRECTION('ref_axis',(0.,0.986393923832144,0.164398987305357)) ;
#108201=DIRECTION('',(-1.,-1.0450141421547E-16,-1.7416902369245E-17)) ;
#108202=DIRECTION('',(0.,-0.986393923832144,-0.164398987305357)) ;
#108203=DIRECTION('',(1.,0.,0.)) ;
#108204=DIRECTION('',(0.,0.986393923832144,0.164398987305357)) ;
#108205=DIRECTION('center_axis',(0.,-1.,0.)) ;
#108206=DIRECTION('ref_axis',(0.,0.,-1.)) ;
#108207=DIRECTION('',(0.,0.,1.)) ;
#108208=DIRECTION('',(0.,0.,-1.)) ;
#108209=DIRECTION('',(-1.,0.,0.)) ;
#108210=DIRECTION('center_axis',(0.,0.164398987305357,0.986393923832144)) ;
#108211=DIRECTION('ref_axis',(0.,-0.986393923832144,0.164398987305357)) ;
#108212=DIRECTION('',(0.,0.986393923832144,-0.164398987305357)) ;
#108213=DIRECTION('',(1.,1.0450141421547E-16,-1.7416902369245E-17)) ;
#108214=DIRECTION('',(0.,-0.986393923832144,0.164398987305357)) ;
#108215=DIRECTION('center_axis',(-1.,0.,0.)) ;
#108216=DIRECTION('ref_axis',(0.,0.,1.)) ;
#108217=DIRECTION('',(0.,0.,1.)) ;
#108218=DIRECTION('center_axis',(-1.,0.,0.)) ;
#108219=DIRECTION('ref_axis',(0.,0.,1.)) ;
#108220=DIRECTION('',(0.,-0.986393923832144,0.164398987305357)) ;
#108221=DIRECTION('',(0.,0.,-1.)) ;
#108222=DIRECTION('',(0.,0.986393923832144,0.164398987305357)) ;
#108223=DIRECTION('center_axis',(1.,0.,0.)) ;
#108224=DIRECTION('ref_axis',(0.,0.,-1.)) ;
#108225=DIRECTION('center_axis',(1.,0.,0.)) ;
#108226=DIRECTION('ref_axis',(0.,0.,-1.)) ;
#108227=DIRECTION('center_axis',(1.,0.,0.)) ;
#108228=DIRECTION('ref_axis',(0.,0.,1.)) ;
#108229=DIRECTION('center_axis',(1.,0.,0.)) ;
#108230=DIRECTION('ref_axis',(0.,8.88178419700125E-16,1.)) ;
#108231=DIRECTION('center_axis',(1.,0.,0.)) ;
#108232=DIRECTION('ref_axis',(0.,-1.77635683940025E-15,1.)) ;
#108233=DIRECTION('',(1.,0.,0.)) ;
#108234=DIRECTION('center_axis',(-1.,0.,0.)) ;
#108235=DIRECTION('ref_axis',(0.,0.,1.)) ;
#108236=DIRECTION('',(-1.,0.,0.)) ;
#108237=DIRECTION('center_axis',(0.,0.,-1.)) ;
#108238=DIRECTION('ref_axis',(1.,0.,0.)) ;
#108239=DIRECTION('center_axis',(0.,-1.,0.)) ;
#108240=DIRECTION('ref_axis',(0.,0.,1.)) ;
#108241=DIRECTION('center_axis',(0.971399006496778,0.,-0.23745309047699)) ;
#108242=DIRECTION('ref_axis',(-0.23745309047699,0.,-0.971399006496778)) ;
#108243=DIRECTION('center_axis',(0.971399006496778,0.,-0.237453090476989)) ;
#108244=DIRECTION('ref_axis',(-0.237453090476989,0.,-0.971399006496778)) ;
#108245=DIRECTION('center_axis',(0.655772517804501,-0.73774408253007,-0.160299948796655)) ;
#108246=DIRECTION('ref_axis',(-0.747409318683662,-0.664363838829917,4.77072893932298E-16)) ;
#108247=DIRECTION('center_axis',(-0.439210132176035,-4.72038307384659E-10,
-0.898384360835556)) ;
#108248=DIRECTION('ref_axis',(0.882040291644994,-0.189880214239185,-0.431219698245912)) ;
#108249=DIRECTION('center_axis',(0.655772517804504,-0.737744082530068,-0.160299948796656)) ;
#108250=DIRECTION('ref_axis',(0.74740931868366,0.664363838829919,-2.08334010827303E-16)) ;
#108251=DIRECTION('center_axis',(0.655772517804505,-0.737744082530068,-0.16029994879665)) ;
#108252=DIRECTION('ref_axis',(0.74740931868366,0.66436383882992,-5.75609428574487E-16)) ;
#108253=DIRECTION('center_axis',(0.664363838829919,-0.74740931868366,0.)) ;
#108254=DIRECTION('ref_axis',(0.74740931868366,0.664363838829919,0.)) ;
#108255=DIRECTION('center_axis',(-0.664363838829918,0.747409318683661,0.)) ;
#108256=DIRECTION('ref_axis',(-0.747409318683661,-0.664363838829918,0.)) ;
#108257=DIRECTION('center_axis',(0.,1.,0.)) ;
#108258=DIRECTION('ref_axis',(0.,0.,1.)) ;
#108259=DIRECTION('center_axis',(0.,-1.,0.)) ;
#108260=DIRECTION('ref_axis',(0.,0.,-1.)) ;
#108261=DIRECTION('center_axis',(0.,0.,1.)) ;
#108262=DIRECTION('ref_axis',(1.,0.,0.)) ;
#108263=DIRECTION('center_axis',(0.,0.,-1.)) ;
#108264=DIRECTION('ref_axis',(-1.,0.,0.)) ;
#108265=DIRECTION('center_axis',(0.,0.,-1.)) ;
#108266=DIRECTION('ref_axis',(-1.,0.,0.)) ;
#108267=DIRECTION('center_axis',(0.439210132176171,4.7241906959143E-10,
-0.898384360835489)) ;
#108268=DIRECTION('ref_axis',(0.882040291644681,-0.189880214240793,0.431219698245845)) ;
#108269=DIRECTION('center_axis',(-0.971399006496778,0.,-0.23745309047699)) ;
#108270=DIRECTION('ref_axis',(-0.23745309047699,0.,0.971399006496777)) ;
#108271=DIRECTION('center_axis',(0.971399006496778,0.,0.237453090476989)) ;
#108272=DIRECTION('ref_axis',(0.237453090476989,0.,-0.971399006496778)) ;
#108273=DIRECTION('center_axis',(0.,1.,0.)) ;
#108274=DIRECTION('ref_axis',(1.,0.,0.)) ;
#108275=DIRECTION('center_axis',(-3.54829801904343E-14,1.,8.67361737988405E-15)) ;
#108276=DIRECTION('ref_axis',(1.,3.54829801904343E-14,6.83923985932746E-30)) ;
#108277=DIRECTION('center_axis',(-0.948683298050516,0.316227766016832,4.61630059016357E-15)) ;
#108278=DIRECTION('ref_axis',(0.316227766016832,0.948683298050516,-4.49018244226562E-13)) ;
#108279=DIRECTION('center_axis',(0.,0.,-1.)) ;
#108280=DIRECTION('ref_axis',(1.,0.,0.)) ;
#108281=DIRECTION('center_axis',(0.,-1.,0.)) ;
#108282=DIRECTION('ref_axis',(0.,0.,1.)) ;
#108283=DIRECTION('center_axis',(0.655772517804503,-0.737744082530069,0.160299948796655)) ;
#108284=DIRECTION('ref_axis',(-0.747409318683661,-0.664363838829918,1.99521945175207E-17)) ;
#108285=DIRECTION('center_axis',(0.,1.,0.)) ;
#108286=DIRECTION('ref_axis',(0.,0.,1.)) ;
#108287=DIRECTION('center_axis',(2.73957817177508E-14,1.,0.)) ;
#108288=DIRECTION('ref_axis',(-1.,2.73957817177508E-14,0.)) ;
#108289=DIRECTION('center_axis',(0.894427190999917,0.447213595499956,0.)) ;
#108290=DIRECTION('ref_axis',(-0.447213595499956,0.894427190999917,0.)) ;
#108291=DIRECTION('center_axis',(-0.894427190999916,-0.447213595499958,
0.)) ;
#108292=DIRECTION('ref_axis',(0.447213595499958,-0.894427190999916,0.)) ;
#108293=DIRECTION('center_axis',(0.,0.,1.)) ;
#108294=DIRECTION('ref_axis',(1.,0.,0.)) ;
#108295=DIRECTION('center_axis',(0.,0.,-1.)) ;
#108296=DIRECTION('ref_axis',(-1.,0.,0.)) ;
#108297=DIRECTION('center_axis',(0.,1.,0.)) ;
#108298=DIRECTION('ref_axis',(0.,0.,1.)) ;
#108299=DIRECTION('center_axis',(0.,-1.,0.)) ;
#108300=DIRECTION('ref_axis',(0.,0.,-1.)) ;
#108301=DIRECTION('center_axis',(-0.664363838829919,0.74740931868366,0.)) ;
#108302=DIRECTION('ref_axis',(-0.74740931868366,-0.664363838829919,0.)) ;
#108303=DIRECTION('center_axis',(-0.66436383882992,0.747409318683659,2.52106651083074E-15)) ;
#108304=DIRECTION('ref_axis',(-0.747409318683659,-0.66436383882992,7.82575143531171E-30)) ;
#108305=DIRECTION('center_axis',(-0.655772517804504,0.737744082530068,-0.160299948796656)) ;
#108306=DIRECTION('ref_axis',(-0.74740931868366,-0.664363838829919,2.31673158493852E-16)) ;
#108307=DIRECTION('center_axis',(0.655772517804496,-0.737744082530075,0.160299948796656)) ;
#108308=DIRECTION('ref_axis',(0.747409318683667,0.664363838829911,-2.10122272487167E-17)) ;
#108309=DIRECTION('center_axis',(0.,1.,0.)) ;
#108310=DIRECTION('ref_axis',(1.,0.,0.)) ;
#108311=DIRECTION('center_axis',(-0.873786407766988,-0.436893203883498,
0.213592233009711)) ;
#108312=DIRECTION('ref_axis',(-0.447213595499961,0.894427190999914,5.03515095507592E-16)) ;
#108313=DIRECTION('center_axis',(-0.948683298050516,0.316227766016832,-3.71868658652085E-15)) ;
#108314=DIRECTION('ref_axis',(0.316227766016832,0.948683298050516,-1.37175731938863E-12)) ;
#108315=DIRECTION('center_axis',(0.,1.,0.)) ;
#108316=DIRECTION('ref_axis',(1.,0.,0.)) ;
#108317=DIRECTION('center_axis',(-5.47915634355017E-14,1.,0.)) ;
#108318=DIRECTION('ref_axis',(1.,5.47915634355017E-14,3.46944695195361E-14)) ;
#108319=DIRECTION('center_axis',(-0.971399006496778,0.,0.23745309047699)) ;
#108320=DIRECTION('ref_axis',(0.23745309047699,0.,0.971399006496777)) ;
#108321=DIRECTION('center_axis',(0.971399006496778,-3.69787733965917E-15,
-0.237453090476989)) ;
#108322=DIRECTION('ref_axis',(-0.237453090476989,3.58403898099287E-30,-0.971399006496778)) ;
#108323=DIRECTION('center_axis',(0.873786407766991,0.436893203883493,-0.213592233009709)) ;
#108324=DIRECTION('ref_axis',(-0.447213595499956,0.894427190999917,2.83414331365695E-16)) ;
#108325=DIRECTION('center_axis',(-0.873786407766992,-0.436893203883492,
0.21359223300971)) ;
#108326=DIRECTION('ref_axis',(0.447213595499955,-0.894427190999918,-1.48231119036019E-16)) ;
#108327=DIRECTION('center_axis',(-0.894427190999917,-0.447213595499956,
0.)) ;
#108328=DIRECTION('ref_axis',(0.447213595499956,-0.894427190999917,0.)) ;
#108329=DIRECTION('center_axis',(-0.894427190999917,-0.447213595499955,
0.)) ;
#108330=DIRECTION('ref_axis',(0.447213595499955,-0.894427190999917,0.)) ;
#108331=DIRECTION('center_axis',(0.,1.,0.)) ;
#108332=DIRECTION('ref_axis',(0.,0.,1.)) ;
#108333=DIRECTION('center_axis',(2.66122351428257E-14,1.,6.50521303491301E-15)) ;
#108334=DIRECTION('ref_axis',(-1.,2.66122351428257E-14,3.84707242087163E-30)) ;
#108335=DIRECTION('center_axis',(-0.439210132004979,2.9556401387078E-13,
-0.898384360919183)) ;
#108336=DIRECTION('ref_axis',(0.898384360919183,-2.12487583469939E-11,-0.439210132004979)) ;
#108337=DIRECTION('center_axis',(0.,1.,0.)) ;
#108338=DIRECTION('ref_axis',(1.,0.,0.)) ;
#108339=DIRECTION('center_axis',(-0.87378640776699,-0.436893203883495,-0.213592233009712)) ;
#108340=DIRECTION('ref_axis',(-0.447213595499958,0.894427190999916,1.8708344946598E-16)) ;
#108341=DIRECTION('center_axis',(0.,0.,1.)) ;
#108342=DIRECTION('ref_axis',(1.,0.,0.)) ;
#108343=DIRECTION('center_axis',(0.439210132005031,-4.72579842096268E-13,
-0.898384360919158)) ;
#108344=DIRECTION('ref_axis',(0.898384360919158,-2.70958403094291E-11,0.439210132005031)) ;
#108345=DIRECTION('center_axis',(-0.873786407766991,-0.436893203883493,
-0.213592233009709)) ;
#108346=DIRECTION('ref_axis',(0.447213595499956,-0.894427190999917,-1.06780556900622E-16)) ;
#108347=DIRECTION('center_axis',(-0.873786407766992,-0.436893203883492,
-0.213592233009707)) ;
#108348=DIRECTION('ref_axis',(0.447213595499955,-0.894427190999918,-7.04543255365314E-18)) ;
#108349=DIRECTION('center_axis',(-0.971399006496778,0.,-0.237453090476989)) ;
#108350=DIRECTION('ref_axis',(0.237453090476989,0.,-0.971399006496778)) ;
#108351=DIRECTION('center_axis',(0.971399006496778,0.,0.23745309047699)) ;
#108352=DIRECTION('ref_axis',(0.23745309047699,0.,-0.971399006496777)) ;
#108353=DIRECTION('center_axis',(0.,0.,-1.)) ;
#108354=DIRECTION('ref_axis',(-1.,0.,0.)) ;
#108355=DIRECTION('center_axis',(1.,1.0450141421547E-16,1.7416902369245E-17)) ;
#108356=DIRECTION('ref_axis',(-1.0450141421547E-16,1.,-1.82009092883888E-33)) ;
#108357=DIRECTION('center_axis',(0.672672795322857,0.739940072189994,-7.49312539869347E-10)) ;
#108358=DIRECTION('ref_axis',(0.738044870607246,-0.670949884714448,0.0715263669705305)) ;
#108359=DIRECTION('center_axis',(-1.,0.,0.)) ;
#108360=DIRECTION('ref_axis',(0.,-0.646374896130194,-0.763019982472727)) ;
#108361=DIRECTION('center_axis',(-1.,0.,0.)) ;
#108362=DIRECTION('ref_axis',(0.,0.,1.)) ;
#108363=DIRECTION('center_axis',(-1.,0.,0.)) ;
#108364=DIRECTION('ref_axis',(0.,0.,1.)) ;
#108365=DIRECTION('center_axis',(0.,0.986393923832144,0.164398987305357)) ;
#108366=DIRECTION('ref_axis',(0.,-0.164398987305357,0.986393923832144)) ;
#108367=DIRECTION('center_axis',(0.,-0.986393923832144,-0.164398987305358)) ;
#108368=DIRECTION('ref_axis',(0.,0.164398987305358,-0.986393923832144)) ;
#108369=DIRECTION('center_axis',(0.,0.,1.)) ;
#108370=DIRECTION('ref_axis',(1.,0.,0.)) ;
#108371=DIRECTION('center_axis',(0.,0.,1.)) ;
#108372=DIRECTION('ref_axis',(1.,0.,0.)) ;
#108373=DIRECTION('center_axis',(0.,0.,1.)) ;
#108374=DIRECTION('ref_axis',(1.,0.,0.)) ;
#108375=DIRECTION('center_axis',(0.,0.,-1.)) ;
#108376=DIRECTION('ref_axis',(1.,0.,0.)) ;
#108377=DIRECTION('center_axis',(-1.,0.,0.)) ;
#108378=DIRECTION('ref_axis',(0.,-0.646374896130192,-0.763019982472729)) ;
#108379=DIRECTION('center_axis',(0.,0.,1.)) ;
#108380=DIRECTION('ref_axis',(-1.,0.,0.)) ;
#108381=DIRECTION('center_axis',(0.,0.,-1.)) ;
#108382=DIRECTION('ref_axis',(-1.,0.,0.)) ;
#108383=DIRECTION('center_axis',(1.,1.0450141421547E-16,-1.7416902369245E-17)) ;
#108384=DIRECTION('ref_axis',(-1.0450141421547E-16,1.,1.82009092883888E-33)) ;
#108385=DIRECTION('center_axis',(0.672672795323056,0.739940072189814,7.49430034663666E-10)) ;
#108386=DIRECTION('ref_axis',(0.738044870609142,-0.670949884716522,-0.0715263669315059)) ;
#108387=DIRECTION('center_axis',(1.,0.,0.)) ;
#108388=DIRECTION('ref_axis',(0.,4.33680868994204E-14,1.)) ;
#108389=DIRECTION('center_axis',(0.,0.,-1.)) ;
#108390=DIRECTION('ref_axis',(-1.,0.,0.)) ;
#108391=DIRECTION('center_axis',(0.,-0.986393923832144,0.164398987305357)) ;
#108392=DIRECTION('ref_axis',(0.,-0.164398987305357,-0.986393923832144)) ;
#108393=DIRECTION('center_axis',(1.,0.,0.)) ;
#108394=DIRECTION('ref_axis',(0.,0.,1.)) ;
#108395=DIRECTION('center_axis',(7.58941520739854E-15,0.,-1.)) ;
#108396=DIRECTION('ref_axis',(-1.,0.,-7.58941520739854E-15)) ;
#108397=DIRECTION('center_axis',(1.,0.,-8.67361737988404E-15)) ;
#108398=DIRECTION('ref_axis',(-8.67361737988404E-15,0.,-1.)) ;
#108399=DIRECTION('center_axis',(1.,0.,0.)) ;
#108400=DIRECTION('ref_axis',(0.,0.,-1.)) ;
#108401=DIRECTION('center_axis',(1.,0.,8.67361737988403E-15)) ;
#108402=DIRECTION('ref_axis',(8.67361737988403E-15,0.,-1.)) ;
#108403=DIRECTION('center_axis',(0.,0.,1.)) ;
#108404=DIRECTION('ref_axis',(1.,0.,0.)) ;
#108405=DIRECTION('center_axis',(0.,0.,-1.)) ;
#108406=DIRECTION('ref_axis',(-1.,0.,0.)) ;
#108407=DIRECTION('center_axis',(1.,0.,0.)) ;
#108408=DIRECTION('ref_axis',(0.,0.,1.)) ;
#108409=DIRECTION('center_axis',(-6.50521303491304E-15,0.,-1.)) ;
#108410=DIRECTION('ref_axis',(-1.,0.,6.50521303491304E-15)) ;
#108411=DIRECTION('center_axis',(1.,0.,0.)) ;
#108412=DIRECTION('ref_axis',(0.,0.,1.)) ;
#108413=DIRECTION('center_axis',(1.,9.40395480657835E-30,8.67361737988403E-15)) ;
#108414=DIRECTION('ref_axis',(8.67361737988403E-15,-5.27711695562625E-58,
-1.)) ;
#108415=DIRECTION('center_axis',(0.,0.,-1.)) ;
#108416=DIRECTION('ref_axis',(-1.,0.,0.)) ;
#108417=DIRECTION('center_axis',(6.50521303491304E-15,0.,-1.)) ;
#108418=DIRECTION('ref_axis',(-1.,0.,-6.50521303491304E-15)) ;
#108419=DIRECTION('center_axis',(-1.,0.,0.)) ;
#108420=DIRECTION('ref_axis',(0.,0.,1.)) ;
#108421=DIRECTION('center_axis',(1.,-8.67361737988409E-15,0.)) ;
#108422=DIRECTION('ref_axis',(8.67361737988409E-15,1.,0.)) ;
#108423=DIRECTION('center_axis',(1.,0.,0.)) ;
#108424=DIRECTION('ref_axis',(0.,0.,1.)) ;
#108425=DIRECTION('center_axis',(-4.33680868994202E-16,0.,1.)) ;
#108426=DIRECTION('ref_axis',(1.,0.,4.33680868994202E-16)) ;
#108427=DIRECTION('center_axis',(0.,0.,-1.)) ;
#108428=DIRECTION('ref_axis',(-1.,0.,0.)) ;
#108429=DIRECTION('center_axis',(0.,0.,1.)) ;
#108430=DIRECTION('ref_axis',(1.,0.,0.)) ;
#108431=DIRECTION('center_axis',(0.,1.,0.)) ;
#108432=DIRECTION('ref_axis',(0.,0.,1.)) ;
#108433=DIRECTION('center_axis',(-1.,0.,0.)) ;
#108434=DIRECTION('ref_axis',(0.,0.,-1.)) ;
#108435=DIRECTION('center_axis',(0.,-1.,0.)) ;
#108436=DIRECTION('ref_axis',(0.,0.,1.)) ;
#108437=DIRECTION('center_axis',(0.,1.,0.)) ;
#108438=DIRECTION('ref_axis',(0.,0.,1.)) ;
#108439=DIRECTION('center_axis',(0.,-1.,0.)) ;
#108440=DIRECTION('ref_axis',(0.,0.,1.)) ;
#108441=DIRECTION('center_axis',(-1.,0.,0.)) ;
#108442=DIRECTION('ref_axis',(0.,0.,-1.)) ;
#108443=DIRECTION('center_axis',(-1.,0.,-1.73472347597681E-16)) ;
#108444=DIRECTION('ref_axis',(-1.73472347597681E-16,0.,1.)) ;
#108445=DIRECTION('center_axis',(-1.,0.,0.)) ;
#108446=DIRECTION('ref_axis',(0.,0.,1.)) ;
#108447=DIRECTION('center_axis',(0.,1.,0.)) ;
#108448=DIRECTION('ref_axis',(0.,0.,1.)) ;
#108449=DIRECTION('center_axis',(0.,-1.,0.)) ;
#108450=DIRECTION('ref_axis',(0.,0.,-1.)) ;
#108451=DIRECTION('center_axis',(-4.33680868994202E-16,0.,1.)) ;
#108452=DIRECTION('ref_axis',(1.,0.,4.33680868994202E-16)) ;
#108453=DIRECTION('center_axis',(0.,0.,1.)) ;
#108454=DIRECTION('ref_axis',(1.,0.,0.)) ;
#108455=DIRECTION('center_axis',(0.,0.,-1.)) ;
#108456=DIRECTION('ref_axis',(-1.,0.,0.)) ;
#108457=DIRECTION('center_axis',(0.,1.,0.)) ;
#108458=DIRECTION('ref_axis',(0.,0.,1.)) ;
#108459=DIRECTION('center_axis',(0.,-1.,0.)) ;
#108460=DIRECTION('ref_axis',(0.,0.,-1.)) ;
#108461=DIRECTION('center_axis',(1.,0.,-1.73472347597681E-16)) ;
#108462=DIRECTION('ref_axis',(-1.73472347597681E-16,0.,-1.)) ;
#108463=DIRECTION('center_axis',(-1.,0.,0.)) ;
#108464=DIRECTION('ref_axis',(0.,0.,1.)) ;
#108465=DIRECTION('center_axis',(0.,0.,-1.)) ;
#108466=DIRECTION('ref_axis',(-1.,0.,0.)) ;
#108467=DIRECTION('center_axis',(0.,0.,1.)) ;
#108468=DIRECTION('ref_axis',(1.,0.,0.)) ;
#108469=DIRECTION('center_axis',(0.,0.,-1.)) ;
#108470=DIRECTION('ref_axis',(-1.,0.,0.)) ;
#108471=DIRECTION('center_axis',(0.,1.,0.)) ;
#108472=DIRECTION('ref_axis',(0.,0.,1.)) ;
#108473=DIRECTION('center_axis',(0.,-1.,0.)) ;
#108474=DIRECTION('ref_axis',(0.,0.,1.)) ;
#108475=DIRECTION('center_axis',(0.,1.,0.)) ;
#108476=DIRECTION('ref_axis',(1.,0.,0.)) ;
#108477=DIRECTION('center_axis',(1.,0.,0.)) ;
#108478=DIRECTION('ref_axis',(0.,0.,1.)) ;
#108479=DIRECTION('center_axis',(0.,1.,0.)) ;
#108480=DIRECTION('ref_axis',(1.,0.,0.)) ;
#108481=DIRECTION('center_axis',(1.,0.,0.)) ;
#108482=DIRECTION('ref_axis',(0.,0.,1.)) ;
#108483=DIRECTION('center_axis',(0.,1.,0.)) ;
#108484=DIRECTION('ref_axis',(0.,0.,1.)) ;
#108485=DIRECTION('center_axis',(0.,-1.,0.)) ;
#108486=DIRECTION('ref_axis',(0.,0.,1.)) ;
#108487=DIRECTION('center_axis',(0.,1.,0.)) ;
#108488=DIRECTION('ref_axis',(0.,0.,1.)) ;
#108489=DIRECTION('center_axis',(0.,-1.,0.)) ;
#108490=DIRECTION('ref_axis',(0.,0.,-1.)) ;
#108491=DIRECTION('center_axis',(-1.,0.,-1.73472347597681E-16)) ;
#108492=DIRECTION('ref_axis',(-1.73472347597681E-16,0.,1.)) ;
#108493=DIRECTION('center_axis',(1.,0.,0.)) ;
#108494=DIRECTION('ref_axis',(0.,0.,-1.)) ;
#108495=DIRECTION('center_axis',(1.,0.,-1.73472347597681E-16)) ;
#108496=DIRECTION('ref_axis',(-1.73472347597681E-16,0.,-1.)) ;
#108497=DIRECTION('center_axis',(1.,0.,0.)) ;
#108498=DIRECTION('ref_axis',(0.,0.,-1.)) ;
#108499=DIRECTION('center_axis',(0.,1.,0.)) ;
#108500=DIRECTION('ref_axis',(0.,0.,1.)) ;
#108501=DIRECTION('center_axis',(0.,-1.,0.)) ;
#108502=DIRECTION('ref_axis',(0.,0.,-1.)) ;
#108503=DIRECTION('center_axis',(0.,1.,0.)) ;
#108504=DIRECTION('ref_axis',(1.,0.,0.)) ;
#108505=DIRECTION('center_axis',(0.,0.,1.)) ;
#108506=DIRECTION('ref_axis',(-1.,0.,0.)) ;
#108507=DIRECTION('center_axis',(0.,1.,0.)) ;
#108508=DIRECTION('ref_axis',(1.,0.,0.)) ;
#108509=DIRECTION('center_axis',(0.,0.,-1.)) ;
#108510=DIRECTION('ref_axis',(1.,0.,0.)) ;
#108511=DIRECTION('center_axis',(0.,0.,-1.)) ;
#108512=DIRECTION('ref_axis',(-1.,0.,0.)) ;
#108513=DIRECTION('center_axis',(2.16840434497101E-16,0.,1.)) ;
#108514=DIRECTION('ref_axis',(1.,0.,-2.16840434497101E-16)) ;
#108515=DIRECTION('center_axis',(0.,0.,-1.)) ;
#108516=DIRECTION('ref_axis',(-1.,0.,0.)) ;
#108517=DIRECTION('center_axis',(0.,0.,1.)) ;
#108518=DIRECTION('ref_axis',(1.,0.,0.)) ;
#108519=DIRECTION('center_axis',(0.,-1.,0.)) ;
#108520=DIRECTION('ref_axis',(0.,0.,-1.)) ;
#108521=DIRECTION('center_axis',(1.,0.,0.)) ;
#108522=DIRECTION('ref_axis',(0.,0.,1.)) ;
#108523=DIRECTION('center_axis',(0.,1.,0.)) ;
#108524=DIRECTION('ref_axis',(0.,0.,-1.)) ;
#108525=DIRECTION('center_axis',(0.,-1.,0.)) ;
#108526=DIRECTION('ref_axis',(0.,0.,-1.)) ;
#108527=DIRECTION('center_axis',(0.,1.,0.)) ;
#108528=DIRECTION('ref_axis',(0.,0.,-1.)) ;
#108529=DIRECTION('center_axis',(1.,0.,0.)) ;
#108530=DIRECTION('ref_axis',(0.,0.,1.)) ;
#108531=DIRECTION('center_axis',(1.,0.,-1.73472347597681E-16)) ;
#108532=DIRECTION('ref_axis',(-1.73472347597681E-16,0.,-1.)) ;
#108533=DIRECTION('center_axis',(1.,0.,0.)) ;
#108534=DIRECTION('ref_axis',(0.,0.,-1.)) ;
#108535=DIRECTION('center_axis',(0.,-1.,0.)) ;
#108536=DIRECTION('ref_axis',(0.,0.,-1.)) ;
#108537=DIRECTION('center_axis',(0.,1.,0.)) ;
#108538=DIRECTION('ref_axis',(0.,0.,1.)) ;
#108539=DIRECTION('center_axis',(2.16840434497101E-16,0.,1.)) ;
#108540=DIRECTION('ref_axis',(1.,0.,-2.16840434497101E-16)) ;
#108541=DIRECTION('center_axis',(0.,0.,1.)) ;
#108542=DIRECTION('ref_axis',(1.,0.,0.)) ;
#108543=DIRECTION('center_axis',(0.,0.,-1.)) ;
#108544=DIRECTION('ref_axis',(-1.,0.,0.)) ;
#108545=DIRECTION('center_axis',(0.,-1.,0.)) ;
#108546=DIRECTION('ref_axis',(0.,0.,-1.)) ;
#108547=DIRECTION('center_axis',(0.,1.,0.)) ;
#108548=DIRECTION('ref_axis',(0.,0.,1.)) ;
#108549=DIRECTION('center_axis',(-1.,0.,1.73472347597681E-16)) ;
#108550=DIRECTION('ref_axis',(1.73472347597681E-16,0.,1.)) ;
#108551=DIRECTION('center_axis',(1.,0.,0.)) ;
#108552=DIRECTION('ref_axis',(0.,0.,-1.)) ;
#108553=DIRECTION('center_axis',(-2.16840434497101E-16,0.,-1.)) ;
#108554=DIRECTION('ref_axis',(-1.,0.,2.16840434497101E-16)) ;
#108555=DIRECTION('center_axis',(0.,0.,1.)) ;
#108556=DIRECTION('ref_axis',(1.,0.,0.)) ;
#108557=DIRECTION('center_axis',(0.,0.,-1.)) ;
#108558=DIRECTION('ref_axis',(-1.,0.,0.)) ;
#108559=DIRECTION('center_axis',(0.,-1.,0.)) ;
#108560=DIRECTION('ref_axis',(0.,0.,-1.)) ;
#108561=DIRECTION('center_axis',(0.,1.,0.)) ;
#108562=DIRECTION('ref_axis',(0.,0.,-1.)) ;
#108563=DIRECTION('center_axis',(0.,1.,0.)) ;
#108564=DIRECTION('ref_axis',(1.,0.,0.)) ;
#108565=DIRECTION('center_axis',(-1.,0.,0.)) ;
#108566=DIRECTION('ref_axis',(0.,0.,-1.)) ;
#108567=DIRECTION('center_axis',(0.,1.,0.)) ;
#108568=DIRECTION('ref_axis',(1.,0.,0.)) ;
#108569=DIRECTION('center_axis',(-1.,0.,0.)) ;
#108570=DIRECTION('ref_axis',(0.,0.,-1.)) ;
#108571=DIRECTION('center_axis',(0.,-1.,0.)) ;
#108572=DIRECTION('ref_axis',(0.,0.,-1.)) ;
#108573=DIRECTION('center_axis',(0.,1.,0.)) ;
#108574=DIRECTION('ref_axis',(0.,0.,-1.)) ;
#108575=DIRECTION('center_axis',(0.,-1.,0.)) ;
#108576=DIRECTION('ref_axis',(0.,0.,-1.)) ;
#108577=DIRECTION('center_axis',(0.,1.,0.)) ;
#108578=DIRECTION('ref_axis',(0.,0.,1.)) ;
#108579=DIRECTION('center_axis',(1.,0.,-1.73472347597681E-16)) ;
#108580=DIRECTION('ref_axis',(-1.73472347597681E-16,0.,-1.)) ;
#108581=DIRECTION('center_axis',(-1.,0.,0.)) ;
#108582=DIRECTION('ref_axis',(0.,0.,1.)) ;
#108583=DIRECTION('center_axis',(-1.,0.,1.73472347597681E-16)) ;
#108584=DIRECTION('ref_axis',(1.73472347597681E-16,0.,1.)) ;
#108585=DIRECTION('center_axis',(-1.,0.,0.)) ;
#108586=DIRECTION('ref_axis',(0.,0.,1.)) ;
#108587=DIRECTION('center_axis',(0.,-1.,0.)) ;
#108588=DIRECTION('ref_axis',(0.,0.,-1.)) ;
#108589=DIRECTION('center_axis',(0.,1.,0.)) ;
#108590=DIRECTION('ref_axis',(0.,0.,1.)) ;
#108591=DIRECTION('center_axis',(0.,1.,0.)) ;
#108592=DIRECTION('ref_axis',(1.,0.,0.)) ;
#108593=DIRECTION('center_axis',(0.,0.,1.)) ;
#108594=DIRECTION('ref_axis',(-1.,0.,0.)) ;
#108595=DIRECTION('center_axis',(0.,1.,0.)) ;
#108596=DIRECTION('ref_axis',(1.,0.,0.)) ;
#108597=DIRECTION('center_axis',(0.,0.,-1.)) ;
#108598=DIRECTION('ref_axis',(1.,0.,0.)) ;
#108599=DIRECTION('center_axis',(-2.16840434497101E-16,0.,-1.)) ;
#108600=DIRECTION('ref_axis',(-1.,0.,2.16840434497101E-16)) ;
#108601=DIRECTION('center_axis',(-1.,0.,0.)) ;
#108602=DIRECTION('ref_axis',(0.,0.,1.)) ;
#108603=DIRECTION('center_axis',(0.,-0.632948931301575,-0.774193548387091)) ;
#108604=DIRECTION('ref_axis',(0.,0.774193548387091,-0.632948931301575)) ;
#108605=DIRECTION('center_axis',(0.,0.,1.)) ;
#108606=DIRECTION('ref_axis',(1.,0.,0.)) ;
#108607=DIRECTION('center_axis',(8.67361737988401E-15,0.,1.)) ;
#108608=DIRECTION('ref_axis',(1.,0.,-8.67361737988401E-15)) ;
#108609=DIRECTION('center_axis',(0.,1.,0.)) ;
#108610=DIRECTION('ref_axis',(1.,0.,0.)) ;
#108611=DIRECTION('center_axis',(-1.,0.,0.)) ;
#108612=DIRECTION('ref_axis',(0.,0.,-1.)) ;
#108613=DIRECTION('center_axis',(1.,0.,0.)) ;
#108614=DIRECTION('ref_axis',(0.,0.,-1.)) ;
#108615=DIRECTION('center_axis',(-1.,0.,0.)) ;
#108616=DIRECTION('ref_axis',(0.,0.,1.)) ;
#108617=DIRECTION('center_axis',(0.,0.,-1.)) ;
#108618=DIRECTION('ref_axis',(-1.,0.,0.)) ;
#108619=DIRECTION('center_axis',(0.,0.,-1.)) ;
#108620=DIRECTION('ref_axis',(-1.,0.,0.)) ;
#108621=DIRECTION('center_axis',(-1.,0.,0.)) ;
#108622=DIRECTION('ref_axis',(0.,0.,1.)) ;
#108623=DIRECTION('center_axis',(0.,-0.632948931301567,-0.774193548387097)) ;
#108624=DIRECTION('ref_axis',(0.,-0.774193548387097,0.632948931301567)) ;
#108625=DIRECTION('center_axis',(-1.,0.,0.)) ;
#108626=DIRECTION('ref_axis',(0.,0.,1.)) ;
#108627=DIRECTION('center_axis',(0.,0.632948931301567,-0.774193548387097)) ;
#108628=DIRECTION('ref_axis',(0.,0.774193548387097,0.632948931301567)) ;
#108629=DIRECTION('center_axis',(0.,0.,-1.)) ;
#108630=DIRECTION('ref_axis',(-1.,0.,0.)) ;
#108631=DIRECTION('center_axis',(0.,0.,1.)) ;
#108632=DIRECTION('ref_axis',(1.,0.,0.)) ;
#108633=DIRECTION('center_axis',(-1.,0.,0.)) ;
#108634=DIRECTION('ref_axis',(0.,0.,1.)) ;
#108635=DIRECTION('center_axis',(1.,0.,0.)) ;
#108636=DIRECTION('ref_axis',(0.,0.,1.)) ;
#108637=DIRECTION('center_axis',(1.,0.,0.)) ;
#108638=DIRECTION('ref_axis',(0.,0.,-1.)) ;
#108639=DIRECTION('center_axis',(1.,0.,0.)) ;
#108640=DIRECTION('ref_axis',(0.,0.,-1.)) ;
#108641=DIRECTION('center_axis',(0.,0.,1.)) ;
#108642=DIRECTION('ref_axis',(1.,0.,0.)) ;
#108643=DIRECTION('center_axis',(0.,8.67361737988405E-15,-1.)) ;
#108644=DIRECTION('ref_axis',(0.,1.,8.67361737988405E-15)) ;
#108645=DIRECTION('center_axis',(0.,1.,0.)) ;
#108646=DIRECTION('ref_axis',(1.,0.,0.)) ;
#108647=DIRECTION('center_axis',(1.22050154678007E-14,0.632948931301567,
-0.774193548387097)) ;
#108648=DIRECTION('ref_axis',(1.7347234759768E-14,-0.774193548387097,-0.632948931301567)) ;
#108649=DIRECTION('center_axis',(-1.,0.,0.)) ;
#108650=DIRECTION('ref_axis',(0.,0.,1.)) ;
#108651=DIRECTION('center_axis',(0.,0.,1.)) ;
#108652=DIRECTION('ref_axis',(1.,0.,0.)) ;
#108653=DIRECTION('center_axis',(0.,0.,-1.)) ;
#108654=DIRECTION('ref_axis',(-1.,0.,0.)) ;
#108655=DIRECTION('center_axis',(0.,0.,-1.)) ;
#108656=DIRECTION('ref_axis',(-1.,0.,0.)) ;
#108657=DIRECTION('center_axis',(0.,0.,-1.)) ;
#108658=DIRECTION('ref_axis',(-1.,0.,0.)) ;
#108659=DIRECTION('center_axis',(0.,0.,-1.)) ;
#108660=DIRECTION('ref_axis',(-1.,0.,0.)) ;
#108661=DIRECTION('center_axis',(0.,0.,-1.)) ;
#108662=DIRECTION('ref_axis',(-1.,0.,0.)) ;
#108663=DIRECTION('center_axis',(-0.422618261740697,0.,0.906307787036651)) ;
#108664=DIRECTION('ref_axis',(0.906307787036651,0.,0.422618261740697)) ;
#108665=DIRECTION('center_axis',(0.422618261740697,0.,-0.906307787036651)) ;
#108666=DIRECTION('ref_axis',(-0.906307787036651,0.,-0.422618261740697)) ;
#108667=DIRECTION('center_axis',(0.422618261740697,0.,-0.906307787036651)) ;
#108668=DIRECTION('ref_axis',(-0.906307787036651,0.,-0.422618261740697)) ;
#108669=DIRECTION('center_axis',(-0.422618261740697,0.,0.906307787036651)) ;
#108670=DIRECTION('ref_axis',(0.906307787036651,0.,0.422618261740697)) ;
#108671=DIRECTION('center_axis',(0.,0.,-1.)) ;
#108672=DIRECTION('ref_axis',(-1.,0.,0.)) ;
#108673=DIRECTION('center_axis',(0.,0.,-1.)) ;
#108674=DIRECTION('ref_axis',(-1.,0.,0.)) ;
#108675=DIRECTION('center_axis',(0.,0.,1.)) ;
#108676=DIRECTION('ref_axis',(1.,0.,0.)) ;
#108677=DIRECTION('center_axis',(0.,0.,1.)) ;
#108678=DIRECTION('ref_axis',(1.,0.,0.)) ;
#108679=DIRECTION('center_axis',(0.,0.,-1.)) ;
#108680=DIRECTION('ref_axis',(-1.,0.,0.)) ;
#108681=DIRECTION('center_axis',(0.,0.,-1.)) ;
#108682=DIRECTION('ref_axis',(-1.,0.,0.)) ;
#108683=DIRECTION('center_axis',(0.,0.,1.)) ;
#108684=DIRECTION('ref_axis',(1.,0.,0.)) ;
#108685=DIRECTION('center_axis',(0.,1.,0.)) ;
#108686=DIRECTION('ref_axis',(1.,0.,0.)) ;
#108687=DIRECTION('center_axis',(0.,-0.986393923832144,0.164398987305358)) ;
#108688=DIRECTION('ref_axis',(0.,-0.164398987305358,-0.986393923832144)) ;
#108689=DIRECTION('center_axis',(0.,0.986393923832144,-0.164398987305357)) ;
#108690=DIRECTION('ref_axis',(0.,0.164398987305357,0.986393923832144)) ;
#108691=DIRECTION('center_axis',(0.,-0.986393923832144,0.164398987305358)) ;
#108692=DIRECTION('ref_axis',(0.,-0.164398987305358,-0.986393923832144)) ;
#108693=DIRECTION('center_axis',(-1.,0.,0.)) ;
#108694=DIRECTION('ref_axis',(0.,0.107567764393764,-0.994197755008191)) ;
#108695=DIRECTION('center_axis',(4.02631181035923E-15,-0.928404294083138,
-0.371571617226061)) ;
#108696=DIRECTION('ref_axis',(1.27444840229953E-29,0.371571617226061,-0.928404294083138)) ;
#108697=DIRECTION('center_axis',(0.275516865537137,-0.50093975551097,-0.820457078800105)) ;
#108698=DIRECTION('ref_axis',(3.47276585739718E-16,0.853490367006418,-0.521108619605597)) ;
#108699=DIRECTION('center_axis',(0.,0.,-1.)) ;
#108700=DIRECTION('ref_axis',(-1.,0.,0.)) ;
#108701=DIRECTION('center_axis',(0.,0.,-1.)) ;
#108702=DIRECTION('ref_axis',(-1.,0.,0.)) ;
#108703=DIRECTION('center_axis',(0.,0.,-1.)) ;
#108704=DIRECTION('ref_axis',(-1.,0.,0.)) ;
#108705=DIRECTION('center_axis',(0.,0.,-1.)) ;
#108706=DIRECTION('ref_axis',(-1.,0.,0.)) ;
#108707=DIRECTION('center_axis',(-0.275516865538071,0.500939755523742,-0.820457078791993)) ;
#108708=DIRECTION('ref_axis',(1.34532370065023E-15,0.853490366998217,0.521108619619028)) ;
#108709=DIRECTION('center_axis',(0.,-0.986393923832144,-0.164398987305357)) ;
#108710=DIRECTION('ref_axis',(0.,0.164398987305357,-0.986393923832144)) ;
#108711=DIRECTION('center_axis',(3.5648347838177E-16,0.986393923832144,
0.164398987305358)) ;
#108712=DIRECTION('ref_axis',(3.79675591822878E-31,-0.164398987305358,0.986393923832144)) ;
#108713=DIRECTION('center_axis',(0.,1.,0.)) ;
#108714=DIRECTION('ref_axis',(1.,0.,0.)) ;
#108715=DIRECTION('center_axis',(-1.,0.,0.)) ;
#108716=DIRECTION('ref_axis',(0.,0.,1.)) ;
#108717=DIRECTION('center_axis',(0.,0.,-1.)) ;
#108718=DIRECTION('ref_axis',(-1.,0.,0.)) ;
#108719=DIRECTION('center_axis',(0.,0.,-1.)) ;
#108720=DIRECTION('ref_axis',(-1.,0.,0.)) ;
#108721=DIRECTION('center_axis',(0.,0.,-1.)) ;
#108722=DIRECTION('ref_axis',(-1.,0.,0.)) ;
#108723=DIRECTION('center_axis',(2.168404344971E-15,0.,1.)) ;
#108724=DIRECTION('ref_axis',(1.,0.,-2.168404344971E-15)) ;
#108725=DIRECTION('center_axis',(0.795723237447208,-7.53302716311723E-12,
0.605660407643206)) ;
#108726=DIRECTION('ref_axis',(0.605660407643206,2.00215687134887E-26,-0.795723237447208)) ;
#108727=DIRECTION('center_axis',(1.57772181044204E-26,2.36658271566302E-26,
1.)) ;
#108728=DIRECTION('ref_axis',(3.73380916671669E-52,-1.,2.36658271566302E-26)) ;
#108729=DIRECTION('center_axis',(-0.795723237415222,-2.11663082418553E-11,
0.605660407685229)) ;
#108730=DIRECTION('ref_axis',(0.605660407685229,-9.75816058447732E-26,0.795723237415222)) ;
#132551=CARTESIAN_POINT('',(0.,0.,0.)) ;
#132552=CARTESIAN_POINT('Origin',(4.6,2.65,-6.57304604217164)) ;
#132553=CARTESIAN_POINT('',(4.5,2.61712020253893,-6.37576725740521)) ;
#132554=CARTESIAN_POINT('',(4.5,2.72431432344521,-6.38736518335501)) ;
#132555=CARTESIAN_POINT('Origin',(4.5,2.65,-6.57304604217164)) ;
#132556=CARTESIAN_POINT('',(4.6,2.63356010126946,-6.47440664978842)) ;
#132557=CARTESIAN_POINT('Origin',(4.6,2.61712020253893,-6.37576725740521)) ;
#132558=CARTESIAN_POINT('',(4.6,2.68715716172261,-6.48020561276332)) ;
#132559=CARTESIAN_POINT('Origin',(4.6,2.65,-6.57304604217164)) ;
#132560=CARTESIAN_POINT('Origin',(4.6,2.72431432344521,-6.38736518335501)) ;
#132561=CARTESIAN_POINT('Origin',(0.,10.85,-5.08)) ;
#132562=CARTESIAN_POINT('',(-2.44929359829471E-16,10.95,-3.08)) ;
#132563=CARTESIAN_POINT('Origin',(0.,10.95,-5.08)) ;
#132564=CARTESIAN_POINT('',(-2.32682891837997E-16,10.85,-3.18)) ;
#132565=CARTESIAN_POINT('Origin',(-2.44929359829471E-16,10.85,-3.08)) ;
#132566=CARTESIAN_POINT('',(2.32682891837997E-16,10.85,-6.98)) ;
#132567=CARTESIAN_POINT('Origin',(0.,10.85,-5.08)) ;
#132568=CARTESIAN_POINT('Origin',(0.,10.85,-5.08)) ;
#132569=CARTESIAN_POINT('Origin',(11.0914213562373,0.,-5.08)) ;
#132570=CARTESIAN_POINT('',(11.0207106781187,-1.80110112442984E-16,-3.60928932188135)) ;
#132571=CARTESIAN_POINT('Origin',(11.0207106781187,0.,-5.08)) ;
#132572=CARTESIAN_POINT('',(11.0914213562373,-1.83697019872103E-16,-3.58)) ;
#132573=CARTESIAN_POINT('Origin',(11.0914213562373,-1.71450551880629E-16,
-3.68)) ;
#132574=CARTESIAN_POINT('Origin',(11.0914213562373,0.,-5.08)) ;
#132575=CARTESIAN_POINT('Origin',(12.7,0.,-5.08)) ;
#132576=CARTESIAN_POINT('',(12.8,-1.95943487863576E-16,-6.68)) ;
#132577=CARTESIAN_POINT('Origin',(12.8,0.,-5.08)) ;
#132578=CARTESIAN_POINT('',(12.7,-1.83697019872103E-16,-6.58)) ;
#132579=CARTESIAN_POINT('Origin',(12.7,-1.95943487863577E-16,-6.68)) ;
#132580=CARTESIAN_POINT('',(12.7,1.83697019872103E-16,-3.58)) ;
#132581=CARTESIAN_POINT('Origin',(12.7,0.,-5.08)) ;
#132582=CARTESIAN_POINT('Origin',(12.7,0.,-5.08)) ;
#132583=CARTESIAN_POINT('Origin',(12.7,2.1,-3.69804604217164)) ;
#132584=CARTESIAN_POINT('',(12.7,2.,-3.69804604217164)) ;
#132585=CARTESIAN_POINT('',(12.7,2.11643989873054,-3.59940664978842)) ;
#132586=CARTESIAN_POINT('Origin',(12.7,2.1,-3.69804604217164)) ;
#132587=CARTESIAN_POINT('',(12.8,2.13287979746107,-3.50076725740521)) ;
#132588=CARTESIAN_POINT('Origin',(12.7,2.13287979746107,-3.50076725740521)) ;
#132589=CARTESIAN_POINT('',(12.8,1.9,-3.69804604217164)) ;
#132590=CARTESIAN_POINT('Origin',(12.8,2.1,-3.69804604217164)) ;
#132591=CARTESIAN_POINT('Origin',(12.7,1.9,-3.69804604217164)) ;
#132592=CARTESIAN_POINT('Origin',(12.7,2.65,-3.58695395782836)) ;
#132593=CARTESIAN_POINT('',(12.7,2.63356010126947,-3.68559335021158)) ;
#132594=CARTESIAN_POINT('',(12.7,2.75,-3.58695395782836)) ;
#132595=CARTESIAN_POINT('Origin',(12.7,2.65,-3.58695395782836)) ;
#132596=CARTESIAN_POINT('',(12.8,2.65,-3.58695395782836)) ;
#132597=CARTESIAN_POINT('Origin',(12.7,2.65,-3.58695395782836)) ;
#132598=CARTESIAN_POINT('Origin',(12.7,2.65,-3.58695395782836)) ;
#132599=CARTESIAN_POINT('Origin',(4.5,2.1,-3.69804604217164)) ;
#132600=CARTESIAN_POINT('',(4.6,2.,-3.69804604217164)) ;
#132601=CARTESIAN_POINT('',(12.8,2.,-3.69804604217164)) ;
#132602=CARTESIAN_POINT('',(4.6,2.11643989873054,-3.59940664978842)) ;
#132603=CARTESIAN_POINT('Origin',(4.6,2.1,-3.69804604217164)) ;
#132604=CARTESIAN_POINT('',(4.5,2.11643989873054,-3.59940664978842)) ;
#132605=CARTESIAN_POINT('Origin',(12.7,2.65,-6.57304604217164)) ;
#132606=CARTESIAN_POINT('',(12.8,2.65,-6.57304604217164)) ;
#132607=CARTESIAN_POINT('',(12.7,2.63356010126947,-6.47440664978842)) ;
#132608=CARTESIAN_POINT('Origin',(12.7,2.65,-6.57304604217164)) ;
#132609=CARTESIAN_POINT('',(12.7,2.75,-6.57304604217164)) ;
#132610=CARTESIAN_POINT('Origin',(12.7,2.65,-6.57304604217164)) ;
#132611=CARTESIAN_POINT('Origin',(12.7,2.65,-6.57304604217164)) ;
#132612=CARTESIAN_POINT('Origin',(11.05,0.,-5.08)) ;
#132613=CARTESIAN_POINT('',(10.3,-9.1848509936051E-17,-4.33)) ;
#132614=CARTESIAN_POINT('Origin',(10.3,0.,-5.08)) ;
#132615=CARTESIAN_POINT('',(11.05,-1.83697019872103E-16,-3.58)) ;
#132616=CARTESIAN_POINT('Origin',(11.05,0.,-5.08)) ;
#132617=CARTESIAN_POINT('',(11.05,-1.83697019872103E-16,-3.58)) ;
#132618=CARTESIAN_POINT('Origin',(0.,9.95,-5.08)) ;
#132619=CARTESIAN_POINT('',(0.218101234104781,9.95,-6.96744055580089)) ;
#132620=CARTESIAN_POINT('',(-2.32682891837997E-16,9.95,-6.98)) ;
#132621=CARTESIAN_POINT('Origin',(0.,9.95,-5.08)) ;
#132622=CARTESIAN_POINT('',(0.321518176280636,9.85,-6.9525987456797)) ;
#132623=CARTESIAN_POINT('Ctrl Pts',(0.218101234104783,9.95,-6.96744055580089)) ;
#132624=CARTESIAN_POINT('Ctrl Pts',(0.231193919344581,9.95,-6.9659276441493)) ;
#132625=CARTESIAN_POINT('Ctrl Pts',(0.245192892440024,9.94751445938575,
-6.96415658257392)) ;
#132626=CARTESIAN_POINT('Ctrl Pts',(0.270990685773162,9.93716996065971,
-6.96062157894673)) ;
#132627=CARTESIAN_POINT('Ctrl Pts',(0.282791986325045,9.92931613918426,
-6.95886070936675)) ;
#132628=CARTESIAN_POINT('Ctrl Pts',(0.300953024019397,9.91135900604096,
-6.95603502666193)) ;
#132629=CARTESIAN_POINT('Ctrl Pts',(0.308688523153916,9.90025653083842,
-6.95476256180095)) ;
#132630=CARTESIAN_POINT('Ctrl Pts',(0.318969164829205,9.87583423571802,
-6.95304298667495)) ;
#132631=CARTESIAN_POINT('Ctrl Pts',(0.321518176280638,9.86251584266313,
-6.9525987456797)) ;
#132632=CARTESIAN_POINT('Ctrl Pts',(0.321518176280638,9.85,-6.9525987456797)) ;
#132633=CARTESIAN_POINT('',(0.321518176280636,9.05,-6.9525987456797)) ;
#132634=CARTESIAN_POINT('',(0.321518176280636,8.95,-6.9525987456797)) ;
#132635=CARTESIAN_POINT('',(0.422455466606969,8.95,-6.93243930500675)) ;
#132636=CARTESIAN_POINT('Ctrl Pts',(0.321518176280635,9.05,-6.9525987456797)) ;
#132637=CARTESIAN_POINT('Ctrl Pts',(0.321518176280635,9.03744936090869,
-6.9525987456797)) ;
#132638=CARTESIAN_POINT('Ctrl Pts',(0.324085473150911,9.02409774280079,
-6.95216456224267)) ;
#132639=CARTESIAN_POINT('Ctrl Pts',(0.334387313650439,8.99960748025859,
-6.95034985790769)) ;
#132640=CARTESIAN_POINT('Ctrl Pts',(0.342122499456567,8.98846937989492,
-6.94896564206148)) ;
#132641=CARTESIAN_POINT('Ctrl Pts',(0.360004521225396,8.97064401154629,
-6.94560497807954)) ;
#132642=CARTESIAN_POINT('Ctrl Pts',(0.37144710874947,8.96285745107738,-6.94338208404762)) ;
#132643=CARTESIAN_POINT('Ctrl Pts',(0.396373979529697,8.95253508546271,
-6.93823730327889)) ;
#132644=CARTESIAN_POINT('Ctrl Pts',(0.409857901997329,8.95,-6.93531222506459)) ;
#132645=CARTESIAN_POINT('Ctrl Pts',(0.422455466606967,8.95,-6.93243930500675)) ;
#132646=CARTESIAN_POINT('',(1.14750169623629,8.95,-6.59434469561419)) ;
#132647=CARTESIAN_POINT('Origin',(0.,8.95,-5.08)) ;
#132648=CARTESIAN_POINT('',(1.22782596331729,9.05,-6.529980483939)) ;
#132649=CARTESIAN_POINT('Ctrl Pts',(1.14750169623629,8.95,-6.59434469561419)) ;
#132650=CARTESIAN_POINT('Ctrl Pts',(1.15780003912542,8.95,-6.58654107866494)) ;
#132651=CARTESIAN_POINT('Ctrl Pts',(1.16870807732935,8.95253508546271,-6.57809199882069)) ;
#132652=CARTESIAN_POINT('Ctrl Pts',(1.18867189173408,8.96285745107738,-6.56230390930784)) ;
#132653=CARTESIAN_POINT('Ctrl Pts',(1.19772988083811,8.97064401154629,-6.55496722746149)) ;
#132654=CARTESIAN_POINT('Ctrl Pts',(1.21179864083581,8.98846937989492,-6.54342899722165)) ;
#132655=CARTESIAN_POINT('Ctrl Pts',(1.21783109328768,8.99960748025859,-6.53839325791345)) ;
#132656=CARTESIAN_POINT('Ctrl Pts',(1.22584313288946,9.02409774280079,-6.53166805970666)) ;
#132657=CARTESIAN_POINT('Ctrl Pts',(1.22782596331729,9.03744936090869,-6.529980483939)) ;
#132658=CARTESIAN_POINT('Ctrl Pts',(1.22782596331729,9.05,-6.529980483939)) ;
#132659=CARTESIAN_POINT('',(1.22782596331729,9.85,-6.529980483939)) ;
#132660=CARTESIAN_POINT('',(1.22782596331729,8.95,-6.529980483939)) ;
#132661=CARTESIAN_POINT('',(1.30567057854876,9.95,-6.46029864171205)) ;
#132662=CARTESIAN_POINT('Ctrl Pts',(1.22782596331729,9.85,-6.529980483939)) ;
#132663=CARTESIAN_POINT('Ctrl Pts',(1.22782596331729,9.85579162428539,-6.529980483939)) ;
#132664=CARTESIAN_POINT('Ctrl Pts',(1.22822745887816,9.86162764920015,-6.52964057146522)) ;
#132665=CARTESIAN_POINT('Ctrl Pts',(1.22902753823169,9.86736607146313,-6.52896195467785)) ;
#132666=CARTESIAN_POINT('Ctrl Pts',(1.22973095933684,9.87241123018669,-6.52836532214579)) ;
#132667=CARTESIAN_POINT('Ctrl Pts',(1.23074168751918,9.87738020477702,-6.52750743025347)) ;
#132668=CARTESIAN_POINT('Ctrl Pts',(1.23203099150182,9.88218322835582,-6.52640922147928)) ;
#132669=CARTESIAN_POINT('Ctrl Pts',(1.23351897101726,9.88772637473068,-6.52514178402336)) ;
#132670=CARTESIAN_POINT('Ctrl Pts',(1.2354014557903,9.89313280655103,-6.52353433657835)) ;
#132671=CARTESIAN_POINT('Ctrl Pts',(1.23763252770622,9.89827011881554,-6.52161898274845)) ;
#132672=CARTESIAN_POINT('Ctrl Pts',(1.23953000874363,9.90263929783465,-6.51999001348654)) ;
#132673=CARTESIAN_POINT('Ctrl Pts',(1.24167862345459,9.90681364346946,-6.51813903119877)) ;
#132674=CARTESIAN_POINT('Ctrl Pts',(1.24403025306866,9.91072825704926,-6.51610192167908)) ;
#132675=CARTESIAN_POINT('Ctrl Pts',(1.24687926059923,9.91547082513966,-6.51363395634666)) ;
#132676=CARTESIAN_POINT('Ctrl Pts',(1.25006974298106,9.91990270163235,-6.51085512653216)) ;
#132677=CARTESIAN_POINT('Ctrl Pts',(1.25351940932651,9.92391762881324,-6.50782661463088)) ;
#132678=CARTESIAN_POINT('Ctrl Pts',(1.25634620505523,9.92720762206753,-6.50534492983889)) ;
#132679=CARTESIAN_POINT('Ctrl Pts',(1.25934609941474,9.93021806933733,-6.50269631015879)) ;
#132680=CARTESIAN_POINT('Ctrl Pts',(1.26246241000317,9.93291206679729,-6.49992558372932)) ;
#132681=CARTESIAN_POINT('Ctrl Pts',(1.2664914591119,9.93639511117204,-6.49634333718027)) ;
#132682=CARTESIAN_POINT('Ctrl Pts',(1.27077652588472,9.93940081548805,-6.49250226252408)) ;
#132683=CARTESIAN_POINT('Ctrl Pts',(1.27520851369616,9.94185862744775,-6.48848967391021)) ;
#132684=CARTESIAN_POINT('Ctrl Pts',(1.27864718185097,9.9437655820866,-6.48537640707106)) ;
#132685=CARTESIAN_POINT('Ctrl Pts',(1.28217366418729,9.94534362661778,-6.48216049976224)) ;
#132686=CARTESIAN_POINT('Ctrl Pts',(1.28573335778225,9.94658081625577,-6.47888874922024)) ;
#132687=CARTESIAN_POINT('Ctrl Pts',(1.29026904082682,9.94815721599755,-6.47471995686114)) ;
#132688=CARTESIAN_POINT('Ctrl Pts',(1.29492021413416,9.9491996901822,-6.47040365182261)) ;
#132689=CARTESIAN_POINT('Ctrl Pts',(1.29957290046267,9.9496832238817,-6.46604122438749)) ;
#132690=CARTESIAN_POINT('Ctrl Pts',(1.30160833994479,9.94989475836166,-6.46413276625978)) ;
#132691=CARTESIAN_POINT('Ctrl Pts',(1.30364403319566,9.95,-6.46221561863551)) ;
#132692=CARTESIAN_POINT('Ctrl Pts',(1.30567057854876,9.95,-6.46029864171205)) ;
#132693=CARTESIAN_POINT('',(-0.218101234104782,9.95,-3.19255944419911)) ;
#132694=CARTESIAN_POINT('Origin',(0.,9.95,-5.08)) ;
#132695=CARTESIAN_POINT('',(-0.321518176280637,9.85,-3.2074012543203)) ;
#132696=CARTESIAN_POINT('Ctrl Pts',(-0.218101234104781,9.95,-3.19255944419911)) ;
#132697=CARTESIAN_POINT('Ctrl Pts',(-0.231193919344579,9.95,-3.19407235585069)) ;
#132698=CARTESIAN_POINT('Ctrl Pts',(-0.245192892440022,9.94751445938575,
-3.19584341742608)) ;
#132699=CARTESIAN_POINT('Ctrl Pts',(-0.27099068577316,9.93716996065971,
-3.19937842105326)) ;
#132700=CARTESIAN_POINT('Ctrl Pts',(-0.282791986325042,9.92931613918426,
-3.20113929063325)) ;
#132701=CARTESIAN_POINT('Ctrl Pts',(-0.300953024019395,9.91135900604096,
-3.20396497333807)) ;
#132702=CARTESIAN_POINT('Ctrl Pts',(-0.308688523153914,9.90025653083842,
-3.20523743819905)) ;
#132703=CARTESIAN_POINT('Ctrl Pts',(-0.318969164829203,9.87583423571802,
-3.20695701332505)) ;
#132704=CARTESIAN_POINT('Ctrl Pts',(-0.321518176280636,9.86251584266313,
-3.2074012543203)) ;
#132705=CARTESIAN_POINT('Ctrl Pts',(-0.321518176280636,9.85,-3.2074012543203)) ;
#132706=CARTESIAN_POINT('',(-0.321518176280637,9.05,-3.2074012543203)) ;
#132707=CARTESIAN_POINT('',(-0.321518176280637,8.95,-3.2074012543203)) ;
#132708=CARTESIAN_POINT('',(-0.422455466606969,8.95,-3.22756069499325)) ;
#132709=CARTESIAN_POINT('Ctrl Pts',(-0.321518176280636,9.05,-3.2074012543203)) ;
#132710=CARTESIAN_POINT('Ctrl Pts',(-0.321518176280636,9.03744936090869,
-3.2074012543203)) ;
#132711=CARTESIAN_POINT('Ctrl Pts',(-0.324085473150912,9.02409774280079,
-3.20783543775733)) ;
#132712=CARTESIAN_POINT('Ctrl Pts',(-0.334387313650441,8.99960748025859,
-3.20965014209231)) ;
#132713=CARTESIAN_POINT('Ctrl Pts',(-0.342122499456569,8.98846937989492,
-3.21103435793852)) ;
#132714=CARTESIAN_POINT('Ctrl Pts',(-0.360004521225397,8.97064401154629,
-3.21439502192046)) ;
#132715=CARTESIAN_POINT('Ctrl Pts',(-0.371447108749472,8.96285745107738,
-3.21661791595238)) ;
#132716=CARTESIAN_POINT('Ctrl Pts',(-0.396373979529699,8.95253508546271,
-3.22176269672111)) ;
#132717=CARTESIAN_POINT('Ctrl Pts',(-0.409857901997331,8.95,-3.22468777493542)) ;
#132718=CARTESIAN_POINT('Ctrl Pts',(-0.422455466606968,8.95,-3.22756069499325)) ;
#132719=CARTESIAN_POINT('',(-1.14750169623629,8.95,-3.56565530438581)) ;
#132720=CARTESIAN_POINT('Origin',(0.,8.95,-5.08)) ;
#132721=CARTESIAN_POINT('',(-1.22782596331729,9.05,-3.630019516061)) ;
#132722=CARTESIAN_POINT('Ctrl Pts',(-1.14750169623629,8.95,-3.56565530438581)) ;
#132723=CARTESIAN_POINT('Ctrl Pts',(-1.15780003912542,8.95,-3.57345892133506)) ;
#132724=CARTESIAN_POINT('Ctrl Pts',(-1.16870807732935,8.95253508546271,
-3.58190800117931)) ;
#132725=CARTESIAN_POINT('Ctrl Pts',(-1.18867189173408,8.96285745107738,
-3.59769609069216)) ;
#132726=CARTESIAN_POINT('Ctrl Pts',(-1.19772988083811,8.97064401154629,
-3.60503277253851)) ;
#132727=CARTESIAN_POINT('Ctrl Pts',(-1.21179864083581,8.98846937989492,
-3.61657100277835)) ;
#132728=CARTESIAN_POINT('Ctrl Pts',(-1.21783109328768,8.99960748025859,
-3.62160674208655)) ;
#132729=CARTESIAN_POINT('Ctrl Pts',(-1.22584313288946,9.02409774280079,
-3.62833194029334)) ;
#132730=CARTESIAN_POINT('Ctrl Pts',(-1.22782596331729,9.03744936090869,
-3.630019516061)) ;
#132731=CARTESIAN_POINT('Ctrl Pts',(-1.22782596331729,9.05,-3.630019516061)) ;
#132732=CARTESIAN_POINT('',(-1.22782596331729,9.85,-3.630019516061)) ;
#132733=CARTESIAN_POINT('',(-1.22782596331729,8.95,-3.630019516061)) ;
#132734=CARTESIAN_POINT('',(-1.30567057854876,9.95,-3.69970135828795)) ;
#132735=CARTESIAN_POINT('Ctrl Pts',(-1.22782596331729,9.85,-3.630019516061)) ;
#132736=CARTESIAN_POINT('Ctrl Pts',(-1.22782596331729,9.85579162428539,
-3.630019516061)) ;
#132737=CARTESIAN_POINT('Ctrl Pts',(-1.22822745887816,9.86162764920015,
-3.63035942853478)) ;
#132738=CARTESIAN_POINT('Ctrl Pts',(-1.22902753823169,9.86736607146313,
-3.63103804532216)) ;
#132739=CARTESIAN_POINT('Ctrl Pts',(-1.22973095933683,9.87241123018669,
-3.63163467785421)) ;
#132740=CARTESIAN_POINT('Ctrl Pts',(-1.23074168751918,9.87738020477703,
-3.63249256974653)) ;
#132741=CARTESIAN_POINT('Ctrl Pts',(-1.23203099150181,9.88218322835582,
-3.63359077852072)) ;
#132742=CARTESIAN_POINT('Ctrl Pts',(-1.23351897101725,9.88772637473068,
-3.63485821597664)) ;
#132743=CARTESIAN_POINT('Ctrl Pts',(-1.2354014557903,9.89313280655104,-3.63646566342165)) ;
#132744=CARTESIAN_POINT('Ctrl Pts',(-1.23763252770622,9.89827011881554,
-3.63838101725155)) ;
#132745=CARTESIAN_POINT('Ctrl Pts',(-1.23953000874363,9.90263929783465,
-3.64000998651346)) ;
#132746=CARTESIAN_POINT('Ctrl Pts',(-1.24167862345459,9.90681364346947,
-3.64186096880123)) ;
#132747=CARTESIAN_POINT('Ctrl Pts',(-1.24403025306866,9.91072825704926,
-3.64389807832092)) ;
#132748=CARTESIAN_POINT('Ctrl Pts',(-1.24687926059923,9.91547082513966,
-3.64636604365334)) ;
#132749=CARTESIAN_POINT('Ctrl Pts',(-1.25006974298106,9.91990270163235,
-3.64914487346785)) ;
#132750=CARTESIAN_POINT('Ctrl Pts',(-1.2535194093265,9.92391762881324,-3.65217338536913)) ;
#132751=CARTESIAN_POINT('Ctrl Pts',(-1.25634620505523,9.92720762206753,
-3.65465507016111)) ;
#132752=CARTESIAN_POINT('Ctrl Pts',(-1.25934609941474,9.93021806933733,
-3.65730368984121)) ;
#132753=CARTESIAN_POINT('Ctrl Pts',(-1.26246241000317,9.9329120667973,-3.66007441627069)) ;
#132754=CARTESIAN_POINT('Ctrl Pts',(-1.26649145911191,9.93639511117205,
-3.66365666281975)) ;
#132755=CARTESIAN_POINT('Ctrl Pts',(-1.27077652588473,9.93940081548806,
-3.66749773747593)) ;
#132756=CARTESIAN_POINT('Ctrl Pts',(-1.27520851369618,9.94185862744776,
-3.67151032608981)) ;
#132757=CARTESIAN_POINT('Ctrl Pts',(-1.27864718185098,9.94376558208661,
-3.67462359292896)) ;
#132758=CARTESIAN_POINT('Ctrl Pts',(-1.2821736641873,9.94534362661778,-3.67783950023776)) ;
#132759=CARTESIAN_POINT('Ctrl Pts',(-1.28573335778225,9.94658081625577,
-3.68111125077976)) ;
#132760=CARTESIAN_POINT('Ctrl Pts',(-1.29026904082681,9.94815721599755,
-3.68528004313886)) ;
#132761=CARTESIAN_POINT('Ctrl Pts',(-1.29492021413415,9.9491996901822,-3.68959634817738)) ;
#132762=CARTESIAN_POINT('Ctrl Pts',(-1.29957290046265,9.9496832238817,-3.6939587756125)) ;
#132763=CARTESIAN_POINT('Ctrl Pts',(-1.30160833994478,9.94989475836166,
-3.69586723374022)) ;
#132764=CARTESIAN_POINT('Ctrl Pts',(-1.30364403319566,9.95,-3.69778438136449)) ;
#132765=CARTESIAN_POINT('Ctrl Pts',(-1.30567057854876,9.95,-3.69970135828795)) ;
#132766=CARTESIAN_POINT('Origin',(0.,9.95,-5.08)) ;
#132767=CARTESIAN_POINT('',(-2.32682891837997E-16,9.95,-6.98)) ;
#132768=CARTESIAN_POINT('Origin',(4.6,2.65,-1.49304604217164)) ;
#132769=CARTESIAN_POINT('',(4.5,2.61712020253893,-1.29576725740521)) ;
#132770=CARTESIAN_POINT('',(4.5,2.72431432344521,-1.30736518335501)) ;
#132771=CARTESIAN_POINT('Origin',(4.5,2.65,-1.49304604217164)) ;
#132772=CARTESIAN_POINT('',(4.6,2.63356010126946,-1.39440664978842)) ;
#132773=CARTESIAN_POINT('Origin',(4.6,2.61712020253893,-1.29576725740521)) ;
#132774=CARTESIAN_POINT('',(4.6,2.68715716172261,-1.40020561276332)) ;
#132775=CARTESIAN_POINT('Origin',(4.6,2.65,-1.49304604217164)) ;
#132776=CARTESIAN_POINT('Origin',(4.6,2.72431432344521,-1.30736518335501)) ;
#132777=CARTESIAN_POINT('Origin',(-4.52198039027186,10.1,2.54)) ;
#132778=CARTESIAN_POINT('',(-4.42392232270277,10.0803883864862,-7.62)) ;
#132779=CARTESIAN_POINT('',(-4.52198039027186,10.2,-7.62)) ;
#132780=CARTESIAN_POINT('Origin',(-4.52198039027186,10.1,-7.62)) ;
#132781=CARTESIAN_POINT('',(-4.42392232270277,10.0803883864862,2.54)) ;
#132782=CARTESIAN_POINT('',(-4.42392232270277,10.0803883864862,-2.54)) ;
#132783=CARTESIAN_POINT('',(-4.52198039027186,10.2,2.54)) ;
#132784=CARTESIAN_POINT('Origin',(-4.52198039027186,10.1,2.54)) ;
#132785=CARTESIAN_POINT('',(-4.52198039027186,10.2,2.54)) ;
#132786=CARTESIAN_POINT('Origin',(0.,10.85,0.)) ;
#132787=CARTESIAN_POINT('',(-2.44929359829471E-16,10.95,2.)) ;
#132788=CARTESIAN_POINT('Origin',(0.,10.95,0.)) ;
#132789=CARTESIAN_POINT('',(-2.32682891837997E-16,10.85,1.9)) ;
#132790=CARTESIAN_POINT('Origin',(-2.44929359829471E-16,10.85,2.)) ;
#132791=CARTESIAN_POINT('',(2.32682891837997E-16,10.85,-1.9)) ;
#132792=CARTESIAN_POINT('Origin',(0.,10.85,0.)) ;
#132793=CARTESIAN_POINT('Origin',(0.,10.85,0.)) ;
#132794=CARTESIAN_POINT('Origin',(11.0914213562373,0.,0.)) ;
#132795=CARTESIAN_POINT('',(11.0207106781187,-1.80110112442984E-16,1.47071067811866)) ;
#132796=CARTESIAN_POINT('Origin',(11.0207106781187,0.,0.)) ;
#132797=CARTESIAN_POINT('',(11.0914213562373,-1.83697019872103E-16,1.5)) ;
#132798=CARTESIAN_POINT('Origin',(11.0914213562373,-1.71450551880629E-16,
1.4)) ;
#132799=CARTESIAN_POINT('Origin',(11.0914213562373,0.,0.)) ;
#132800=CARTESIAN_POINT('Origin',(12.7,0.,0.)) ;
#132801=CARTESIAN_POINT('',(12.8,-1.95943487863577E-16,-1.6)) ;
#132802=CARTESIAN_POINT('Origin',(12.8,0.,0.)) ;
#132803=CARTESIAN_POINT('',(12.7,-1.83697019872103E-16,-1.5)) ;
#132804=CARTESIAN_POINT('Origin',(12.7,-1.95943487863577E-16,-1.6)) ;
#132805=CARTESIAN_POINT('',(12.7,1.83697019872103E-16,1.5)) ;
#132806=CARTESIAN_POINT('Origin',(12.7,0.,0.)) ;
#132807=CARTESIAN_POINT('Origin',(12.7,0.,0.)) ;
#132808=CARTESIAN_POINT('Origin',(12.7,2.1,1.38195395782836)) ;
#132809=CARTESIAN_POINT('',(12.7,2.,1.38195395782836)) ;
#132810=CARTESIAN_POINT('',(12.7,2.11643989873054,1.48059335021158)) ;
#132811=CARTESIAN_POINT('Origin',(12.7,2.1,1.38195395782836)) ;
#132812=CARTESIAN_POINT('',(12.8,2.13287979746107,1.57923274259479)) ;
#132813=CARTESIAN_POINT('Origin',(12.7,2.13287979746107,1.57923274259479)) ;
#132814=CARTESIAN_POINT('',(12.8,1.9,1.38195395782836)) ;
#132815=CARTESIAN_POINT('Origin',(12.8,2.1,1.38195395782836)) ;
#132816=CARTESIAN_POINT('Origin',(12.7,1.9,1.38195395782836)) ;
#132817=CARTESIAN_POINT('Origin',(12.7,2.65,1.49304604217164)) ;
#132818=CARTESIAN_POINT('',(12.7,2.63356010126947,1.39440664978842)) ;
#132819=CARTESIAN_POINT('',(12.7,2.75,1.49304604217164)) ;
#132820=CARTESIAN_POINT('Origin',(12.7,2.65,1.49304604217164)) ;
#132821=CARTESIAN_POINT('',(12.8,2.65,1.49304604217164)) ;
#132822=CARTESIAN_POINT('Origin',(12.7,2.65,1.49304604217164)) ;
#132823=CARTESIAN_POINT('Origin',(12.7,2.65,1.49304604217164)) ;
#132824=CARTESIAN_POINT('Origin',(4.5,2.1,1.38195395782836)) ;
#132825=CARTESIAN_POINT('',(4.6,2.,1.38195395782836)) ;
#132826=CARTESIAN_POINT('',(12.8,2.,1.38195395782836)) ;
#132827=CARTESIAN_POINT('',(4.6,2.11643989873054,1.48059335021158)) ;
#132828=CARTESIAN_POINT('Origin',(4.6,2.1,1.38195395782836)) ;
#132829=CARTESIAN_POINT('',(4.5,2.11643989873054,1.48059335021158)) ;
#132830=CARTESIAN_POINT('Origin',(12.7,2.65,-1.49304604217164)) ;
#132831=CARTESIAN_POINT('',(12.8,2.65,-1.49304604217164)) ;
#132832=CARTESIAN_POINT('',(12.7,2.63356010126947,-1.39440664978842)) ;
#132833=CARTESIAN_POINT('Origin',(12.7,2.65,-1.49304604217164)) ;
#132834=CARTESIAN_POINT('',(12.7,2.75,-1.49304604217164)) ;
#132835=CARTESIAN_POINT('Origin',(12.7,2.65,-1.49304604217164)) ;
#132836=CARTESIAN_POINT('Origin',(12.7,2.65,-1.49304604217164)) ;
#132837=CARTESIAN_POINT('Origin',(11.05,0.,0.)) ;
#132838=CARTESIAN_POINT('',(10.3,-9.1848509936051E-17,0.749999999999996)) ;
#132839=CARTESIAN_POINT('Origin',(10.3,0.,0.)) ;
#132840=CARTESIAN_POINT('',(11.05,-1.83697019872103E-16,1.5)) ;
#132841=CARTESIAN_POINT('Origin',(11.05,0.,0.)) ;
#132842=CARTESIAN_POINT('',(11.05,-1.83697019872103E-16,1.5)) ;
#132843=CARTESIAN_POINT('Origin',(0.,9.95,0.)) ;
#132844=CARTESIAN_POINT('',(0.218101234104781,9.95,-1.88744055580089)) ;
#132845=CARTESIAN_POINT('',(-2.32682891837997E-16,9.95,-1.9)) ;
#132846=CARTESIAN_POINT('Origin',(0.,9.95,0.)) ;
#132847=CARTESIAN_POINT('',(0.321518176280636,9.85,-1.8725987456797)) ;
#132848=CARTESIAN_POINT('Ctrl Pts',(0.218101234104784,9.95,-1.88744055580089)) ;
#132849=CARTESIAN_POINT('Ctrl Pts',(0.231193919344581,9.95,-1.8859276441493)) ;
#132850=CARTESIAN_POINT('Ctrl Pts',(0.245192892440025,9.94751445938575,
-1.88415658257392)) ;
#132851=CARTESIAN_POINT('Ctrl Pts',(0.270990685773162,9.93716996065971,
-1.88062157894673)) ;
#132852=CARTESIAN_POINT('Ctrl Pts',(0.282791986325045,9.92931613918426,
-1.87886070936675)) ;
#132853=CARTESIAN_POINT('Ctrl Pts',(0.300953024019397,9.91135900604096,
-1.87603502666193)) ;
#132854=CARTESIAN_POINT('Ctrl Pts',(0.308688523153917,9.90025653083842,
-1.87476256180095)) ;
#132855=CARTESIAN_POINT('Ctrl Pts',(0.318969164829205,9.87583423571802,
-1.87304298667494)) ;
#132856=CARTESIAN_POINT('Ctrl Pts',(0.321518176280638,9.86251584266313,
-1.8725987456797)) ;
#132857=CARTESIAN_POINT('Ctrl Pts',(0.321518176280638,9.85,-1.8725987456797)) ;
#132858=CARTESIAN_POINT('',(0.321518176280636,9.05,-1.8725987456797)) ;
#132859=CARTESIAN_POINT('',(0.321518176280636,8.95,-1.8725987456797)) ;
#132860=CARTESIAN_POINT('',(0.422455466606969,8.95,-1.85243930500675)) ;
#132861=CARTESIAN_POINT('Ctrl Pts',(0.321518176280636,9.05,-1.8725987456797)) ;
#132862=CARTESIAN_POINT('Ctrl Pts',(0.321518176280636,9.03744936090869,
-1.8725987456797)) ;
#132863=CARTESIAN_POINT('Ctrl Pts',(0.324085473150911,9.02409774280079,
-1.87216456224267)) ;
#132864=CARTESIAN_POINT('Ctrl Pts',(0.33438731365044,8.99960748025859,-1.87034985790769)) ;
#132865=CARTESIAN_POINT('Ctrl Pts',(0.342122499456568,8.98846937989492,
-1.86896564206148)) ;
#132866=CARTESIAN_POINT('Ctrl Pts',(0.360004521225396,8.97064401154629,
-1.86560497807954)) ;
#132867=CARTESIAN_POINT('Ctrl Pts',(0.371447108749471,8.96285745107738,
-1.86338208404762)) ;
#132868=CARTESIAN_POINT('Ctrl Pts',(0.396373979529698,8.95253508546271,
-1.85823730327889)) ;
#132869=CARTESIAN_POINT('Ctrl Pts',(0.40985790199733,8.95,-1.85531222506458)) ;
#132870=CARTESIAN_POINT('Ctrl Pts',(0.422455466606968,8.95,-1.85243930500675)) ;
#132871=CARTESIAN_POINT('',(1.14750169623629,8.95,-1.51434469561419)) ;
#132872=CARTESIAN_POINT('Origin',(0.,8.95,0.)) ;
#132873=CARTESIAN_POINT('',(1.22782596331729,9.05,-1.449980483939)) ;
#132874=CARTESIAN_POINT('Ctrl Pts',(1.14750169623629,8.95,-1.51434469561419)) ;
#132875=CARTESIAN_POINT('Ctrl Pts',(1.15780003912542,8.95,-1.50654107866494)) ;
#132876=CARTESIAN_POINT('Ctrl Pts',(1.16870807732935,8.95253508546271,-1.49809199882069)) ;
#132877=CARTESIAN_POINT('Ctrl Pts',(1.18867189173408,8.96285745107738,-1.48230390930784)) ;
#132878=CARTESIAN_POINT('Ctrl Pts',(1.19772988083811,8.97064401154629,-1.47496722746149)) ;
#132879=CARTESIAN_POINT('Ctrl Pts',(1.21179864083581,8.98846937989492,-1.46342899722165)) ;
#132880=CARTESIAN_POINT('Ctrl Pts',(1.21783109328768,8.99960748025859,-1.45839325791345)) ;
#132881=CARTESIAN_POINT('Ctrl Pts',(1.22584313288946,9.02409774280079,-1.45166805970666)) ;
#132882=CARTESIAN_POINT('Ctrl Pts',(1.22782596331729,9.03744936090869,-1.449980483939)) ;
#132883=CARTESIAN_POINT('Ctrl Pts',(1.22782596331729,9.05,-1.449980483939)) ;
#132884=CARTESIAN_POINT('',(1.22782596331729,9.85,-1.449980483939)) ;
#132885=CARTESIAN_POINT('',(1.22782596331729,8.95,-1.449980483939)) ;
#132886=CARTESIAN_POINT('',(1.30567057854876,9.95,-1.38029864171205)) ;
#132887=CARTESIAN_POINT('Ctrl Pts',(1.22782596331729,9.85,-1.449980483939)) ;
#132888=CARTESIAN_POINT('Ctrl Pts',(1.22782596331729,9.85579162428539,-1.449980483939)) ;
#132889=CARTESIAN_POINT('Ctrl Pts',(1.22822745887816,9.86162764920015,-1.44964057146522)) ;
#132890=CARTESIAN_POINT('Ctrl Pts',(1.22902753823169,9.86736607146313,-1.44896195467784)) ;
#132891=CARTESIAN_POINT('Ctrl Pts',(1.22973095933684,9.87241123018669,-1.44836532214579)) ;
#132892=CARTESIAN_POINT('Ctrl Pts',(1.23074168751918,9.87738020477702,-1.44750743025347)) ;
#132893=CARTESIAN_POINT('Ctrl Pts',(1.23203099150182,9.88218322835582,-1.44640922147928)) ;
#132894=CARTESIAN_POINT('Ctrl Pts',(1.23351897101726,9.88772637473068,-1.44514178402336)) ;
#132895=CARTESIAN_POINT('Ctrl Pts',(1.2354014557903,9.89313280655104,-1.44353433657835)) ;
#132896=CARTESIAN_POINT('Ctrl Pts',(1.23763252770622,9.89827011881554,-1.44161898274845)) ;
#132897=CARTESIAN_POINT('Ctrl Pts',(1.23953000874363,9.90263929783464,-1.43999001348654)) ;
#132898=CARTESIAN_POINT('Ctrl Pts',(1.2416786234546,9.90681364346947,-1.43813903119877)) ;
#132899=CARTESIAN_POINT('Ctrl Pts',(1.24403025306866,9.91072825704926,-1.43610192167909)) ;
#132900=CARTESIAN_POINT('Ctrl Pts',(1.24687926059923,9.91547082513966,-1.43363395634667)) ;
#132901=CARTESIAN_POINT('Ctrl Pts',(1.25006974298105,9.91990270163234,-1.43085512653216)) ;
#132902=CARTESIAN_POINT('Ctrl Pts',(1.2535194093265,9.92391762881323,-1.42782661463089)) ;
#132903=CARTESIAN_POINT('Ctrl Pts',(1.25634620505522,9.92720762206753,-1.4253449298389)) ;
#132904=CARTESIAN_POINT('Ctrl Pts',(1.25934609941474,9.93021806933732,-1.4226963101588)) ;
#132905=CARTESIAN_POINT('Ctrl Pts',(1.26246241000318,9.9329120667973,-1.41992558372932)) ;
#132906=CARTESIAN_POINT('Ctrl Pts',(1.26649145911191,9.93639511117205,-1.41634333718026)) ;
#132907=CARTESIAN_POINT('Ctrl Pts',(1.27077652588474,9.93940081548806,-1.41250226252407)) ;
#132908=CARTESIAN_POINT('Ctrl Pts',(1.27520851369618,9.94185862744776,-1.40848967391019)) ;
#132909=CARTESIAN_POINT('Ctrl Pts',(1.27864718185098,9.9437655820866,-1.40537640707105)) ;
#132910=CARTESIAN_POINT('Ctrl Pts',(1.2821736641873,9.94534362661778,-1.40216049976224)) ;
#132911=CARTESIAN_POINT('Ctrl Pts',(1.28573335778226,9.94658081625577,-1.39888874922024)) ;
#132912=CARTESIAN_POINT('Ctrl Pts',(1.29026904082681,9.94815721599755,-1.39471995686114)) ;
#132913=CARTESIAN_POINT('Ctrl Pts',(1.29492021413414,9.9491996901822,-1.39040365182263)) ;
#132914=CARTESIAN_POINT('Ctrl Pts',(1.29957290046265,9.9496832238817,-1.38604122438751)) ;
#132915=CARTESIAN_POINT('Ctrl Pts',(1.30160833994478,9.94989475836166,-1.3841327662598)) ;
#132916=CARTESIAN_POINT('Ctrl Pts',(1.30364403319565,9.95,-1.38221561863552)) ;
#132917=CARTESIAN_POINT('Ctrl Pts',(1.30567057854876,9.95,-1.38029864171205)) ;
#132918=CARTESIAN_POINT('',(-0.218101234104782,9.95,1.88744055580089)) ;
#132919=CARTESIAN_POINT('Origin',(0.,9.95,0.)) ;
#132920=CARTESIAN_POINT('',(-0.321518176280637,9.85,1.8725987456797)) ;
#132921=CARTESIAN_POINT('Ctrl Pts',(-0.218101234104781,9.95,1.88744055580089)) ;
#132922=CARTESIAN_POINT('Ctrl Pts',(-0.231193919344579,9.95,1.88592764414931)) ;
#132923=CARTESIAN_POINT('Ctrl Pts',(-0.245192892440022,9.94751445938575,
1.88415658257392)) ;
#132924=CARTESIAN_POINT('Ctrl Pts',(-0.27099068577316,9.93716996065971,
1.88062157894673)) ;
#132925=CARTESIAN_POINT('Ctrl Pts',(-0.282791986325042,9.92931613918426,
1.87886070936675)) ;
#132926=CARTESIAN_POINT('Ctrl Pts',(-0.300953024019395,9.91135900604096,
1.87603502666193)) ;
#132927=CARTESIAN_POINT('Ctrl Pts',(-0.308688523153914,9.90025653083842,
1.87476256180095)) ;
#132928=CARTESIAN_POINT('Ctrl Pts',(-0.318969164829203,9.87583423571802,
1.87304298667495)) ;
#132929=CARTESIAN_POINT('Ctrl Pts',(-0.321518176280635,9.86251584266313,
1.8725987456797)) ;
#132930=CARTESIAN_POINT('Ctrl Pts',(-0.321518176280635,9.85,1.8725987456797)) ;
#132931=CARTESIAN_POINT('',(-0.321518176280637,9.05,1.8725987456797)) ;
#132932=CARTESIAN_POINT('',(-0.321518176280637,8.95,1.8725987456797)) ;
#132933=CARTESIAN_POINT('',(-0.422455466606969,8.95,1.85243930500675)) ;
#132934=CARTESIAN_POINT('Ctrl Pts',(-0.321518176280636,9.05,1.8725987456797)) ;
#132935=CARTESIAN_POINT('Ctrl Pts',(-0.321518176280636,9.03744936090869,
1.8725987456797)) ;
#132936=CARTESIAN_POINT('Ctrl Pts',(-0.324085473150912,9.02409774280079,
1.87216456224267)) ;
#132937=CARTESIAN_POINT('Ctrl Pts',(-0.334387313650441,8.99960748025859,
1.87034985790769)) ;
#132938=CARTESIAN_POINT('Ctrl Pts',(-0.342122499456569,8.98846937989492,
1.86896564206148)) ;
#132939=CARTESIAN_POINT('Ctrl Pts',(-0.360004521225397,8.97064401154629,
1.86560497807954)) ;
#132940=CARTESIAN_POINT('Ctrl Pts',(-0.371447108749472,8.96285745107738,
1.86338208404762)) ;
#132941=CARTESIAN_POINT('Ctrl Pts',(-0.396373979529699,8.95253508546271,
1.85823730327889)) ;
#132942=CARTESIAN_POINT('Ctrl Pts',(-0.409857901997331,8.95,1.85531222506458)) ;
#132943=CARTESIAN_POINT('Ctrl Pts',(-0.422455466606969,8.95,1.85243930500675)) ;
#132944=CARTESIAN_POINT('',(-1.14750169623629,8.95,1.51434469561419)) ;
#132945=CARTESIAN_POINT('Origin',(0.,8.95,0.)) ;
#132946=CARTESIAN_POINT('',(-1.22782596331729,9.05,1.449980483939)) ;
#132947=CARTESIAN_POINT('Ctrl Pts',(-1.14750169623629,8.95,1.51434469561419)) ;
#132948=CARTESIAN_POINT('Ctrl Pts',(-1.15780003912542,8.95,1.50654107866494)) ;
#132949=CARTESIAN_POINT('Ctrl Pts',(-1.16870807732935,8.95253508546271,
1.49809199882069)) ;
#132950=CARTESIAN_POINT('Ctrl Pts',(-1.18867189173408,8.96285745107738,
1.48230390930784)) ;
#132951=CARTESIAN_POINT('Ctrl Pts',(-1.19772988083811,8.97064401154629,
1.47496722746149)) ;
#132952=CARTESIAN_POINT('Ctrl Pts',(-1.21179864083581,8.98846937989492,
1.46342899722165)) ;
#132953=CARTESIAN_POINT('Ctrl Pts',(-1.21783109328768,8.99960748025859,
1.45839325791345)) ;
#132954=CARTESIAN_POINT('Ctrl Pts',(-1.22584313288946,9.02409774280079,
1.45166805970666)) ;
#132955=CARTESIAN_POINT('Ctrl Pts',(-1.22782596331729,9.03744936090869,
1.449980483939)) ;
#132956=CARTESIAN_POINT('Ctrl Pts',(-1.22782596331729,9.05,1.449980483939)) ;
#132957=CARTESIAN_POINT('',(-1.22782596331729,9.85,1.449980483939)) ;
#132958=CARTESIAN_POINT('',(-1.22782596331729,8.95,1.449980483939)) ;
#132959=CARTESIAN_POINT('',(-1.30567057854876,9.95,1.38029864171205)) ;
#132960=CARTESIAN_POINT('Ctrl Pts',(-1.22782596331729,9.85,1.449980483939)) ;
#132961=CARTESIAN_POINT('Ctrl Pts',(-1.22782596331729,9.85579162428539,
1.449980483939)) ;
#132962=CARTESIAN_POINT('Ctrl Pts',(-1.22822745887816,9.86162764920014,
1.44964057146522)) ;
#132963=CARTESIAN_POINT('Ctrl Pts',(-1.22902753823169,9.86736607146313,
1.44896195467784)) ;
#132964=CARTESIAN_POINT('Ctrl Pts',(-1.22973095933683,9.87241123018669,
1.44836532214579)) ;
#132965=CARTESIAN_POINT('Ctrl Pts',(-1.23074168751918,9.87738020477702,
1.44750743025347)) ;
#132966=CARTESIAN_POINT('Ctrl Pts',(-1.23203099150181,9.88218322835582,
1.44640922147928)) ;
#132967=CARTESIAN_POINT('Ctrl Pts',(-1.23351897101725,9.88772637473068,
1.44514178402336)) ;
#132968=CARTESIAN_POINT('Ctrl Pts',(-1.2354014557903,9.89313280655104,1.44353433657835)) ;
#132969=CARTESIAN_POINT('Ctrl Pts',(-1.23763252770622,9.89827011881554,
1.44161898274845)) ;
#132970=CARTESIAN_POINT('Ctrl Pts',(-1.23953000874363,9.90263929783465,
1.43999001348654)) ;
#132971=CARTESIAN_POINT('Ctrl Pts',(-1.24167862345459,9.90681364346947,
1.43813903119877)) ;
#132972=CARTESIAN_POINT('Ctrl Pts',(-1.24403025306866,9.91072825704926,
1.43610192167908)) ;
#132973=CARTESIAN_POINT('Ctrl Pts',(-1.24687926059922,9.91547082513966,
1.43363395634666)) ;
#132974=CARTESIAN_POINT('Ctrl Pts',(-1.25006974298106,9.91990270163235,
1.43085512653216)) ;
#132975=CARTESIAN_POINT('Ctrl Pts',(-1.2535194093265,9.92391762881324,1.42782661463088)) ;
#132976=CARTESIAN_POINT('Ctrl Pts',(-1.25634620505523,9.92720762206753,
1.42534492983889)) ;
#132977=CARTESIAN_POINT('Ctrl Pts',(-1.25934609941474,9.93021806933733,
1.42269631015879)) ;
#132978=CARTESIAN_POINT('Ctrl Pts',(-1.26246241000317,9.9329120667973,1.41992558372931)) ;
#132979=CARTESIAN_POINT('Ctrl Pts',(-1.26649145911191,9.93639511117205,
1.41634333718025)) ;
#132980=CARTESIAN_POINT('Ctrl Pts',(-1.27077652588474,9.93940081548806,
1.41250226252406)) ;
#132981=CARTESIAN_POINT('Ctrl Pts',(-1.27520851369618,9.94185862744776,
1.40848967391019)) ;
#132982=CARTESIAN_POINT('Ctrl Pts',(-1.27864718185098,9.94376558208661,
1.40537640707104)) ;
#132983=CARTESIAN_POINT('Ctrl Pts',(-1.2821736641873,9.94534362661778,1.40216049976224)) ;
#132984=CARTESIAN_POINT('Ctrl Pts',(-1.28573335778225,9.94658081625577,
1.39888874922024)) ;
#132985=CARTESIAN_POINT('Ctrl Pts',(-1.29026904082681,9.94815721599755,
1.39471995686114)) ;
#132986=CARTESIAN_POINT('Ctrl Pts',(-1.29492021413415,9.9491996901822,1.39040365182262)) ;
#132987=CARTESIAN_POINT('Ctrl Pts',(-1.29957290046265,9.9496832238817,1.3860412243875)) ;
#132988=CARTESIAN_POINT('Ctrl Pts',(-1.30160833994478,9.94989475836166,
1.38413276625978)) ;
#132989=CARTESIAN_POINT('Ctrl Pts',(-1.30364403319566,9.95,1.38221561863551)) ;
#132990=CARTESIAN_POINT('Ctrl Pts',(-1.30567057854876,9.95,1.38029864171205)) ;
#132991=CARTESIAN_POINT('Origin',(0.,9.95,0.)) ;
#132992=CARTESIAN_POINT('',(-2.32682891837997E-16,9.95,-1.9)) ;
#132993=CARTESIAN_POINT('Origin',(3.95,3.75,2.54)) ;
#132994=CARTESIAN_POINT('',(3.95,3.77568567655479,-7.62)) ;
#132995=CARTESIAN_POINT('',(3.95,6.92431432344521,-7.62)) ;
#132996=CARTESIAN_POINT('',(3.95,3.75,-7.62)) ;
#132997=CARTESIAN_POINT('',(3.95,6.92431432344521,2.54)) ;
#132998=CARTESIAN_POINT('',(3.95,6.92431432344521,2.54)) ;
#132999=CARTESIAN_POINT('',(3.95,3.77568567655479,2.54)) ;
#133000=CARTESIAN_POINT('',(3.95,3.75,2.54)) ;
#133001=CARTESIAN_POINT('',(3.95,3.77568567655479,-2.54)) ;
#133002=CARTESIAN_POINT('',(3.95,4.6,-1.275)) ;
#133003=CARTESIAN_POINT('',(3.95,4.4,-1.475)) ;
#133004=CARTESIAN_POINT('Origin',(3.95,4.6,-1.475)) ;
#133005=CARTESIAN_POINT('',(3.95,5.88396692803319,-1.275)) ;
#133006=CARTESIAN_POINT('',(3.95,3.75,-1.275)) ;
#133007=CARTESIAN_POINT('',(3.95,6.08618232569815,-1.475)) ;
#133008=CARTESIAN_POINT('Ctrl Pts',(3.95,6.08618232569815,-1.475)) ;
#133009=CARTESIAN_POINT('Ctrl Pts',(3.95,6.08618232225605,-1.36605743722782)) ;
#133010=CARTESIAN_POINT('Ctrl Pts',(3.95,5.99411624638819,-1.27500000329373)) ;
#133011=CARTESIAN_POINT('Ctrl Pts',(3.95,5.88396692803319,-1.275)) ;
#133012=CARTESIAN_POINT('',(3.95,6.08618232569815,-2.775)) ;
#133013=CARTESIAN_POINT('',(3.95,6.08618232569815,2.54)) ;
#133014=CARTESIAN_POINT('',(3.95,5.88396692803319,-2.975)) ;
#133015=CARTESIAN_POINT('Ctrl Pts',(3.95,5.88396692803319,-2.975)) ;
#133016=CARTESIAN_POINT('Ctrl Pts',(3.95,5.99411624638818,-2.97499999670621)) ;
#133017=CARTESIAN_POINT('Ctrl Pts',(3.95,6.08618232225605,-2.88394256277222)) ;
#133018=CARTESIAN_POINT('Ctrl Pts',(3.95,6.08618232569815,-2.775)) ;
#133019=CARTESIAN_POINT('',(3.95,4.6,-2.975)) ;
#133020=CARTESIAN_POINT('',(3.95,4.5,-2.975)) ;
#133021=CARTESIAN_POINT('',(3.95,4.4,-2.775)) ;
#133022=CARTESIAN_POINT('Origin',(3.95,4.6,-2.775)) ;
#133023=CARTESIAN_POINT('',(3.95,4.4,2.54)) ;
#133024=CARTESIAN_POINT('Origin',(3.4,7.95,2.54)) ;
#133025=CARTESIAN_POINT('',(3.34087287789487,7.95,2.04)) ;
#133026=CARTESIAN_POINT('',(3.,7.95,2.04)) ;
#133027=CARTESIAN_POINT('',(3.4,7.95,2.04)) ;
#133028=CARTESIAN_POINT('',(3.34087287789487,7.95,-7.62)) ;
#133029=CARTESIAN_POINT('',(3.34087287789487,7.95,2.54)) ;
#133030=CARTESIAN_POINT('',(3.,7.95,-7.62)) ;
#133031=CARTESIAN_POINT('',(3.4,7.95,-7.62)) ;
#133032=CARTESIAN_POINT('',(3.,7.95,2.54)) ;
#133033=CARTESIAN_POINT('Origin',(2.9,7.95,2.54)) ;
#133034=CARTESIAN_POINT('',(2.9,8.05,2.04)) ;
#133035=CARTESIAN_POINT('',(2.9,9.85,2.04)) ;
#133036=CARTESIAN_POINT('',(2.9,10.05,2.04)) ;
#133037=CARTESIAN_POINT('',(2.9,8.05,-7.62)) ;
#133038=CARTESIAN_POINT('',(2.9,8.05,-2.54)) ;
#133039=CARTESIAN_POINT('',(2.9,9.85,-7.62)) ;
#133040=CARTESIAN_POINT('',(2.9,7.95,-7.62)) ;
#133041=CARTESIAN_POINT('',(2.9,9.85,2.54)) ;
#133042=CARTESIAN_POINT('Origin',(2.9,9.95,2.54)) ;
#133043=CARTESIAN_POINT('',(3.,9.95,2.04)) ;
#133044=CARTESIAN_POINT('',(3.3,9.95,2.04)) ;
#133045=CARTESIAN_POINT('',(2.9,9.95,2.04)) ;
#133046=CARTESIAN_POINT('',(3.,9.95,-7.62)) ;
#133047=CARTESIAN_POINT('',(3.,9.95,-2.54)) ;
#133048=CARTESIAN_POINT('',(3.3,9.95,-7.62)) ;
#133049=CARTESIAN_POINT('',(2.9,9.95,-7.62)) ;
#133050=CARTESIAN_POINT('',(3.3,9.95,2.54)) ;
#133051=CARTESIAN_POINT('Origin',(3.3,10.05,2.54)) ;
#133052=CARTESIAN_POINT('',(3.4,10.05,2.04)) ;
#133053=CARTESIAN_POINT('',(3.4,10.05,-7.62)) ;
#133054=CARTESIAN_POINT('',(3.4,10.05,2.54)) ;
#133055=CARTESIAN_POINT('Origin',(3.3,10.05,2.04)) ;
#133056=CARTESIAN_POINT('Origin',(3.3,10.05,-7.62)) ;
#133057=CARTESIAN_POINT('Origin',(3.,9.85,2.54)) ;
#133058=CARTESIAN_POINT('Origin',(3.,9.85,2.04)) ;
#133059=CARTESIAN_POINT('Origin',(3.,9.85,-7.62)) ;
#133060=CARTESIAN_POINT('Origin',(3.,8.05,2.54)) ;
#133061=CARTESIAN_POINT('Origin',(3.,8.05,2.04)) ;
#133062=CARTESIAN_POINT('Origin',(3.,8.05,-7.62)) ;
#133063=CARTESIAN_POINT('Origin',(3.34087287789487,7.85,2.54)) ;
#133064=CARTESIAN_POINT('',(3.4,7.93064727789309,2.04)) ;
#133065=CARTESIAN_POINT('Origin',(3.34087287789487,7.85,2.04)) ;
#133066=CARTESIAN_POINT('',(3.4,7.93064727789309,2.54)) ;
#133067=CARTESIAN_POINT('',(3.4,7.93064727789309,2.54)) ;
#133068=CARTESIAN_POINT('',(3.42849446876253,7.89819187497721,2.54)) ;
#133069=CARTESIAN_POINT('Origin',(3.34087287789487,7.85,2.54)) ;
#133070=CARTESIAN_POINT('',(3.42849446876253,7.89819187497721,-7.62)) ;
#133071=CARTESIAN_POINT('',(3.42849446876253,7.89819187497721,2.54)) ;
#133072=CARTESIAN_POINT('Origin',(3.34087287789487,7.85,-7.62)) ;
#133073=CARTESIAN_POINT('Origin',(4.5,-2.8,2.54)) ;
#133074=CARTESIAN_POINT('',(4.5,-2.4,-1.96214168703486)) ;
#133075=CARTESIAN_POINT('',(4.5,-2.7,-1.52315462117279)) ;
#133076=CARTESIAN_POINT('Origin',(4.5,0.,0.)) ;
#133077=CARTESIAN_POINT('',(4.5,-2.7,-3.55684537882722)) ;
#133078=CARTESIAN_POINT('',(4.5,-2.7,2.54)) ;
#133079=CARTESIAN_POINT('',(4.5,-2.4,-3.11785831296514)) ;
#133080=CARTESIAN_POINT('Origin',(4.5,0.,-5.08)) ;
#133081=CARTESIAN_POINT('',(4.5,-2.4,-1.92613602842582)) ;
#133082=CARTESIAN_POINT('Origin',(4.5,-2.3,2.54)) ;
#133083=CARTESIAN_POINT('',(4.6,-2.3,2.54)) ;
#133084=CARTESIAN_POINT('',(12.7,-2.3,2.54)) ;
#133085=CARTESIAN_POINT('',(4.5,-2.3,2.54)) ;
#133086=CARTESIAN_POINT('',(4.6,-2.3,1.96214168703486)) ;
#133087=CARTESIAN_POINT('',(4.6,-2.3,1.92613602842582)) ;
#133088=CARTESIAN_POINT('',(12.7,-2.3,1.96214168703486)) ;
#133089=CARTESIAN_POINT('',(4.5,-2.3,1.96214168703486)) ;
#133090=CARTESIAN_POINT('',(12.7,-2.3,2.54)) ;
#133091=CARTESIAN_POINT('Origin',(12.8,2.75,2.54)) ;
#133092=CARTESIAN_POINT('',(12.7,2.75,2.54)) ;
#133093=CARTESIAN_POINT('',(4.55912712210513,2.75,-3.58695395782836)) ;
#133094=CARTESIAN_POINT('',(12.8,2.75,-3.58695395782836)) ;
#133095=CARTESIAN_POINT('',(4.55912712210513,2.75,-1.49304604217164)) ;
#133096=CARTESIAN_POINT('',(4.55912712210514,2.75,-1.49304604217164)) ;
#133097=CARTESIAN_POINT('',(12.8,2.75,-1.49304604217164)) ;
#133098=CARTESIAN_POINT('Origin',(0.,9.95,0.)) ;
#133099=CARTESIAN_POINT('',(0.230887397576971,9.95,-1.91486057185377)) ;
#133100=CARTESIAN_POINT('Origin',(12.8,-2.3,2.54)) ;
#133101=CARTESIAN_POINT('',(12.8,-2.3359925337019,2.32404479778862)) ;
#133102=CARTESIAN_POINT('',(12.8,2.65,2.54)) ;
#133103=CARTESIAN_POINT('',(12.8,2.65,2.54)) ;
#133104=CARTESIAN_POINT('',(12.8,-2.2,2.54)) ;
#133105=CARTESIAN_POINT('',(12.8,-2.3,2.54)) ;
#133106=CARTESIAN_POINT('',(12.8,-2.2,1.96214168703486)) ;
#133107=CARTESIAN_POINT('',(12.8,-2.2,2.54)) ;
#133108=CARTESIAN_POINT('',(12.8,-2.24516129032258,1.83555190077454)) ;
#133109=CARTESIAN_POINT('Origin',(12.8,-2.4,1.96214168703486)) ;
#133110=CARTESIAN_POINT('',(12.8,-2.24516129032258,-1.83555190077454)) ;
#133111=CARTESIAN_POINT('Origin',(12.8,0.,0.)) ;
#133112=CARTESIAN_POINT('',(12.8,-2.2,-1.96214168703486)) ;
#133113=CARTESIAN_POINT('Origin',(12.8,-2.4,-1.96214168703486)) ;
#133114=CARTESIAN_POINT('',(12.8,-2.2,-3.11785831296514)) ;
#133115=CARTESIAN_POINT('',(12.8,-2.2,2.54)) ;
#133116=CARTESIAN_POINT('',(12.8,-2.24516129032258,-3.24444809922546)) ;
#133117=CARTESIAN_POINT('Origin',(12.8,-2.4,-3.11785831296514)) ;
#133118=CARTESIAN_POINT('',(12.8,-2.24516129032258,-6.91555190077455)) ;
#133119=CARTESIAN_POINT('Origin',(12.8,0.,-5.08)) ;
#133120=CARTESIAN_POINT('',(12.8,-2.2,-7.04214168703486)) ;
#133121=CARTESIAN_POINT('Origin',(12.8,-2.4,-7.04214168703486)) ;
#133122=CARTESIAN_POINT('',(12.8,-2.2,-7.62)) ;
#133123=CARTESIAN_POINT('',(12.8,-2.2,-2.54)) ;
#133124=CARTESIAN_POINT('',(12.8,2.65,-7.62)) ;
#133125=CARTESIAN_POINT('',(12.8,-2.3,-7.62)) ;
#133126=CARTESIAN_POINT('',(12.8,2.65,-2.54)) ;
#133127=CARTESIAN_POINT('',(12.8,2.13287979746107,-6.65923274259479)) ;
#133128=CARTESIAN_POINT('',(12.8,-1.51220874991811,-7.26674750049132)) ;
#133129=CARTESIAN_POINT('',(12.8,1.9,-6.46195395782836)) ;
#133130=CARTESIAN_POINT('Origin',(12.8,2.1,-6.46195395782836)) ;
#133131=CARTESIAN_POINT('',(12.8,1.9,-2.54)) ;
#133132=CARTESIAN_POINT('',(12.8,-2.3359925337019,-2.75595520221138)) ;
#133133=CARTESIAN_POINT('',(12.8,2.65,2.54)) ;
#133134=CARTESIAN_POINT('',(12.8,2.13287979746107,-1.57923274259479)) ;
#133135=CARTESIAN_POINT('',(12.8,-1.51220874991811,-2.18674750049132)) ;
#133136=CARTESIAN_POINT('',(12.8,1.9,-1.38195395782836)) ;
#133137=CARTESIAN_POINT('Origin',(12.8,2.1,-1.38195395782836)) ;
#133138=CARTESIAN_POINT('',(12.8,1.9,2.54)) ;
#133139=CARTESIAN_POINT('Origin',(12.8,2.75,2.54)) ;
#133140=CARTESIAN_POINT('',(4.55912712210513,2.75,1.49304604217164)) ;
#133141=CARTESIAN_POINT('',(12.8,2.75,1.49304604217164)) ;
#133142=CARTESIAN_POINT('',(4.55912712210514,2.75,2.54)) ;
#133143=CARTESIAN_POINT('',(4.55912712210514,2.75,2.54)) ;
#133144=CARTESIAN_POINT('',(12.7,2.75,2.54)) ;
#133145=CARTESIAN_POINT('',(12.8,2.75,2.54)) ;
#133146=CARTESIAN_POINT('',(12.7,2.75,2.54)) ;
#133147=CARTESIAN_POINT('Origin',(4.5,2.75,2.54)) ;
#133148=CARTESIAN_POINT('',(4.47150553123747,2.80180812502278,2.54)) ;
#133149=CARTESIAN_POINT('',(3.96237840913234,3.72749380157757,2.54)) ;
#133150=CARTESIAN_POINT('',(4.5,2.75,2.54)) ;
#133151=CARTESIAN_POINT('',(4.47150553123747,2.80180812502279,1.49304604217164)) ;
#133152=CARTESIAN_POINT('',(4.47150553123747,2.80180812502278,1.49304604217164)) ;
#133153=CARTESIAN_POINT('',(4.48762159086767,2.77250619842243,1.38882431825052)) ;
#133154=CARTESIAN_POINT('Origin',(4.56263299594614,2.63612182555249,1.48339970590384)) ;
#133155=CARTESIAN_POINT('',(4.48762159086767,2.77250619842243,-1.38882431824783)) ;
#133156=CARTESIAN_POINT('',(4.48762159086767,2.77250619842243,2.54)) ;
#133157=CARTESIAN_POINT('',(4.47150553123747,2.80180812502279,-1.49304604217164)) ;
#133158=CARTESIAN_POINT('Origin',(4.5626329959691,2.63612182551074,-1.48339970589483)) ;
#133159=CARTESIAN_POINT('',(4.47150553123747,2.80180812502279,-3.58695395782836)) ;
#133160=CARTESIAN_POINT('',(4.47150553123747,2.80180812502278,-2.54)) ;
#133161=CARTESIAN_POINT('',(4.48762159086767,2.77250619842243,-3.69117568174948)) ;
#133162=CARTESIAN_POINT('Origin',(4.56263299594449,2.63612182555554,-3.59660029409665)) ;
#133163=CARTESIAN_POINT('',(4.48762159086767,2.77250619842243,-6.46882431824783)) ;
#133164=CARTESIAN_POINT('',(4.48762159086767,2.77250619842243,-2.54)) ;
#133165=CARTESIAN_POINT('',(4.47150553123747,2.80180812502279,-6.57304604217164)) ;
#133166=CARTESIAN_POINT('Origin',(4.56263299596772,2.63612182551324,-6.56339970589523)) ;
#133167=CARTESIAN_POINT('',(4.47150553123747,2.80180812502278,-7.62)) ;
#133168=CARTESIAN_POINT('',(4.47150553123747,2.80180812502278,-7.62)) ;
#133169=CARTESIAN_POINT('',(3.96237840913234,3.72749380157757,-7.62)) ;
#133170=CARTESIAN_POINT('',(4.5,2.75,-7.62)) ;
#133171=CARTESIAN_POINT('',(3.96237840913234,3.72749380157757,2.54)) ;
#133172=CARTESIAN_POINT('Origin',(3.95,6.95,2.54)) ;
#133173=CARTESIAN_POINT('',(3.93762159086767,6.97250619842243,2.54)) ;
#133174=CARTESIAN_POINT('',(3.93762159086767,6.97250619842243,-7.62)) ;
#133175=CARTESIAN_POINT('',(3.93762159086767,6.97250619842243,2.54)) ;
#133176=CARTESIAN_POINT('',(3.95,6.95,-7.62)) ;
#133177=CARTESIAN_POINT('',(3.95,6.95,2.54)) ;
#133178=CARTESIAN_POINT('Origin',(3.4,9.95,2.54)) ;
#133179=CARTESIAN_POINT('',(3.4,10.85,-7.62)) ;
#133180=CARTESIAN_POINT('',(3.4,9.95,-7.62)) ;
#133181=CARTESIAN_POINT('',(3.4,10.85,2.54)) ;
#133182=CARTESIAN_POINT('',(3.4,10.85,2.54)) ;
#133183=CARTESIAN_POINT('',(3.4,9.95,2.54)) ;
#133184=CARTESIAN_POINT('',(3.4,10.05,2.04)) ;
#133185=CARTESIAN_POINT('Origin',(3.4,10.95,2.54)) ;
#133186=CARTESIAN_POINT('',(3.3,10.95,2.54)) ;
#133187=CARTESIAN_POINT('',(3.3,10.95,-7.62)) ;
#133188=CARTESIAN_POINT('',(3.3,10.95,2.54)) ;
#133189=CARTESIAN_POINT('',(-4.8,10.95,-7.62)) ;
#133190=CARTESIAN_POINT('',(3.4,10.95,-7.62)) ;
#133191=CARTESIAN_POINT('',(-4.8,10.95,2.54)) ;
#133192=CARTESIAN_POINT('',(-4.8,10.95,2.54)) ;
#133193=CARTESIAN_POINT('',(3.4,10.95,2.54)) ;
#133194=CARTESIAN_POINT('',(-2.55,10.95,-5.98)) ;
#133195=CARTESIAN_POINT('',(-2.75,10.95,-6.18)) ;
#133196=CARTESIAN_POINT('Origin',(-2.75,10.95,-5.98)) ;
#133197=CARTESIAN_POINT('',(-2.55,10.95,-4.18)) ;
#133198=CARTESIAN_POINT('',(-2.55,10.95,-2.54)) ;
#133199=CARTESIAN_POINT('',(-2.75,10.95,-3.98)) ;
#133200=CARTESIAN_POINT('Origin',(-2.75,10.95,-4.18)) ;
#133201=CARTESIAN_POINT('',(-3.8,10.95,-3.98)) ;
#133202=CARTESIAN_POINT('',(3.4,10.95,-3.98)) ;
#133203=CARTESIAN_POINT('',(-4.,10.95,-4.18)) ;
#133204=CARTESIAN_POINT('Origin',(-3.8,10.95,-4.18)) ;
#133205=CARTESIAN_POINT('',(-4.,10.95,-5.98)) ;
#133206=CARTESIAN_POINT('',(-4.,10.95,-2.54)) ;
#133207=CARTESIAN_POINT('',(-3.8,10.95,-6.18)) ;
#133208=CARTESIAN_POINT('Origin',(-3.8,10.95,-5.98)) ;
#133209=CARTESIAN_POINT('',(3.4,10.95,-6.18)) ;
#133210=CARTESIAN_POINT('',(-2.55,10.95,-0.900000000000001)) ;
#133211=CARTESIAN_POINT('',(-2.75,10.95,-1.1)) ;
#133212=CARTESIAN_POINT('Origin',(-2.75,10.95,-0.900000000000001)) ;
#133213=CARTESIAN_POINT('',(-2.55,10.95,0.899999999999999)) ;
#133214=CARTESIAN_POINT('',(-2.55,10.95,2.54)) ;
#133215=CARTESIAN_POINT('',(-2.75,10.95,1.1)) ;
#133216=CARTESIAN_POINT('Origin',(-2.75,10.95,0.899999999999999)) ;
#133217=CARTESIAN_POINT('',(-3.8,10.95,1.1)) ;
#133218=CARTESIAN_POINT('',(3.4,10.95,1.1)) ;
#133219=CARTESIAN_POINT('',(-4.,10.95,0.9)) ;
#133220=CARTESIAN_POINT('Origin',(-3.8,10.95,0.9)) ;
#133221=CARTESIAN_POINT('',(-4.,10.95,-0.9)) ;
#133222=CARTESIAN_POINT('',(-4.,10.95,2.54)) ;
#133223=CARTESIAN_POINT('',(-3.8,10.95,-1.1)) ;
#133224=CARTESIAN_POINT('Origin',(-3.8,10.95,-0.9)) ;
#133225=CARTESIAN_POINT('',(3.4,10.95,-1.1)) ;
#133226=CARTESIAN_POINT('Origin',(-4.9,10.95,2.54)) ;
#133227=CARTESIAN_POINT('',(-4.9,10.85,2.54)) ;
#133228=CARTESIAN_POINT('',(-4.9,10.85,-7.62)) ;
#133229=CARTESIAN_POINT('',(-4.9,10.85,2.54)) ;
#133230=CARTESIAN_POINT('',(-4.9,10.3,-7.62)) ;
#133231=CARTESIAN_POINT('',(-4.9,10.95,-7.62)) ;
#133232=CARTESIAN_POINT('',(-4.9,10.3,2.54)) ;
#133233=CARTESIAN_POINT('',(-4.9,10.3,2.54)) ;
#133234=CARTESIAN_POINT('',(-4.9,10.95,2.54)) ;
#133235=CARTESIAN_POINT('Origin',(-4.9,10.2,2.54)) ;
#133236=CARTESIAN_POINT('',(-4.8,10.2,2.54)) ;
#133237=CARTESIAN_POINT('',(-4.8,10.2,-7.62)) ;
#133238=CARTESIAN_POINT('',(-4.8,10.2,2.54)) ;
#133239=CARTESIAN_POINT('',(-4.9,10.2,-7.62)) ;
#133240=CARTESIAN_POINT('',(-4.9,10.2,2.54)) ;
#133241=CARTESIAN_POINT('Origin',(-4.4,10.2,2.54)) ;
#133242=CARTESIAN_POINT('',(-5.39805806756909,5.20970966215454,-7.62)) ;
#133243=CARTESIAN_POINT('',(-4.4,10.2,-7.62)) ;
#133244=CARTESIAN_POINT('',(-5.39805806756909,5.20970966215454,2.54)) ;
#133245=CARTESIAN_POINT('',(-5.39805806756909,5.20970966215454,2.54)) ;
#133246=CARTESIAN_POINT('',(-4.4,10.2,2.54)) ;
#133247=CARTESIAN_POINT('Origin',(-5.4,5.2,2.54)) ;
#133248=CARTESIAN_POINT('',(-5.4,5.19009804864072,2.54)) ;
#133249=CARTESIAN_POINT('',(-5.4,5.19009804864072,-7.62)) ;
#133250=CARTESIAN_POINT('',(-5.4,5.19009804864072,2.54)) ;
#133251=CARTESIAN_POINT('',(-5.4,-3.95,-7.62)) ;
#133252=CARTESIAN_POINT('',(-5.4,5.2,-7.62)) ;
#133253=CARTESIAN_POINT('',(-5.4,-3.95,2.54)) ;
#133254=CARTESIAN_POINT('',(-5.4,-3.95,2.54)) ;
#133255=CARTESIAN_POINT('',(-5.4,5.2,2.54)) ;
#133256=CARTESIAN_POINT('',(-5.4,4.23801993223491,-6.98)) ;
#133257=CARTESIAN_POINT('',(-5.4,4.23801993223491,-3.18)) ;
#133258=CARTESIAN_POINT('',(-5.4,4.23801993223491,-3.08)) ;
#133259=CARTESIAN_POINT('',(-5.4,3.9369800677651,-2.98)) ;
#133260=CARTESIAN_POINT('Ctrl Pts',(-5.4,4.23801993223491,-3.18)) ;
#133261=CARTESIAN_POINT('Ctrl Pts',(-5.4,4.23801992976516,-3.12749312809026)) ;
#133262=CARTESIAN_POINT('Ctrl Pts',(-5.4,4.20557579169425,-3.07560257376825)) ;
#133263=CARTESIAN_POINT('Ctrl Pts',(-5.4,4.09411900298411,-3.00155471375713)) ;
#133264=CARTESIAN_POINT('Ctrl Pts',(-5.4,4.0160133758189,-2.98000000048114)) ;
#133265=CARTESIAN_POINT('Ctrl Pts',(-5.4,3.9369800677651,-2.98)) ;
#133266=CARTESIAN_POINT('',(-5.4,-1.88819660112502,-2.98)) ;
#133267=CARTESIAN_POINT('',(-5.4,-2.05,-2.98)) ;
#133268=CARTESIAN_POINT('',(-5.4,-2.11180339887499,-3.18)) ;
#133269=CARTESIAN_POINT('Ctrl Pts',(-5.4,-2.11180339887499,-3.18)) ;
#133270=CARTESIAN_POINT('Ctrl Pts',(-5.4,-2.11180339704051,-3.12749316010866)) ;
#133271=CARTESIAN_POINT('Ctrl Pts',(-5.4,-2.0877044485962,-3.07560253112148)) ;
#133272=CARTESIAN_POINT('Ctrl Pts',(-5.4,-2.00491651967066,-3.0015547564039)) ;
#133273=CARTESIAN_POINT('Ctrl Pts',(-5.4,-1.946901032774,-2.98000000117411)) ;
#133274=CARTESIAN_POINT('Ctrl Pts',(-5.4,-1.88819660112502,-2.98)) ;
#133275=CARTESIAN_POINT('',(-5.4,-2.11180339887499,-6.98)) ;
#133276=CARTESIAN_POINT('',(-5.4,-2.11180339887499,-7.08)) ;
#133277=CARTESIAN_POINT('',(-5.4,-1.88819660112501,-7.18)) ;
#133278=CARTESIAN_POINT('Ctrl Pts',(-5.4,-1.88819660112501,-7.18)) ;
#133279=CARTESIAN_POINT('Ctrl Pts',(-5.4,-1.946901032774,-7.17999999882592)) ;
#133280=CARTESIAN_POINT('Ctrl Pts',(-5.4,-2.00491651967066,-7.1584452435961)) ;
#133281=CARTESIAN_POINT('Ctrl Pts',(-5.4,-2.0877044485962,-7.08439746887852)) ;
#133282=CARTESIAN_POINT('Ctrl Pts',(-5.4,-2.11180339704051,-7.03250683989134)) ;
#133283=CARTESIAN_POINT('Ctrl Pts',(-5.4,-2.11180339887499,-6.98)) ;
#133284=CARTESIAN_POINT('',(-5.4,3.9369800677651,-7.18)) ;
#133285=CARTESIAN_POINT('',(-5.4,4.20000000000001,-7.18)) ;
#133286=CARTESIAN_POINT('Ctrl Pts',(-5.4,3.9369800677651,-7.18)) ;
#133287=CARTESIAN_POINT('Ctrl Pts',(-5.4,4.01601337581889,-7.17999999951891)) ;
#133288=CARTESIAN_POINT('Ctrl Pts',(-5.4,4.09411900298413,-7.15844528624287)) ;
#133289=CARTESIAN_POINT('Ctrl Pts',(-5.4,4.20557579169423,-7.08439742623175)) ;
#133290=CARTESIAN_POINT('Ctrl Pts',(-5.4,4.23801992976516,-7.03250687190974)) ;
#133291=CARTESIAN_POINT('Ctrl Pts',(-5.4,4.23801993223491,-6.98)) ;
#133292=CARTESIAN_POINT('',(-5.4,4.23801993223491,-1.9)) ;
#133293=CARTESIAN_POINT('',(-5.4,4.23801993223491,1.9)) ;
#133294=CARTESIAN_POINT('',(-5.4,4.23801993223491,2.)) ;
#133295=CARTESIAN_POINT('',(-5.4,3.9369800677651,2.1)) ;
#133296=CARTESIAN_POINT('Ctrl Pts',(-5.4,4.23801993223491,1.9)) ;
#133297=CARTESIAN_POINT('Ctrl Pts',(-5.4,4.23801992976516,1.95250687190974)) ;
#133298=CARTESIAN_POINT('Ctrl Pts',(-5.4,4.20557579169425,2.00439742623175)) ;
#133299=CARTESIAN_POINT('Ctrl Pts',(-5.4,4.09411900298411,2.07844528624287)) ;
#133300=CARTESIAN_POINT('Ctrl Pts',(-5.4,4.01601337581891,2.09999999951886)) ;
#133301=CARTESIAN_POINT('Ctrl Pts',(-5.4,3.9369800677651,2.1)) ;
#133302=CARTESIAN_POINT('',(-5.4,-1.88819660112502,2.1)) ;
#133303=CARTESIAN_POINT('',(-5.4,-2.05,2.1)) ;
#133304=CARTESIAN_POINT('',(-5.4,-2.11180339887499,1.9)) ;
#133305=CARTESIAN_POINT('Ctrl Pts',(-5.4,-2.11180339887499,1.9)) ;
#133306=CARTESIAN_POINT('Ctrl Pts',(-5.4,-2.11180339704051,1.95250683989134)) ;
#133307=CARTESIAN_POINT('Ctrl Pts',(-5.4,-2.0877044485962,2.00439746887852)) ;
#133308=CARTESIAN_POINT('Ctrl Pts',(-5.4,-2.00491651967066,2.0784452435961)) ;
#133309=CARTESIAN_POINT('Ctrl Pts',(-5.4,-1.946901032774,2.09999999882593)) ;
#133310=CARTESIAN_POINT('Ctrl Pts',(-5.4,-1.88819660112502,2.1)) ;
#133311=CARTESIAN_POINT('',(-5.4,-2.11180339887499,-1.9)) ;
#133312=CARTESIAN_POINT('',(-5.4,-2.11180339887499,-2.)) ;
#133313=CARTESIAN_POINT('',(-5.4,-1.88819660112501,-2.1)) ;
#133314=CARTESIAN_POINT('Ctrl Pts',(-5.4,-1.88819660112501,-2.1)) ;
#133315=CARTESIAN_POINT('Ctrl Pts',(-5.4,-1.946901032774,-2.09999999882593)) ;
#133316=CARTESIAN_POINT('Ctrl Pts',(-5.4,-2.00491651967066,-2.07844524359609)) ;
#133317=CARTESIAN_POINT('Ctrl Pts',(-5.4,-2.0877044485962,-2.00439746887853)) ;
#133318=CARTESIAN_POINT('Ctrl Pts',(-5.4,-2.11180339704051,-1.95250683989133)) ;
#133319=CARTESIAN_POINT('Ctrl Pts',(-5.4,-2.11180339887499,-1.9)) ;
#133320=CARTESIAN_POINT('',(-5.4,3.9369800677651,-2.1)) ;
#133321=CARTESIAN_POINT('',(-5.4,4.20000000000001,-2.1)) ;
#133322=CARTESIAN_POINT('Ctrl Pts',(-5.4,3.9369800677651,-2.1)) ;
#133323=CARTESIAN_POINT('Ctrl Pts',(-5.4,4.01601337581889,-2.09999999951886)) ;
#133324=CARTESIAN_POINT('Ctrl Pts',(-5.4,4.09411900298413,-2.07844528624287)) ;
#133325=CARTESIAN_POINT('Ctrl Pts',(-5.4,4.20557579169423,-2.00439742623175)) ;
#133326=CARTESIAN_POINT('Ctrl Pts',(-5.4,4.23801992976516,-1.95250687190974)) ;
#133327=CARTESIAN_POINT('Ctrl Pts',(-5.4,4.23801993223491,-1.9)) ;
#133328=CARTESIAN_POINT('Origin',(-5.4,-4.05,2.54)) ;
#133329=CARTESIAN_POINT('',(-5.3,-4.05,2.54)) ;
#133330=CARTESIAN_POINT('',(-5.3,-4.05,-7.62)) ;
#133331=CARTESIAN_POINT('',(-5.3,-4.05,2.54)) ;
#133332=CARTESIAN_POINT('',(3.5,-4.05,-7.62)) ;
#133333=CARTESIAN_POINT('',(-5.4,-4.05,-7.62)) ;
#133334=CARTESIAN_POINT('',(3.5,-4.05,2.54)) ;
#133335=CARTESIAN_POINT('',(3.5,-4.05,2.54)) ;
#133336=CARTESIAN_POINT('',(-5.4,-4.05,2.54)) ;
#133337=CARTESIAN_POINT('',(-4.5,-4.05,-5.98)) ;
#133338=CARTESIAN_POINT('',(-4.3,-4.05,-6.18)) ;
#133339=CARTESIAN_POINT('Origin',(-4.3,-4.05,-5.98)) ;
#133340=CARTESIAN_POINT('',(-4.5,-4.05,-4.18)) ;
#133341=CARTESIAN_POINT('',(-4.5,-4.05,-2.54)) ;
#133342=CARTESIAN_POINT('',(-4.3,-4.05,-3.98)) ;
#133343=CARTESIAN_POINT('Origin',(-4.3,-4.05,-4.18)) ;
#133344=CARTESIAN_POINT('',(-3.25,-4.05,-3.98)) ;
#133345=CARTESIAN_POINT('',(-5.4,-4.05,-3.98)) ;
#133346=CARTESIAN_POINT('',(-3.05,-4.05,-4.18)) ;
#133347=CARTESIAN_POINT('Origin',(-3.25,-4.05,-4.18)) ;
#133348=CARTESIAN_POINT('',(-3.05,-4.05,-5.98)) ;
#133349=CARTESIAN_POINT('',(-3.05,-4.05,-2.54)) ;
#133350=CARTESIAN_POINT('',(-3.25,-4.05,-6.18)) ;
#133351=CARTESIAN_POINT('Origin',(-3.25,-4.05,-5.98)) ;
#133352=CARTESIAN_POINT('',(-5.4,-4.05,-6.18)) ;
#133353=CARTESIAN_POINT('',(-4.5,-4.05,-0.900000000000001)) ;
#133354=CARTESIAN_POINT('',(-4.3,-4.05,-1.1)) ;
#133355=CARTESIAN_POINT('Origin',(-4.3,-4.05,-0.900000000000001)) ;
#133356=CARTESIAN_POINT('',(-4.5,-4.05,0.899999999999999)) ;
#133357=CARTESIAN_POINT('',(-4.5,-4.05,2.54)) ;
#133358=CARTESIAN_POINT('',(-4.3,-4.05,1.1)) ;
#133359=CARTESIAN_POINT('Origin',(-4.3,-4.05,0.899999999999999)) ;
#133360=CARTESIAN_POINT('',(-3.25,-4.05,1.1)) ;
#133361=CARTESIAN_POINT('',(-5.4,-4.05,1.1)) ;
#133362=CARTESIAN_POINT('',(-3.05,-4.05,0.9)) ;
#133363=CARTESIAN_POINT('Origin',(-3.25,-4.05,0.9)) ;
#133364=CARTESIAN_POINT('',(-3.05,-4.05,-0.900000000000001)) ;
#133365=CARTESIAN_POINT('',(-3.05,-4.05,2.54)) ;
#133366=CARTESIAN_POINT('',(-3.25,-4.05,-1.1)) ;
#133367=CARTESIAN_POINT('Origin',(-3.25,-4.05,-0.900000000000001)) ;
#133368=CARTESIAN_POINT('',(-5.4,-4.05,-1.1)) ;
#133369=CARTESIAN_POINT('Origin',(3.6,-4.05,2.54)) ;
#133370=CARTESIAN_POINT('',(3.6,-3.95,2.54)) ;
#133371=CARTESIAN_POINT('',(3.6,-3.95,-7.62)) ;
#133372=CARTESIAN_POINT('',(3.6,-3.95,2.54)) ;
#133373=CARTESIAN_POINT('',(3.6,-2.9,-7.62)) ;
#133374=CARTESIAN_POINT('',(3.6,-4.05,-7.62)) ;
#133375=CARTESIAN_POINT('',(3.6,-2.9,2.54)) ;
#133376=CARTESIAN_POINT('',(3.6,-2.9,2.54)) ;
#133377=CARTESIAN_POINT('',(3.6,-4.05,2.54)) ;
#133378=CARTESIAN_POINT('Origin',(3.6,-2.8,2.54)) ;
#133379=CARTESIAN_POINT('',(4.4,-2.8,-1.52315462117279)) ;
#133380=CARTESIAN_POINT('',(4.54880051362943,-2.79999999972164,-1.07643786073294)) ;
#133381=CARTESIAN_POINT('Ctrl Pts',(4.4,-2.8,-1.52315462117279)) ;
#133382=CARTESIAN_POINT('Ctrl Pts',(4.40001102013632,-2.8,-1.48644001985269)) ;
#133383=CARTESIAN_POINT('Ctrl Pts',(4.40220140384615,-2.79999999812164,
-1.45006816610693)) ;
#133384=CARTESIAN_POINT('Ctrl Pts',(4.40664174993564,-2.79999999722267,
-1.41407273800855)) ;
#133385=CARTESIAN_POINT('Ctrl Pts',(4.41108209602513,-2.79999999632371,
-1.37807730991017)) ;
#133386=CARTESIAN_POINT('Ctrl Pts',(4.41777240449452,-2.79999999692353,
-1.34245830745924)) ;
#133387=CARTESIAN_POINT('Ctrl Pts',(4.42678327414915,-2.79999999844302,
-1.30724940872871)) ;
#133388=CARTESIAN_POINT('Ctrl Pts',(4.42864654534902,-2.79999999875722,
-1.29996889868936)) ;
#133389=CARTESIAN_POINT('Ctrl Pts',(4.43060908636007,-2.79999999907333,
-1.29270591711623)) ;
#133390=CARTESIAN_POINT('Ctrl Pts',(4.43267155768737,-2.79999999933982,
-1.28546075906515)) ;
#133391=CARTESIAN_POINT('Ctrl Pts',(4.4352900037877,-2.79999999967816,-1.27626254350986)) ;
#133392=CARTESIAN_POINT('Ctrl Pts',(4.4380733085653,-2.79999999966608,-1.2670911025424)) ;
#133393=CARTESIAN_POINT('Ctrl Pts',(4.44102157277561,-2.79999999954234,
-1.25794807820152)) ;
#133394=CARTESIAN_POINT('Ctrl Pts',(4.45046499569138,-2.79999999914597,
-1.22866255986902)) ;
#133395=CARTESIAN_POINT('Ctrl Pts',(4.46157908226632,-2.79999999505379,
-1.19972021349317)) ;
#133396=CARTESIAN_POINT('Ctrl Pts',(4.47540732315415,-2.79999999166095,
-1.1722492625065)) ;
#133397=CARTESIAN_POINT('Ctrl Pts',(4.47702479055525,-2.79999999126409,
-1.16903602894638)) ;
#133398=CARTESIAN_POINT('Ctrl Pts',(4.47867903313992,-2.79999999107055,
-1.16584272212549)) ;
#133399=CARTESIAN_POINT('Ctrl Pts',(4.48037187481471,-2.79999999105954,
-1.162671097194)) ;
#133400=CARTESIAN_POINT('Ctrl Pts',(4.48545039983908,-2.79999999102651,
-1.15315622239953)) ;
#133401=CARTESIAN_POINT('Ctrl Pts',(4.49087631667453,-2.79999999265304,
-1.14383648460966)) ;
#133402=CARTESIAN_POINT('Ctrl Pts',(4.49669887079745,-2.79999999431461,
-1.13475927287888)) ;
#133403=CARTESIAN_POINT('Ctrl Pts',(4.50888705006189,-2.79999999779274,
-1.11575821570355)) ;
#133404=CARTESIAN_POINT('Ctrl Pts',(4.52313265843748,-2.79999999982394,
-1.09737449917999)) ;
#133405=CARTESIAN_POINT('Ctrl Pts',(4.54066913339539,-2.79999999997241,
-1.08273042197106)) ;
#133406=CARTESIAN_POINT('Ctrl Pts',(4.54329026609835,-2.7999999999946,-1.08054160866798)) ;
#133407=CARTESIAN_POINT('Ctrl Pts',(4.5460045281952,-2.8,-1.07843934457872)) ;
#133408=CARTESIAN_POINT('Ctrl Pts',(4.54880363749516,-2.8,-1.07645020604105)) ;
#133409=CARTESIAN_POINT('',(4.4,-2.8,-3.84865454255039E-12)) ;
#133410=CARTESIAN_POINT('Ctrl Pts',(4.54879236168152,-2.8,-1.07643444348001)) ;
#133411=CARTESIAN_POINT('Ctrl Pts',(4.51096310105345,-2.8,-1.04764090781959)) ;
#133412=CARTESIAN_POINT('Ctrl Pts',(4.49022331291407,-2.8,-1.00382911927614)) ;
#133413=CARTESIAN_POINT('Ctrl Pts',(4.45698031182017,-2.8,-0.917623871395766)) ;
#133414=CARTESIAN_POINT('Ctrl Pts',(4.44561000227039,-2.8,-0.872361144958552)) ;
#133415=CARTESIAN_POINT('Ctrl Pts',(4.41911102299977,-2.8,-0.735880791656898)) ;
#133416=CARTESIAN_POINT('Ctrl Pts',(4.41155688769424,-2.8,-0.644231375192043)) ;
#133417=CARTESIAN_POINT('Ctrl Pts',(4.39763503647248,-2.8,-0.368710456932986)) ;
#133418=CARTESIAN_POINT('Ctrl Pts',(4.4,-2.8,-0.184260662117819)) ;
#133419=CARTESIAN_POINT('Ctrl Pts',(4.4,-2.8,-3.84865454255039E-12)) ;
#133420=CARTESIAN_POINT('',(4.54879236179094,-2.79999999953044,1.07643444349586)) ;
#133421=CARTESIAN_POINT('Ctrl Pts',(4.4,-2.8,-3.84865750380219E-12)) ;
#133422=CARTESIAN_POINT('Ctrl Pts',(4.4,-2.8,0.184515281657094)) ;
#133423=CARTESIAN_POINT('Ctrl Pts',(4.39760751905643,-2.8,0.369216326714866)) ;
#133424=CARTESIAN_POINT('Ctrl Pts',(4.40696794948104,-2.8,0.553410676296662)) ;
#133425=CARTESIAN_POINT('Ctrl Pts',(4.41164816469334,-2.8,0.645507851087552)) ;
#133426=CARTESIAN_POINT('Ctrl Pts',(4.41940496802384,-2.80000000000001,
0.737842856499212)) ;
#133427=CARTESIAN_POINT('Ctrl Pts',(4.43698455094237,-2.8,0.827933846251606)) ;
#133428=CARTESIAN_POINT('Ctrl Pts',(4.44577434240165,-2.8,0.872979341127799)) ;
#133429=CARTESIAN_POINT('Ctrl Pts',(4.456925956929,-2.80000000000001,0.917523082510354)) ;
#133430=CARTESIAN_POINT('Ctrl Pts',(4.47366127850408,-2.8,0.960880593909591)) ;
#133431=CARTESIAN_POINT('Ctrl Pts',(4.47575319370098,-2.8,0.966300282834483)) ;
#133432=CARTESIAN_POINT('Ctrl Pts',(4.4779117359051,-2.79999999997843,0.971725845219423)) ;
#133433=CARTESIAN_POINT('Ctrl Pts',(4.48016062485991,-2.80000000010461,
0.977126712477952)) ;
#133434=CARTESIAN_POINT('Ctrl Pts',(4.48803173620173,-2.80000000054624,
0.996029747882805)) ;
#133435=CARTESIAN_POINT('Ctrl Pts',(4.49700942865457,-2.80000000534986,
1.01463033418563)) ;
#133436=CARTESIAN_POINT('Ctrl Pts',(4.50810946414921,-2.80000000469598,
1.03161833486068)) ;
#133437=CARTESIAN_POINT('Ctrl Pts',(4.51435323411495,-2.80000000432818,
1.04117408524039)) ;
#133438=CARTESIAN_POINT('Ctrl Pts',(4.52126852668377,-2.80000000204489,
1.05021960344861)) ;
#133439=CARTESIAN_POINT('Ctrl Pts',(4.52903612565461,-2.80000000089509,
1.05852171333236)) ;
#133440=CARTESIAN_POINT('Ctrl Pts',(4.5320568585877,-2.80000000044794,1.06175031162049)) ;
#133441=CARTESIAN_POINT('Ctrl Pts',(4.53520648971123,-2.80000000018876,
1.06486648087189)) ;
#133442=CARTESIAN_POINT('Ctrl Pts',(4.53849565154302,-2.80000000008376,
1.06785650719406)) ;
#133443=CARTESIAN_POINT('Ctrl Pts',(4.54178481337482,-2.79999999997876,
1.07084653351624)) ;
#133444=CARTESIAN_POINT('Ctrl Pts',(4.54521363891046,-2.8,1.07371024217815)) ;
#133445=CARTESIAN_POINT('Ctrl Pts',(4.54879236168087,-2.8,1.07643444348047)) ;
#133446=CARTESIAN_POINT('',(4.4,-2.8,1.52315462117279)) ;
#133447=CARTESIAN_POINT('Ctrl Pts',(4.54879236168109,-2.79999999812176,
1.07643444348078)) ;
#133448=CARTESIAN_POINT('Ctrl Pts',(4.54599316991904,-2.79999999835896,
1.07842438566453)) ;
#133449=CARTESIAN_POINT('Ctrl Pts',(4.54327885465675,-2.7999999985882,1.08052734316011)) ;
#133450=CARTESIAN_POINT('Ctrl Pts',(4.523116040633,-2.80000000023132,1.09736894030692)) ;
#133451=CARTESIAN_POINT('Ctrl Pts',(4.50886780632328,-2.80000000100533,
1.11575780035687)) ;
#133452=CARTESIAN_POINT('Ctrl Pts',(4.48892103801304,-2.79999999510252,
1.14687097816957)) ;
#133453=CARTESIAN_POINT('Ctrl Pts',(4.4818652331329,-2.7999999909955,1.1594167949763)) ;
#133454=CARTESIAN_POINT('Ctrl Pts',(4.46162186753408,-2.79999997126272,
1.19974328605816)) ;
#133455=CARTESIAN_POINT('Ctrl Pts',(4.45052849087262,-2.7999999685384,1.2286810382908)) ;
#133456=CARTESIAN_POINT('Ctrl Pts',(4.43813540717735,-2.79999997674815,
1.2670939408709)) ;
#133457=CARTESIAN_POINT('Ctrl Pts',(4.43535270120343,-2.79999997903695,
1.27624973594923)) ;
#133458=CARTESIAN_POINT('Ctrl Pts',(4.41677772588063,-2.79999999273252,
1.34133119849698)) ;
#133459=CARTESIAN_POINT('Ctrl Pts',(4.40678488791375,-2.79999999887621,
1.39828048147345)) ;
#133460=CARTESIAN_POINT('Ctrl Pts',(4.40081887576623,-2.80000000006435,
1.47838010320481)) ;
#133461=CARTESIAN_POINT('Ctrl Pts',(4.4,-2.8,1.50069810180457)) ;
#133462=CARTESIAN_POINT('Ctrl Pts',(4.4,-2.8,1.52315462117279)) ;
#133463=CARTESIAN_POINT('',(4.4,-2.8,2.54)) ;
#133464=CARTESIAN_POINT('',(4.4,-2.8,2.54)) ;
#133465=CARTESIAN_POINT('',(3.7,-2.8,2.54)) ;
#133466=CARTESIAN_POINT('',(3.6,-2.8,2.54)) ;
#133467=CARTESIAN_POINT('',(3.7,-2.8,-7.62)) ;
#133468=CARTESIAN_POINT('',(3.7,-2.8,-2.54)) ;
#133469=CARTESIAN_POINT('',(4.4,-2.8,-7.62)) ;
#133470=CARTESIAN_POINT('',(3.6,-2.8,-7.62)) ;
#133471=CARTESIAN_POINT('',(4.4,-2.8,-6.60315462117279)) ;
#133472=CARTESIAN_POINT('',(4.4,-2.8,-2.54)) ;
#133473=CARTESIAN_POINT('',(4.54880051362943,-2.79999999972164,-6.15643786073294)) ;
#133474=CARTESIAN_POINT('Ctrl Pts',(4.4,-2.8,-6.60315462117279)) ;
#133475=CARTESIAN_POINT('Ctrl Pts',(4.40001102013632,-2.8,-6.56644001985245)) ;
#133476=CARTESIAN_POINT('Ctrl Pts',(4.40220140384618,-2.79999999812164,
-6.53006816610646)) ;
#133477=CARTESIAN_POINT('Ctrl Pts',(4.40664174993573,-2.79999999722267,
-6.49407273800786)) ;
#133478=CARTESIAN_POINT('Ctrl Pts',(4.41108209602527,-2.79999999632371,
-6.45807730990925)) ;
#133479=CARTESIAN_POINT('Ctrl Pts',(4.41777240449475,-2.79999999692353,
-6.42245830745811)) ;
#133480=CARTESIAN_POINT('Ctrl Pts',(4.4267832741495,-2.79999999844302,-6.38724940872736)) ;
#133481=CARTESIAN_POINT('Ctrl Pts',(4.42864654534927,-2.79999999875722,
-6.37996889868846)) ;
#133482=CARTESIAN_POINT('Ctrl Pts',(4.4306090863602,-2.79999999907333,-6.37270591711578)) ;
#133483=CARTESIAN_POINT('Ctrl Pts',(4.43267155768737,-2.79999999933982,
-6.36546075906515)) ;
#133484=CARTESIAN_POINT('Ctrl Pts',(4.4352900037877,-2.79999999967816,-6.35626254350987)) ;
#133485=CARTESIAN_POINT('Ctrl Pts',(4.4380733085653,-2.79999999966609,-6.3470911025424)) ;
#133486=CARTESIAN_POINT('Ctrl Pts',(4.44102157277561,-2.79999999954234,
-6.33794807820151)) ;
#133487=CARTESIAN_POINT('Ctrl Pts',(4.45046499569138,-2.79999999914597,
-6.30866255986902)) ;
#133488=CARTESIAN_POINT('Ctrl Pts',(4.46157908226632,-2.79999999505379,
-6.27972021349316)) ;
#133489=CARTESIAN_POINT('Ctrl Pts',(4.47540732315415,-2.79999999166095,
-6.2522492625065)) ;
#133490=CARTESIAN_POINT('Ctrl Pts',(4.47702479055525,-2.79999999126409,
-6.24903602894638)) ;
#133491=CARTESIAN_POINT('Ctrl Pts',(4.47867903313992,-2.79999999107055,
-6.24584272212549)) ;
#133492=CARTESIAN_POINT('Ctrl Pts',(4.48037187481471,-2.79999999105954,
-6.242671097194)) ;
#133493=CARTESIAN_POINT('Ctrl Pts',(4.48545039983908,-2.79999999102651,
-6.23315622239953)) ;
#133494=CARTESIAN_POINT('Ctrl Pts',(4.49087631667453,-2.79999999265304,
-6.22383648460966)) ;
#133495=CARTESIAN_POINT('Ctrl Pts',(4.49669887079746,-2.79999999431461,
-6.21475927287888)) ;
#133496=CARTESIAN_POINT('Ctrl Pts',(4.50888705006191,-2.79999999779274,
-6.19575821570356)) ;
#133497=CARTESIAN_POINT('Ctrl Pts',(4.52313265843748,-2.79999999982394,
-6.17737449917998)) ;
#133498=CARTESIAN_POINT('Ctrl Pts',(4.54066913339539,-2.79999999997241,
-6.16273042197107)) ;
#133499=CARTESIAN_POINT('Ctrl Pts',(4.54329026609835,-2.79999999999461,
-6.16054160866799)) ;
#133500=CARTESIAN_POINT('Ctrl Pts',(4.5460045281952,-2.8,-6.15843934457872)) ;
#133501=CARTESIAN_POINT('Ctrl Pts',(4.54880363749516,-2.8,-6.15645020604105)) ;
#133502=CARTESIAN_POINT('',(4.4,-2.8,-5.08000000000385)) ;
#133503=CARTESIAN_POINT('Ctrl Pts',(4.54879236168152,-2.8,-6.15643444348001)) ;
#133504=CARTESIAN_POINT('Ctrl Pts',(4.51096310105345,-2.8,-6.1276409078196)) ;
#133505=CARTESIAN_POINT('Ctrl Pts',(4.49022331291407,-2.8,-6.08382911927614)) ;
#133506=CARTESIAN_POINT('Ctrl Pts',(4.45698031182017,-2.8,-5.99762387139577)) ;
#133507=CARTESIAN_POINT('Ctrl Pts',(4.4456100022704,-2.8,-5.95236114495855)) ;
#133508=CARTESIAN_POINT('Ctrl Pts',(4.41911102299977,-2.8,-5.8158807916569)) ;
#133509=CARTESIAN_POINT('Ctrl Pts',(4.41155688769424,-2.8,-5.72423137519204)) ;
#133510=CARTESIAN_POINT('Ctrl Pts',(4.39763503647248,-2.8,-5.44871045693299)) ;
#133511=CARTESIAN_POINT('Ctrl Pts',(4.4,-2.8,-5.26426066211782)) ;
#133512=CARTESIAN_POINT('Ctrl Pts',(4.4,-2.8,-5.08000000000385)) ;
#133513=CARTESIAN_POINT('',(4.54879236179094,-2.79999999953044,-4.00356555650414)) ;
#133514=CARTESIAN_POINT('Ctrl Pts',(4.4,-2.8,-5.08000000000385)) ;
#133515=CARTESIAN_POINT('Ctrl Pts',(4.4,-2.8,-4.89548471834291)) ;
#133516=CARTESIAN_POINT('Ctrl Pts',(4.39760751905643,-2.8,-4.71078367328513)) ;
#133517=CARTESIAN_POINT('Ctrl Pts',(4.40696794948104,-2.8,-4.52658932370334)) ;
#133518=CARTESIAN_POINT('Ctrl Pts',(4.41164816469334,-2.8,-4.43449214891245)) ;
#133519=CARTESIAN_POINT('Ctrl Pts',(4.41940496802384,-2.80000000000001,
-4.34215714350079)) ;
#133520=CARTESIAN_POINT('Ctrl Pts',(4.43698455094237,-2.8,-4.2520661537484)) ;
#133521=CARTESIAN_POINT('Ctrl Pts',(4.44577434240163,-2.8,-4.2070206588722)) ;
#133522=CARTESIAN_POINT('Ctrl Pts',(4.456925956929,-2.80000000000001,-4.16247691748965)) ;
#133523=CARTESIAN_POINT('Ctrl Pts',(4.47366127850408,-2.8,-4.11911940609041)) ;
#133524=CARTESIAN_POINT('Ctrl Pts',(4.47575319370098,-2.8,-4.11369971716551)) ;
#133525=CARTESIAN_POINT('Ctrl Pts',(4.47791173590511,-2.79999999997843,
-4.10827415478058)) ;
#133526=CARTESIAN_POINT('Ctrl Pts',(4.48016062485992,-2.80000000010461,
-4.10287328752205)) ;
#133527=CARTESIAN_POINT('Ctrl Pts',(4.48803173620173,-2.80000000054624,
-4.08397025211719)) ;
#133528=CARTESIAN_POINT('Ctrl Pts',(4.49700942865457,-2.80000000534986,
-4.06536966581437)) ;
#133529=CARTESIAN_POINT('Ctrl Pts',(4.50810946414922,-2.80000000469598,
-4.04838166513932)) ;
#133530=CARTESIAN_POINT('Ctrl Pts',(4.51435323411496,-2.80000000432818,
-4.03882591475961)) ;
#133531=CARTESIAN_POINT('Ctrl Pts',(4.52126852668377,-2.80000000204489,
-4.02978039655139)) ;
#133532=CARTESIAN_POINT('Ctrl Pts',(4.5290361256546,-2.80000000089509,-4.02147828666764)) ;
#133533=CARTESIAN_POINT('Ctrl Pts',(4.5320568585877,-2.80000000044794,-4.01824968837951)) ;
#133534=CARTESIAN_POINT('Ctrl Pts',(4.53520648971123,-2.80000000018876,
-4.01513351912811)) ;
#133535=CARTESIAN_POINT('Ctrl Pts',(4.53849565154302,-2.80000000008376,
-4.01214349280594)) ;
#133536=CARTESIAN_POINT('Ctrl Pts',(4.54178481337482,-2.79999999997876,
-4.00915346648376)) ;
#133537=CARTESIAN_POINT('Ctrl Pts',(4.54521363891047,-2.8,-4.00628975782185)) ;
#133538=CARTESIAN_POINT('Ctrl Pts',(4.54879236168087,-2.8,-4.00356555651953)) ;
#133539=CARTESIAN_POINT('',(4.4,-2.8,-3.55684537882721)) ;
#133540=CARTESIAN_POINT('Ctrl Pts',(4.54879236168109,-2.79999999812176,
-4.00356555651922)) ;
#133541=CARTESIAN_POINT('Ctrl Pts',(4.54599316991904,-2.79999999835896,
-4.00157561433547)) ;
#133542=CARTESIAN_POINT('Ctrl Pts',(4.54327885465675,-2.7999999985882,-3.99947265683989)) ;
#133543=CARTESIAN_POINT('Ctrl Pts',(4.523116040633,-2.80000000023133,-3.98263105969307)) ;
#133544=CARTESIAN_POINT('Ctrl Pts',(4.50886780632328,-2.80000000100533,
-3.96424219964312)) ;
#133545=CARTESIAN_POINT('Ctrl Pts',(4.48892103801304,-2.79999999510252,
-3.93312902183043)) ;
#133546=CARTESIAN_POINT('Ctrl Pts',(4.4818652331329,-2.7999999909955,-3.9205832050237)) ;
#133547=CARTESIAN_POINT('Ctrl Pts',(4.46162186753408,-2.79999997126272,
-3.88025671394184)) ;
#133548=CARTESIAN_POINT('Ctrl Pts',(4.45052849087262,-2.7999999685384,-3.85131896170919)) ;
#133549=CARTESIAN_POINT('Ctrl Pts',(4.43813540717735,-2.79999997674815,
-3.8129060591291)) ;
#133550=CARTESIAN_POINT('Ctrl Pts',(4.43535270120344,-2.79999997903695,
-3.80375026405077)) ;
#133551=CARTESIAN_POINT('Ctrl Pts',(4.41677772588091,-2.79999999273252,
-3.738668801504)) ;
#133552=CARTESIAN_POINT('Ctrl Pts',(4.4067848879141,-2.79999999887621,-3.68171951852853)) ;
#133553=CARTESIAN_POINT('Ctrl Pts',(4.40081887576631,-2.80000000006435,
-3.60161989679722)) ;
#133554=CARTESIAN_POINT('Ctrl Pts',(4.4,-2.8,-3.57930189819645)) ;
#133555=CARTESIAN_POINT('Ctrl Pts',(4.4,-2.8,-3.55684537882721)) ;
#133556=CARTESIAN_POINT('',(4.4,-2.8,2.54)) ;
#133557=CARTESIAN_POINT('Origin',(4.5,-2.8,2.54)) ;
#133558=CARTESIAN_POINT('',(4.5,-2.7,2.54)) ;
#133559=CARTESIAN_POINT('',(4.5,-2.4,2.54)) ;
#133560=CARTESIAN_POINT('',(4.5,-2.8,2.54)) ;
#133561=CARTESIAN_POINT('',(4.5,-2.7,1.52315462117279)) ;
#133562=CARTESIAN_POINT('',(4.5,-2.7,2.54)) ;
#133563=CARTESIAN_POINT('',(4.5,-2.4,1.96214168703486)) ;
#133564=CARTESIAN_POINT('Origin',(4.5,0.,0.)) ;
#133565=CARTESIAN_POINT('',(4.5,-2.4,2.54)) ;
#133566=CARTESIAN_POINT('Origin',(4.5,-2.3,2.54)) ;
#133567=CARTESIAN_POINT('',(12.7,-2.3,-1.96214168703486)) ;
#133568=CARTESIAN_POINT('',(4.6,-2.3,-1.96214168703486)) ;
#133569=CARTESIAN_POINT('',(4.5,-2.3,-1.96214168703486)) ;
#133570=CARTESIAN_POINT('',(4.6,-2.3,-3.11785831296514)) ;
#133571=CARTESIAN_POINT('',(4.6,-2.3,-2.54)) ;
#133572=CARTESIAN_POINT('',(12.7,-2.3,-3.11785831296514)) ;
#133573=CARTESIAN_POINT('',(4.5,-2.3,-3.11785831296514)) ;
#133574=CARTESIAN_POINT('',(12.7,-2.3,2.54)) ;
#133575=CARTESIAN_POINT('Origin',(0.,0.,2.54)) ;
#133576=CARTESIAN_POINT('Origin',(3.3,10.85,2.54)) ;
#133577=CARTESIAN_POINT('Origin',(-4.8,10.85,2.54)) ;
#133578=CARTESIAN_POINT('Origin',(-4.8,10.3,2.54)) ;
#133579=CARTESIAN_POINT('Origin',(-5.3,5.19009804864072,2.54)) ;
#133580=CARTESIAN_POINT('Origin',(-5.3,-3.95,2.54)) ;
#133581=CARTESIAN_POINT('Origin',(3.5,-3.95,2.54)) ;
#133582=CARTESIAN_POINT('Origin',(3.7,-2.9,2.54)) ;
#133583=CARTESIAN_POINT('Origin',(4.4,-2.7,2.54)) ;
#133584=CARTESIAN_POINT('Origin',(4.6,-2.4,2.54)) ;
#133585=CARTESIAN_POINT('Origin',(12.7,-2.2,2.54)) ;
#133586=CARTESIAN_POINT('Origin',(12.7,2.65,2.54)) ;
#133587=CARTESIAN_POINT('Origin',(4.55912712210514,2.85,2.54)) ;
#133588=CARTESIAN_POINT('Origin',(4.05,3.77568567655479,2.54)) ;
#133589=CARTESIAN_POINT('Origin',(3.85,6.92431432344521,2.54)) ;
#133590=CARTESIAN_POINT('Origin',(-4.65,1.95,-2.)) ;
#133591=CARTESIAN_POINT('',(-4.66204490261456,3.21928058320648,-2.)) ;
#133592=CARTESIAN_POINT('',(-5.3,3.9369800677651,-2.)) ;
#133593=CARTESIAN_POINT('',(-5.47474093186837,4.13356361611701,-2.)) ;
#133594=CARTESIAN_POINT('',(-5.3,-1.88819660112501,-2.)) ;
#133595=CARTESIAN_POINT('',(-5.3,-2.05,-2.)) ;
#133596=CARTESIAN_POINT('',(-4.66204490261456,-1.5692190524323,-2.)) ;
#133597=CARTESIAN_POINT('',(-4.69472135955,-1.58555728090001,-2.)) ;
#133598=CARTESIAN_POINT('',(-4.66204490261456,3.35625,-2.)) ;
#133599=CARTESIAN_POINT('Origin',(-5.4,1.95,2.)) ;
#133600=CARTESIAN_POINT('',(-4.66204490261456,-1.5692190524323,2.)) ;
#133601=CARTESIAN_POINT('',(-5.3,-1.88819660112502,2.)) ;
#133602=CARTESIAN_POINT('',(-5.44472135955,-1.96055728090001,2.)) ;
#133603=CARTESIAN_POINT('',(-5.3,3.9369800677651,2.)) ;
#133604=CARTESIAN_POINT('',(-5.3,4.20000000000001,2.)) ;
#133605=CARTESIAN_POINT('',(-4.66204490261456,3.21928058320648,2.)) ;
#133606=CARTESIAN_POINT('',(-4.72474093186837,3.28981361611701,2.)) ;
#133607=CARTESIAN_POINT('',(-4.66204490261456,-1.67500000000001,2.)) ;
#133608=CARTESIAN_POINT('Origin',(-4.65,1.95,2.)) ;
#133609=CARTESIAN_POINT('',(-3.33134808452128,1.85,1.6776628651052)) ;
#133610=CARTESIAN_POINT('',(-3.48082994825801,1.91712723223402,1.71420287624085)) ;
#133611=CARTESIAN_POINT('Origin',(-3.343288636449,2.02341244982204,1.68058166668753)) ;
#133612=CARTESIAN_POINT('',(-2.4,1.85,1.45)) ;
#133613=CARTESIAN_POINT('',(-4.65,1.85,2.)) ;
#133614=CARTESIAN_POINT('',(-2.4,-0.95,1.45)) ;
#133615=CARTESIAN_POINT('',(-2.4,1.95,1.45)) ;
#133616=CARTESIAN_POINT('',(-3.3526478932023,-0.95,1.68286948500501)) ;
#133617=CARTESIAN_POINT('',(-3.39999999999998,-0.95,1.69444444444444)) ;
#133618=CARTESIAN_POINT('',(-3.44209061230229,-0.971114561800017,1.70473326078501)) ;
#133619=CARTESIAN_POINT('Origin',(-3.36201220558073,-1.11033257691858,1.68515853914196)) ;
#133620=CARTESIAN_POINT('',(-4.63829959356686,-1.5692190524323,1.99713990064968)) ;
#133621=CARTESIAN_POINT('',(-4.68814869588294,-1.59414360359034,2.00932523677139)) ;
#133622=CARTESIAN_POINT('',(-4.63829959356686,3.21928058320648,1.99713990064968)) ;
#133623=CARTESIAN_POINT('',(-4.63829959356686,3.35625,1.99713990064968)) ;
#133624=CARTESIAN_POINT('',(-3.45989661114215,1.89357722797868,1.70908583827919)) ;
#133625=CARTESIAN_POINT('Origin',(-2.4,1.95,1.45)) ;
#133626=CARTESIAN_POINT('',(-2.4,1.85,-1.45)) ;
#133627=CARTESIAN_POINT('',(-2.4,-0.95,-1.45)) ;
#133628=CARTESIAN_POINT('',(-2.4,1.95,-1.45)) ;
#133629=CARTESIAN_POINT('',(-2.4,-1.05,-1.347055690472)) ;
#133630=CARTESIAN_POINT('Origin',(-2.4,-0.950000000000003,-1.347055690472)) ;
#133631=CARTESIAN_POINT('',(-2.4,-1.05,1.347055690472)) ;
#133632=CARTESIAN_POINT('',(-2.4,-1.05,1.45)) ;
#133633=CARTESIAN_POINT('Origin',(-2.4,-0.950000000000021,1.34705569047202)) ;
#133634=CARTESIAN_POINT('',(-2.4,1.95,1.347055690472)) ;
#133635=CARTESIAN_POINT('Origin',(-2.4,1.85000000000002,1.34705569047202)) ;
#133636=CARTESIAN_POINT('',(-2.4,1.95,-1.347055690472)) ;
#133637=CARTESIAN_POINT('',(-2.4,1.95,1.45)) ;
#133638=CARTESIAN_POINT('Origin',(-2.4,1.85000000000002,-1.34705569047202)) ;
#133639=CARTESIAN_POINT('Origin',(-2.4,1.95,-1.45)) ;
#133640=CARTESIAN_POINT('',(-3.3526478932023,-0.95,-1.68286948500501)) ;
#133641=CARTESIAN_POINT('',(-3.44209061230229,-0.971114561800017,-1.70473326078501)) ;
#133642=CARTESIAN_POINT('Origin',(-3.36201220558183,-1.11033257691343,-1.68515853914223)) ;
#133643=CARTESIAN_POINT('',(-2.4,-0.95,-1.45)) ;
#133644=CARTESIAN_POINT('',(-3.33134808452128,1.85,-1.6776628651052)) ;
#133645=CARTESIAN_POINT('',(-2.4,1.85,-1.45)) ;
#133646=CARTESIAN_POINT('',(-3.48082994825801,1.91712723223402,-1.71420287624085)) ;
#133647=CARTESIAN_POINT('Origin',(-3.34328863644904,2.02341244982232,-1.68058166668754)) ;
#133648=CARTESIAN_POINT('',(-4.63829959356686,3.21928058320648,-1.99713990064968)) ;
#133649=CARTESIAN_POINT('',(-4.70989661114216,3.29982722797869,-2.01464139383475)) ;
#133650=CARTESIAN_POINT('',(-4.63829959356686,-1.5692190524323,-1.99713990064968)) ;
#133651=CARTESIAN_POINT('',(-4.63829959356686,-1.67500000000001,-1.99713990064968)) ;
#133652=CARTESIAN_POINT('',(-3.43814869588292,-0.969143603590331,-1.70376968121583)) ;
#133653=CARTESIAN_POINT('Origin',(0.,1.95,0.)) ;
#133654=CARTESIAN_POINT('',(-3.35509339356897,1.95,1.58052296445552)) ;
#133655=CARTESIAN_POINT('',(0.175392621986784,1.95,0.717515271764115)) ;
#133656=CARTESIAN_POINT('',(-3.35509339356897,1.95,-1.58052296445552)) ;
#133657=CARTESIAN_POINT('',(-3.35509339356897,1.95,-1.69444444444444)) ;
#133658=CARTESIAN_POINT('',(0.175392621986784,1.95,-0.717515271764115)) ;
#133659=CARTESIAN_POINT('Origin',(0.,-1.05,0.)) ;
#133660=CARTESIAN_POINT('',(-3.37639320225,-1.05,-1.58572958435533)) ;
#133661=CARTESIAN_POINT('',(-3.42374530904768,-1.05,-1.59730454379476)) ;
#133662=CARTESIAN_POINT('',(-3.37639320225,-1.05,1.58572958435533)) ;
#133663=CARTESIAN_POINT('',(-3.37639320225,-1.05,0.)) ;
#133664=CARTESIAN_POINT('',(-2.4237453090477,-1.05,1.35286009935032)) ;
#133665=CARTESIAN_POINT('Origin',(-3.39999999999998,-1.05,0.)) ;
#133666=CARTESIAN_POINT('',(-3.4211145618,-1.06055728090001,1.60759336013533)) ;
#133667=CARTESIAN_POINT('',(-3.4211145618,-1.06055728090001,-1.60759336013533)) ;
#133668=CARTESIAN_POINT('',(-3.4211145618,-1.06055728090001,0.)) ;
#133669=CARTESIAN_POINT('',(-4.61732354306457,-1.65866177153229,-1.9)) ;
#133670=CARTESIAN_POINT('',(-4.66717264538064,-1.68358632269033,-1.91218533612171)) ;
#133671=CARTESIAN_POINT('',(-5.34472135954999,-2.022360679775,-1.9)) ;
#133672=CARTESIAN_POINT('',(-5.4,-2.05,-1.9)) ;
#133673=CARTESIAN_POINT('',(-5.34472135954999,-2.022360679775,1.9)) ;
#133674=CARTESIAN_POINT('',(-5.34472135954999,-2.022360679775,2.)) ;
#133675=CARTESIAN_POINT('',(-4.61732354306457,-1.65866177153229,1.9)) ;
#133676=CARTESIAN_POINT('',(-4.65,-1.67500000000001,1.9)) ;
#133677=CARTESIAN_POINT('',(-3.41717264538063,-1.05858632269032,1.60662978056615)) ;
#133678=CARTESIAN_POINT('Origin',(-5.4,4.20000000000001,2.54)) ;
#133679=CARTESIAN_POINT('',(-5.37474093186837,4.17158354835192,1.9)) ;
#133680=CARTESIAN_POINT('',(-5.37474093186837,4.17158354835192,-1.9)) ;
#133681=CARTESIAN_POINT('',(-5.37474093186837,4.17158354835192,-2.)) ;
#133682=CARTESIAN_POINT('',(-4.58730397074619,3.28571696708947,-1.9)) ;
#133683=CARTESIAN_POINT('',(-4.65,3.35625,-1.9)) ;
#133684=CARTESIAN_POINT('',(-3.42983432543734,1.98356361611701,-1.61706297559117)) ;
#133685=CARTESIAN_POINT('',(-3.40890098832149,1.96001361186167,-1.61194593762952)) ;
#133686=CARTESIAN_POINT('',(-3.42983432543734,1.98356361611701,1.61706297559117)) ;
#133687=CARTESIAN_POINT('',(-3.42983432543734,1.98356361611701,1.69444444444444)) ;
#133688=CARTESIAN_POINT('',(-4.58730397074619,3.28571696708947,1.9)) ;
#133689=CARTESIAN_POINT('',(-4.65890098832149,3.36626361186168,1.91750149318507)) ;
#133690=CARTESIAN_POINT('',(-5.4,4.20000000000001,1.9)) ;
#133691=CARTESIAN_POINT('Origin',(-3.15,-3.9,1.)) ;
#133692=CARTESIAN_POINT('',(-3.15,-3.95,0.9)) ;
#133693=CARTESIAN_POINT('',(-3.15,-3.85,0.9)) ;
#133694=CARTESIAN_POINT('',(-3.15,-3.75,0.9)) ;
#133695=CARTESIAN_POINT('',(-3.15,-3.85,-0.900000000000001)) ;
#133696=CARTESIAN_POINT('',(-3.15,-3.85,1.)) ;
#133697=CARTESIAN_POINT('',(-3.15,-3.95,-0.900000000000001)) ;
#133698=CARTESIAN_POINT('',(-3.15,-4.05,-0.900000000000001)) ;
#133699=CARTESIAN_POINT('',(-3.15,-3.95,1.)) ;
#133700=CARTESIAN_POINT('Origin',(-4.4,-3.9,-1.)) ;
#133701=CARTESIAN_POINT('',(-3.25,-3.85,-1.)) ;
#133702=CARTESIAN_POINT('',(-4.3,-3.85,-1.)) ;
#133703=CARTESIAN_POINT('',(-4.4,-3.85,-1.)) ;
#133704=CARTESIAN_POINT('',(-4.3,-3.95,-1.)) ;
#133705=CARTESIAN_POINT('',(-4.3,-4.05,-1.)) ;
#133706=CARTESIAN_POINT('',(-3.25,-3.95,-1.)) ;
#133707=CARTESIAN_POINT('',(-4.4,-3.95,-1.)) ;
#133708=CARTESIAN_POINT('',(-3.25,-3.75,-1.)) ;
#133709=CARTESIAN_POINT('Origin',(-4.4,-3.9,0.999999999999999)) ;
#133710=CARTESIAN_POINT('',(-4.4,-3.85,-0.900000000000001)) ;
#133711=CARTESIAN_POINT('',(-4.4,-3.85,0.899999999999999)) ;
#133712=CARTESIAN_POINT('',(-4.4,-3.85,0.999999999999999)) ;
#133713=CARTESIAN_POINT('',(-4.4,-3.95,0.899999999999999)) ;
#133714=CARTESIAN_POINT('',(-4.4,-4.05,0.899999999999999)) ;
#133715=CARTESIAN_POINT('',(-4.4,-3.95,-0.900000000000001)) ;
#133716=CARTESIAN_POINT('',(-4.4,-3.95,0.999999999999999)) ;
#133717=CARTESIAN_POINT('',(-4.4,-3.75,-0.900000000000001)) ;
#133718=CARTESIAN_POINT('Origin',(-4.4,-3.9,0.999999999999999)) ;
#133719=CARTESIAN_POINT('',(-4.3,-3.95,0.999999999999999)) ;
#133720=CARTESIAN_POINT('',(-4.3,-3.85,0.999999999999999)) ;
#133721=CARTESIAN_POINT('',(-4.3,-3.75,0.999999999999999)) ;
#133722=CARTESIAN_POINT('',(-3.25,-3.85,1.)) ;
#133723=CARTESIAN_POINT('',(-4.4,-3.85,0.999999999999999)) ;
#133724=CARTESIAN_POINT('',(-3.25,-3.95,1.)) ;
#133725=CARTESIAN_POINT('',(-3.25,-4.05,1.)) ;
#133726=CARTESIAN_POINT('',(-4.4,-3.95,0.999999999999999)) ;
#133727=CARTESIAN_POINT('Origin',(0.,-3.75,0.)) ;
#133728=CARTESIAN_POINT('',(-3.25,-3.75,0.9)) ;
#133729=CARTESIAN_POINT('',(-4.3,-3.75,0.899999999999999)) ;
#133730=CARTESIAN_POINT('',(-1.56125112837913E-16,-3.75,0.9)) ;
#133731=CARTESIAN_POINT('',(-4.3,-3.75,-0.900000000000001)) ;
#133732=CARTESIAN_POINT('',(-4.3,-3.75,0.)) ;
#133733=CARTESIAN_POINT('',(-3.25,-3.75,-0.900000000000001)) ;
#133734=CARTESIAN_POINT('',(-1.56125112837913E-16,-3.75,-0.900000000000001)) ;
#133735=CARTESIAN_POINT('',(-3.25,-3.75,-1.40946282423115E-15)) ;
#133736=CARTESIAN_POINT('',(-4.15,-3.75,-0.850000000000001)) ;
#133737=CARTESIAN_POINT('',(-3.4,-3.75,-0.850000000000001)) ;
#133738=CARTESIAN_POINT('',(-4.15,-3.75,-0.850000000000001)) ;
#133739=CARTESIAN_POINT('',(-4.25,-3.75,-0.75)) ;
#133740=CARTESIAN_POINT('Origin',(-4.15,-3.75,-0.750000000000001)) ;
#133741=CARTESIAN_POINT('',(-4.25,-3.75,0.749999999999999)) ;
#133742=CARTESIAN_POINT('',(-4.25,-3.75,0.749999999999999)) ;
#133743=CARTESIAN_POINT('',(-4.15,-3.75,0.85)) ;
#133744=CARTESIAN_POINT('Origin',(-4.15,-3.75,0.75)) ;
#133745=CARTESIAN_POINT('',(-3.4,-3.75,0.85)) ;
#133746=CARTESIAN_POINT('',(-3.4,-3.75,0.85)) ;
#133747=CARTESIAN_POINT('',(-3.3,-3.75,0.749999999999999)) ;
#133748=CARTESIAN_POINT('Origin',(-3.4,-3.75,0.75)) ;
#133749=CARTESIAN_POINT('',(-3.3,-3.75,-0.75)) ;
#133750=CARTESIAN_POINT('',(-3.3,-3.75,-0.75)) ;
#133751=CARTESIAN_POINT('Origin',(-3.4,-3.75,-0.750000000000001)) ;
#133752=CARTESIAN_POINT('Origin',(-3.4,-3.75,-0.750000000000001)) ;
#133753=CARTESIAN_POINT('',(-3.4,-3.9,-0.850000000000001)) ;
#133754=CARTESIAN_POINT('',(-3.3,-3.9,-0.75)) ;
#133755=CARTESIAN_POINT('Origin',(-3.4,-3.9,-0.750000000000001)) ;
#133756=CARTESIAN_POINT('',(-3.4,-3.75,-0.850000000000001)) ;
#133757=CARTESIAN_POINT('',(-3.3,-3.75,-0.75)) ;
#133758=CARTESIAN_POINT('Origin',(-4.15,-3.75,-0.850000000000001)) ;
#133759=CARTESIAN_POINT('',(-4.15,-3.9,-0.850000000000001)) ;
#133760=CARTESIAN_POINT('',(-4.15,-3.9,-0.850000000000001)) ;
#133761=CARTESIAN_POINT('',(-4.15,-3.75,-0.850000000000001)) ;
#133762=CARTESIAN_POINT('Origin',(-4.15,-3.75,-0.750000000000001)) ;
#133763=CARTESIAN_POINT('',(-4.25,-3.9,-0.75)) ;
#133764=CARTESIAN_POINT('Origin',(-4.15,-3.9,-0.750000000000001)) ;
#133765=CARTESIAN_POINT('',(-4.25,-3.75,-0.75)) ;
#133766=CARTESIAN_POINT('Origin',(-4.25,-3.75,0.749999999999999)) ;
#133767=CARTESIAN_POINT('',(-4.25,-3.9,0.749999999999999)) ;
#133768=CARTESIAN_POINT('',(-4.25,-3.9,0.749999999999999)) ;
#133769=CARTESIAN_POINT('',(-4.25,-3.75,0.749999999999999)) ;
#133770=CARTESIAN_POINT('Origin',(-4.15,-3.75,0.75)) ;
#133771=CARTESIAN_POINT('',(-4.15,-3.9,0.85)) ;
#133772=CARTESIAN_POINT('Origin',(-4.15,-3.9,0.75)) ;
#133773=CARTESIAN_POINT('',(-4.15,-3.75,0.85)) ;
#133774=CARTESIAN_POINT('Origin',(-3.4,-3.75,0.85)) ;
#133775=CARTESIAN_POINT('',(-3.4,-3.9,0.85)) ;
#133776=CARTESIAN_POINT('',(-3.4,-3.9,0.85)) ;
#133777=CARTESIAN_POINT('',(-3.4,-3.75,0.85)) ;
#133778=CARTESIAN_POINT('Origin',(-3.4,-3.75,0.75)) ;
#133779=CARTESIAN_POINT('',(-3.3,-3.9,0.749999999999999)) ;
#133780=CARTESIAN_POINT('Origin',(-3.4,-3.9,0.75)) ;
#133781=CARTESIAN_POINT('',(-3.3,-3.75,0.749999999999999)) ;
#133782=CARTESIAN_POINT('Origin',(-3.3,-3.75,-0.75)) ;
#133783=CARTESIAN_POINT('',(-3.3,-3.9,-0.75)) ;
#133784=CARTESIAN_POINT('Origin',(0.,-3.9,0.)) ;
#133785=CARTESIAN_POINT('Origin',(0.,9.95,0.)) ;
#133786=CARTESIAN_POINT('',(-0.230887397576972,9.95,1.91486057185377)) ;
#133787=CARTESIAN_POINT('Origin',(-0.321518176280637,8.95,1.8725987456797)) ;
#133788=CARTESIAN_POINT('',(-0.321518176280637,9.05,1.8725987456797)) ;
#133789=CARTESIAN_POINT('',(1.22782596331729,9.85,-1.449980483939)) ;
#133790=CARTESIAN_POINT('Origin',(-1.22782596331729,8.95,1.449980483939)) ;
#133791=CARTESIAN_POINT('',(-1.22782596331729,9.05,1.449980483939)) ;
#133792=CARTESIAN_POINT('',(-1.22782596331729,9.85,1.449980483939)) ;
#133793=CARTESIAN_POINT('Origin',(0.,8.95,0.)) ;
#133794=CARTESIAN_POINT('',(-0.362523114814661,8.95,-0.169047304696279)) ;
#133795=CARTESIAN_POINT('',(0.36252311481466,8.95,0.169047304696279)) ;
#133796=CARTESIAN_POINT('Origin',(-2.65,10.8,-1.)) ;
#133797=CARTESIAN_POINT('',(-2.65,10.75,-0.900000000000001)) ;
#133798=CARTESIAN_POINT('',(-2.65,10.75,0.899999999999999)) ;
#133799=CARTESIAN_POINT('',(-2.65,10.75,-1.)) ;
#133800=CARTESIAN_POINT('',(-2.65,10.85,0.899999999999999)) ;
#133801=CARTESIAN_POINT('',(-2.65,10.95,0.899999999999999)) ;
#133802=CARTESIAN_POINT('',(-2.65,10.85,-0.900000000000001)) ;
#133803=CARTESIAN_POINT('',(-2.65,10.85,-1.)) ;
#133804=CARTESIAN_POINT('',(-2.65,10.65,-0.900000000000001)) ;
#133805=CARTESIAN_POINT('Origin',(-3.9,10.8,1.)) ;
#133806=CARTESIAN_POINT('',(-2.75,10.85,0.999999999999999)) ;
#133807=CARTESIAN_POINT('',(-2.75,10.75,0.999999999999999)) ;
#133808=CARTESIAN_POINT('',(-2.75,10.65,0.999999999999999)) ;
#133809=CARTESIAN_POINT('',(-3.8,10.75,1.)) ;
#133810=CARTESIAN_POINT('',(-3.9,10.75,1.)) ;
#133811=CARTESIAN_POINT('',(-3.8,10.85,1.)) ;
#133812=CARTESIAN_POINT('',(-3.8,10.95,1.)) ;
#133813=CARTESIAN_POINT('',(-3.9,10.85,1.)) ;
#133814=CARTESIAN_POINT('Origin',(-3.9,10.8,-1.)) ;
#133815=CARTESIAN_POINT('',(-3.9,10.85,0.9)) ;
#133816=CARTESIAN_POINT('',(-3.9,10.75,0.9)) ;
#133817=CARTESIAN_POINT('',(-3.9,10.65,0.9)) ;
#133818=CARTESIAN_POINT('',(-3.9,10.75,-0.9)) ;
#133819=CARTESIAN_POINT('',(-3.9,10.75,-1.)) ;
#133820=CARTESIAN_POINT('',(-3.9,10.85,-0.9)) ;
#133821=CARTESIAN_POINT('',(-3.9,10.95,-0.9)) ;
#133822=CARTESIAN_POINT('',(-3.9,10.85,-1.)) ;
#133823=CARTESIAN_POINT('Origin',(-3.9,10.8,-1.)) ;
#133824=CARTESIAN_POINT('',(-3.8,10.75,-1.)) ;
#133825=CARTESIAN_POINT('',(-2.75,10.75,-1.)) ;
#133826=CARTESIAN_POINT('',(-3.9,10.75,-1.)) ;
#133827=CARTESIAN_POINT('',(-2.75,10.85,-1.)) ;
#133828=CARTESIAN_POINT('',(-2.75,10.95,-1.)) ;
#133829=CARTESIAN_POINT('',(-3.8,10.85,-1.)) ;
#133830=CARTESIAN_POINT('',(-3.9,10.85,-1.)) ;
#133831=CARTESIAN_POINT('',(-3.8,10.65,-1.)) ;
#133832=CARTESIAN_POINT('Origin',(0.,10.65,0.)) ;
#133833=CARTESIAN_POINT('',(-3.8,10.65,0.9)) ;
#133834=CARTESIAN_POINT('',(-2.75,10.65,0.899999999999999)) ;
#133835=CARTESIAN_POINT('',(1.56125112837912E-16,10.65,0.899999999999999)) ;
#133836=CARTESIAN_POINT('',(-2.75,10.65,-0.900000000000001)) ;
#133837=CARTESIAN_POINT('',(-2.75,10.65,5.96311194867028E-16)) ;
#133838=CARTESIAN_POINT('',(-3.8,10.65,-0.9)) ;
#133839=CARTESIAN_POINT('',(-1.56125112837913E-16,10.65,-0.900000000000001)) ;
#133840=CARTESIAN_POINT('',(-3.8,10.65,8.23993651088984E-16)) ;
#133841=CARTESIAN_POINT('',(-3.65,10.65,0.85)) ;
#133842=CARTESIAN_POINT('',(-2.9,10.65,0.85)) ;
#133843=CARTESIAN_POINT('',(-3.65,10.65,0.85)) ;
#133844=CARTESIAN_POINT('',(-3.75,10.65,0.749999999999999)) ;
#133845=CARTESIAN_POINT('Origin',(-3.65,10.65,0.75)) ;
#133846=CARTESIAN_POINT('',(-3.75,10.65,-0.75)) ;
#133847=CARTESIAN_POINT('',(-3.75,10.65,-0.75)) ;
#133848=CARTESIAN_POINT('',(-3.65,10.65,-0.850000000000001)) ;
#133849=CARTESIAN_POINT('Origin',(-3.65,10.65,-0.750000000000001)) ;
#133850=CARTESIAN_POINT('',(-2.9,10.65,-0.850000000000001)) ;
#133851=CARTESIAN_POINT('',(-2.9,10.65,-0.850000000000001)) ;
#133852=CARTESIAN_POINT('',(-2.8,10.65,-0.75)) ;
#133853=CARTESIAN_POINT('Origin',(-2.9,10.65,-0.750000000000001)) ;
#133854=CARTESIAN_POINT('',(-2.8,10.65,0.749999999999999)) ;
#133855=CARTESIAN_POINT('',(-2.8,10.65,0.749999999999999)) ;
#133856=CARTESIAN_POINT('Origin',(-2.9,10.65,0.75)) ;
#133857=CARTESIAN_POINT('Origin',(-2.9,10.65,0.75)) ;
#133858=CARTESIAN_POINT('',(-2.8,10.7,0.749999999999999)) ;
#133859=CARTESIAN_POINT('',(-2.8,10.65,0.749999999999999)) ;
#133860=CARTESIAN_POINT('',(-2.9,10.7,0.85)) ;
#133861=CARTESIAN_POINT('Origin',(-2.9,10.7,0.75)) ;
#133862=CARTESIAN_POINT('',(-2.9,10.65,0.85)) ;
#133863=CARTESIAN_POINT('Origin',(-3.65,10.65,0.85)) ;
#133864=CARTESIAN_POINT('',(-3.65,10.7,0.85)) ;
#133865=CARTESIAN_POINT('',(-3.65,10.7,0.85)) ;
#133866=CARTESIAN_POINT('',(-3.65,10.65,0.85)) ;
#133867=CARTESIAN_POINT('Origin',(-3.65,10.65,0.75)) ;
#133868=CARTESIAN_POINT('',(-3.75,10.7,0.749999999999999)) ;
#133869=CARTESIAN_POINT('Origin',(-3.65,10.7,0.75)) ;
#133870=CARTESIAN_POINT('',(-3.75,10.65,0.749999999999999)) ;
#133871=CARTESIAN_POINT('Origin',(-3.75,10.65,-0.75)) ;
#133872=CARTESIAN_POINT('',(-3.75,10.7,-0.75)) ;
#133873=CARTESIAN_POINT('',(-3.75,10.7,-0.75)) ;
#133874=CARTESIAN_POINT('',(-3.75,10.65,-0.75)) ;
#133875=CARTESIAN_POINT('Origin',(-3.65,10.65,-0.750000000000001)) ;
#133876=CARTESIAN_POINT('',(-3.65,10.7,-0.850000000000001)) ;
#133877=CARTESIAN_POINT('Origin',(-3.65,10.7,-0.750000000000001)) ;
#133878=CARTESIAN_POINT('',(-3.65,10.65,-0.850000000000001)) ;
#133879=CARTESIAN_POINT('Origin',(-2.9,10.65,-0.850000000000001)) ;
#133880=CARTESIAN_POINT('',(-2.9,10.7,-0.850000000000001)) ;
#133881=CARTESIAN_POINT('',(-2.9,10.7,-0.850000000000001)) ;
#133882=CARTESIAN_POINT('',(-2.9,10.65,-0.850000000000001)) ;
#133883=CARTESIAN_POINT('Origin',(-2.9,10.65,-0.750000000000001)) ;
#133884=CARTESIAN_POINT('',(-2.8,10.7,-0.75)) ;
#133885=CARTESIAN_POINT('Origin',(-2.9,10.7,-0.750000000000001)) ;
#133886=CARTESIAN_POINT('',(-2.8,10.65,-0.75)) ;
#133887=CARTESIAN_POINT('Origin',(-2.8,10.65,0.749999999999999)) ;
#133888=CARTESIAN_POINT('',(-2.8,10.7,0.749999999999999)) ;
#133889=CARTESIAN_POINT('Origin',(0.,10.8,0.)) ;
#133890=CARTESIAN_POINT('',(-3.65,10.8,0.75)) ;
#133891=CARTESIAN_POINT('',(-2.9,10.8,0.75)) ;
#133892=CARTESIAN_POINT('',(0.,10.8,0.75)) ;
#133893=CARTESIAN_POINT('',(-2.9,10.8,-0.750000000000001)) ;
#133894=CARTESIAN_POINT('',(-2.9,10.8,0.)) ;
#133895=CARTESIAN_POINT('',(-3.65,10.8,-0.750000000000001)) ;
#133896=CARTESIAN_POINT('',(0.,10.8,-0.750000000000001)) ;
#133897=CARTESIAN_POINT('',(-3.65,10.8,0.)) ;
#133898=CARTESIAN_POINT('Origin',(4.5,2.75,-1.375)) ;
#133899=CARTESIAN_POINT('',(4.5,2.63356010126946,-1.39440664978842)) ;
#133900=CARTESIAN_POINT('',(4.6,2.11643989873054,-1.48059335021158)) ;
#133901=CARTESIAN_POINT('',(4.6,2.11643989873054,-1.48059335021158)) ;
#133902=CARTESIAN_POINT('',(12.7,2.11643989873054,-1.48059335021158)) ;
#133903=CARTESIAN_POINT('',(12.8,2.11643989873054,-1.48059335021158)) ;
#133904=CARTESIAN_POINT('',(12.7,2.75,-1.375)) ;
#133905=CARTESIAN_POINT('Origin',(4.5,2.,-1.5)) ;
#133906=CARTESIAN_POINT('',(4.6,2.,-1.38195395782836)) ;
#133907=CARTESIAN_POINT('',(4.6,2.,1.5)) ;
#133908=CARTESIAN_POINT('',(12.7,2.,-1.38195395782836)) ;
#133909=CARTESIAN_POINT('',(12.7,2.,-1.5)) ;
#133910=CARTESIAN_POINT('',(4.5,2.,-1.38195395782836)) ;
#133911=CARTESIAN_POINT('Origin',(4.5,2.,1.5)) ;
#133912=CARTESIAN_POINT('',(4.6,2.63356010126946,1.39440664978842)) ;
#133913=CARTESIAN_POINT('',(4.6,2.63356010126947,1.39440664978842)) ;
#133914=CARTESIAN_POINT('',(4.5,2.63356010126946,1.39440664978842)) ;
#133915=CARTESIAN_POINT('',(12.7,2.,1.5)) ;
#133916=CARTESIAN_POINT('Origin',(4.5,0.,0.)) ;
#133917=CARTESIAN_POINT('',(4.5,2.72431432344521,1.30736518335501)) ;
#133918=CARTESIAN_POINT('',(4.5,2.72431432344521,0.)) ;
#133919=CARTESIAN_POINT('',(4.5,2.61712020253893,1.29576725740521)) ;
#133920=CARTESIAN_POINT('Origin',(4.5,2.65,1.49304604217164)) ;
#133921=CARTESIAN_POINT('',(4.5,2.1,1.38195395782836)) ;
#133922=CARTESIAN_POINT('',(4.5,2.1,1.38195395782836)) ;
#133923=CARTESIAN_POINT('',(4.5,2.1,-1.38195395782836)) ;
#133924=CARTESIAN_POINT('',(4.5,2.1,-1.5)) ;
#133925=CARTESIAN_POINT('',(4.5,2.61712020253893,-1.29576725740521)) ;
#133926=CARTESIAN_POINT('Origin',(10.3,0.,0.)) ;
#133927=CARTESIAN_POINT('Origin',(0.584645609909621,0.,0.)) ;
#133928=CARTESIAN_POINT('',(4.6,-2.32258064516129,1.8988467939047)) ;
#133929=CARTESIAN_POINT('',(4.6,-2.79310344827574,1.09479364595807)) ;
#133930=CARTESIAN_POINT('Origin',(4.6,0.,0.)) ;
#133931=CARTESIAN_POINT('',(4.6,-2.79310344827574,-1.09479364595807)) ;
#133932=CARTESIAN_POINT('Origin',(4.6,0.,0.)) ;
#133933=CARTESIAN_POINT('',(4.6,-2.32258064516129,-1.8988467939047)) ;
#133934=CARTESIAN_POINT('Origin',(4.6,0.,0.)) ;
#133935=CARTESIAN_POINT('',(12.7,-2.32258064516129,-1.8988467939047)) ;
#133936=CARTESIAN_POINT('',(0.584645609909621,-2.32258064516129,-1.8988467939047)) ;
#133937=CARTESIAN_POINT('',(12.7,-2.32258064516129,1.8988467939047)) ;
#133938=CARTESIAN_POINT('Origin',(12.7,0.,0.)) ;
#133939=CARTESIAN_POINT('',(0.584645609909621,-2.32258064516129,1.8988467939047)) ;
#133940=CARTESIAN_POINT('Ctrl Pts',(-5.37474093186837,4.17158354835192,
1.9)) ;
#133941=CARTESIAN_POINT('Ctrl Pts',(-5.4,4.2,1.9)) ;
#133942=CARTESIAN_POINT('Ctrl Pts',(-5.4,4.23801993223491,1.9)) ;
#133943=CARTESIAN_POINT('Ctrl Pts',(-5.37474093064202,4.17158354697228,
1.92625343593895)) ;
#133944=CARTESIAN_POINT('Ctrl Pts',(-5.4,4.19999999724801,1.93751858720109)) ;
#133945=CARTESIAN_POINT('Ctrl Pts',(-5.4,4.23801992976516,1.95250687190974)) ;
#133946=CARTESIAN_POINT('Ctrl Pts',(-5.36668583490655,4.14629949399955,
1.95219871311588)) ;
#133947=CARTESIAN_POINT('Ctrl Pts',(-5.4,4.16739198385624,1.97533216493415)) ;
#133948=CARTESIAN_POINT('Ctrl Pts',(-5.4,4.20557579169425,2.00439742623175)) ;
#133949=CARTESIAN_POINT('Ctrl Pts',(-5.33901380460609,4.05944006555646,
1.98922264312143)) ;
#133950=CARTESIAN_POINT('Ctrl Pts',(-5.4,4.06625640449639,2.01686736338588)) ;
#133951=CARTESIAN_POINT('Ctrl Pts',(-5.4,4.09411900298411,2.07844528624287)) ;
#133952=CARTESIAN_POINT('Ctrl Pts',(-5.31962206268973,3.99857154231912,
2.)) ;
#133953=CARTESIAN_POINT('Ctrl Pts',(-5.4,3.99346933127513,2.01799649257355)) ;
#133954=CARTESIAN_POINT('Ctrl Pts',(-5.4,4.01601337581891,2.09999999951886)) ;
#133955=CARTESIAN_POINT('Ctrl Pts',(-5.3,3.9369800677651,2.)) ;
#133956=CARTESIAN_POINT('Ctrl Pts',(-5.4,3.9369800677651,2.)) ;
#133957=CARTESIAN_POINT('Ctrl Pts',(-5.4,3.9369800677651,2.1)) ;
#133958=CARTESIAN_POINT('Origin',(-5.3,4.23801993223491,1.9)) ;
#133959=CARTESIAN_POINT('Ctrl Pts',(-5.3,3.9369800677651,2.)) ;
#133960=CARTESIAN_POINT('Ctrl Pts',(-5.31962206268973,3.99857154231912,
2.)) ;
#133961=CARTESIAN_POINT('Ctrl Pts',(-5.33901380460609,4.05944006555646,
1.98922264312143)) ;
#133962=CARTESIAN_POINT('Ctrl Pts',(-5.36668583490655,4.14629949399955,
1.95219871311588)) ;
#133963=CARTESIAN_POINT('Ctrl Pts',(-5.37474093064202,4.17158354697228,
1.92625343593895)) ;
#133964=CARTESIAN_POINT('Ctrl Pts',(-5.37474093186837,4.17158354835192,
1.9)) ;
#133965=CARTESIAN_POINT('Origin',(-5.3,3.9369800677651,2.1)) ;
#133966=CARTESIAN_POINT('Origin',(-4.6737453090477,1.85,1.90286009935032)) ;
#133967=CARTESIAN_POINT('Origin',(-3.35509339356897,1.85,1.58052296445552)) ;
#133968=CARTESIAN_POINT('Ctrl Pts',(-3.35509339356897,1.95,1.58052296445552)) ;
#133969=CARTESIAN_POINT('Ctrl Pts',(-3.33134808452128,1.95,1.6776628651052)) ;
#133970=CARTESIAN_POINT('Ctrl Pts',(-3.33134808452128,1.85,1.6776628651052)) ;
#133971=CARTESIAN_POINT('Ctrl Pts',(-3.38343213690419,1.95,1.59437746119719)) ;
#133972=CARTESIAN_POINT('Ctrl Pts',(-3.36046743872484,1.94345445676969,
1.68478092946605)) ;
#133973=CARTESIAN_POINT('Ctrl Pts',(-3.38803897426452,1.85000000162387,
1.69152063815355)) ;
#133974=CARTESIAN_POINT('Ctrl Pts',(-3.41101314049054,1.96238978305186,
1.60786150708384)) ;
#133975=CARTESIAN_POINT('Ctrl Pts',(-3.39538881861724,1.95068928167334,
1.69331726677308)) ;
#133976=CARTESIAN_POINT('Ctrl Pts',(-3.44316973238528,1.87475949194143,
1.70499704569418)) ;
#133977=CARTESIAN_POINT('Ctrl Pts',(-3.42983432543734,1.98356361611701,
1.61706297559117)) ;
#133978=CARTESIAN_POINT('Ctrl Pts',(-3.42093333711585,1.97355000425533,
1.6995614824061)) ;
#133979=CARTESIAN_POINT('Ctrl Pts',(-3.48082994825801,1.91712723223402,
1.71420287624085)) ;
#133980=CARTESIAN_POINT('Origin',(-3.50457525730571,1.91712723223402,1.61706297559117)) ;
#133981=CARTESIAN_POINT('Origin',(-3.36128627567748,2.03621361435751,1.58355059566492)) ;
#133982=CARTESIAN_POINT('Origin',(-4.05330900605469,2.53445269957662,1.75119789195203)) ;
#133983=CARTESIAN_POINT('Origin',(-4.66204490261456,3.21928058320648,1.9)) ;
#133984=CARTESIAN_POINT('Origin',(-4.35749955255802,2.87666706439287,1.9)) ;
#133985=CARTESIAN_POINT('Origin',(-4.66204490261456,3.21928058320648,1.9)) ;
#133986=CARTESIAN_POINT('Origin',(-5.3,5.2,2.1)) ;
#133987=CARTESIAN_POINT('Origin',(-5.3,-1.88819660112502,2.1)) ;
#133988=CARTESIAN_POINT('Origin',(-5.3,4.23801993223491,2.54)) ;
#133989=CARTESIAN_POINT('Origin',(-5.3,4.23801993223491,-1.9)) ;
#133990=CARTESIAN_POINT('Origin',(-3.35509339356897,2.05,0.)) ;
#133991=CARTESIAN_POINT('Origin',(-3.36128627567765,2.03621361435713,-1.583550595665)) ;
#133992=CARTESIAN_POINT('Origin',(-2.4237453090477,1.85,-1.35286009935032)) ;
#133993=CARTESIAN_POINT('Origin',(-3.35509339356897,1.85,-1.58052296445552)) ;
#133994=CARTESIAN_POINT('Origin',(-4.66204490261456,3.21928058320648,1.9)) ;
#133995=CARTESIAN_POINT('Origin',(-4.66204490261456,3.21928058320648,1.9)) ;
#133996=CARTESIAN_POINT('Ctrl Pts',(-5.29976814257746,-1.88802911972917,
2.00000017262218)) ;
#133997=CARTESIAN_POINT('Ctrl Pts',(-5.4,-1.88802831720455,1.99976740645701)) ;
#133998=CARTESIAN_POINT('Ctrl Pts',(-5.4,-1.8879174628307,2.09999983753763)) ;
#133999=CARTESIAN_POINT('Ctrl Pts',(-5.31153957531162,-1.92331224822995,
2.00001353231107)) ;
#134000=CARTESIAN_POINT('Ctrl Pts',(-5.4,-1.92148676945292,2.01102210746197)) ;
#134001=CARTESIAN_POINT('Ctrl Pts',(-5.4,-1.94671708614656,2.10006828697156)) ;
#134002=CARTESIAN_POINT('Ctrl Pts',(-5.32318090226696,-1.95817527052251,
1.98921550273188)) ;
#134003=CARTESIAN_POINT('Ctrl Pts',(-5.4,-1.96527310172482,2.00783661624713)) ;
#134004=CARTESIAN_POINT('Ctrl Pts',(-5.4,-2.00485091174287,2.07850392511067)) ;
#134005=CARTESIAN_POINT('Ctrl Pts',(-5.33978950165953,-2.00789652656154,
1.95213503498037)) ;
#134006=CARTESIAN_POINT('Ctrl Pts',(-5.4,-2.02908601268744,1.96863348546834)) ;
#134007=CARTESIAN_POINT('Ctrl Pts',(-5.4,-2.087770056524,2.00433878736395)) ;
#134008=CARTESIAN_POINT('Ctrl Pts',(-5.34461954754096,-2.02234798681675,
1.92615385528167)) ;
#134009=CARTESIAN_POINT('Ctrl Pts',(-5.4,-2.04997459329993,1.93432433515997)) ;
#134010=CARTESIAN_POINT('Ctrl Pts',(-5.4,-2.11187974550671,1.95234231302604)) ;
#134011=CARTESIAN_POINT('Ctrl Pts',(-5.34460423617422,-2.02230212313482,
1.89987524812986)) ;
#134012=CARTESIAN_POINT('Ctrl Pts',(-5.4,-2.0499093833863,1.89983624572346)) ;
#134013=CARTESIAN_POINT('Ctrl Pts',(-5.4,-2.11180321723903,1.89975033111955)) ;
#134014=CARTESIAN_POINT('Origin',(-5.30000000000002,-1.88819660112507,1.90000000000004)) ;
#134015=CARTESIAN_POINT('Origin',(-5.3,-2.11180339887499,1.9)) ;
#134016=CARTESIAN_POINT('Ctrl Pts',(-5.3,3.9369800677651,-2.)) ;
#134017=CARTESIAN_POINT('Ctrl Pts',(-5.4,3.9369800677651,-2.)) ;
#134018=CARTESIAN_POINT('Ctrl Pts',(-5.4,3.9369800677651,-2.1)) ;
#134019=CARTESIAN_POINT('Ctrl Pts',(-5.31962206268973,3.9985715423191,-2.)) ;
#134020=CARTESIAN_POINT('Ctrl Pts',(-5.4,3.99346933127511,-2.01799649257355)) ;
#134021=CARTESIAN_POINT('Ctrl Pts',(-5.4,4.01601337581889,-2.09999999951886)) ;
#134022=CARTESIAN_POINT('Ctrl Pts',(-5.3390138046061,4.05944006555648,-1.98922264312143)) ;
#134023=CARTESIAN_POINT('Ctrl Pts',(-5.4,4.06625640449641,-2.01686736338588)) ;
#134024=CARTESIAN_POINT('Ctrl Pts',(-5.4,4.09411900298413,-2.07844528624287)) ;
#134025=CARTESIAN_POINT('Ctrl Pts',(-5.36668583490655,4.14629949399953,
-1.95219871311588)) ;
#134026=CARTESIAN_POINT('Ctrl Pts',(-5.4,4.16739198385622,-1.97533216493415)) ;
#134027=CARTESIAN_POINT('Ctrl Pts',(-5.4,4.20557579169423,-2.00439742623175)) ;
#134028=CARTESIAN_POINT('Ctrl Pts',(-5.37474093064202,4.17158354697228,
-1.92625343593895)) ;
#134029=CARTESIAN_POINT('Ctrl Pts',(-5.4,4.19999999724801,-1.93751858720109)) ;
#134030=CARTESIAN_POINT('Ctrl Pts',(-5.4,4.23801992976516,-1.95250687190974)) ;
#134031=CARTESIAN_POINT('Ctrl Pts',(-5.37474093186837,4.17158354835192,
-1.9)) ;
#134032=CARTESIAN_POINT('Ctrl Pts',(-5.4,4.2,-1.9)) ;
#134033=CARTESIAN_POINT('Ctrl Pts',(-5.4,4.23801993223491,-1.9)) ;
#134034=CARTESIAN_POINT('Origin',(-5.3,3.9369800677651,-2.1)) ;
#134035=CARTESIAN_POINT('Ctrl Pts',(-5.37474093186837,4.17158354835192,
-1.9)) ;
#134036=CARTESIAN_POINT('Ctrl Pts',(-5.37474093064202,4.17158354697228,
-1.92625343593895)) ;
#134037=CARTESIAN_POINT('Ctrl Pts',(-5.36668583490655,4.14629949399953,
-1.95219871311588)) ;
#134038=CARTESIAN_POINT('Ctrl Pts',(-5.3390138046061,4.05944006555648,-1.98922264312143)) ;
#134039=CARTESIAN_POINT('Ctrl Pts',(-5.31962206268973,3.9985715423191,-2.)) ;
#134040=CARTESIAN_POINT('Ctrl Pts',(-5.3,3.9369800677651,-2.)) ;
#134041=CARTESIAN_POINT('Ctrl Pts',(-3.42983432543734,1.98356361611701,
-1.61706297559117)) ;
#134042=CARTESIAN_POINT('Ctrl Pts',(-3.42093333711585,1.97355000425533,
-1.6995614824061)) ;
#134043=CARTESIAN_POINT('Ctrl Pts',(-3.48082994825801,1.91712723223402,
-1.71420287624085)) ;
#134044=CARTESIAN_POINT('Ctrl Pts',(-3.41101314049054,1.96238978305185,
-1.60786150708389)) ;
#134045=CARTESIAN_POINT('Ctrl Pts',(-3.39538881861726,1.95068928167333,
-1.69331726677314)) ;
#134046=CARTESIAN_POINT('Ctrl Pts',(-3.44316973238526,1.87475949194143,
-1.70499704569417)) ;
#134047=CARTESIAN_POINT('Ctrl Pts',(-3.38343213690418,1.95,-1.59437746119719)) ;
#134048=CARTESIAN_POINT('Ctrl Pts',(-3.36046743872482,1.94345445676967,
-1.68478092946604)) ;
#134049=CARTESIAN_POINT('Ctrl Pts',(-3.38803897426454,1.85000000162387,
-1.69152063815355)) ;
#134050=CARTESIAN_POINT('Ctrl Pts',(-3.35509339356897,1.95,-1.58052296445552)) ;
#134051=CARTESIAN_POINT('Ctrl Pts',(-3.33134808452127,1.95,-1.6776628651052)) ;
#134052=CARTESIAN_POINT('Ctrl Pts',(-3.33134808452128,1.85,-1.6776628651052)) ;
#134053=CARTESIAN_POINT('Origin',(-3.50457525730571,1.91712723223402,-1.61706297559117)) ;
#134054=CARTESIAN_POINT('Origin',(-4.66204490261456,1.95,1.9)) ;
#134055=CARTESIAN_POINT('Origin',(-4.66204490261456,-1.5692190524323,1.9)) ;
#134056=CARTESIAN_POINT('Origin',(-3.84472135955,-1.16055728090002,1.9)) ;
#134057=CARTESIAN_POINT('Origin',(-4.66204490261456,-1.5692190524323,1.9)) ;
#134058=CARTESIAN_POINT('Origin',(-5.3,-2.11180339887499,2.54)) ;
#134059=CARTESIAN_POINT('Origin',(-5.3,-2.11180339887499,-1.9)) ;
#134060=CARTESIAN_POINT('Origin',(-5.3,1.95,-2.1)) ;
#134061=CARTESIAN_POINT('Origin',(-5.3,-1.88819660112501,-2.1)) ;
#134062=CARTESIAN_POINT('Origin',(-4.0264650697994,2.50425327128942,-1.9)) ;
#134063=CARTESIAN_POINT('Origin',(-4.66204490261456,3.21928058320648,-1.9)) ;
#134064=CARTESIAN_POINT('Origin',(-3.02790825149799,1.38087685070033,-1.5005443741715)) ;
#134065=CARTESIAN_POINT('Origin',(-4.66204490261456,3.21928058320648,-1.9)) ;
#134066=CARTESIAN_POINT('Origin',(-4.66204490261456,-1.5692190524323,1.9)) ;
#134067=CARTESIAN_POINT('Origin',(-4.66204490261456,-1.5692190524323,1.9)) ;
#134068=CARTESIAN_POINT('Ctrl Pts',(-5.34460423617422,-2.02230212313483,
-1.89987524812986)) ;
#134069=CARTESIAN_POINT('Ctrl Pts',(-5.4,-2.0499093833863,-1.89983624572346)) ;
#134070=CARTESIAN_POINT('Ctrl Pts',(-5.4,-2.11180321723903,-1.89975033111956)) ;
#134071=CARTESIAN_POINT('Ctrl Pts',(-5.34461954754096,-2.02234798681675,
-1.92615385528167)) ;
#134072=CARTESIAN_POINT('Ctrl Pts',(-5.4,-2.04997459329992,-1.93432433515996)) ;
#134073=CARTESIAN_POINT('Ctrl Pts',(-5.4,-2.11187974550671,-1.95234231302603)) ;
#134074=CARTESIAN_POINT('Ctrl Pts',(-5.33978950165954,-2.00789652656154,
-1.95213503498037)) ;
#134075=CARTESIAN_POINT('Ctrl Pts',(-5.4,-2.02908601268745,-1.96863348546836)) ;
#134076=CARTESIAN_POINT('Ctrl Pts',(-5.4,-2.087770056524,-2.00433878736397)) ;
#134077=CARTESIAN_POINT('Ctrl Pts',(-5.32318090226696,-1.95817527052251,
-1.98921550273188)) ;
#134078=CARTESIAN_POINT('Ctrl Pts',(-5.4,-1.96527310172481,-2.00783661624711)) ;
#134079=CARTESIAN_POINT('Ctrl Pts',(-5.4,-2.00485091174287,-2.07850392511065)) ;
#134080=CARTESIAN_POINT('Ctrl Pts',(-5.31153957531163,-1.92331224822995,
-2.00001353231107)) ;
#134081=CARTESIAN_POINT('Ctrl Pts',(-5.4,-1.92148676945294,-2.01102210746198)) ;
#134082=CARTESIAN_POINT('Ctrl Pts',(-5.4,-1.94671708614656,-2.10006828697156)) ;
#134083=CARTESIAN_POINT('Ctrl Pts',(-5.29976814257746,-1.88802911972917,
-2.00000017262218)) ;
#134084=CARTESIAN_POINT('Ctrl Pts',(-5.4,-1.88802831720455,-1.99976740645701)) ;
#134085=CARTESIAN_POINT('Ctrl Pts',(-5.4,-1.8879174628307,-2.09999983753763)) ;
#134086=CARTESIAN_POINT('Origin',(-5.30000000000002,-1.88819660112507,-1.90000000000004)) ;
#134087=CARTESIAN_POINT('Origin',(-4.66204490261456,3.21928058320648,-1.9)) ;
#134088=CARTESIAN_POINT('Origin',(-4.66204490261456,3.21928058320648,-1.9)) ;
#134089=CARTESIAN_POINT('Origin',(0.175392621986784,-0.95,0.717515271764115)) ;
#134090=CARTESIAN_POINT('Origin',(-3.37639320225,-0.95,1.58572958435533)) ;
#134091=CARTESIAN_POINT('Origin',(-3.32804538583365,-0.902219294041845,
1.57391122923133)) ;
#134092=CARTESIAN_POINT('Origin',(-3.46583592134999,-0.971114561800017,
1.60759336013533)) ;
#134093=CARTESIAN_POINT('Origin',(-3.24472135955,-0.860557280900019,-1.9)) ;
#134094=CARTESIAN_POINT('Origin',(-4.66204490261456,-1.5692190524323,-1.9)) ;
#134095=CARTESIAN_POINT('Origin',(-4.66204490261456,1.95,-1.9)) ;
#134096=CARTESIAN_POINT('Origin',(-4.66204490261456,-1.5692190524323,-1.9)) ;
#134097=CARTESIAN_POINT('Ctrl Pts',(-3.4211145618,-1.06055728090001,1.60759336013533)) ;
#134098=CARTESIAN_POINT('Ctrl Pts',(-3.40394191641935,-1.05197095820969,
1.69540802401362)) ;
#134099=CARTESIAN_POINT('Ctrl Pts',(-3.44209061230229,-0.971114561800017,
1.70473326078501)) ;
#134100=CARTESIAN_POINT('Ctrl Pts',(-3.40727897628736,-1.05363948814369,
1.6008292960084)) ;
#134101=CARTESIAN_POINT('Ctrl Pts',(-3.38665319245547,-1.04670310838586,
1.69118189148914)) ;
#134102=CARTESIAN_POINT('Ctrl Pts',(-3.41441594520969,-0.957277229261624,
1.69796834216237)) ;
#134103=CARTESIAN_POINT('Ctrl Pts',(-3.3918627446443,-1.05,1.5932924717481)) ;
#134104=CARTESIAN_POINT('Ctrl Pts',(-3.36870744055524,-1.04639008266723,
1.68679515213573)) ;
#134105=CARTESIAN_POINT('Ctrl Pts',(-3.38358960366098,-0.950000000886305,
1.69043301422824)) ;
#134106=CARTESIAN_POINT('Ctrl Pts',(-3.37639320225,-1.05,1.58572958435533)) ;
#134107=CARTESIAN_POINT('Ctrl Pts',(-3.3526478932023,-1.05,1.68286948500501)) ;
#134108=CARTESIAN_POINT('Ctrl Pts',(-3.3526478932023,-0.95,1.68286948500501)) ;
#134109=CARTESIAN_POINT('Origin',(-3.3763932022502,-1.14999999999944,1.58572958435544)) ;
#134110=CARTESIAN_POINT('Origin',(-4.66204490261456,-1.5692190524323,-1.9)) ;
#134111=CARTESIAN_POINT('Origin',(-4.66204490261456,-1.5692190524323,-1.9)) ;
#134112=CARTESIAN_POINT('Origin',(-3.37639320225,-1.15,0.)) ;
#134113=CARTESIAN_POINT('Origin',(-3.37639320224909,-1.15000000000409,-1.58572958435489)) ;
#134114=CARTESIAN_POINT('Origin',(-1.50751564693271,0.00804557540861825,
-1.1288928486111)) ;
#134115=CARTESIAN_POINT('Origin',(-3.46583592134999,-0.971114561800017,
-1.60759336013533)) ;
#134116=CARTESIAN_POINT('Ctrl Pts',(-3.37639320225,-1.05,-1.58572958435533)) ;
#134117=CARTESIAN_POINT('Ctrl Pts',(-3.3526478932023,-1.05,-1.68286948500501)) ;
#134118=CARTESIAN_POINT('Ctrl Pts',(-3.3526478932023,-0.95,-1.68286948500501)) ;
#134119=CARTESIAN_POINT('Ctrl Pts',(-3.3918627446443,-1.05,-1.5932924717481)) ;
#134120=CARTESIAN_POINT('Ctrl Pts',(-3.36870744055523,-1.04639008266724,
-1.68679515213575)) ;
#134121=CARTESIAN_POINT('Ctrl Pts',(-3.38358960366098,-0.950000000886305,
-1.69043301422824)) ;
#134122=CARTESIAN_POINT('Ctrl Pts',(-3.40727897628736,-1.05363948814369,
-1.6008292960084)) ;
#134123=CARTESIAN_POINT('Ctrl Pts',(-3.38665319245549,-1.04670310838585,
-1.69118189148912)) ;
#134124=CARTESIAN_POINT('Ctrl Pts',(-3.4144159452097,-0.957277229261623,
-1.69796834216237)) ;
#134125=CARTESIAN_POINT('Ctrl Pts',(-3.4211145618,-1.06055728090001,-1.60759336013533)) ;
#134126=CARTESIAN_POINT('Ctrl Pts',(-3.40394191641936,-1.05197095820969,
-1.69540802401362)) ;
#134127=CARTESIAN_POINT('Ctrl Pts',(-3.4420906123023,-0.971114561800017,
-1.70473326078501)) ;
#134128=CARTESIAN_POINT('Origin',(-3.37639320225,-0.95,-1.58572958435533)) ;
#134129=CARTESIAN_POINT('Origin',(0.175392621986784,-0.95,-0.717515271764115)) ;
#134130=CARTESIAN_POINT('Origin',(12.7,2.65,2.54)) ;
#134131=CARTESIAN_POINT('Origin',(12.8,2.65,-1.49304604217164)) ;
#134132=CARTESIAN_POINT('',(4.57524318173533,2.73534903669982,-1.44093518020973)) ;
#134133=CARTESIAN_POINT('Origin',(4.65232986200348,2.66527023615519,-1.48875421118475)) ;
#134134=CARTESIAN_POINT('Ctrl Pts',(4.57524318173533,2.73534903669982,-1.44093518020973)) ;
#134135=CARTESIAN_POINT('Ctrl Pts',(4.5761458558036,2.73452842391049,-1.43959115118323)) ;
#134136=CARTESIAN_POINT('Ctrl Pts',(4.57705238626145,2.73367683201792,-1.43826812933933)) ;
#134137=CARTESIAN_POINT('Ctrl Pts',(4.5779495181309,2.73280244902547,-1.43697684888884)) ;
#134138=CARTESIAN_POINT('Ctrl Pts',(4.58144263576937,2.72939790755538,-1.43194905456852)) ;
#134139=CARTESIAN_POINT('Ctrl Pts',(4.58496694799988,2.72549786515178,-1.4271699445179)) ;
#134140=CARTESIAN_POINT('Ctrl Pts',(4.58815670056909,2.72107165565041,-1.42269819385267)) ;
#134141=CARTESIAN_POINT('Ctrl Pts',(4.59069123847476,2.71755464437251,-1.41914499612971)) ;
#134142=CARTESIAN_POINT('Ctrl Pts',(4.59301454561855,2.71370459823904,-1.41578631272423)) ;
#134143=CARTESIAN_POINT('Ctrl Pts',(4.5949431309995,2.70950205848693,-1.41267499616739)) ;
#134144=CARTESIAN_POINT('Ctrl Pts',(4.59651854606292,2.70606910472949,-1.41013343642151)) ;
#134145=CARTESIAN_POINT('Ctrl Pts',(4.59783685868317,2.70233705077434,-1.40771608615721)) ;
#134146=CARTESIAN_POINT('Ctrl Pts',(4.5987311897142,2.69838744820012,-1.4055323012124)) ;
#134147=CARTESIAN_POINT('Ctrl Pts',(4.59916508318196,2.69647125978917,-1.40447281653651)) ;
#134148=CARTESIAN_POINT('Ctrl Pts',(4.59949917984822,2.69450444432192,-1.40346779888205)) ;
#134149=CARTESIAN_POINT('Ctrl Pts',(4.5997144226265,2.69249922659198,-1.40252634409943)) ;
#134150=CARTESIAN_POINT('Ctrl Pts',(4.59990113259977,2.6907598225955,-1.40170968953523)) ;
#134151=CARTESIAN_POINT('Ctrl Pts',(4.6,2.68896788689974,-1.40093031221453)) ;
#134152=CARTESIAN_POINT('Ctrl Pts',(4.6,2.68715716172261,-1.40020561276333)) ;
#134153=CARTESIAN_POINT('Origin',(4.5,2.1,-1.38195395782836)) ;
#134154=CARTESIAN_POINT('Origin',(4.6,2.1,-1.38195395782836)) ;
#134155=CARTESIAN_POINT('Origin',(12.7,2.1,-1.38195395782836)) ;
#134156=CARTESIAN_POINT('Origin',(12.7,2.76643989873054,-1.47363939238321)) ;
#134157=CARTESIAN_POINT('Origin',(12.7,2.13287979746107,-1.57923274259479)) ;
#134158=CARTESIAN_POINT('Origin',(4.4,2.72431432344521,0.)) ;
#134159=CARTESIAN_POINT('Ctrl Pts',(4.48762159086959,2.77250619842349,1.38882431825052)) ;
#134160=CARTESIAN_POINT('Ctrl Pts',(4.48806820038223,2.77169418112776,1.38616443291017)) ;
#134161=CARTESIAN_POINT('Ctrl Pts',(4.48852084821546,2.77084293101113,1.38351728498153)) ;
#134162=CARTESIAN_POINT('Ctrl Pts',(4.49012932137855,2.76769877392855,1.37423699047925)) ;
#134163=CARTESIAN_POINT('Ctrl Pts',(4.49131046584975,2.76517764467227,1.36765586829652)) ;
#134164=CARTESIAN_POINT('Ctrl Pts',(4.49351977821777,2.75978760391029,1.35536471983786)) ;
#134165=CARTESIAN_POINT('Ctrl Pts',(4.49455195297829,2.75697653750121,1.34963225939859)) ;
#134166=CARTESIAN_POINT('Ctrl Pts',(4.49620670090467,2.75163165728869,1.34005667839666)) ;
#134167=CARTESIAN_POINT('Ctrl Pts',(4.49686252944493,2.74924176842721,1.33613597379662)) ;
#134168=CARTESIAN_POINT('Ctrl Pts',(4.49822764032851,2.74331716058947,1.32735536836523)) ;
#134169=CARTESIAN_POINT('Ctrl Pts',(4.49890203357906,2.73961076902699,1.32251349983941)) ;
#134170=CARTESIAN_POINT('Ctrl Pts',(4.49975897856023,2.73206576252672,1.31417222156017)) ;
#134171=CARTESIAN_POINT('Ctrl Pts',(4.5,2.72833175948612,1.31058099770818)) ;
#134172=CARTESIAN_POINT('Ctrl Pts',(4.5,2.72431432344521,1.30736518335501)) ;
#134173=CARTESIAN_POINT('Ctrl Pts',(4.5,2.72431432344521,-1.30736518335501)) ;
#134174=CARTESIAN_POINT('Ctrl Pts',(4.5,2.72904669151435,-1.31115327531372)) ;
#134175=CARTESIAN_POINT('Ctrl Pts',(4.49966645684473,2.73338556955569,-1.31546141017617)) ;
#134176=CARTESIAN_POINT('Ctrl Pts',(4.49869539480391,2.74072289096386,-1.32398024143758)) ;
#134177=CARTESIAN_POINT('Ctrl Pts',(4.49811062025686,2.74382502998089,-1.3281080596587)) ;
#134178=CARTESIAN_POINT('Ctrl Pts',(4.49664125196625,2.75020211699688,-1.33755926494058)) ;
#134179=CARTESIAN_POINT('Ctrl Pts',(4.4957072138971,2.75339870015142,-1.34301039031936)) ;
#134180=CARTESIAN_POINT('Ctrl Pts',(4.49363760641476,2.7595286326395,-1.35475170518698)) ;
#134181=CARTESIAN_POINT('Ctrl Pts',(4.49249077386341,2.76240287369075,-1.36107122583085)) ;
#134182=CARTESIAN_POINT('Ctrl Pts',(4.49055019898871,2.7667775727014,-1.37191412562091)) ;
#134183=CARTESIAN_POINT('Ctrl Pts',(4.48975662823143,2.76842729450635,-1.37638729192265)) ;
#134184=CARTESIAN_POINT('Ctrl Pts',(4.4885208482156,2.77084293101086,-1.38351728498073)) ;
#134185=CARTESIAN_POINT('Ctrl Pts',(4.48806820038252,2.77169418112725,-1.38616443290854)) ;
#134186=CARTESIAN_POINT('Ctrl Pts',(4.48762159086959,2.77250619842348,-1.38882431824782)) ;
#134187=CARTESIAN_POINT('Origin',(4.6,2.1,0.)) ;
#134188=CARTESIAN_POINT('Origin',(4.6,2.1,1.38195395782836)) ;
#134189=CARTESIAN_POINT('Origin',(4.6,2.1,-1.38195395782836)) ;
#134190=CARTESIAN_POINT('Origin',(12.7,2.1,-1.38195395782836)) ;
#134191=CARTESIAN_POINT('Origin',(12.7,1.9,-1.38195395782836)) ;
#134192=CARTESIAN_POINT('Origin',(12.7,2.65,2.54)) ;
#134193=CARTESIAN_POINT('Origin',(4.5,2.65,1.49304604217164)) ;
#134194=CARTESIAN_POINT('',(4.6,2.68715716172261,1.40020561276332)) ;
#134195=CARTESIAN_POINT('',(4.57524318173443,2.73534903670064,1.44093518021108)) ;
#134196=CARTESIAN_POINT('Ctrl Pts',(4.6,2.68715716172261,1.40020561276333)) ;
#134197=CARTESIAN_POINT('Ctrl Pts',(4.6,2.69106036671412,1.40176777722153)) ;
#134198=CARTESIAN_POINT('Ctrl Pts',(4.59952510519173,2.69488861888988,1.4035902905253)) ;
#134199=CARTESIAN_POINT('Ctrl Pts',(4.59869497748254,2.6985274364077,1.40560984877499)) ;
#134200=CARTESIAN_POINT('Ctrl Pts',(4.59815316003464,2.70090246232127,1.40692799763887)) ;
#134201=CARTESIAN_POINT('Ctrl Pts',(4.59746001108778,2.70319720658047,1.40832903195479)) ;
#134202=CARTESIAN_POINT('Ctrl Pts',(4.59664880273703,2.7053865971179,1.40978545810151)) ;
#134203=CARTESIAN_POINT('Ctrl Pts',(4.59612777291939,2.70679281754376,1.41072090390766)) ;
#134204=CARTESIAN_POINT('Ctrl Pts',(4.59555051815356,2.70817855133085,1.41169507009278)) ;
#134205=CARTESIAN_POINT('Ctrl Pts',(4.59494172533681,2.70950512149367,1.41267726393019)) ;
#134206=CARTESIAN_POINT('Ctrl Pts',(4.59250947890865,2.71480502887008,1.4166013205009)) ;
#134207=CARTESIAN_POINT('Ctrl Pts',(4.58944857812999,2.7195451700524,1.42091766241906)) ;
#134208=CARTESIAN_POINT('Ctrl Pts',(4.58612768646826,2.72376361218902,1.42552619681616)) ;
#134209=CARTESIAN_POINT('Ctrl Pts',(4.58350334758184,2.72709724148709,1.42916809702239)) ;
#134210=CARTESIAN_POINT('Ctrl Pts',(4.58071664514667,2.73010548898771,1.43299400406844)) ;
#134211=CARTESIAN_POINT('Ctrl Pts',(4.5779495181309,2.73280244902548,1.43697684888885)) ;
#134212=CARTESIAN_POINT('Ctrl Pts',(4.57705238626115,2.73367683201822,1.43826812933977)) ;
#134213=CARTESIAN_POINT('Ctrl Pts',(4.576145855803,2.73452842391106,1.43959115118411)) ;
#134214=CARTESIAN_POINT('Ctrl Pts',(4.57524318173443,2.73534903670064,1.44093518021108)) ;
#134215=CARTESIAN_POINT('Origin',(4.65232986199958,2.66527023615875,1.48875421118384)) ;
#134216=CARTESIAN_POINT('Origin',(4.6,2.65,1.49304604217164)) ;
#134217=CARTESIAN_POINT('Origin',(12.7,1.9,-1.5)) ;
#134218=CARTESIAN_POINT('Origin',(12.7,2.01643989873054,1.59863939238321)) ;
#134219=CARTESIAN_POINT('Origin',(-3.65,10.7,0.75)) ;
#134220=CARTESIAN_POINT('Origin',(-3.65,10.7,0.75)) ;
#134221=CARTESIAN_POINT('Origin',(-3.65,10.7,0.75)) ;
#134222=CARTESIAN_POINT('Origin',(0.,10.7,0.75)) ;
#134223=CARTESIAN_POINT('Origin',(-2.9,10.7,0.75)) ;
#134224=CARTESIAN_POINT('Origin',(-3.65,10.7,0.)) ;
#134225=CARTESIAN_POINT('Origin',(-3.65,10.7,-0.75)) ;
#134226=CARTESIAN_POINT('Origin',(-2.9,10.7,0.75)) ;
#134227=CARTESIAN_POINT('Origin',(-2.9,10.7,0.75)) ;
#134228=CARTESIAN_POINT('Origin',(-3.65,10.7,-0.750000000000001)) ;
#134229=CARTESIAN_POINT('Origin',(-3.65,10.7,-0.750000000000001)) ;
#134230=CARTESIAN_POINT('Origin',(-2.9,10.7,0.)) ;
#134231=CARTESIAN_POINT('Origin',(-2.9,10.7,-0.750000000000001)) ;
#134232=CARTESIAN_POINT('Origin',(0.,10.7,-0.750000000000001)) ;
#134233=CARTESIAN_POINT('Origin',(-2.9,10.7,-0.750000000000001)) ;
#134234=CARTESIAN_POINT('Origin',(-2.9,10.7,-0.750000000000001)) ;
#134235=CARTESIAN_POINT('Origin',(-3.05,-3.95,1.)) ;
#134236=CARTESIAN_POINT('Origin',(-3.05,-3.95,-0.900000000000001)) ;
#134237=CARTESIAN_POINT('Origin',(-3.05,-3.95,0.9)) ;
#134238=CARTESIAN_POINT('Origin',(-3.25,-3.95,0.9)) ;
#134239=CARTESIAN_POINT('Origin',(-3.25,-3.95,1.1)) ;
#134240=CARTESIAN_POINT('Origin',(-3.25,-3.95,0.9)) ;
#134241=CARTESIAN_POINT('Origin',(-3.25,-3.95,-0.900000000000001)) ;
#134242=CARTESIAN_POINT('Origin',(-3.25,-3.95,-0.900000000000001)) ;
#134243=CARTESIAN_POINT('Origin',(-3.25,-3.95,-1.1)) ;
#134244=CARTESIAN_POINT('Origin',(-4.4,-3.95,1.1)) ;
#134245=CARTESIAN_POINT('Origin',(-4.3,-3.95,1.1)) ;
#134246=CARTESIAN_POINT('Origin',(-3.25,-3.9,0.9)) ;
#134247=CARTESIAN_POINT('Origin',(-3.25,-3.85,0.9)) ;
#134248=CARTESIAN_POINT('Origin',(-3.25,-3.85,-1.40946282423115E-15)) ;
#134249=CARTESIAN_POINT('Origin',(-3.25,-3.85,-0.900000000000001)) ;
#134250=CARTESIAN_POINT('Origin',(-3.25,-3.85,0.9)) ;
#134251=CARTESIAN_POINT('Origin',(-3.25,-3.9,-0.900000000000001)) ;
#134252=CARTESIAN_POINT('Origin',(-3.25,-3.85,-0.900000000000001)) ;
#134253=CARTESIAN_POINT('Origin',(-4.4,-3.95,-1.1)) ;
#134254=CARTESIAN_POINT('Origin',(-4.3,-3.95,-1.1)) ;
#134255=CARTESIAN_POINT('Origin',(-4.5,-3.95,0.999999999999999)) ;
#134256=CARTESIAN_POINT('Origin',(-4.5,-3.95,0.899999999999999)) ;
#134257=CARTESIAN_POINT('Origin',(-4.5,-3.95,-0.900000000000001)) ;
#134258=CARTESIAN_POINT('Origin',(-4.3,-3.95,0.899999999999999)) ;
#134259=CARTESIAN_POINT('Origin',(-4.3,-3.95,0.899999999999999)) ;
#134260=CARTESIAN_POINT('Origin',(-3.25,-3.85,0.9)) ;
#134261=CARTESIAN_POINT('Origin',(-3.25,-3.85,0.9)) ;
#134262=CARTESIAN_POINT('Origin',(-3.25,-3.85,-0.900000000000001)) ;
#134263=CARTESIAN_POINT('Origin',(-3.25,-3.85,-0.900000000000001)) ;
#134264=CARTESIAN_POINT('Origin',(-4.3,-3.95,-0.900000000000001)) ;
#134265=CARTESIAN_POINT('Origin',(-4.3,-3.95,-0.900000000000001)) ;
#134266=CARTESIAN_POINT('Origin',(-4.3,-3.9,0.899999999999999)) ;
#134267=CARTESIAN_POINT('Origin',(-4.3,-3.85,0.899999999999999)) ;
#134268=CARTESIAN_POINT('Origin',(-1.56125112837913E-16,-3.85,0.9)) ;
#134269=CARTESIAN_POINT('Origin',(-4.3,-3.85,0.899999999999999)) ;
#134270=CARTESIAN_POINT('Origin',(-1.56125112837913E-16,-3.85,-0.900000000000001)) ;
#134271=CARTESIAN_POINT('Origin',(-4.3,-3.85,-0.900000000000001)) ;
#134272=CARTESIAN_POINT('Origin',(-4.3,-3.9,-0.900000000000001)) ;
#134273=CARTESIAN_POINT('Origin',(-4.3,-3.85,-0.900000000000001)) ;
#134274=CARTESIAN_POINT('Origin',(-4.3,-3.85,0.899999999999999)) ;
#134275=CARTESIAN_POINT('Origin',(-4.3,-3.85,0.899999999999999)) ;
#134276=CARTESIAN_POINT('Origin',(-4.3,-3.85,-0.900000000000001)) ;
#134277=CARTESIAN_POINT('Origin',(-4.3,-3.85,-0.900000000000001)) ;
#134278=CARTESIAN_POINT('Origin',(-4.3,-3.85,0.)) ;
#134279=CARTESIAN_POINT('Origin',(-4.,10.85,-1.)) ;
#134280=CARTESIAN_POINT('Origin',(-4.,10.85,-0.9)) ;
#134281=CARTESIAN_POINT('Origin',(-4.,10.85,0.9)) ;
#134282=CARTESIAN_POINT('Origin',(-3.8,10.85,0.9)) ;
#134283=CARTESIAN_POINT('Origin',(-3.8,10.85,1.1)) ;
#134284=CARTESIAN_POINT('Origin',(-3.8,10.85,0.9)) ;
#134285=CARTESIAN_POINT('Origin',(-3.8,10.85,-0.9)) ;
#134286=CARTESIAN_POINT('Origin',(-3.8,10.85,-0.9)) ;
#134287=CARTESIAN_POINT('Origin',(-3.8,10.85,-1.1)) ;
#134288=CARTESIAN_POINT('Origin',(-3.9,10.85,1.1)) ;
#134289=CARTESIAN_POINT('Origin',(-2.75,10.85,1.1)) ;
#134290=CARTESIAN_POINT('Origin',(-3.8,10.8,0.9)) ;
#134291=CARTESIAN_POINT('Origin',(-3.8,10.75,0.9)) ;
#134292=CARTESIAN_POINT('Origin',(-3.8,10.75,8.23993651088984E-16)) ;
#134293=CARTESIAN_POINT('Origin',(-3.8,10.75,-0.9)) ;
#134294=CARTESIAN_POINT('Origin',(-3.8,10.75,0.9)) ;
#134295=CARTESIAN_POINT('Origin',(-3.8,10.8,-0.9)) ;
#134296=CARTESIAN_POINT('Origin',(-3.8,10.75,-0.9)) ;
#134297=CARTESIAN_POINT('Origin',(-3.9,10.85,-1.1)) ;
#134298=CARTESIAN_POINT('Origin',(-2.75,10.85,-1.1)) ;
#134299=CARTESIAN_POINT('Origin',(-2.55,10.85,-1.)) ;
#134300=CARTESIAN_POINT('Origin',(-2.55,10.85,0.899999999999999)) ;
#134301=CARTESIAN_POINT('Origin',(-2.55,10.85,-0.900000000000001)) ;
#134302=CARTESIAN_POINT('Origin',(-2.75,10.85,0.899999999999999)) ;
#134303=CARTESIAN_POINT('Origin',(-2.75,10.85,0.899999999999999)) ;
#134304=CARTESIAN_POINT('Origin',(-3.8,10.75,0.9)) ;
#134305=CARTESIAN_POINT('Origin',(-3.8,10.75,0.9)) ;
#134306=CARTESIAN_POINT('Origin',(-3.8,10.75,-0.9)) ;
#134307=CARTESIAN_POINT('Origin',(-3.8,10.75,-0.9)) ;
#134308=CARTESIAN_POINT('Origin',(-2.75,10.85,-0.900000000000001)) ;
#134309=CARTESIAN_POINT('Origin',(-2.75,10.85,-0.900000000000001)) ;
#134310=CARTESIAN_POINT('Origin',(-2.75,10.8,0.899999999999999)) ;
#134311=CARTESIAN_POINT('Origin',(-2.75,10.75,0.899999999999999)) ;
#134312=CARTESIAN_POINT('Origin',(1.56125112837912E-16,10.75,0.899999999999999)) ;
#134313=CARTESIAN_POINT('Origin',(-2.75,10.75,0.899999999999999)) ;
#134314=CARTESIAN_POINT('Origin',(-1.56125112837913E-16,10.75,-0.900000000000001)) ;
#134315=CARTESIAN_POINT('Origin',(-2.75,10.75,-0.900000000000001)) ;
#134316=CARTESIAN_POINT('Origin',(-2.75,10.8,-0.900000000000001)) ;
#134317=CARTESIAN_POINT('Origin',(-2.75,10.75,-0.900000000000001)) ;
#134318=CARTESIAN_POINT('Origin',(-2.75,10.75,0.899999999999999)) ;
#134319=CARTESIAN_POINT('Origin',(-2.75,10.75,0.899999999999999)) ;
#134320=CARTESIAN_POINT('Origin',(-2.75,10.75,-0.900000000000001)) ;
#134321=CARTESIAN_POINT('Origin',(-2.75,10.75,-0.900000000000001)) ;
#134322=CARTESIAN_POINT('Origin',(-2.75,10.75,5.96311194867028E-16)) ;
#134323=CARTESIAN_POINT('Origin',(4.6,0.,0.)) ;
#134324=CARTESIAN_POINT('Ctrl Pts',(4.5,-2.7,1.52315462117279)) ;
#134325=CARTESIAN_POINT('Ctrl Pts',(4.5,-2.71827986285823,1.44803526082493)) ;
#134326=CARTESIAN_POINT('Ctrl Pts',(4.50597963419107,-2.73556801027185,
1.37326013954719)) ;
#134327=CARTESIAN_POINT('Ctrl Pts',(4.52394923367545,-2.75977758633329,
1.26156316597844)) ;
#134328=CARTESIAN_POINT('Ctrl Pts',(4.53141024883993,-2.76757607569523,
1.22431671760971)) ;
#134329=CARTESIAN_POINT('Ctrl Pts',(4.54734065524867,-2.77857284247615,
1.16983431041704)) ;
#134330=CARTESIAN_POINT('Ctrl Pts',(4.55339248498575,-2.78214991573955,
1.15176172558506)) ;
#134331=CARTESIAN_POINT('Ctrl Pts',(4.56567492147096,-2.787183259287,1.12585327813928)) ;
#134332=CARTESIAN_POINT('Ctrl Pts',(4.57024691433051,-2.78880341224557,
1.11742739494919)) ;
#134333=CARTESIAN_POINT('Ctrl Pts',(4.58215938980081,-2.79169669265294,
1.10225652011491)) ;
#134334=CARTESIAN_POINT('Ctrl Pts',(4.59005470866978,-2.79310344827587,
1.09479364595774)) ;
#134335=CARTESIAN_POINT('Ctrl Pts',(4.6,-2.79310344827586,1.09479364595777)) ;
#134336=CARTESIAN_POINT('Origin',(4.6,-2.4,1.96214168703486)) ;
#134337=CARTESIAN_POINT('Origin',(4.6,-2.4,2.54)) ;
#134338=CARTESIAN_POINT('Origin',(4.6,-2.4,1.96214168703486)) ;
#134339=CARTESIAN_POINT('Origin',(4.6,-2.4,1.96214168703486)) ;
#134340=CARTESIAN_POINT('Origin',(4.6,-2.4,1.96214168703486)) ;
#134341=CARTESIAN_POINT('Origin',(0.584645609909622,-2.4,1.96214168703486)) ;
#134342=CARTESIAN_POINT('Origin',(12.7,-2.4,1.96214168703486)) ;
#134343=CARTESIAN_POINT('Origin',(12.7,-2.2,2.54)) ;
#134344=CARTESIAN_POINT('Origin',(12.7,-2.2,1.96214168703486)) ;
#134345=CARTESIAN_POINT('Origin',(12.7,-2.4,1.96214168703486)) ;
#134346=CARTESIAN_POINT('Origin',(12.7,-2.24516129032258,1.83555190077454)) ;
#134347=CARTESIAN_POINT('Origin',(12.7,0.,0.)) ;
#134348=CARTESIAN_POINT('Origin',(12.7,-2.24516129032258,-1.83555190077454)) ;
#134349=CARTESIAN_POINT('Origin',(12.7,-2.2,2.54)) ;
#134350=CARTESIAN_POINT('Origin',(12.7,-2.2,-3.11785831296514)) ;
#134351=CARTESIAN_POINT('Origin',(12.7,-2.2,-1.96214168703486)) ;
#134352=CARTESIAN_POINT('Origin',(12.7,-2.4,-1.96214168703486)) ;
#134353=CARTESIAN_POINT('Origin',(12.7,-2.4,-1.96214168703486)) ;
#134354=CARTESIAN_POINT('Origin',(0.584645609909622,-2.4,-1.96214168703486)) ;
#134355=CARTESIAN_POINT('Origin',(4.6,-2.4,-1.96214168703486)) ;
#134356=CARTESIAN_POINT('Origin',(4.6,-2.4,2.54)) ;
#134357=CARTESIAN_POINT('Origin',(4.6,-2.4,-3.11785831296514)) ;
#134358=CARTESIAN_POINT('Origin',(4.6,-2.4,-1.96214168703486)) ;
#134359=CARTESIAN_POINT('Origin',(4.6,-2.4,-1.96214168703486)) ;
#134360=CARTESIAN_POINT('Origin',(4.6,-2.4,-1.96214168703486)) ;
#134361=CARTESIAN_POINT('Origin',(4.6,0.,0.)) ;
#134362=CARTESIAN_POINT('Ctrl Pts',(4.6,-2.79310344827586,-1.09479364595777)) ;
#134363=CARTESIAN_POINT('Ctrl Pts',(4.59007568892311,-2.79310344827586,
-1.09479364595777)) ;
#134364=CARTESIAN_POINT('Ctrl Pts',(4.58219207637239,-2.79170232102182,
-1.10222674227604)) ;
#134365=CARTESIAN_POINT('Ctrl Pts',(4.57028631514659,-2.78881527838255,
-1.11736543899001)) ;
#134366=CARTESIAN_POINT('Ctrl Pts',(4.56571532154372,-2.78719767797524,
-1.12577848858352)) ;
#134367=CARTESIAN_POINT('Ctrl Pts',(4.55343865632726,-2.78217307830036,
-1.15164363330887)) ;
#134368=CARTESIAN_POINT('Ctrl Pts',(4.54738888873343,-2.77860151743012,
-1.16969008596606)) ;
#134369=CARTESIAN_POINT('Ctrl Pts',(4.53146440752601,-2.76762263748298,
-1.2240903156831)) ;
#134370=CARTESIAN_POINT('Ctrl Pts',(4.52400917967609,-2.75984503873828,
-1.26124550630579)) ;
#134371=CARTESIAN_POINT('Ctrl Pts',(4.50599905604505,-2.7356206423885,-1.37303013546926)) ;
#134372=CARTESIAN_POINT('Ctrl Pts',(4.5,-2.71826422026483,-1.4480995425769)) ;
#134373=CARTESIAN_POINT('Ctrl Pts',(4.5,-2.7,-1.52315462117279)) ;
#134374=CARTESIAN_POINT('Origin',(3.7,-2.9,2.54)) ;
#134375=CARTESIAN_POINT('Origin',(3.7,-2.9,-7.62)) ;
#134376=CARTESIAN_POINT('Origin',(3.5,-3.95,2.54)) ;
#134377=CARTESIAN_POINT('Origin',(3.5,-3.95,-7.62)) ;
#134378=CARTESIAN_POINT('Origin',(-5.3,-3.95,2.54)) ;
#134379=CARTESIAN_POINT('Origin',(-5.3,-3.95,-7.62)) ;
#134380=CARTESIAN_POINT('Origin',(-5.3,5.19009804864072,2.54)) ;
#134381=CARTESIAN_POINT('Origin',(-5.3,5.19009804864072,-7.62)) ;
#134382=CARTESIAN_POINT('Origin',(-4.8,10.3,2.54)) ;
#134383=CARTESIAN_POINT('Origin',(-4.8,10.3,-7.62)) ;
#134384=CARTESIAN_POINT('Origin',(-4.8,10.85,2.54)) ;
#134385=CARTESIAN_POINT('Origin',(-4.8,10.85,-7.62)) ;
#134386=CARTESIAN_POINT('Origin',(-0.362523114814661,9.05,-0.169047304696279)) ;
#134387=CARTESIAN_POINT('Origin',(0.36252311481466,9.05,0.169047304696279)) ;
#134388=CARTESIAN_POINT('Origin',(-1.31845674202095,9.85,1.40771865776493)) ;
#134389=CARTESIAN_POINT('Origin',(-0.230887397576972,9.85,1.91486057185377)) ;
#134390=CARTESIAN_POINT('Origin',(3.3,10.85,2.54)) ;
#134391=CARTESIAN_POINT('Origin',(3.3,10.85,-7.62)) ;
#134392=CARTESIAN_POINT('Origin',(3.85,6.92431432344521,2.54)) ;
#134393=CARTESIAN_POINT('Origin',(3.85,6.92431432344521,-7.62)) ;
#134394=CARTESIAN_POINT('Origin',(4.05,3.77568567655479,2.54)) ;
#134395=CARTESIAN_POINT('Origin',(4.05,3.77568567655479,-7.62)) ;
#134396=CARTESIAN_POINT('Origin',(4.6,2.1,1.38195395782836)) ;
#134397=CARTESIAN_POINT('Origin',(4.6,2.1,1.38195395782836)) ;
#134398=CARTESIAN_POINT('Origin',(4.6,0.280857398566761,1.68514439140057)) ;
#134399=CARTESIAN_POINT('Origin',(4.6,2.61712020253893,1.29576725740521)) ;
#134400=CARTESIAN_POINT('Origin',(4.6,2.65,1.49304604217164)) ;
#134401=CARTESIAN_POINT('Origin',(4.6,2.72431432344521,1.30736518335501)) ;
#134402=CARTESIAN_POINT('Ctrl Pts',(4.48762159086906,2.77250619842445,1.38882431825039)) ;
#134403=CARTESIAN_POINT('Ctrl Pts',(4.51316716229104,2.72605970493114,1.42576120580283)) ;
#134404=CARTESIAN_POINT('Ctrl Pts',(4.57527453405851,2.73535372386122,1.44094284680199)) ;
#134405=CARTESIAN_POINT('Ctrl Pts',(4.49363662433156,2.76156977394745,1.3530004075283)) ;
#134406=CARTESIAN_POINT('Ctrl Pts',(4.5146945995807,2.70766535161865,1.40379915260673)) ;
#134407=CARTESIAN_POINT('Ctrl Pts',(4.58732693581885,2.72440392220678,1.42300495876594)) ;
#134408=CARTESIAN_POINT('Ctrl Pts',(4.5,2.74488438438029,1.32383078393385)) ;
#134409=CARTESIAN_POINT('Ctrl Pts',(4.50856472873626,2.69031482079672,1.40150888629529)) ;
#134410=CARTESIAN_POINT('Ctrl Pts',(4.60003980620507,2.70775073269832,1.40844768862527)) ;
#134411=CARTESIAN_POINT('Ctrl Pts',(4.5,2.72431432344521,1.30736518335501)) ;
#134412=CARTESIAN_POINT('Ctrl Pts',(4.5,2.68714136424467,1.4002450841483)) ;
#134413=CARTESIAN_POINT('Ctrl Pts',(4.60004250625997,2.68715716507935,1.4002056043762)) ;
#134414=CARTESIAN_POINT('Origin',(4.57524318173443,2.82069807340128,1.38882431825052)) ;
#134415=CARTESIAN_POINT('Ctrl Pts',(4.47150553123747,2.80180812502279,1.49304604217164)) ;
#134416=CARTESIAN_POINT('Ctrl Pts',(4.5,2.75,1.49304604217164)) ;
#134417=CARTESIAN_POINT('Ctrl Pts',(4.55912712210514,2.75,1.49304604217164)) ;
#134418=CARTESIAN_POINT('Ctrl Pts',(4.47150553186688,2.8018081238784,1.45642552726532)) ;
#134419=CARTESIAN_POINT('Ctrl Pts',(4.50000000073523,2.74999999866316,1.46874191573125)) ;
#134420=CARTESIAN_POINT('Ctrl Pts',(4.5591271227348,2.75,1.47472795424071)) ;
#134421=CARTESIAN_POINT('Ctrl Pts',(4.47712448971609,2.79159183687984,1.42008346264768)) ;
#134422=CARTESIAN_POINT('Ctrl Pts',(4.50480340096852,2.74126654369362,1.44446204900192)) ;
#134423=CARTESIAN_POINT('Ctrl Pts',(4.56473907811159,2.74489822224645,1.45657517841774)) ;
#134424=CARTESIAN_POINT('Ctrl Pts',(4.48762159086676,2.77250619842407,1.38882431825052)) ;
#134425=CARTESIAN_POINT('Ctrl Pts',(4.51315802400618,2.72607631998876,1.4257479925657)) ;
#134426=CARTESIAN_POINT('Ctrl Pts',(4.57524318173443,2.73534903670064,1.44093518021108)) ;
#134427=CARTESIAN_POINT('Origin',(4.55912712210513,2.85,1.49304604217164)) ;
#134428=CARTESIAN_POINT('Origin',(4.55912712210514,2.85,2.54)) ;
#134429=CARTESIAN_POINT('Origin',(4.55912712210514,2.85,2.54)) ;
#134430=CARTESIAN_POINT('Origin',(4.55912712210513,2.85,-3.58695395782836)) ;
#134431=CARTESIAN_POINT('Origin',(4.55912712210514,2.85,-1.49304604217164)) ;
#134432=CARTESIAN_POINT('Ctrl Pts',(4.48762159086766,2.77250619842243,-1.38882431824783)) ;
#134433=CARTESIAN_POINT('Ctrl Pts',(4.51315802400691,2.72607631998743,-1.42574799256407)) ;
#134434=CARTESIAN_POINT('Ctrl Pts',(4.57524318173533,2.73534903669982,-1.44093518020973)) ;
#134435=CARTESIAN_POINT('Ctrl Pts',(4.47712448971642,2.79159183687923,-1.42008346264562)) ;
#134436=CARTESIAN_POINT('Ctrl Pts',(4.5048034009688,2.74126654369307,-1.44446204900057)) ;
#134437=CARTESIAN_POINT('Ctrl Pts',(4.56473907811194,2.74489822224616,-1.45657517841671)) ;
#134438=CARTESIAN_POINT('Ctrl Pts',(4.47150553186688,2.8018081238784,-1.45642552726424)) ;
#134439=CARTESIAN_POINT('Ctrl Pts',(4.50000000073523,2.74999999866316,-1.46874191573051)) ;
#134440=CARTESIAN_POINT('Ctrl Pts',(4.5591271227348,2.75,-1.47472795424017)) ;
#134441=CARTESIAN_POINT('Ctrl Pts',(4.47150553123747,2.80180812502279,-1.49304604217164)) ;
#134442=CARTESIAN_POINT('Ctrl Pts',(4.5,2.75,-1.49304604217164)) ;
#134443=CARTESIAN_POINT('Ctrl Pts',(4.55912712210513,2.75,-1.49304604217164)) ;
#134444=CARTESIAN_POINT('Origin',(4.57524318173533,2.82069807339964,-1.38882431824783)) ;
#134445=CARTESIAN_POINT('Ctrl Pts',(4.57527448145476,2.73535371598842,-1.44094283394186)) ;
#134446=CARTESIAN_POINT('Ctrl Pts',(4.51316714695682,2.72605973281052,-1.42576118362916)) ;
#134447=CARTESIAN_POINT('Ctrl Pts',(4.48762159086951,2.77250619842363,-1.3888243182477)) ;
#134448=CARTESIAN_POINT('Ctrl Pts',(4.58732687742634,2.72440390874891,-1.42300494332461)) ;
#134449=CARTESIAN_POINT('Ctrl Pts',(4.51469458626358,2.70766538570651,-1.40379912048168)) ;
#134450=CARTESIAN_POINT('Ctrl Pts',(4.49363662433186,2.76156977394666,-1.35300040752687)) ;
#134451=CARTESIAN_POINT('Ctrl Pts',(4.60003973844306,2.70775071978181,-1.40844768348499)) ;
#134452=CARTESIAN_POINT('Ctrl Pts',(4.50856472285792,2.69031485824818,-1.40150883298414)) ;
#134453=CARTESIAN_POINT('Ctrl Pts',(4.5,2.74488438437976,-1.32383078393342)) ;
#134454=CARTESIAN_POINT('Ctrl Pts',(4.60004243494348,2.6871571650681,-1.40020560440432)) ;
#134455=CARTESIAN_POINT('Ctrl Pts',(4.5,2.68714139075512,-1.40024501790962)) ;
#134456=CARTESIAN_POINT('Ctrl Pts',(4.5,2.72431432344521,-1.30736518335501)) ;
#134457=CARTESIAN_POINT('Origin',(4.6,0.280857398566761,-1.68514439140057)) ;
#134458=CARTESIAN_POINT('Origin',(4.6,2.1,-1.38195395782836)) ;
#134459=CARTESIAN_POINT('Origin',(4.6,2.1,-1.38195395782836)) ;
#134460=CARTESIAN_POINT('Origin',(4.6,0.,0.)) ;
#134461=CARTESIAN_POINT('',(4.5,-2.9,-3.84865454255039E-12)) ;
#134462=CARTESIAN_POINT('',(4.57439618084313,-2.80937499999937,-1.04279586712545)) ;
#134463=CARTESIAN_POINT('Ctrl Pts',(4.5,-2.9,-3.84865454255039E-12)) ;
#134464=CARTESIAN_POINT('Ctrl Pts',(4.5,-2.9000000234111,-0.176176262570291)) ;
#134465=CARTESIAN_POINT('Ctrl Pts',(4.49893459747296,-2.89187728142186,
-0.352293822555195)) ;
#134466=CARTESIAN_POINT('Ctrl Pts',(4.50498172725087,-2.86839426105774,
-0.614943276887172)) ;
#134467=CARTESIAN_POINT('Ctrl Pts',(4.50826226558342,-2.85869729223562,
-0.702287027113486)) ;
#134468=CARTESIAN_POINT('Ctrl Pts',(4.52028413974051,-2.84160518746962,
-0.832840965432797)) ;
#134469=CARTESIAN_POINT('Ctrl Pts',(4.52545003690602,-2.8354696349403,-0.876363113622023)) ;
#134470=CARTESIAN_POINT('Ctrl Pts',(4.53741870680498,-2.82581179679252,
-0.940639455010752)) ;
#134471=CARTESIAN_POINT('Ctrl Pts',(4.54209540184575,-2.82251395224859,
-0.961920018260584)) ;
#134472=CARTESIAN_POINT('Ctrl Pts',(4.55451190949429,-2.81582803324483,
-1.0038742105328)) ;
#134473=CARTESIAN_POINT('Ctrl Pts',(4.56139306411848,-2.8124020390272,-1.02474353182486)) ;
#134474=CARTESIAN_POINT('Ctrl Pts',(4.57439618084313,-2.80937499999937,
-1.04279586712545)) ;
#134475=CARTESIAN_POINT('Ctrl Pts',(4.57439618084313,-2.80937499999937,
-1.04279586712545)) ;
#134476=CARTESIAN_POINT('Ctrl Pts',(4.57788811720511,-2.80856205104935,
-1.0476438845913)) ;
#134477=CARTESIAN_POINT('Ctrl Pts',(4.58132110715664,-2.80743849592503,
-1.05265431141975)) ;
#134478=CARTESIAN_POINT('Ctrl Pts',(4.58591063786561,-2.80541025280316,
-1.0600683491598)) ;
#134479=CARTESIAN_POINT('Ctrl Pts',(4.587216947305,-2.80476695238162,-1.06226832508373)) ;
#134480=CARTESIAN_POINT('Ctrl Pts',(4.5887449802686,-2.80393035430395,-1.06497171464084)) ;
#134481=CARTESIAN_POINT('Ctrl Pts',(4.58900094431508,-2.8037870887984,-1.06542942337304)) ;
#134482=CARTESIAN_POINT('Ctrl Pts',(4.58924476828968,-2.80364801935069,
-1.06586949326004)) ;
#134483=CARTESIAN_POINT('Ctrl Pts',(4.58924931741448,-2.80364542371033,
-1.0658777053493)) ;
#134484=CARTESIAN_POINT('Ctrl Pts',(4.59158188358133,-2.80231401319274,
-1.07008924012213)) ;
#134485=CARTESIAN_POINT('Ctrl Pts',(4.59377134212491,-2.800813098491,-1.07443839239641)) ;
#134486=CARTESIAN_POINT('Ctrl Pts',(4.59570408210448,-2.79909049146271,
-1.0791378632085)) ;
#134487=CARTESIAN_POINT('Ctrl Pts',(4.59570848738489,-2.79908656285628,
-1.07914857957787)) ;
#134488=CARTESIAN_POINT('Ctrl Pts',(4.59603576097761,-2.79879453264351,
-1.07994507543617)) ;
#134489=CARTESIAN_POINT('Ctrl Pts',(4.59633794834607,-2.79851279959495,
-1.08070652531885)) ;
#134490=CARTESIAN_POINT('Ctrl Pts',(4.59727216584803,-2.79759800070515,
-1.08316063340996)) ;
#134491=CARTESIAN_POINT('Ctrl Pts',(4.59785661125443,-2.79695684051616,
-1.08485291560937)) ;
#134492=CARTESIAN_POINT('Ctrl Pts',(4.59875882816121,-2.7958009226755,-1.08786832422156)) ;
#134493=CARTESIAN_POINT('Ctrl Pts',(4.59910960512328,-2.79529211440565,
-1.08918449921755)) ;
#134494=CARTESIAN_POINT('Ctrl Pts',(4.59950074890552,-2.79458032370896,
-1.09101507841206)) ;
#134495=CARTESIAN_POINT('Ctrl Pts',(4.59959271145697,-2.79439474074568,
-1.09149484058078)) ;
#134496=CARTESIAN_POINT('Ctrl Pts',(4.59970479219924,-2.79411978912796,
-1.09220257104619)) ;
#134497=CARTESIAN_POINT('Ctrl Pts',(4.59973686334512,-2.7940323188425,-1.09242726844519)) ;
#134498=CARTESIAN_POINT('Ctrl Pts',(4.59980956306601,-2.79380428276742,
-1.09301082640206)) ;
#134499=CARTESIAN_POINT('Ctrl Pts',(4.59984405921136,-2.79366555090846,
-1.09336897900421)) ;
#134500=CARTESIAN_POINT('Ctrl Pts',(4.59992170638736,-2.79338632637293,
-1.0940824135446)) ;
#134501=CARTESIAN_POINT('Ctrl Pts',(4.59995882625634,-2.79324305250059,
-1.09443747925646)) ;
#134502=CARTESIAN_POINT('Ctrl Pts',(4.59999999999999,-2.79310344827586,
-1.09479364595777)) ;
#134503=CARTESIAN_POINT('',(4.57439618084271,-2.80937499999947,1.04279586712486)) ;
#134504=CARTESIAN_POINT('Ctrl Pts',(4.59999999999999,-2.79310344827586,
1.09479364595777)) ;
#134505=CARTESIAN_POINT('Ctrl Pts',(4.59995895305209,-2.79324111387631,
1.09443799295581)) ;
#134506=CARTESIAN_POINT('Ctrl Pts',(4.59992125133673,-2.79338175512528,
1.09408335000483)) ;
#134507=CARTESIAN_POINT('Ctrl Pts',(4.59984242179761,-2.79365985893298,
1.09337278174528)) ;
#134508=CARTESIAN_POINT('Ctrl Pts',(4.5998070294299,-2.79379858543765,1.09301809599704)) ;
#134509=CARTESIAN_POINT('Ctrl Pts',(4.59973261548695,-2.79401893257626,
1.09245417872038)) ;
#134510=CARTESIAN_POINT('Ctrl Pts',(4.59970092564442,-2.7941005010842,1.09224529554737)) ;
#134511=CARTESIAN_POINT('Ctrl Pts',(4.59958060815602,-2.79437456977472,
1.09154292574229)) ;
#134512=CARTESIAN_POINT('Ctrl Pts',(4.59947821517875,-2.79456857658396,
1.09104490461926)) ;
#134513=CARTESIAN_POINT('Ctrl Pts',(4.5990597198479,-2.79527981802028,1.08921493561152)) ;
#134514=CARTESIAN_POINT('Ctrl Pts',(4.59869396429225,-2.79579226918928,
1.08788859879992)) ;
#134515=CARTESIAN_POINT('Ctrl Pts',(4.59768320083748,-2.79706868650734,
1.08455592610668)) ;
#134516=CARTESIAN_POINT('Ctrl Pts',(4.59698254015873,-2.79783590182172,
1.08252680033734)) ;
#134517=CARTESIAN_POINT('Ctrl Pts',(4.5959970522588,-2.79876532988112,1.08001531576155)) ;
#134518=CARTESIAN_POINT('Ctrl Pts',(4.59580678362761,-2.79893964110239,
1.07954189499608)) ;
#134519=CARTESIAN_POINT('Ctrl Pts',(4.59367882781299,-2.80083904916685,
1.0743550880029)) ;
#134520=CARTESIAN_POINT('Ctrl Pts',(4.5915070708769,-2.80233337893514,1.07002067229589)) ;
#134521=CARTESIAN_POINT('Ctrl Pts',(4.58628071719234,-2.80532570224271,
1.06054853257076)) ;
#134522=CARTESIAN_POINT('Ctrl Pts',(4.58313959595707,-2.8067311076741,1.05548975193422)) ;
#134523=CARTESIAN_POINT('Ctrl Pts',(4.57802611146331,-2.80844040952816,
1.04790364250821)) ;
#134524=CARTESIAN_POINT('Ctrl Pts',(4.57624387811645,-2.80894486836997,
1.04536104065828)) ;
#134525=CARTESIAN_POINT('Ctrl Pts',(4.57439618084271,-2.80937499999947,
1.04279586712486)) ;
#134526=CARTESIAN_POINT('Ctrl Pts',(4.57439618084271,-2.80937499999947,
1.04279586712486)) ;
#134527=CARTESIAN_POINT('Ctrl Pts',(4.56149777794589,-2.81237766235468,
1.0248889068332)) ;
#134528=CARTESIAN_POINT('Ctrl Pts',(4.55451596106519,-2.81582788236477,
1.00387375770319)) ;
#134529=CARTESIAN_POINT('Ctrl Pts',(4.54213610452188,-2.82249001163036,
0.962071640371718)) ;
#134530=CARTESIAN_POINT('Ctrl Pts',(4.53742891479326,-2.82580422498964,
0.940689032764001)) ;
#134531=CARTESIAN_POINT('Ctrl Pts',(4.525451614243,-2.8354670333868,0.876382056205111)) ;
#134532=CARTESIAN_POINT('Ctrl Pts',(4.52032009146395,-2.84156292603926,
0.833143426521514)) ;
#134533=CARTESIAN_POINT('Ctrl Pts',(4.50830110904356,-2.85862448221642,
0.70288357404262)) ;
#134534=CARTESIAN_POINT('Ctrl Pts',(4.50499166750953,-2.86836219567853,
0.615269961417698)) ;
#134535=CARTESIAN_POINT('Ctrl Pts',(4.49892845988062,-2.8918880660271,0.352237003162138)) ;
#134536=CARTESIAN_POINT('Ctrl Pts',(4.49999999999475,-2.89999999999869,
0.176169909882234)) ;
#134537=CARTESIAN_POINT('Ctrl Pts',(4.5,-2.9,-3.84865454255039E-12)) ;
#134538=CARTESIAN_POINT('Origin',(4.4,-2.7,2.54)) ;
#134539=CARTESIAN_POINT('Origin',(4.4,-2.7,1.52315462117279)) ;
#134540=CARTESIAN_POINT('Ctrl Pts',(4.4022743508907,-2.79999990867355,1.59059930711805)) ;
#134541=CARTESIAN_POINT('Ctrl Pts',(4.51828879250243,-2.80015667527383,
1.58121443320753)) ;
#134542=CARTESIAN_POINT('Ctrl Pts',(4.50118227077258,-2.68533700727764,
1.58202889255053)) ;
#134543=CARTESIAN_POINT('Ctrl Pts',(4.39419482113923,-2.79999992837382,
1.47631230033095)) ;
#134544=CARTESIAN_POINT('Ctrl Pts',(4.48571792501718,-2.80010751836587,
1.49732863324935)) ;
#134545=CARTESIAN_POINT('Ctrl Pts',(4.49717570077253,-2.71006921719245,
1.48296810178551)) ;
#134546=CARTESIAN_POINT('Ctrl Pts',(4.40636790575266,-2.79999994706265,
1.36509109264564)) ;
#134547=CARTESIAN_POINT('Ctrl Pts',(4.47481046024549,-2.80007242131916,
1.38667757220097)) ;
#134548=CARTESIAN_POINT('Ctrl Pts',(4.50328131876403,-2.73353293829091,
1.38297412518993)) ;
#134549=CARTESIAN_POINT('Ctrl Pts',(4.45479736994228,-2.79999997092221,
1.21492633452891)) ;
#134550=CARTESIAN_POINT('Ctrl Pts',(4.49869786247047,-2.80003603117403,
1.23372075650421)) ;
#134551=CARTESIAN_POINT('Ctrl Pts',(4.52748687875416,-2.76348976047506,
1.2437108271413)) ;
#134552=CARTESIAN_POINT('Ctrl Pts',(4.47221929614095,-2.79999997745988,
1.17269593977674)) ;
#134553=CARTESIAN_POINT('Ctrl Pts',(4.50880556767618,-2.8000272573648,1.19172515171411)) ;
#134554=CARTESIAN_POINT('Ctrl Pts',(4.5361913779553,-2.77169834185701,1.20401631763245)) ;
#134555=CARTESIAN_POINT('Ctrl Pts',(4.50882352800135,-2.7999999860536,1.11571565039093)) ;
#134556=CARTESIAN_POINT('Ctrl Pts',(4.53367802911271,-2.80001636071785,
1.13464129757966)) ;
#134557=CARTESIAN_POINT('Ctrl Pts',(4.55447319025664,-2.78248861123825,
1.14990431857449)) ;
#134558=CARTESIAN_POINT('Ctrl Pts',(4.52308919141482,-2.79999998878206,
1.09733743830892)) ;
#134559=CARTESIAN_POINT('Ctrl Pts',(4.54363962638621,-2.80001303821803,
1.11627384982833)) ;
#134560=CARTESIAN_POINT('Ctrl Pts',(4.56159739427507,-2.78591449131412,
1.13234572910531)) ;
#134561=CARTESIAN_POINT('Ctrl Pts',(4.57467506176496,-2.79999999510246,
1.05430349160064)) ;
#134562=CARTESIAN_POINT('Ctrl Pts',(4.58062405303292,-2.80000557393877,
1.07366583672224)) ;
#134563=CARTESIAN_POINT('Ctrl Pts',(4.58735613403295,-2.79385049254303,
1.09108018500675)) ;
#134564=CARTESIAN_POINT('Ctrl Pts',(4.62437069655632,-2.79999999703807,
1.04046865694003)) ;
#134565=CARTESIAN_POINT('Ctrl Pts',(4.61827372661881,-2.80000334969051,
1.05906595451277)) ;
#134566=CARTESIAN_POINT('Ctrl Pts',(4.61212682540736,-2.79628090446616,
1.07759718578196)) ;
#134567=CARTESIAN_POINT('Ctrl Pts',(4.6716136830205,-2.79999998860619,1.09921017323439)) ;
#134568=CARTESIAN_POINT('Ctrl Pts',(4.6540701010266,-2.80001325705937,1.11953626041004)) ;
#134569=CARTESIAN_POINT('Ctrl Pts',(4.63587130780629,-2.78569367459202,
1.13437187040551)) ;
#134570=CARTESIAN_POINT('Ctrl Pts',(4.54879236204369,-2.8,1.0764344436325)) ;
#134571=CARTESIAN_POINT('Ctrl Pts',(4.55448837802386,-2.7999999999815,1.07882117908632)) ;
#134572=CARTESIAN_POINT('Ctrl Pts',(4.56021842726591,-2.7995915078324,1.08116045726579)) ;
#134573=CARTESIAN_POINT('Ctrl Pts',(4.56730671984969,-2.79865167182177,
1.08402111613638)) ;
#134574=CARTESIAN_POINT('Ctrl Pts',(4.56847770958262,-2.79848295770259,
1.08449267316523)) ;
#134575=CARTESIAN_POINT('Ctrl Pts',(4.57107523099021,-2.79808046368154,
1.08553703710302)) ;
#134576=CARTESIAN_POINT('Ctrl Pts',(4.5725009361248,-2.79784058543152,1.08611035697199)) ;
#134577=CARTESIAN_POINT('Ctrl Pts',(4.5764383594612,-2.79713266293194,1.08768631353511)) ;
#134578=CARTESIAN_POINT('Ctrl Pts',(4.57879956048961,-2.79666132938902,
1.08862419960307)) ;
#134579=CARTESIAN_POINT('Ctrl Pts',(4.58293855712952,-2.79579586318667,
1.09023918407038)) ;
#134580=CARTESIAN_POINT('Ctrl Pts',(4.58471363403685,-2.79540911153441,
1.09092538280881)) ;
#134581=CARTESIAN_POINT('Ctrl Pts',(4.58699082729421,-2.7949269768198,1.09175547073797)) ;
#134582=CARTESIAN_POINT('Ctrl Pts',(4.58739952300692,-2.79484234870239,
1.0918980731536)) ;
#134583=CARTESIAN_POINT('Ctrl Pts',(4.58871515235486,-2.79457617288695,
1.09233887089915)) ;
#134584=CARTESIAN_POINT('Ctrl Pts',(4.58961690596143,-2.7944024780556,1.09261501300051)) ;
#134585=CARTESIAN_POINT('Ctrl Pts',(4.59105375065869,-2.79414748185764,
1.09301701818209)) ;
#134586=CARTESIAN_POINT('Ctrl Pts',(4.5915530390955,-2.79406229662442,1.09315075649288)) ;
#134587=CARTESIAN_POINT('Ctrl Pts',(4.5924596538567,-2.79391282221553,1.09338740588514)) ;
#134588=CARTESIAN_POINT('Ctrl Pts',(4.59286388425105,-2.79384761399903,
1.09349157821548)) ;
#134589=CARTESIAN_POINT('Ctrl Pts',(4.59368973959982,-2.79370598615371,
1.09373232734835)) ;
#134590=CARTESIAN_POINT('Ctrl Pts',(4.59407665941124,-2.79363973714591,
1.09384847876684)) ;
#134591=CARTESIAN_POINT('Ctrl Pts',(4.59444371287733,-2.79357284110655,
1.09397320727212)) ;
#134592=CARTESIAN_POINT('Ctrl Pts',(4.5944889025916,-2.79356452972317,1.09398884180049)) ;
#134593=CARTESIAN_POINT('Ctrl Pts',(4.59470842334912,-2.79352377141065,
1.09406617454783)) ;
#134594=CARTESIAN_POINT('Ctrl Pts',(4.59483598733269,-2.79349361011836,
1.09412766851589)) ;
#134595=CARTESIAN_POINT('Ctrl Pts',(4.59514620525223,-2.7934297131363,1.0942540599508)) ;
#134596=CARTESIAN_POINT('Ctrl Pts',(4.59533334275101,-2.79339696908416,
1.0943161621466)) ;
#134597=CARTESIAN_POINT('Ctrl Pts',(4.59563785533348,-2.79335634095568,
1.09438700965973)) ;
#134598=CARTESIAN_POINT('Ctrl Pts',(4.59571710962763,-2.79334654412181,
1.09440360871235)) ;
#134599=CARTESIAN_POINT('Ctrl Pts',(4.59594411915587,-2.79332043135007,
1.0944466503818)) ;
#134600=CARTESIAN_POINT('Ctrl Pts',(4.59600288191153,-2.79330503361987,
1.09446604875921)) ;
#134601=CARTESIAN_POINT('Ctrl Pts',(4.59613307952174,-2.79327450473786,
1.09450071948058)) ;
#134602=CARTESIAN_POINT('Ctrl Pts',(4.59620389659312,-2.79325970788819,
1.09451499394145)) ;
#134603=CARTESIAN_POINT('Ctrl Pts',(4.59651192984771,-2.79322709231927,
1.09454972213713)) ;
#134604=CARTESIAN_POINT('Ctrl Pts',(4.59679543741296,-2.79320989448354,
1.09457065581759)) ;
#134605=CARTESIAN_POINT('Ctrl Pts',(4.59784475938523,-2.793166495242,1.0946421164934)) ;
#134606=CARTESIAN_POINT('Ctrl Pts',(4.59874915064779,-2.79313948637392,
1.09470073568925)) ;
#134607=CARTESIAN_POINT('Ctrl Pts',(4.59999999999999,-2.79310344827586,
1.09479364595777)) ;
#134608=CARTESIAN_POINT('Origin',(4.4,-2.7,2.54)) ;
#134609=CARTESIAN_POINT('Origin',(4.4,-2.7,-3.55684537882721)) ;
#134610=CARTESIAN_POINT('Origin',(4.4,-2.7,-1.52315462117279)) ;
#134611=CARTESIAN_POINT('Ctrl Pts',(4.5011795914298,-2.68531903459927,-1.58202902017228)) ;
#134612=CARTESIAN_POINT('Ctrl Pts',(4.51828670358939,-2.8,-1.58121382514056)) ;
#134613=CARTESIAN_POINT('Ctrl Pts',(4.40240952225579,-2.8,-1.59058837211075)) ;
#134614=CARTESIAN_POINT('Ctrl Pts',(4.49717774927193,-2.71005310920072,
-1.48296553236262)) ;
#134615=CARTESIAN_POINT('Ctrl Pts',(4.48574628541085,-2.8,-1.49731485204045)) ;
#134616=CARTESIAN_POINT('Ctrl Pts',(4.39431668173578,-2.8,-1.47634026950832)) ;
#134617=CARTESIAN_POINT('Ctrl Pts',(4.50328690685191,-2.73351987602563,
-1.38297339786192)) ;
#134618=CARTESIAN_POINT('Ctrl Pts',(4.47485145549547,-2.8,-1.3866766957413)) ;
#134619=CARTESIAN_POINT('Ctrl Pts',(4.40646789472124,-2.8,-1.36512261863837)) ;
#134620=CARTESIAN_POINT('Ctrl Pts',(4.5274931179709,-2.76348183928882,-1.2437129921595)) ;
#134621=CARTESIAN_POINT('Ctrl Pts',(4.49873206155793,-2.8,-1.233733095307)) ;
#134622=CARTESIAN_POINT('Ctrl Pts',(4.4548681704377,-2.8,-1.21495664336612)) ;
#134623=CARTESIAN_POINT('Ctrl Pts',(4.53619745972498,-2.77169205010107,
-1.20401904718522)) ;
#134624=CARTESIAN_POINT('Ctrl Pts',(4.50883664816668,-2.8,-1.19173943817213)) ;
#134625=CARTESIAN_POINT('Ctrl Pts',(4.47227975612149,-2.8,-1.17272738460373)) ;
#134626=CARTESIAN_POINT('Ctrl Pts',(4.55447795090009,-2.7824845983034,-1.14990781273337)) ;
#134627=CARTESIAN_POINT('Ctrl Pts',(4.53370055749885,-2.8,-1.13465791836995)) ;
#134628=CARTESIAN_POINT('Ctrl Pts',(4.50886586566853,-2.8,-1.11574788827223)) ;
#134629=CARTESIAN_POINT('Ctrl Pts',(4.56160154376424,-2.78591123334062,
-1.13234944281567)) ;
#134630=CARTESIAN_POINT('Ctrl Pts',(4.54365878772217,-2.8,-1.11629106645424)) ;
#134631=CARTESIAN_POINT('Ctrl Pts',(4.52312452397684,-2.8,-1.09736999548674)) ;
#134632=CARTESIAN_POINT('Ctrl Pts',(4.58735772267364,-2.79384903998488,
-1.09108429439848)) ;
#134633=CARTESIAN_POINT('Ctrl Pts',(4.58063087367388,-2.8,-1.07368396338091)) ;
#134634=CARTESIAN_POINT('Ctrl Pts',(4.57468550767192,-2.8,-1.05433748660568)) ;
#134635=CARTESIAN_POINT('Ctrl Pts',(4.61212536563475,-2.79628002040279,
-1.07760158659545)) ;
#134636=CARTESIAN_POINT('Ctrl Pts',(4.61826745782982,-2.8,-1.05908487937578)) ;
#134637=CARTESIAN_POINT('Ctrl Pts',(4.62435992349564,-2.8,-1.04050151732138)) ;
#134638=CARTESIAN_POINT('Ctrl Pts',(4.63586710715936,-2.78569036914655,
-1.13437529467537)) ;
#134639=CARTESIAN_POINT('Ctrl Pts',(4.65405106945745,-2.8,-1.11955252388339)) ;
#134640=CARTESIAN_POINT('Ctrl Pts',(4.67158355065754,-2.8,-1.09924507978095)) ;
#134641=CARTESIAN_POINT('Ctrl Pts',(4.59999999999999,-2.79310344827586,
-1.09479364595777)) ;
#134642=CARTESIAN_POINT('Ctrl Pts',(4.59840954578196,-2.79314968944989,
-1.09467567269119)) ;
#134643=CARTESIAN_POINT('Ctrl Pts',(4.59737383489065,-2.79318159606221,
-1.09461332397165)) ;
#134644=CARTESIAN_POINT('Ctrl Pts',(4.59650507521634,-2.79322931786013,
-1.09455037725996)) ;
#134645=CARTESIAN_POINT('Ctrl Pts',(4.59632758424293,-2.79324472590583,
-1.09453457917666)) ;
#134646=CARTESIAN_POINT('Ctrl Pts',(4.5961184721084,-2.79327477162037,-1.09450475657722)) ;
#134647=CARTESIAN_POINT('Ctrl Pts',(4.59606489504922,-2.79328892979787,
-1.09449102658529)) ;
#134648=CARTESIAN_POINT('Ctrl Pts',(4.5959460167769,-2.79331605564258,-1.09445911449494)) ;
#134649=CARTESIAN_POINT('Ctrl Pts',(4.59588597444854,-2.7933285533825,-1.09444265618345)) ;
#134650=CARTESIAN_POINT('Ctrl Pts',(4.59549967474363,-2.79337285752324,
-1.09437027876054)) ;
#134651=CARTESIAN_POINT('Ctrl Pts',(4.59527331486237,-2.79340622385959,
-1.09431008070831)) ;
#134652=CARTESIAN_POINT('Ctrl Pts',(4.5949320123953,-2.79346950514991,-1.09418704029369)) ;
#134653=CARTESIAN_POINT('Ctrl Pts',(4.59480393230129,-2.79349821606422,
-1.09412847427896)) ;
#134654=CARTESIAN_POINT('Ctrl Pts',(4.59460326813595,-2.79353924388982,
-1.09404763514903)) ;
#134655=CARTESIAN_POINT('Ctrl Pts',(4.59455075953096,-2.7935496343265,-1.09402742767144)) ;
#134656=CARTESIAN_POINT('Ctrl Pts',(4.59417008680874,-2.79361944405451,
-1.09389559371761)) ;
#134657=CARTESIAN_POINT('Ctrl Pts',(4.5937774209655,-2.79368602572532,-1.09377734615547)) ;
#134658=CARTESIAN_POINT('Ctrl Pts',(4.59289939109636,-2.7938335466559,-1.09352541902408)) ;
#134659=CARTESIAN_POINT('Ctrl Pts',(4.59245006584788,-2.79390305456782,
-1.09341603619896)) ;
#134660=CARTESIAN_POINT('Ctrl Pts',(4.5909955251919,-2.79413629528614,-1.09305685240916)) ;
#134661=CARTESIAN_POINT('Ctrl Pts',(4.59002197881477,-2.79430302757335,
-1.0928063701757)) ;
#134662=CARTESIAN_POINT('Ctrl Pts',(4.58861122644569,-2.79456793455722,
-1.0923921365665)) ;
#134663=CARTESIAN_POINT('Ctrl Pts',(4.58817904894343,-2.79465210327465,
-1.09225852343037)) ;
#134664=CARTESIAN_POINT('Ctrl Pts',(4.58736872283364,-2.79481449815582,
-1.09199418358962)) ;
#134665=CARTESIAN_POINT('Ctrl Pts',(4.58699491219414,-2.79489135860975,
-1.09186658235812)) ;
#134666=CARTESIAN_POINT('Ctrl Pts',(4.58468897497186,-2.79537899446709,
-1.09103519061959)) ;
#134667=CARTESIAN_POINT('Ctrl Pts',(4.58290717718701,-2.79577019617637,
-1.09034206422841)) ;
#134668=CARTESIAN_POINT('Ctrl Pts',(4.57867627871777,-2.79666451416568,
-1.08867078828749)) ;
#134669=CARTESIAN_POINT('Ctrl Pts',(4.57626321554132,-2.79715040843618,
-1.08768776514286)) ;
#134670=CARTESIAN_POINT('Ctrl Pts',(4.57243386308706,-2.79784156172336,
-1.0861367865103)) ;
#134671=CARTESIAN_POINT('Ctrl Pts',(4.57107519984215,-2.79807176647234,
-1.08558402144498)) ;
#134672=CARTESIAN_POINT('Ctrl Pts',(4.56513452430488,-2.79900074294388,
-1.0831693903581)) ;
#134673=CARTESIAN_POINT('Ctrl Pts',(4.56062162665772,-2.79951267011375,
-1.08133092934958)) ;
#134674=CARTESIAN_POINT('Ctrl Pts',(4.55365420596664,-2.79992470862866,
-1.07846103027848)) ;
#134675=CARTESIAN_POINT('Ctrl Pts',(4.55124660967283,-2.79999983267432,
-1.07746323925077)) ;
#134676=CARTESIAN_POINT('Ctrl Pts',(4.54880051362943,-2.79999999972164,
-1.07643786073294)) ;
#134677=CARTESIAN_POINT('Ctrl Pts',(4.54879236166275,-2.8,1.07643444348484)) ;
#134678=CARTESIAN_POINT('Ctrl Pts',(4.5622387183224,-2.79999999999679,1.05876847372513)) ;
#134679=CARTESIAN_POINT('Ctrl Pts',(4.57442182196495,-2.80939476060286,
1.0427621795332)) ;
#134680=CARTESIAN_POINT('Ctrl Pts',(4.55556842517599,-2.79999999999889,
1.07927493595118)) ;
#134681=CARTESIAN_POINT('Ctrl Pts',(4.56783337210914,-2.80040661803735,
1.06381369844813)) ;
#134682=CARTESIAN_POINT('Ctrl Pts',(4.57961823522366,-2.80818164104597,
1.04998165867271)) ;
#134683=CARTESIAN_POINT('Ctrl Pts',(4.56238982831618,-2.79942602551759,
1.08204714848293)) ;
#134684=CARTESIAN_POINT('Ctrl Pts',(4.57357810388181,-2.80014618986472,
1.06906892785879)) ;
#134685=CARTESIAN_POINT('Ctrl Pts',(4.58462643299473,-2.80630261261111,
1.05747672883513)) ;
#134686=CARTESIAN_POINT('Ctrl Pts',(4.57328757735259,-2.7977370397245,1.08643000204986)) ;
#134687=CARTESIAN_POINT('Ctrl Pts',(4.58237922839515,-2.79856394574987,
1.07773359106864)) ;
#134688=CARTESIAN_POINT('Ctrl Pts',(4.59151541127592,-2.80237286596198,
1.06991699711942)) ;
#134689=CARTESIAN_POINT('Ctrl Pts',(4.57700059755676,-2.79703714667161,
1.08792392365797)) ;
#134690=CARTESIAN_POINT('Ctrl Pts',(4.58532305318676,-2.79784352093717,
1.08073745699554)) ;
#134691=CARTESIAN_POINT('Ctrl Pts',(4.59370961102545,-2.80088045369937,
1.07425448581055)) ;
#134692=CARTESIAN_POINT('Ctrl Pts',(4.58319893207065,-2.79574016930783,
1.09034532947887)) ;
#134693=CARTESIAN_POINT('Ctrl Pts',(4.58990416109239,-2.79637293360539,
1.08566964543776)) ;
#134694=CARTESIAN_POINT('Ctrl Pts',(4.59665800356694,-2.79825577077759,
1.08141805513029)) ;
#134695=CARTESIAN_POINT('Ctrl Pts',(4.58534994317985,-2.79526732601294,
1.09118113811282)) ;
#134696=CARTESIAN_POINT('Ctrl Pts',(4.59144552977842,-2.79581844972912,
1.08737996338929)) ;
#134697=CARTESIAN_POINT('Ctrl Pts',(4.59758018705035,-2.79731769672696,
1.08391141960612)) ;
#134698=CARTESIAN_POINT('Ctrl Pts',(4.58899927751307,-2.79450268149332,
1.09248269873289)) ;
#134699=CARTESIAN_POINT('Ctrl Pts',(4.59386223202755,-2.79488630507105,
1.09005048296971)) ;
#134700=CARTESIAN_POINT('Ctrl Pts',(4.59874684688641,-2.79582009356912,
1.08781863475525)) ;
#134701=CARTESIAN_POINT('Ctrl Pts',(4.59026755692873,-2.79423885380164,
1.09292560041996)) ;
#134702=CARTESIAN_POINT('Ctrl Pts',(4.59467706068313,-2.79455862385203,
1.09095945666394)) ;
#134703=CARTESIAN_POINT('Ctrl Pts',(4.59910266898803,-2.79530499526365,
1.08915136009784)) ;
#134704=CARTESIAN_POINT('Ctrl Pts',(4.59257623319514,-2.79382131826659,
1.09361586855001)) ;
#134705=CARTESIAN_POINT('Ctrl Pts',(4.59605751036345,-2.79403163929514,
1.09237723896638)) ;
#134706=CARTESIAN_POINT('Ctrl Pts',(4.59954701072604,-2.79449510806573,
1.09123423318303)) ;
#134707=CARTESIAN_POINT('Ctrl Pts',(4.59342976933297,-2.79367543507711,
1.09385546254663)) ;
#134708=CARTESIAN_POINT('Ctrl Pts',(4.59655016100493,-2.79384713427255,
1.09286511046971)) ;
#134709=CARTESIAN_POINT('Ctrl Pts',(4.59967640178298,-2.79421605292372,
1.09194978606297)) ;
#134710=CARTESIAN_POINT('Ctrl Pts',(4.59428414179642,-2.79346156087783,
1.09429306381474)) ;
#134711=CARTESIAN_POINT('Ctrl Pts',(4.59704519451433,-2.79355469746529,
1.09362636425205)) ;
#134712=CARTESIAN_POINT('Ctrl Pts',(4.5998104157401,-2.79379877456676,1.09301762872931)) ;
#134713=CARTESIAN_POINT('Ctrl Pts',(4.59432658472652,-2.7933916625364,1.09446618185051)) ;
#134714=CARTESIAN_POINT('Ctrl Pts',(4.59708408719785,-2.79345234504013,
1.09389092335371)) ;
#134715=CARTESIAN_POINT('Ctrl Pts',(4.59984563524626,-2.79366003518351,
1.09337234564734)) ;
#134716=CARTESIAN_POINT('Ctrl Pts',(4.59537197237733,-2.79324260992761,
1.09471273840615)) ;
#134717=CARTESIAN_POINT('Ctrl Pts',(4.59764722167537,-2.79326383513928,
1.094379038145)) ;
#134718=CARTESIAN_POINT('Ctrl Pts',(4.59992475053754,-2.79338190759658,
1.09408296935242)) ;
#134719=CARTESIAN_POINT('Ctrl Pts',(4.5936418339237,-2.79313407032025,1.09471552115488)) ;
#134720=CARTESIAN_POINT('Ctrl Pts',(4.59684754854893,-2.79327107597597,
1.09436106895479)) ;
#134721=CARTESIAN_POINT('Ctrl Pts',(4.59996664298755,-2.79324102308607,
1.09443822631848)) ;
#134722=CARTESIAN_POINT('Ctrl Pts',(4.59999999999999,-2.79310344827586,
1.09479364595777)) ;
#134723=CARTESIAN_POINT('Ctrl Pts',(4.59999999999999,-2.79310344827586,
1.09479364595777)) ;
#134724=CARTESIAN_POINT('Ctrl Pts',(4.59999999999999,-2.79310344827586,
1.09479364595777)) ;
#134725=CARTESIAN_POINT('Origin',(4.54879236168542,-2.9,1.07643444348393)) ;
#134726=CARTESIAN_POINT('Ctrl Pts',(4.39959973407451,-2.8,-0.110592242802564)) ;
#134727=CARTESIAN_POINT('Ctrl Pts',(4.49922290141881,-2.8,-0.110105248331461)) ;
#134728=CARTESIAN_POINT('Ctrl Pts',(4.49980764094185,-2.89969504276377,
-0.11060804589506)) ;
#134729=CARTESIAN_POINT('Ctrl Pts',(4.40142712570759,-2.8,0.110466103992318)) ;
#134730=CARTESIAN_POINT('Ctrl Pts',(4.5059362211965,-2.8,0.113951986531775)) ;
#134731=CARTESIAN_POINT('Ctrl Pts',(4.50067611734352,-2.90411960318539,
0.110349712874591)) ;
#134732=CARTESIAN_POINT('Ctrl Pts',(4.39573539165433,-2.8,0.332377458211494)) ;
#134733=CARTESIAN_POINT('Ctrl Pts',(4.49039105203445,-2.8,0.313555133991133)) ;
#134734=CARTESIAN_POINT('Ctrl Pts',(4.49793210898571,-2.89506044297344,
0.333407164930358)) ;
#134735=CARTESIAN_POINT('Ctrl Pts',(4.41164816536272,-2.8,0.645507851343547)) ;
#134736=CARTESIAN_POINT('Ctrl Pts',(4.48203507549535,-2.8,0.636992461610863)) ;
#134737=CARTESIAN_POINT('Ctrl Pts',(4.50604587949363,-2.86657833599731,
0.638208366544944)) ;
#134738=CARTESIAN_POINT('Ctrl Pts',(4.41940490599909,-2.8,0.737842868001297)) ;
#134739=CARTESIAN_POINT('Ctrl Pts',(4.48133975791567,-2.8,0.726672536261365)) ;
#134740=CARTESIAN_POINT('Ctrl Pts',(4.50997623336226,-2.85625883833133,
0.726935356761025)) ;
#134741=CARTESIAN_POINT('Ctrl Pts',(4.44577434373642,-2.8,0.872979341174024)) ;
#134742=CARTESIAN_POINT('Ctrl Pts',(4.49360122670478,-2.8,0.860669412332162)) ;
#134743=CARTESIAN_POINT('Ctrl Pts',(4.52318558604183,-2.83896465559564,
0.854514957562391)) ;
#134744=CARTESIAN_POINT('Ctrl Pts',(4.45692583760035,-2.8,0.917523106947224)) ;
#134745=CARTESIAN_POINT('Ctrl Pts',(4.49949391572667,-2.8,0.90394569735387)) ;
#134746=CARTESIAN_POINT('Ctrl Pts',(4.52876348458384,-2.83289258157629,
0.896197011395723)) ;
#134747=CARTESIAN_POINT('Ctrl Pts',(4.50378503771653,-2.8,1.03892408374168)) ;
#134748=CARTESIAN_POINT('Ctrl Pts',(4.52873519606807,-2.8,1.02007465772522)) ;
#134749=CARTESIAN_POINT('Ctrl Pts',(4.55214466721901,-2.81552005845342,
1.00877513019841)) ;
#134750=CARTESIAN_POINT('Ctrl Pts',(4.5471442379017,-2.8,1.11773150495339)) ;
#134751=CARTESIAN_POINT('Ctrl Pts',(4.55761617337306,-2.8,1.09679343581194)) ;
#134752=CARTESIAN_POINT('Ctrl Pts',(4.57259584813394,-2.80338245043794,
1.07876140481136)) ;
#134753=CARTESIAN_POINT('Ctrl Pts',(4.67762904165636,-2.8,1.10850495520363)) ;
#134754=CARTESIAN_POINT('Ctrl Pts',(4.66093484724981,-2.8,1.09293293416154)) ;
#134755=CARTESIAN_POINT('Ctrl Pts',(4.64133868807436,-2.80368623369345,
1.07531199361316)) ;
#134756=CARTESIAN_POINT('Origin',(4.4,-2.9,-3.84865454255039E-12)) ;
#134757=CARTESIAN_POINT('Ctrl Pts',(4.7217278356704,-2.8000000024879,-1.10036295491226)) ;
#134758=CARTESIAN_POINT('Ctrl Pts',(4.69645430308005,-2.79999660525785,
-1.08707004730944)) ;
#134759=CARTESIAN_POINT('Ctrl Pts',(4.66463283185041,-2.80454824226961,
-1.06949036829269)) ;
#134760=CARTESIAN_POINT('Ctrl Pts',(4.55709227475145,-2.80000000030525,
-1.13599643631035)) ;
#134761=CARTESIAN_POINT('Ctrl Pts',(4.56399237478695,-2.79999958643658,
-1.1139593792008)) ;
#134762=CARTESIAN_POINT('Ctrl Pts',(4.57729370999483,-2.80055804294513,
-1.09517590508062)) ;
#134763=CARTESIAN_POINT('Ctrl Pts',(4.50667826286324,-2.80000000784871,
-1.04661464799811)) ;
#134764=CARTESIAN_POINT('Ctrl Pts',(4.53037382014986,-2.79998899178918,
-1.02708460011663)) ;
#134765=CARTESIAN_POINT('Ctrl Pts',(4.55348183854655,-2.814346995092,-1.01594660411382)) ;
#134766=CARTESIAN_POINT('Ctrl Pts',(4.45692280158728,-2.80000001789831,
-0.917642218287593)) ;
#134767=CARTESIAN_POINT('Ctrl Pts',(4.49938029267387,-2.79997354447567,
-0.904099888009291)) ;
#134768=CARTESIAN_POINT('Ctrl Pts',(4.5286414976122,-2.83271033979029,-0.896329062079886)) ;
#134769=CARTESIAN_POINT('Ctrl Pts',(4.44554661086167,-2.80000002126189,
-0.872377440013972)) ;
#134770=CARTESIAN_POINT('Ctrl Pts',(4.49333665154873,-2.79996797963652,
-0.86009693987387)) ;
#134771=CARTESIAN_POINT('Ctrl Pts',(4.52295544156375,-2.83885474437148,
-0.853967858227963)) ;
#134772=CARTESIAN_POINT('Ctrl Pts',(4.41903322104342,-2.8000000307772,-0.735894797577176)) ;
#134773=CARTESIAN_POINT('Ctrl Pts',(4.48100616080269,-2.79995095769185,
-0.724730004020391)) ;
#134774=CARTESIAN_POINT('Ctrl Pts',(4.50969337368917,-2.85623179093908,
-0.725069623608933)) ;
#134775=CARTESIAN_POINT('Ctrl Pts',(4.41147189908676,-2.8000000363501,-0.64424159004353)) ;
#134776=CARTESIAN_POINT('Ctrl Pts',(4.48178828424082,-2.79993989905032,
-0.635789149205618)) ;
#134777=CARTESIAN_POINT('Ctrl Pts',(4.50589025525755,-2.86640526991179,
-0.636968151201155)) ;
#134778=CARTESIAN_POINT('Ctrl Pts',(4.39523119070925,-2.80000005228414,
-0.32317951983275)) ;
#134779=CARTESIAN_POINT('Ctrl Pts',(4.49033836345961,-2.79990261688309,
-0.303074131660309)) ;
#134780=CARTESIAN_POINT('Ctrl Pts',(4.49769757367181,-2.89547737953052,
-0.32433321576161)) ;
#134781=CARTESIAN_POINT('Ctrl Pts',(4.40178225889358,-2.80000005718968,
-0.092623978285313)) ;
#134782=CARTESIAN_POINT('Ctrl Pts',(4.50681341018239,-2.7998878412185,-0.0970581988245104)) ;
#134783=CARTESIAN_POINT('Ctrl Pts',(4.50092255053472,-2.90441958896148,
-0.0924406960392595)) ;
#134784=CARTESIAN_POINT('Ctrl Pts',(4.39924589760313,-2.80000005405718,
0.13696883112012)) ;
#134785=CARTESIAN_POINT('Ctrl Pts',(4.49795607191458,-2.79989746608223,
0.136077062504044)) ;
#134786=CARTESIAN_POINT('Ctrl Pts',(4.49968270404899,-2.89870974459617,
0.136971505408573)) ;
#134787=CARTESIAN_POINT('Origin',(4.54879236168626,-2.9,-1.07643444348457)) ;
#134788=CARTESIAN_POINT('Ctrl Pts',(4.57442492185552,-2.80939715119899,
-1.04275810686208)) ;
#134789=CARTESIAN_POINT('Ctrl Pts',(4.56210583156796,-2.79989612750329,
-1.05894306178873)) ;
#134790=CARTESIAN_POINT('Ctrl Pts',(4.54850917782856,-2.80000109307748,
-1.07680649348805)) ;
#134791=CARTESIAN_POINT('Ctrl Pts',(4.57959763980855,-2.80818914940071,
-1.04994530049547)) ;
#134792=CARTESIAN_POINT('Ctrl Pts',(4.56768008075467,-2.80031924975226,
-1.06394104572908)) ;
#134793=CARTESIAN_POINT('Ctrl Pts',(4.55527876038346,-2.79999229227378,
-1.07958997638678)) ;
#134794=CARTESIAN_POINT('Ctrl Pts',(4.58464248447265,-2.80630474344638,
-1.05748431263834)) ;
#134795=CARTESIAN_POINT('Ctrl Pts',(4.57346944634372,-2.80008318972135,
-1.06920129105218)) ;
#134796=CARTESIAN_POINT('Ctrl Pts',(4.56216307187795,-2.79941338753917,
-1.08232809153345)) ;
#134797=CARTESIAN_POINT('Ctrl Pts',(4.59159231899494,-2.80232720646228,
-1.07005636929591)) ;
#134798=CARTESIAN_POINT('Ctrl Pts',(4.58237910662986,-2.79850221241048,
-1.07791493625778)) ;
#134799=CARTESIAN_POINT('Ctrl Pts',(4.57321634584967,-2.79769868647539,
-1.08666448649469)) ;
#134800=CARTESIAN_POINT('Ctrl Pts',(4.59378564167737,-2.8008235544484,-1.07441458376545)) ;
#134801=CARTESIAN_POINT('Ctrl Pts',(4.58533966160572,-2.79778056279966,
-1.08091806944782)) ;
#134802=CARTESIAN_POINT('Ctrl Pts',(4.5769613009382,-2.79699227428059,-1.08813207403617)) ;
#134803=CARTESIAN_POINT('Ctrl Pts',(4.59669734138576,-2.79821861236081,
-1.08151744690911)) ;
#134804=CARTESIAN_POINT('Ctrl Pts',(4.58989502505307,-2.7963307230051,-1.08578370298498)) ;
#134805=CARTESIAN_POINT('Ctrl Pts',(4.58314295739387,-2.79570785369251,
-1.09047890318143)) ;
#134806=CARTESIAN_POINT('Ctrl Pts',(4.59760632414569,-2.79728965034655,
-1.08398524662906)) ;
#134807=CARTESIAN_POINT('Ctrl Pts',(4.59142619397024,-2.79578507327359,
-1.08746789372294)) ;
#134808=CARTESIAN_POINT('Ctrl Pts',(4.58528630332434,-2.79524119148169,
-1.09128737837496)) ;
#134809=CARTESIAN_POINT('Ctrl Pts',(4.59875741430932,-2.79580683383092,
-1.08785300449597)) ;
#134810=CARTESIAN_POINT('Ctrl Pts',(4.59383193680337,-2.79486773439436,
-1.09009800553385)) ;
#134811=CARTESIAN_POINT('Ctrl Pts',(4.58892874314202,-2.79448758877844,
-1.09254647301294)) ;
#134812=CARTESIAN_POINT('Ctrl Pts',(4.59910834609947,-2.79529718130591,
-1.08917149930144)) ;
#134813=CARTESIAN_POINT('Ctrl Pts',(4.59464343907623,-2.79454543406796,
-1.09099269585011)) ;
#134814=CARTESIAN_POINT('Ctrl Pts',(4.59019511689903,-2.79422790851556,
-1.09297467120907)) ;
#134815=CARTESIAN_POINT('Ctrl Pts',(4.59954688679867,-2.79449699552073,
-1.0912293846587)) ;
#134816=CARTESIAN_POINT('Ctrl Pts',(4.59601732089136,-2.79402779797775,
-1.09238633635182)) ;
#134817=CARTESIAN_POINT('Ctrl Pts',(4.59249627585272,-2.79381771894921,
-1.09364111416748)) ;
#134818=CARTESIAN_POINT('Ctrl Pts',(4.59967529310588,-2.79422450025963,
-1.09193546456122)) ;
#134819=CARTESIAN_POINT('Ctrl Pts',(4.59651100242293,-2.79384821317134,
-1.09286441087348)) ;
#134820=CARTESIAN_POINT('Ctrl Pts',(4.59335287412398,-2.79367727499394,
-1.09387144765738)) ;
#134821=CARTESIAN_POINT('Ctrl Pts',(4.59980981518572,-2.79380630943631,
-1.09300564521014)) ;
#134822=CARTESIAN_POINT('Ctrl Pts',(4.59701056623719,-2.79355888022806,
-1.09362493503647)) ;
#134823=CARTESIAN_POINT('Ctrl Pts',(4.59421559911327,-2.79346462438276,
-1.09430302898986)) ;
#134824=CARTESIAN_POINT('Ctrl Pts',(4.59984534134842,-2.79366726490194,
-1.09336460674889)) ;
#134825=CARTESIAN_POINT('Ctrl Pts',(4.59705039509826,-2.79345667046143,
-1.09389173939615)) ;
#134826=CARTESIAN_POINT('Ctrl Pts',(4.59425962044003,-2.79339574833516,
-1.09447656370425)) ;
#134827=CARTESIAN_POINT('Ctrl Pts',(4.59992484646001,-2.7933873519883,-1.09407980383996)) ;
#134828=CARTESIAN_POINT('Ctrl Pts',(4.59761652863209,-2.7932668237374,-1.09438058953102)) ;
#134829=CARTESIAN_POINT('Ctrl Pts',(4.59531061070856,-2.79324678512396,
-1.09472041373345)) ;
#134830=CARTESIAN_POINT('Ctrl Pts',(4.59996721368508,-2.79324340897637,
-1.09443656979399)) ;
#134831=CARTESIAN_POINT('Ctrl Pts',(4.59680854952868,-2.79327323421043,
-1.09436047786159)) ;
#134832=CARTESIAN_POINT('Ctrl Pts',(4.59356174266139,-2.79313094944462,
-1.09472348332067)) ;
#134833=CARTESIAN_POINT('Ctrl Pts',(4.59999999999999,-2.79310344827586,
-1.09479364595777)) ;
#134834=CARTESIAN_POINT('Ctrl Pts',(4.59999999999999,-2.79310344827586,
-1.09479364595777)) ;
#134835=CARTESIAN_POINT('Ctrl Pts',(4.59999999999999,-2.79310344827586,
-1.09479364595777)) ;
#134836=CARTESIAN_POINT('Origin',(5.6561028345357,10.05,2.04)) ;
#134837=CARTESIAN_POINT('Origin',(7.26810489940853,5.50476046277485,-2.875)) ;
#134838=CARTESIAN_POINT('',(4.03523814377473,5.98727788898885,-2.775)) ;
#134839=CARTESIAN_POINT('',(4.03523814377473,5.98727788898885,-1.475)) ;
#134840=CARTESIAN_POINT('',(4.03523814377473,5.98727788898885,-2.875)) ;
#134841=CARTESIAN_POINT('',(7.26810489940853,5.50476046277485,-1.475)) ;
#134842=CARTESIAN_POINT('',(7.26810489940853,5.50476046277485,-1.475)) ;
#134843=CARTESIAN_POINT('',(7.26810489940853,5.50476046277485,-2.775)) ;
#134844=CARTESIAN_POINT('',(7.26810489940853,5.50476046277485,-2.875)) ;
#134845=CARTESIAN_POINT('',(3.95,6.,-2.775)) ;
#134846=CARTESIAN_POINT('Origin',(7.25334304318326,5.40585602606554,-2.875)) ;
#134847=CARTESIAN_POINT('',(7.32310496992715,5.47750289324744,-1.475)) ;
#134848=CARTESIAN_POINT('Origin',(7.25334304318326,5.40585602606554,-1.475)) ;
#134849=CARTESIAN_POINT('',(7.32310496992715,5.47750289324744,-2.775)) ;
#134850=CARTESIAN_POINT('',(7.32310496992715,5.47750289324744,-2.875)) ;
#134851=CARTESIAN_POINT('Origin',(7.25334304318326,5.40585602606554,-2.775)) ;
#134852=CARTESIAN_POINT('Origin',(8.66976192674389,4.16627481495487,-2.875)) ;
#134853=CARTESIAN_POINT('',(8.66976192674389,4.16627481495487,-1.475)) ;
#134854=CARTESIAN_POINT('',(8.66976192674389,4.16627481495487,-1.475)) ;
#134855=CARTESIAN_POINT('',(8.66976192674389,4.16627481495487,-2.775)) ;
#134856=CARTESIAN_POINT('',(8.66976192674389,4.16627481495487,-2.875)) ;
#134857=CARTESIAN_POINT('',(7.32310496992715,5.47750289324744,-2.775)) ;
#134858=CARTESIAN_POINT('Origin',(8.6,4.09462794777298,-2.875)) ;
#134859=CARTESIAN_POINT('',(8.7,4.09462794777298,-1.475)) ;
#134860=CARTESIAN_POINT('Origin',(8.6,4.09462794777298,-1.475)) ;
#134861=CARTESIAN_POINT('',(8.7,4.09462794777298,-2.775)) ;
#134862=CARTESIAN_POINT('',(8.7,4.09462794777298,-2.875)) ;
#134863=CARTESIAN_POINT('Origin',(8.6,4.09462794777298,-2.775)) ;
#134864=CARTESIAN_POINT('Origin',(8.7,3.95,-2.875)) ;
#134865=CARTESIAN_POINT('',(8.7,3.95,-1.475)) ;
#134866=CARTESIAN_POINT('',(8.7,3.95,-1.475)) ;
#134867=CARTESIAN_POINT('',(8.7,3.95,-2.775)) ;
#134868=CARTESIAN_POINT('',(8.7,3.95,-2.875)) ;
#134869=CARTESIAN_POINT('',(8.7,4.09462794777298,-2.775)) ;
#134870=CARTESIAN_POINT('Origin',(8.6,3.95,-2.875)) ;
#134871=CARTESIAN_POINT('',(8.55460943381591,3.86089502538305,-1.475)) ;
#134872=CARTESIAN_POINT('Origin',(8.6,3.95,-1.475)) ;
#134873=CARTESIAN_POINT('',(8.55460943381591,3.86089502538305,-2.775)) ;
#134874=CARTESIAN_POINT('',(8.55460943381591,3.86089502538305,-2.875)) ;
#134875=CARTESIAN_POINT('Origin',(8.6,3.95,-2.775)) ;
#134876=CARTESIAN_POINT('Origin',(7.3213877252879,4.48910497461695,-2.875)) ;
#134877=CARTESIAN_POINT('',(7.3213877252879,4.48910497461695,-1.475)) ;
#134878=CARTESIAN_POINT('',(7.3213877252879,4.48910497461695,-1.475)) ;
#134879=CARTESIAN_POINT('',(7.3213877252879,4.48910497461695,-2.775)) ;
#134880=CARTESIAN_POINT('',(7.3213877252879,4.48910497461695,-2.875)) ;
#134881=CARTESIAN_POINT('',(8.55460943381591,3.86089502538305,-2.775)) ;
#134882=CARTESIAN_POINT('Origin',(7.27599715910381,4.4,-2.875)) ;
#134883=CARTESIAN_POINT('',(7.27599715910381,4.5,-1.475)) ;
#134884=CARTESIAN_POINT('Origin',(7.27599715910381,4.4,-1.475)) ;
#134885=CARTESIAN_POINT('',(7.27599715910381,4.5,-2.775)) ;
#134886=CARTESIAN_POINT('',(7.27599715910381,4.5,-2.875)) ;
#134887=CARTESIAN_POINT('Origin',(7.27599715910381,4.4,-2.775)) ;
#134888=CARTESIAN_POINT('Origin',(3.95,4.5,-2.875)) ;
#134889=CARTESIAN_POINT('',(4.05,4.5,-1.475)) ;
#134890=CARTESIAN_POINT('',(3.95,4.5,-1.475)) ;
#134891=CARTESIAN_POINT('',(4.05,4.5,-2.775)) ;
#134892=CARTESIAN_POINT('',(4.05,4.5,-2.875)) ;
#134893=CARTESIAN_POINT('',(7.27599715910381,4.5,-2.775)) ;
#134894=CARTESIAN_POINT('Origin',(7.25334304318326,5.40585602606554,-2.875)) ;
#134895=CARTESIAN_POINT('',(7.36677829147199,4.5782099492339,-2.875)) ;
#134896=CARTESIAN_POINT('',(7.27599715910381,4.6,-2.875)) ;
#134897=CARTESIAN_POINT('Origin',(7.27599715910381,4.4,-2.875)) ;
#134898=CARTESIAN_POINT('',(4.05,4.6,-2.875)) ;
#134899=CARTESIAN_POINT('',(3.95,4.6,-2.875)) ;
#134900=CARTESIAN_POINT('',(4.05,5.88396692803319,-2.875)) ;
#134901=CARTESIAN_POINT('',(4.05,6.,-2.875)) ;
#134902=CARTESIAN_POINT('',(7.25334304318326,5.40585602606554,-2.875)) ;
#134903=CARTESIAN_POINT('',(7.25334304318326,5.40585602606554,-2.875)) ;
#134904=CARTESIAN_POINT('',(8.6,4.09462794777298,-2.875)) ;
#134905=CARTESIAN_POINT('',(8.6,4.09462794777298,-2.875)) ;
#134906=CARTESIAN_POINT('',(8.6,3.95,-2.875)) ;
#134907=CARTESIAN_POINT('',(8.6,3.95,-2.875)) ;
#134908=CARTESIAN_POINT('',(7.36677829147199,4.5782099492339,-2.875)) ;
#134909=CARTESIAN_POINT('Origin',(7.25334304318326,5.40585602606554,-1.375)) ;
#134910=CARTESIAN_POINT('',(8.6,4.09462794777298,-1.375)) ;
#134911=CARTESIAN_POINT('',(7.25334304318326,5.40585602606554,-1.375)) ;
#134912=CARTESIAN_POINT('',(7.25334304318326,5.40585602606554,-1.375)) ;
#134913=CARTESIAN_POINT('',(4.05,5.88396692803319,-1.375)) ;
#134914=CARTESIAN_POINT('',(7.25334304318326,5.40585602606554,-1.375)) ;
#134915=CARTESIAN_POINT('',(4.05,4.6,-1.375)) ;
#134916=CARTESIAN_POINT('',(4.05,5.40585602606554,-1.375)) ;
#134917=CARTESIAN_POINT('',(7.27599715910381,4.6,-1.375)) ;
#134918=CARTESIAN_POINT('',(7.25334304318326,4.6,-1.375)) ;
#134919=CARTESIAN_POINT('',(7.36677829147199,4.5782099492339,-1.375)) ;
#134920=CARTESIAN_POINT('Origin',(7.27599715910381,4.4,-1.375)) ;
#134921=CARTESIAN_POINT('',(8.6,3.95,-1.375)) ;
#134922=CARTESIAN_POINT('',(6.94197060168454,4.79460933256464,-1.375)) ;
#134923=CARTESIAN_POINT('',(8.6,5.40585602606554,-1.375)) ;
#134924=CARTESIAN_POINT('Origin',(4.5,-2.8,-2.54)) ;
#134925=CARTESIAN_POINT('',(4.5,-2.4,-7.04214168703486)) ;
#134926=CARTESIAN_POINT('',(4.5,-2.7,-6.60315462117279)) ;
#134927=CARTESIAN_POINT('Origin',(4.5,0.,-5.08)) ;
#134928=CARTESIAN_POINT('',(4.5,-2.7,-7.62)) ;
#134929=CARTESIAN_POINT('',(4.5,-2.7,-2.54)) ;
#134930=CARTESIAN_POINT('',(4.5,-2.4,-7.62)) ;
#134931=CARTESIAN_POINT('',(4.5,-2.8,-7.62)) ;
#134932=CARTESIAN_POINT('',(4.5,-2.4,-7.00613602842582)) ;
#134933=CARTESIAN_POINT('Origin',(12.8,2.75,-2.54)) ;
#134934=CARTESIAN_POINT('',(12.7,2.75,-7.62)) ;
#134935=CARTESIAN_POINT('',(4.55912712210514,2.75,-7.62)) ;
#134936=CARTESIAN_POINT('',(12.8,2.75,-7.62)) ;
#134937=CARTESIAN_POINT('',(4.55912712210513,2.75,-6.57304604217164)) ;
#134938=CARTESIAN_POINT('',(4.55912712210514,2.75,-6.57304604217164)) ;
#134939=CARTESIAN_POINT('',(12.8,2.75,-6.57304604217164)) ;
#134940=CARTESIAN_POINT('',(12.7,2.75,-2.54)) ;
#134941=CARTESIAN_POINT('Origin',(0.,9.95,-5.08)) ;
#134942=CARTESIAN_POINT('',(0.230887397576971,9.95,-6.99486057185377)) ;
#134943=CARTESIAN_POINT('Origin',(4.5,-2.3,-2.54)) ;
#134944=CARTESIAN_POINT('',(12.7,-2.3,-7.04214168703486)) ;
#134945=CARTESIAN_POINT('',(4.6,-2.3,-7.04214168703486)) ;
#134946=CARTESIAN_POINT('',(4.5,-2.3,-7.04214168703486)) ;
#134947=CARTESIAN_POINT('',(4.6,-2.3,-7.62)) ;
#134948=CARTESIAN_POINT('',(4.6,-2.3,-7.62)) ;
#134949=CARTESIAN_POINT('',(12.7,-2.3,-7.62)) ;
#134950=CARTESIAN_POINT('',(4.5,-2.3,-7.62)) ;
#134951=CARTESIAN_POINT('',(12.7,-2.3,-2.54)) ;
#134952=CARTESIAN_POINT('Origin',(0.,0.,-7.62)) ;
#134953=CARTESIAN_POINT('Origin',(4.4,-2.7,-7.62)) ;
#134954=CARTESIAN_POINT('Origin',(4.55912712210514,2.85,-7.62)) ;
#134955=CARTESIAN_POINT('Origin',(12.7,2.65,-7.62)) ;
#134956=CARTESIAN_POINT('Origin',(12.7,-2.2,-7.62)) ;
#134957=CARTESIAN_POINT('Origin',(4.6,-2.4,-7.62)) ;
#134958=CARTESIAN_POINT('Origin',(-4.65,1.95,-7.08)) ;
#134959=CARTESIAN_POINT('',(-4.66204490261456,3.21928058320648,-7.08)) ;
#134960=CARTESIAN_POINT('',(-5.3,3.9369800677651,-7.08)) ;
#134961=CARTESIAN_POINT('',(-5.47474093186837,4.13356361611701,-7.08)) ;
#134962=CARTESIAN_POINT('',(-5.3,-1.88819660112501,-7.08)) ;
#134963=CARTESIAN_POINT('',(-5.3,-2.05,-7.08)) ;
#134964=CARTESIAN_POINT('',(-4.66204490261456,-1.5692190524323,-7.08)) ;
#134965=CARTESIAN_POINT('',(-4.69472135955,-1.58555728090001,-7.08)) ;
#134966=CARTESIAN_POINT('',(-4.66204490261456,3.35625,-7.08)) ;
#134967=CARTESIAN_POINT('Origin',(-5.4,1.95,-3.08)) ;
#134968=CARTESIAN_POINT('',(-4.66204490261456,-1.5692190524323,-3.08)) ;
#134969=CARTESIAN_POINT('',(-5.3,-1.88819660112502,-3.08)) ;
#134970=CARTESIAN_POINT('',(-5.44472135955,-1.96055728090001,-3.08)) ;
#134971=CARTESIAN_POINT('',(-5.3,3.9369800677651,-3.08)) ;
#134972=CARTESIAN_POINT('',(-5.3,4.20000000000001,-3.08)) ;
#134973=CARTESIAN_POINT('',(-4.66204490261456,3.21928058320648,-3.08)) ;
#134974=CARTESIAN_POINT('',(-4.72474093186837,3.28981361611701,-3.08)) ;
#134975=CARTESIAN_POINT('',(-4.66204490261456,-1.67500000000001,-3.08)) ;
#134976=CARTESIAN_POINT('Origin',(-4.65,1.95,-3.08)) ;
#134977=CARTESIAN_POINT('',(-3.33134808452128,1.85,-3.4023371348948)) ;
#134978=CARTESIAN_POINT('',(-3.48082994825801,1.91712723223402,-3.36579712375915)) ;
#134979=CARTESIAN_POINT('Origin',(-3.34328863644912,2.02341244982159,-3.39941833331244)) ;
#134980=CARTESIAN_POINT('',(-2.4,1.85,-3.63)) ;
#134981=CARTESIAN_POINT('',(-4.65,1.85,-3.08)) ;
#134982=CARTESIAN_POINT('',(-2.4,-0.95,-3.63)) ;
#134983=CARTESIAN_POINT('',(-2.4,1.95,-3.63)) ;
#134984=CARTESIAN_POINT('',(-3.3526478932023,-0.95,-3.39713051499499)) ;
#134985=CARTESIAN_POINT('',(-3.39999999999998,-0.95,-3.38555555555556)) ;
#134986=CARTESIAN_POINT('',(-3.44209061230229,-0.971114561800017,-3.37526673921499)) ;
#134987=CARTESIAN_POINT('Origin',(-3.3620122055811,-1.11033257691499,-3.39484146085794)) ;
#134988=CARTESIAN_POINT('',(-4.63829959356686,-1.5692190524323,-3.08286009935032)) ;
#134989=CARTESIAN_POINT('',(-4.68814869588294,-1.59414360359034,-3.07067476322862)) ;
#134990=CARTESIAN_POINT('',(-4.63829959356686,3.21928058320648,-3.08286009935032)) ;
#134991=CARTESIAN_POINT('',(-4.63829959356686,3.35625,-3.08286009935032)) ;
#134992=CARTESIAN_POINT('',(-3.45989661114215,1.89357722797868,-3.37091416172081)) ;
#134993=CARTESIAN_POINT('Origin',(-2.4,1.95,-3.63)) ;
#134994=CARTESIAN_POINT('',(-2.4,1.85,-6.53)) ;
#134995=CARTESIAN_POINT('',(-2.4,-0.95,-6.53)) ;
#134996=CARTESIAN_POINT('',(-2.4,1.95,-6.53)) ;
#134997=CARTESIAN_POINT('',(-2.4,-1.05,-6.427055690472)) ;
#134998=CARTESIAN_POINT('Origin',(-2.4,-0.950000000000003,-6.427055690472)) ;
#134999=CARTESIAN_POINT('',(-2.4,-1.05,-3.73294430952801)) ;
#135000=CARTESIAN_POINT('',(-2.4,-1.05,-3.63)) ;
#135001=CARTESIAN_POINT('Origin',(-2.4,-0.949999999999989,-3.73294430952802)) ;
#135002=CARTESIAN_POINT('',(-2.4,1.95,-3.732944309528)) ;
#135003=CARTESIAN_POINT('Origin',(-2.4,1.84999999999999,-3.73294430952802)) ;
#135004=CARTESIAN_POINT('',(-2.4,1.95,-6.427055690472)) ;
#135005=CARTESIAN_POINT('',(-2.4,1.95,-3.63)) ;
#135006=CARTESIAN_POINT('Origin',(-2.4,1.85000000000005,-6.42705569047205)) ;
#135007=CARTESIAN_POINT('Origin',(-2.4,1.95,-6.53)) ;
#135008=CARTESIAN_POINT('',(-3.3526478932023,-0.95,-6.76286948500501)) ;
#135009=CARTESIAN_POINT('',(-3.44209061230229,-0.971114561800017,-6.78473326078501)) ;
#135010=CARTESIAN_POINT('Origin',(-3.3620122055812,-1.11033257691303,-6.76515853914208)) ;
#135011=CARTESIAN_POINT('',(-2.4,-0.95,-6.53)) ;
#135012=CARTESIAN_POINT('',(-3.33134808452128,1.85,-6.7576628651052)) ;
#135013=CARTESIAN_POINT('',(-2.4,1.85,-6.53)) ;
#135014=CARTESIAN_POINT('',(-3.48082994825801,1.91712723223402,-6.79420287624085)) ;
#135015=CARTESIAN_POINT('Origin',(-3.34328863644907,2.02341244982186,-6.76058166668757)) ;
#135016=CARTESIAN_POINT('',(-4.63829959356686,3.21928058320648,-7.07713990064968)) ;
#135017=CARTESIAN_POINT('',(-4.70989661114216,3.29982722797869,-7.09464139383475)) ;
#135018=CARTESIAN_POINT('',(-4.63829959356686,-1.5692190524323,-7.07713990064968)) ;
#135019=CARTESIAN_POINT('',(-4.63829959356686,-1.67500000000001,-7.07713990064968)) ;
#135020=CARTESIAN_POINT('',(-3.43814869588292,-0.969143603590331,-6.78376968121583)) ;
#135021=CARTESIAN_POINT('Origin',(0.,1.95,-5.08)) ;
#135022=CARTESIAN_POINT('',(-3.35509339356897,1.95,-3.49947703554448)) ;
#135023=CARTESIAN_POINT('',(0.175392621986784,1.95,-4.36248472823589)) ;
#135024=CARTESIAN_POINT('',(-3.35509339356897,1.95,-6.66052296445552)) ;
#135025=CARTESIAN_POINT('',(-3.35509339356897,1.95,-6.77444444444444)) ;
#135026=CARTESIAN_POINT('',(0.175392621986784,1.95,-5.79751527176412)) ;
#135027=CARTESIAN_POINT('Origin',(0.,-1.05,-5.08)) ;
#135028=CARTESIAN_POINT('',(-3.37639320225,-1.05,-6.66572958435533)) ;
#135029=CARTESIAN_POINT('',(-3.42374530904768,-1.05,-6.67730454379476)) ;
#135030=CARTESIAN_POINT('',(-3.37639320225,-1.05,-3.49427041564467)) ;
#135031=CARTESIAN_POINT('',(-3.37639320225,-1.05,-5.08)) ;
#135032=CARTESIAN_POINT('',(-2.4237453090477,-1.05,-3.72713990064968)) ;
#135033=CARTESIAN_POINT('Origin',(-3.39999999999998,-1.05,-5.08)) ;
#135034=CARTESIAN_POINT('',(-3.4211145618,-1.06055728090001,-3.47240663986467)) ;
#135035=CARTESIAN_POINT('',(-3.4211145618,-1.06055728090001,-6.68759336013533)) ;
#135036=CARTESIAN_POINT('',(-3.4211145618,-1.06055728090001,-5.08)) ;
#135037=CARTESIAN_POINT('',(-4.61732354306457,-1.65866177153229,-6.98)) ;
#135038=CARTESIAN_POINT('',(-4.66717264538064,-1.68358632269033,-6.99218533612171)) ;
#135039=CARTESIAN_POINT('',(-5.34472135954999,-2.022360679775,-6.98)) ;
#135040=CARTESIAN_POINT('',(-5.4,-2.05,-6.98)) ;
#135041=CARTESIAN_POINT('',(-5.34472135954999,-2.022360679775,-3.18)) ;
#135042=CARTESIAN_POINT('',(-5.34472135954999,-2.022360679775,-3.08)) ;
#135043=CARTESIAN_POINT('',(-4.61732354306457,-1.65866177153229,-3.18)) ;
#135044=CARTESIAN_POINT('',(-4.65,-1.67500000000001,-3.18)) ;
#135045=CARTESIAN_POINT('',(-3.41717264538063,-1.05858632269032,-3.47337021943385)) ;
#135046=CARTESIAN_POINT('Origin',(-5.4,4.20000000000001,-2.54)) ;
#135047=CARTESIAN_POINT('',(-5.37474093186837,4.17158354835192,-3.18)) ;
#135048=CARTESIAN_POINT('',(-5.37474093186837,4.17158354835192,-6.98)) ;
#135049=CARTESIAN_POINT('',(-5.37474093186837,4.17158354835192,-7.08)) ;
#135050=CARTESIAN_POINT('',(-4.58730397074619,3.28571696708947,-6.98)) ;
#135051=CARTESIAN_POINT('',(-4.65,3.35625,-6.98)) ;
#135052=CARTESIAN_POINT('',(-3.42983432543734,1.98356361611701,-6.69706297559117)) ;
#135053=CARTESIAN_POINT('',(-3.40890098832149,1.96001361186167,-6.69194593762952)) ;
#135054=CARTESIAN_POINT('',(-3.42983432543734,1.98356361611701,-3.46293702440883)) ;
#135055=CARTESIAN_POINT('',(-3.42983432543734,1.98356361611701,-3.38555555555556)) ;
#135056=CARTESIAN_POINT('',(-4.58730397074619,3.28571696708947,-3.18)) ;
#135057=CARTESIAN_POINT('',(-4.65890098832149,3.36626361186168,-3.16249850681493)) ;
#135058=CARTESIAN_POINT('',(-5.4,4.20000000000001,-3.18)) ;
#135059=CARTESIAN_POINT('Origin',(-3.15,-3.9,-4.08)) ;
#135060=CARTESIAN_POINT('',(-3.15,-3.95,-4.18)) ;
#135061=CARTESIAN_POINT('',(-3.15,-3.85,-4.18)) ;
#135062=CARTESIAN_POINT('',(-3.15,-3.75,-4.18)) ;
#135063=CARTESIAN_POINT('',(-3.15,-3.85,-5.98)) ;
#135064=CARTESIAN_POINT('',(-3.15,-3.85,-4.08)) ;
#135065=CARTESIAN_POINT('',(-3.15,-3.95,-5.98)) ;
#135066=CARTESIAN_POINT('',(-3.15,-4.05,-5.98)) ;
#135067=CARTESIAN_POINT('',(-3.15,-3.95,-4.08)) ;
#135068=CARTESIAN_POINT('Origin',(-4.4,-3.9,-6.08)) ;
#135069=CARTESIAN_POINT('',(-3.25,-3.85,-6.08)) ;
#135070=CARTESIAN_POINT('',(-4.3,-3.85,-6.08)) ;
#135071=CARTESIAN_POINT('',(-4.4,-3.85,-6.08)) ;
#135072=CARTESIAN_POINT('',(-4.3,-3.95,-6.08)) ;
#135073=CARTESIAN_POINT('',(-4.3,-4.05,-6.08)) ;
#135074=CARTESIAN_POINT('',(-3.25,-3.95,-6.08)) ;
#135075=CARTESIAN_POINT('',(-4.4,-3.95,-6.08)) ;
#135076=CARTESIAN_POINT('',(-3.25,-3.75,-6.08)) ;
#135077=CARTESIAN_POINT('Origin',(-4.4,-3.9,-4.08)) ;
#135078=CARTESIAN_POINT('',(-4.4,-3.85,-5.98)) ;
#135079=CARTESIAN_POINT('',(-4.4,-3.85,-4.18)) ;
#135080=CARTESIAN_POINT('',(-4.4,-3.85,-4.08)) ;
#135081=CARTESIAN_POINT('',(-4.4,-3.95,-4.18)) ;
#135082=CARTESIAN_POINT('',(-4.4,-4.05,-4.18)) ;
#135083=CARTESIAN_POINT('',(-4.4,-3.95,-5.98)) ;
#135084=CARTESIAN_POINT('',(-4.4,-3.95,-4.08)) ;
#135085=CARTESIAN_POINT('',(-4.4,-3.75,-5.98)) ;
#135086=CARTESIAN_POINT('Origin',(-4.4,-3.9,-4.08)) ;
#135087=CARTESIAN_POINT('',(-4.3,-3.95,-4.08)) ;
#135088=CARTESIAN_POINT('',(-4.3,-3.85,-4.08)) ;
#135089=CARTESIAN_POINT('',(-4.3,-3.75,-4.08)) ;
#135090=CARTESIAN_POINT('',(-3.25,-3.85,-4.08)) ;
#135091=CARTESIAN_POINT('',(-4.4,-3.85,-4.08)) ;
#135092=CARTESIAN_POINT('',(-3.25,-3.95,-4.08)) ;
#135093=CARTESIAN_POINT('',(-3.25,-4.05,-4.08)) ;
#135094=CARTESIAN_POINT('',(-4.4,-3.95,-4.08)) ;
#135095=CARTESIAN_POINT('Origin',(0.,-3.75,-5.08)) ;
#135096=CARTESIAN_POINT('',(-3.25,-3.75,-4.18)) ;
#135097=CARTESIAN_POINT('',(-4.3,-3.75,-4.18)) ;
#135098=CARTESIAN_POINT('',(-1.56125112837913E-16,-3.75,-4.18)) ;
#135099=CARTESIAN_POINT('',(-4.3,-3.75,-5.98)) ;
#135100=CARTESIAN_POINT('',(-4.3,-3.75,-5.08)) ;
#135101=CARTESIAN_POINT('',(-3.25,-3.75,-5.98)) ;
#135102=CARTESIAN_POINT('',(-1.56125112837913E-16,-3.75,-5.98)) ;
#135103=CARTESIAN_POINT('',(-3.25,-3.75,-5.08)) ;
#135104=CARTESIAN_POINT('',(-4.15,-3.75,-5.93)) ;
#135105=CARTESIAN_POINT('',(-3.4,-3.75,-5.93)) ;
#135106=CARTESIAN_POINT('',(-4.15,-3.75,-5.93)) ;
#135107=CARTESIAN_POINT('',(-4.25,-3.75,-5.83)) ;
#135108=CARTESIAN_POINT('Origin',(-4.15,-3.75,-5.83)) ;
#135109=CARTESIAN_POINT('',(-4.25,-3.75,-4.33)) ;
#135110=CARTESIAN_POINT('',(-4.25,-3.75,-4.33)) ;
#135111=CARTESIAN_POINT('',(-4.15,-3.75,-4.23)) ;
#135112=CARTESIAN_POINT('Origin',(-4.15,-3.75,-4.33)) ;
#135113=CARTESIAN_POINT('',(-3.4,-3.75,-4.23)) ;
#135114=CARTESIAN_POINT('',(-3.4,-3.75,-4.23)) ;
#135115=CARTESIAN_POINT('',(-3.3,-3.75,-4.33)) ;
#135116=CARTESIAN_POINT('Origin',(-3.4,-3.75,-4.33)) ;
#135117=CARTESIAN_POINT('',(-3.3,-3.75,-5.83)) ;
#135118=CARTESIAN_POINT('',(-3.3,-3.75,-5.83)) ;
#135119=CARTESIAN_POINT('Origin',(-3.4,-3.75,-5.83)) ;
#135120=CARTESIAN_POINT('Origin',(-3.4,-3.75,-5.83)) ;
#135121=CARTESIAN_POINT('',(-3.4,-3.9,-5.93)) ;
#135122=CARTESIAN_POINT('',(-3.3,-3.9,-5.83)) ;
#135123=CARTESIAN_POINT('Origin',(-3.4,-3.9,-5.83)) ;
#135124=CARTESIAN_POINT('',(-3.4,-3.75,-5.93)) ;
#135125=CARTESIAN_POINT('',(-3.3,-3.75,-5.83)) ;
#135126=CARTESIAN_POINT('Origin',(-4.15,-3.75,-5.93)) ;
#135127=CARTESIAN_POINT('',(-4.15,-3.9,-5.93)) ;
#135128=CARTESIAN_POINT('',(-4.15,-3.9,-5.93)) ;
#135129=CARTESIAN_POINT('',(-4.15,-3.75,-5.93)) ;
#135130=CARTESIAN_POINT('Origin',(-4.15,-3.75,-5.83)) ;
#135131=CARTESIAN_POINT('',(-4.25,-3.9,-5.83)) ;
#135132=CARTESIAN_POINT('Origin',(-4.15,-3.9,-5.83)) ;
#135133=CARTESIAN_POINT('',(-4.25,-3.75,-5.83)) ;
#135134=CARTESIAN_POINT('Origin',(-4.25,-3.75,-4.33)) ;
#135135=CARTESIAN_POINT('',(-4.25,-3.9,-4.33)) ;
#135136=CARTESIAN_POINT('',(-4.25,-3.9,-4.33)) ;
#135137=CARTESIAN_POINT('',(-4.25,-3.75,-4.33)) ;
#135138=CARTESIAN_POINT('Origin',(-4.15,-3.75,-4.33)) ;
#135139=CARTESIAN_POINT('',(-4.15,-3.9,-4.23)) ;
#135140=CARTESIAN_POINT('Origin',(-4.15,-3.9,-4.33)) ;
#135141=CARTESIAN_POINT('',(-4.15,-3.75,-4.23)) ;
#135142=CARTESIAN_POINT('Origin',(-3.4,-3.75,-4.23)) ;
#135143=CARTESIAN_POINT('',(-3.4,-3.9,-4.23)) ;
#135144=CARTESIAN_POINT('',(-3.4,-3.9,-4.23)) ;
#135145=CARTESIAN_POINT('',(-3.4,-3.75,-4.23)) ;
#135146=CARTESIAN_POINT('Origin',(-3.4,-3.75,-4.33)) ;
#135147=CARTESIAN_POINT('',(-3.3,-3.9,-4.33)) ;
#135148=CARTESIAN_POINT('Origin',(-3.4,-3.9,-4.33)) ;
#135149=CARTESIAN_POINT('',(-3.3,-3.75,-4.33)) ;
#135150=CARTESIAN_POINT('Origin',(-3.3,-3.75,-5.83)) ;
#135151=CARTESIAN_POINT('',(-3.3,-3.9,-5.83)) ;
#135152=CARTESIAN_POINT('Origin',(0.,-3.9,-5.08)) ;
#135153=CARTESIAN_POINT('Origin',(0.,9.95,-5.08)) ;
#135154=CARTESIAN_POINT('',(-0.230887397576972,9.95,-3.16513942814623)) ;
#135155=CARTESIAN_POINT('Origin',(-0.321518176280637,8.95,-3.2074012543203)) ;
#135156=CARTESIAN_POINT('',(-0.321518176280637,9.05,-3.2074012543203)) ;
#135157=CARTESIAN_POINT('',(1.22782596331729,9.85,-6.529980483939)) ;
#135158=CARTESIAN_POINT('Origin',(-1.22782596331729,8.95,-3.630019516061)) ;
#135159=CARTESIAN_POINT('',(-1.22782596331729,9.05,-3.630019516061)) ;
#135160=CARTESIAN_POINT('',(-1.22782596331729,9.85,-3.630019516061)) ;
#135161=CARTESIAN_POINT('Origin',(0.,8.95,-5.08)) ;
#135162=CARTESIAN_POINT('',(-0.362523114814661,8.95,-5.24904730469628)) ;
#135163=CARTESIAN_POINT('',(0.36252311481466,8.95,-4.91095269530372)) ;
#135164=CARTESIAN_POINT('Origin',(-2.65,10.8,-6.08)) ;
#135165=CARTESIAN_POINT('',(-2.65,10.75,-5.98)) ;
#135166=CARTESIAN_POINT('',(-2.65,10.75,-4.18)) ;
#135167=CARTESIAN_POINT('',(-2.65,10.75,-6.08)) ;
#135168=CARTESIAN_POINT('',(-2.65,10.85,-4.18)) ;
#135169=CARTESIAN_POINT('',(-2.65,10.95,-4.18)) ;
#135170=CARTESIAN_POINT('',(-2.65,10.85,-5.98)) ;
#135171=CARTESIAN_POINT('',(-2.65,10.85,-6.08)) ;
#135172=CARTESIAN_POINT('',(-2.65,10.65,-5.98)) ;
#135173=CARTESIAN_POINT('Origin',(-3.9,10.8,-4.08)) ;
#135174=CARTESIAN_POINT('',(-2.75,10.85,-4.08)) ;
#135175=CARTESIAN_POINT('',(-2.75,10.75,-4.08)) ;
#135176=CARTESIAN_POINT('',(-2.75,10.65,-4.08)) ;
#135177=CARTESIAN_POINT('',(-3.8,10.75,-4.08)) ;
#135178=CARTESIAN_POINT('',(-3.9,10.75,-4.08)) ;
#135179=CARTESIAN_POINT('',(-3.8,10.85,-4.08)) ;
#135180=CARTESIAN_POINT('',(-3.8,10.95,-4.08)) ;
#135181=CARTESIAN_POINT('',(-3.9,10.85,-4.08)) ;
#135182=CARTESIAN_POINT('Origin',(-3.9,10.8,-6.08)) ;
#135183=CARTESIAN_POINT('',(-3.9,10.85,-4.18)) ;
#135184=CARTESIAN_POINT('',(-3.9,10.75,-4.18)) ;
#135185=CARTESIAN_POINT('',(-3.9,10.65,-4.18)) ;
#135186=CARTESIAN_POINT('',(-3.9,10.75,-5.98)) ;
#135187=CARTESIAN_POINT('',(-3.9,10.75,-6.08)) ;
#135188=CARTESIAN_POINT('',(-3.9,10.85,-5.98)) ;
#135189=CARTESIAN_POINT('',(-3.9,10.95,-5.98)) ;
#135190=CARTESIAN_POINT('',(-3.9,10.85,-6.08)) ;
#135191=CARTESIAN_POINT('Origin',(-3.9,10.8,-6.08)) ;
#135192=CARTESIAN_POINT('',(-3.8,10.75,-6.08)) ;
#135193=CARTESIAN_POINT('',(-2.75,10.75,-6.08)) ;
#135194=CARTESIAN_POINT('',(-3.9,10.75,-6.08)) ;
#135195=CARTESIAN_POINT('',(-2.75,10.85,-6.08)) ;
#135196=CARTESIAN_POINT('',(-2.75,10.95,-6.08)) ;
#135197=CARTESIAN_POINT('',(-3.8,10.85,-6.08)) ;
#135198=CARTESIAN_POINT('',(-3.9,10.85,-6.08)) ;
#135199=CARTESIAN_POINT('',(-3.8,10.65,-6.08)) ;
#135200=CARTESIAN_POINT('Origin',(0.,10.65,-5.08)) ;
#135201=CARTESIAN_POINT('',(-3.8,10.65,-4.18)) ;
#135202=CARTESIAN_POINT('',(-2.75,10.65,-4.18)) ;
#135203=CARTESIAN_POINT('',(1.56125112837912E-16,10.65,-4.18)) ;
#135204=CARTESIAN_POINT('',(-2.75,10.65,-5.98)) ;
#135205=CARTESIAN_POINT('',(-2.75,10.65,-5.08)) ;
#135206=CARTESIAN_POINT('',(-3.8,10.65,-5.98)) ;
#135207=CARTESIAN_POINT('',(-1.56125112837913E-16,10.65,-5.98)) ;
#135208=CARTESIAN_POINT('',(-3.8,10.65,-5.08)) ;
#135209=CARTESIAN_POINT('',(-3.65,10.65,-4.23)) ;
#135210=CARTESIAN_POINT('',(-2.9,10.65,-4.23)) ;
#135211=CARTESIAN_POINT('',(-3.65,10.65,-4.23)) ;
#135212=CARTESIAN_POINT('',(-3.75,10.65,-4.33)) ;
#135213=CARTESIAN_POINT('Origin',(-3.65,10.65,-4.33)) ;
#135214=CARTESIAN_POINT('',(-3.75,10.65,-5.83)) ;
#135215=CARTESIAN_POINT('',(-3.75,10.65,-5.83)) ;
#135216=CARTESIAN_POINT('',(-3.65,10.65,-5.93)) ;
#135217=CARTESIAN_POINT('Origin',(-3.65,10.65,-5.83)) ;
#135218=CARTESIAN_POINT('',(-2.9,10.65,-5.93)) ;
#135219=CARTESIAN_POINT('',(-2.9,10.65,-5.93)) ;
#135220=CARTESIAN_POINT('',(-2.8,10.65,-5.83)) ;
#135221=CARTESIAN_POINT('Origin',(-2.9,10.65,-5.83)) ;
#135222=CARTESIAN_POINT('',(-2.8,10.65,-4.33)) ;
#135223=CARTESIAN_POINT('',(-2.8,10.65,-4.33)) ;
#135224=CARTESIAN_POINT('Origin',(-2.9,10.65,-4.33)) ;
#135225=CARTESIAN_POINT('Origin',(-2.9,10.65,-4.33)) ;
#135226=CARTESIAN_POINT('',(-2.8,10.7,-4.33)) ;
#135227=CARTESIAN_POINT('',(-2.8,10.65,-4.33)) ;
#135228=CARTESIAN_POINT('',(-2.9,10.7,-4.23)) ;
#135229=CARTESIAN_POINT('Origin',(-2.9,10.7,-4.33)) ;
#135230=CARTESIAN_POINT('',(-2.9,10.65,-4.23)) ;
#135231=CARTESIAN_POINT('Origin',(-3.65,10.65,-4.23)) ;
#135232=CARTESIAN_POINT('',(-3.65,10.7,-4.23)) ;
#135233=CARTESIAN_POINT('',(-3.65,10.7,-4.23)) ;
#135234=CARTESIAN_POINT('',(-3.65,10.65,-4.23)) ;
#135235=CARTESIAN_POINT('Origin',(-3.65,10.65,-4.33)) ;
#135236=CARTESIAN_POINT('',(-3.75,10.7,-4.33)) ;
#135237=CARTESIAN_POINT('Origin',(-3.65,10.7,-4.33)) ;
#135238=CARTESIAN_POINT('',(-3.75,10.65,-4.33)) ;
#135239=CARTESIAN_POINT('Origin',(-3.75,10.65,-5.83)) ;
#135240=CARTESIAN_POINT('',(-3.75,10.7,-5.83)) ;
#135241=CARTESIAN_POINT('',(-3.75,10.7,-5.83)) ;
#135242=CARTESIAN_POINT('',(-3.75,10.65,-5.83)) ;
#135243=CARTESIAN_POINT('Origin',(-3.65,10.65,-5.83)) ;
#135244=CARTESIAN_POINT('',(-3.65,10.7,-5.93)) ;
#135245=CARTESIAN_POINT('Origin',(-3.65,10.7,-5.83)) ;
#135246=CARTESIAN_POINT('',(-3.65,10.65,-5.93)) ;
#135247=CARTESIAN_POINT('Origin',(-2.9,10.65,-5.93)) ;
#135248=CARTESIAN_POINT('',(-2.9,10.7,-5.93)) ;
#135249=CARTESIAN_POINT('',(-2.9,10.7,-5.93)) ;
#135250=CARTESIAN_POINT('',(-2.9,10.65,-5.93)) ;
#135251=CARTESIAN_POINT('Origin',(-2.9,10.65,-5.83)) ;
#135252=CARTESIAN_POINT('',(-2.8,10.7,-5.83)) ;
#135253=CARTESIAN_POINT('Origin',(-2.9,10.7,-5.83)) ;
#135254=CARTESIAN_POINT('',(-2.8,10.65,-5.83)) ;
#135255=CARTESIAN_POINT('Origin',(-2.8,10.65,-4.33)) ;
#135256=CARTESIAN_POINT('',(-2.8,10.7,-4.33)) ;
#135257=CARTESIAN_POINT('Origin',(0.,10.8,-5.08)) ;
#135258=CARTESIAN_POINT('',(-3.65,10.8,-4.33)) ;
#135259=CARTESIAN_POINT('',(-2.9,10.8,-4.33)) ;
#135260=CARTESIAN_POINT('',(0.,10.8,-4.33)) ;
#135261=CARTESIAN_POINT('',(-2.9,10.8,-5.83)) ;
#135262=CARTESIAN_POINT('',(-2.9,10.8,-5.08)) ;
#135263=CARTESIAN_POINT('',(-3.65,10.8,-5.83)) ;
#135264=CARTESIAN_POINT('',(0.,10.8,-5.83)) ;
#135265=CARTESIAN_POINT('',(-3.65,10.8,-5.08)) ;
#135266=CARTESIAN_POINT('Origin',(4.5,2.75,-6.455)) ;
#135267=CARTESIAN_POINT('',(4.5,2.63356010126946,-6.47440664978842)) ;
#135268=CARTESIAN_POINT('',(4.6,2.11643989873054,-6.56059335021158)) ;
#135269=CARTESIAN_POINT('',(4.6,2.11643989873054,-6.56059335021158)) ;
#135270=CARTESIAN_POINT('',(12.7,2.11643989873054,-6.56059335021158)) ;
#135271=CARTESIAN_POINT('',(12.8,2.11643989873054,-6.56059335021158)) ;
#135272=CARTESIAN_POINT('',(12.7,2.75,-6.455)) ;
#135273=CARTESIAN_POINT('Origin',(4.5,2.,-6.58)) ;
#135274=CARTESIAN_POINT('',(4.6,2.,-6.46195395782836)) ;
#135275=CARTESIAN_POINT('',(4.6,2.,-3.58)) ;
#135276=CARTESIAN_POINT('',(12.7,2.,-6.46195395782836)) ;
#135277=CARTESIAN_POINT('',(12.7,2.,-6.58)) ;
#135278=CARTESIAN_POINT('',(4.5,2.,-6.46195395782836)) ;
#135279=CARTESIAN_POINT('Origin',(4.5,2.,-3.58)) ;
#135280=CARTESIAN_POINT('',(4.6,2.63356010126946,-3.68559335021158)) ;
#135281=CARTESIAN_POINT('',(4.6,2.63356010126947,-3.68559335021158)) ;
#135282=CARTESIAN_POINT('',(4.5,2.63356010126946,-3.68559335021158)) ;
#135283=CARTESIAN_POINT('',(12.7,2.,-3.58)) ;
#135284=CARTESIAN_POINT('Origin',(4.5,0.,-5.08)) ;
#135285=CARTESIAN_POINT('',(4.5,2.72431432344521,-3.77263481664499)) ;
#135286=CARTESIAN_POINT('',(4.5,2.72431432344521,-5.08)) ;
#135287=CARTESIAN_POINT('',(4.5,2.61712020253893,-3.78423274259479)) ;
#135288=CARTESIAN_POINT('Origin',(4.5,2.65,-3.58695395782836)) ;
#135289=CARTESIAN_POINT('',(4.5,2.1,-3.69804604217164)) ;
#135290=CARTESIAN_POINT('',(4.5,2.1,-3.69804604217164)) ;
#135291=CARTESIAN_POINT('',(4.5,2.1,-6.46195395782836)) ;
#135292=CARTESIAN_POINT('',(4.5,2.1,-6.58)) ;
#135293=CARTESIAN_POINT('',(4.5,2.61712020253893,-6.37576725740521)) ;
#135294=CARTESIAN_POINT('Origin',(10.3,0.,-5.08)) ;
#135295=CARTESIAN_POINT('Origin',(0.584645609909621,0.,-5.08)) ;
#135296=CARTESIAN_POINT('',(4.6,-2.32258064516129,-3.1811532060953)) ;
#135297=CARTESIAN_POINT('',(4.6,-2.79310344827574,-3.98520635404193)) ;
#135298=CARTESIAN_POINT('Origin',(4.6,0.,-5.08)) ;
#135299=CARTESIAN_POINT('',(4.6,-2.79310344827574,-6.17479364595807)) ;
#135300=CARTESIAN_POINT('Origin',(4.6,0.,-5.08)) ;
#135301=CARTESIAN_POINT('',(4.6,-2.32258064516129,-6.9788467939047)) ;
#135302=CARTESIAN_POINT('Origin',(4.6,0.,-5.08)) ;
#135303=CARTESIAN_POINT('',(12.7,-2.32258064516129,-6.9788467939047)) ;
#135304=CARTESIAN_POINT('',(0.584645609909621,-2.32258064516129,-6.9788467939047)) ;
#135305=CARTESIAN_POINT('',(12.7,-2.32258064516129,-3.1811532060953)) ;
#135306=CARTESIAN_POINT('Origin',(12.7,0.,-5.08)) ;
#135307=CARTESIAN_POINT('',(0.584645609909621,-2.32258064516129,-3.1811532060953)) ;
#135308=CARTESIAN_POINT('Ctrl Pts',(-5.37474093186837,4.17158354835192,
-3.18)) ;
#135309=CARTESIAN_POINT('Ctrl Pts',(-5.4,4.2,-3.18)) ;
#135310=CARTESIAN_POINT('Ctrl Pts',(-5.4,4.23801993223491,-3.18)) ;
#135311=CARTESIAN_POINT('Ctrl Pts',(-5.37474093064202,4.17158354697228,
-3.15374656406104)) ;
#135312=CARTESIAN_POINT('Ctrl Pts',(-5.4,4.19999999724801,-3.1424814127989)) ;
#135313=CARTESIAN_POINT('Ctrl Pts',(-5.4,4.23801992976516,-3.12749312809026)) ;
#135314=CARTESIAN_POINT('Ctrl Pts',(-5.36668583490655,4.14629949399955,
-3.12780128688412)) ;
#135315=CARTESIAN_POINT('Ctrl Pts',(-5.4,4.16739198385624,-3.10466783506586)) ;
#135316=CARTESIAN_POINT('Ctrl Pts',(-5.4,4.20557579169425,-3.07560257376825)) ;
#135317=CARTESIAN_POINT('Ctrl Pts',(-5.33901380460609,4.05944006555646,
-3.09077735687857)) ;
#135318=CARTESIAN_POINT('Ctrl Pts',(-5.4,4.06625640449639,-3.06313263661411)) ;
#135319=CARTESIAN_POINT('Ctrl Pts',(-5.4,4.09411900298411,-3.00155471375713)) ;
#135320=CARTESIAN_POINT('Ctrl Pts',(-5.31962206268973,3.99857154231911,
-3.08)) ;
#135321=CARTESIAN_POINT('Ctrl Pts',(-5.39999999999997,3.99346933127512,
-3.06200350742645)) ;
#135322=CARTESIAN_POINT('Ctrl Pts',(-5.4,4.0160133758189,-2.98000000048114)) ;
#135323=CARTESIAN_POINT('Ctrl Pts',(-5.3,3.9369800677651,-3.08)) ;
#135324=CARTESIAN_POINT('Ctrl Pts',(-5.4,3.9369800677651,-3.08)) ;
#135325=CARTESIAN_POINT('Ctrl Pts',(-5.4,3.9369800677651,-2.98)) ;
#135326=CARTESIAN_POINT('Origin',(-5.3,4.23801993223491,-3.18)) ;
#135327=CARTESIAN_POINT('Ctrl Pts',(-5.3,3.9369800677651,-3.08)) ;
#135328=CARTESIAN_POINT('Ctrl Pts',(-5.31962206268973,3.99857154231912,
-3.08)) ;
#135329=CARTESIAN_POINT('Ctrl Pts',(-5.33901380460609,4.05944006555646,
-3.09077735687857)) ;
#135330=CARTESIAN_POINT('Ctrl Pts',(-5.36668583490655,4.14629949399955,
-3.12780128688412)) ;
#135331=CARTESIAN_POINT('Ctrl Pts',(-5.37474093064202,4.17158354697228,
-3.15374656406104)) ;
#135332=CARTESIAN_POINT('Ctrl Pts',(-5.37474093186837,4.17158354835192,
-3.18)) ;
#135333=CARTESIAN_POINT('Origin',(-5.3,3.9369800677651,-2.98)) ;
#135334=CARTESIAN_POINT('Origin',(-4.6737453090477,1.85,-3.17713990064968)) ;
#135335=CARTESIAN_POINT('Origin',(-3.35509339356897,1.85,-3.49947703554448)) ;
#135336=CARTESIAN_POINT('Ctrl Pts',(-3.35509339356897,1.95,-3.49947703554448)) ;
#135337=CARTESIAN_POINT('Ctrl Pts',(-3.33134808452128,1.95,-3.4023371348948)) ;
#135338=CARTESIAN_POINT('Ctrl Pts',(-3.33134808452128,1.85,-3.4023371348948)) ;
#135339=CARTESIAN_POINT('Ctrl Pts',(-3.38343213690418,1.95,-3.48562253880281)) ;
#135340=CARTESIAN_POINT('Ctrl Pts',(-3.36046743872482,1.94345445676969,
-3.39521907053391)) ;
#135341=CARTESIAN_POINT('Ctrl Pts',(-3.38803897426452,1.85000000162387,
-3.38847936184645)) ;
#135342=CARTESIAN_POINT('Ctrl Pts',(-3.41101314049054,1.96238978305186,
-3.47213849291613)) ;
#135343=CARTESIAN_POINT('Ctrl Pts',(-3.39538881861724,1.95068928167333,
-3.38668273322682)) ;
#135344=CARTESIAN_POINT('Ctrl Pts',(-3.44316973238528,1.87475949194142,
-3.37500295430582)) ;
#135345=CARTESIAN_POINT('Ctrl Pts',(-3.42983432543734,1.98356361611701,
-3.46293702440883)) ;
#135346=CARTESIAN_POINT('Ctrl Pts',(-3.42093333711585,1.97355000425533,
-3.3804385175939)) ;
#135347=CARTESIAN_POINT('Ctrl Pts',(-3.48082994825801,1.91712723223402,
-3.36579712375916)) ;
#135348=CARTESIAN_POINT('Origin',(-3.50457525730571,1.91712723223402,-3.46293702440883)) ;
#135349=CARTESIAN_POINT('Origin',(-3.36128627567757,2.03621361435731,-3.49644940433506)) ;
#135350=CARTESIAN_POINT('Origin',(-4.05330900605469,2.53445269957662,-3.32880210804797)) ;
#135351=CARTESIAN_POINT('Origin',(-4.66204490261456,3.21928058320648,-3.18)) ;
#135352=CARTESIAN_POINT('Origin',(-4.35749955255802,2.87666706439287,-3.18)) ;
#135353=CARTESIAN_POINT('Origin',(-4.66204490261456,3.21928058320648,-3.18)) ;
#135354=CARTESIAN_POINT('Origin',(-5.3,5.2,-2.98)) ;
#135355=CARTESIAN_POINT('Origin',(-5.3,-1.88819660112502,-2.98)) ;
#135356=CARTESIAN_POINT('Origin',(-5.3,4.23801993223491,-2.54)) ;
#135357=CARTESIAN_POINT('Origin',(-5.3,4.23801993223491,-6.98)) ;
#135358=CARTESIAN_POINT('Origin',(-3.35509339356897,2.05,-5.08)) ;
#135359=CARTESIAN_POINT('Origin',(-3.36128627567745,2.03621361435763,-6.66355059566492)) ;
#135360=CARTESIAN_POINT('Origin',(-2.4237453090477,1.85,-6.43286009935032)) ;
#135361=CARTESIAN_POINT('Origin',(-3.35509339356897,1.85,-6.66052296445552)) ;
#135362=CARTESIAN_POINT('Origin',(-4.66204490261456,3.21928058320648,-3.18)) ;
#135363=CARTESIAN_POINT('Origin',(-4.66204490261456,3.21928058320648,-3.18)) ;
#135364=CARTESIAN_POINT('Ctrl Pts',(-5.29976814257747,-1.88802911972918,
-3.07999982737782)) ;
#135365=CARTESIAN_POINT('Ctrl Pts',(-5.4,-1.88802831720456,-3.08023259354298)) ;
#135366=CARTESIAN_POINT('Ctrl Pts',(-5.4,-1.88791746283071,-2.98000016246237)) ;
#135367=CARTESIAN_POINT('Ctrl Pts',(-5.31153957531164,-1.92331224822996,
-3.07998646768893)) ;
#135368=CARTESIAN_POINT('Ctrl Pts',(-5.4,-1.92148676945295,-3.06897789253806)) ;
#135369=CARTESIAN_POINT('Ctrl Pts',(-5.4,-1.94671708614657,-2.97993171302848)) ;
#135370=CARTESIAN_POINT('Ctrl Pts',(-5.32318090226695,-1.95817527052251,
-3.09078449726813)) ;
#135371=CARTESIAN_POINT('Ctrl Pts',(-5.4,-1.96527310172481,-3.07216338375286)) ;
#135372=CARTESIAN_POINT('Ctrl Pts',(-5.4,-2.00485091174287,-3.00149607488934)) ;
#135373=CARTESIAN_POINT('Ctrl Pts',(-5.33978950165956,-2.00789652656154,
-3.12786496501963)) ;
#135374=CARTESIAN_POINT('Ctrl Pts',(-5.4,-2.02908601268745,-3.11136651453166)) ;
#135375=CARTESIAN_POINT('Ctrl Pts',(-5.4,-2.087770056524,-3.07566121263605)) ;
#135376=CARTESIAN_POINT('Ctrl Pts',(-5.34461954754097,-2.02234798681675,
-3.15384614471832)) ;
#135377=CARTESIAN_POINT('Ctrl Pts',(-5.4,-2.04997459329993,-3.14567566484002)) ;
#135378=CARTESIAN_POINT('Ctrl Pts',(-5.4,-2.1118797455067,-3.12765768697395)) ;
#135379=CARTESIAN_POINT('Ctrl Pts',(-5.34460423617422,-2.02230212313483,
-3.18012475187013)) ;
#135380=CARTESIAN_POINT('Ctrl Pts',(-5.4,-2.04990938338631,-3.18016375427654)) ;
#135381=CARTESIAN_POINT('Ctrl Pts',(-5.4,-2.11180321723903,-3.18024966888043)) ;
#135382=CARTESIAN_POINT('Origin',(-5.29999999999999,-1.88819660112499,-3.18000000000002)) ;
#135383=CARTESIAN_POINT('Origin',(-5.3,-2.11180339887499,-3.18)) ;
#135384=CARTESIAN_POINT('Ctrl Pts',(-5.3,3.9369800677651,-7.08)) ;
#135385=CARTESIAN_POINT('Ctrl Pts',(-5.4,3.9369800677651,-7.08)) ;
#135386=CARTESIAN_POINT('Ctrl Pts',(-5.4,3.9369800677651,-7.18)) ;
#135387=CARTESIAN_POINT('Ctrl Pts',(-5.31962206268973,3.99857154231911,
-7.08)) ;
#135388=CARTESIAN_POINT('Ctrl Pts',(-5.4,3.99346933127505,-7.09799649257373)) ;
#135389=CARTESIAN_POINT('Ctrl Pts',(-5.4,4.01601337581889,-7.17999999951891)) ;
#135390=CARTESIAN_POINT('Ctrl Pts',(-5.3390138046061,4.05944006555648,-7.06922264312143)) ;
#135391=CARTESIAN_POINT('Ctrl Pts',(-5.4,4.06625640449641,-7.09686736338591)) ;
#135392=CARTESIAN_POINT('Ctrl Pts',(-5.4,4.09411900298413,-7.15844528624287)) ;
#135393=CARTESIAN_POINT('Ctrl Pts',(-5.36668583490654,4.14629949399953,
-7.03219871311588)) ;
#135394=CARTESIAN_POINT('Ctrl Pts',(-5.4,4.16739198385622,-7.05533216493412)) ;
#135395=CARTESIAN_POINT('Ctrl Pts',(-5.4,4.20557579169423,-7.08439742623175)) ;
#135396=CARTESIAN_POINT('Ctrl Pts',(-5.37474093064202,4.17158354697228,
-7.00625343593896)) ;
#135397=CARTESIAN_POINT('Ctrl Pts',(-5.4,4.19999999724801,-7.01751858720111)) ;
#135398=CARTESIAN_POINT('Ctrl Pts',(-5.4,4.23801992976516,-7.03250687190974)) ;
#135399=CARTESIAN_POINT('Ctrl Pts',(-5.37474093186837,4.17158354835192,
-6.98)) ;
#135400=CARTESIAN_POINT('Ctrl Pts',(-5.4,4.2,-6.98)) ;
#135401=CARTESIAN_POINT('Ctrl Pts',(-5.4,4.23801993223491,-6.98)) ;
#135402=CARTESIAN_POINT('Origin',(-5.3,3.9369800677651,-7.18)) ;
#135403=CARTESIAN_POINT('Ctrl Pts',(-5.37474093186837,4.17158354835192,
-6.98)) ;
#135404=CARTESIAN_POINT('Ctrl Pts',(-5.37474093064202,4.17158354697228,
-7.00625343593896)) ;
#135405=CARTESIAN_POINT('Ctrl Pts',(-5.36668583490654,4.14629949399953,
-7.03219871311588)) ;
#135406=CARTESIAN_POINT('Ctrl Pts',(-5.3390138046061,4.05944006555648,-7.06922264312143)) ;
#135407=CARTESIAN_POINT('Ctrl Pts',(-5.31962206268973,3.99857154231911,
-7.08)) ;
#135408=CARTESIAN_POINT('Ctrl Pts',(-5.3,3.9369800677651,-7.08)) ;
#135409=CARTESIAN_POINT('Ctrl Pts',(-3.42983432543734,1.98356361611701,
-6.69706297559117)) ;
#135410=CARTESIAN_POINT('Ctrl Pts',(-3.42093333711585,1.97355000425533,
-6.7795614824061)) ;
#135411=CARTESIAN_POINT('Ctrl Pts',(-3.48082994825801,1.91712723223402,
-6.79420287624085)) ;
#135412=CARTESIAN_POINT('Ctrl Pts',(-3.41101314049054,1.96238978305186,
-6.68786150708384)) ;
#135413=CARTESIAN_POINT('Ctrl Pts',(-3.3953888186174,1.95068928167321,-6.77331726677318)) ;
#135414=CARTESIAN_POINT('Ctrl Pts',(-3.44316973238528,1.87475949194143,
-6.78499704569418)) ;
#135415=CARTESIAN_POINT('Ctrl Pts',(-3.38343213690421,1.95,-6.67437746119715)) ;
#135416=CARTESIAN_POINT('Ctrl Pts',(-3.36046743872472,1.94345445676975,
-6.76478092946601)) ;
#135417=CARTESIAN_POINT('Ctrl Pts',(-3.38803897426452,1.85000000162387,
-6.77152063815355)) ;
#135418=CARTESIAN_POINT('Ctrl Pts',(-3.35509339356897,1.95,-6.66052296445552)) ;
#135419=CARTESIAN_POINT('Ctrl Pts',(-3.33134808452127,1.95,-6.7576628651052)) ;
#135420=CARTESIAN_POINT('Ctrl Pts',(-3.33134808452128,1.85,-6.7576628651052)) ;
#135421=CARTESIAN_POINT('Origin',(-3.50457525730571,1.91712723223402,-6.69706297559117)) ;
#135422=CARTESIAN_POINT('Origin',(-4.66204490261456,1.95,-3.18)) ;
#135423=CARTESIAN_POINT('Origin',(-4.66204490261456,-1.5692190524323,-3.18)) ;
#135424=CARTESIAN_POINT('Origin',(-3.84472135955,-1.16055728090002,-3.18)) ;
#135425=CARTESIAN_POINT('Origin',(-4.66204490261456,-1.5692190524323,-3.18)) ;
#135426=CARTESIAN_POINT('Origin',(-5.3,-2.11180339887499,-2.54)) ;
#135427=CARTESIAN_POINT('Origin',(-5.3,-2.11180339887499,-6.98)) ;
#135428=CARTESIAN_POINT('Origin',(-5.3,1.95,-7.18)) ;
#135429=CARTESIAN_POINT('Origin',(-5.3,-1.88819660112501,-7.18)) ;
#135430=CARTESIAN_POINT('Origin',(-4.0264650697994,2.50425327128942,-6.98)) ;
#135431=CARTESIAN_POINT('Origin',(-4.66204490261456,3.21928058320648,-6.98)) ;
#135432=CARTESIAN_POINT('Origin',(-3.02790825149799,1.38087685070033,-6.5805443741715)) ;
#135433=CARTESIAN_POINT('Origin',(-4.66204490261456,3.21928058320648,-6.98)) ;
#135434=CARTESIAN_POINT('Origin',(-4.66204490261456,-1.5692190524323,-3.18)) ;
#135435=CARTESIAN_POINT('Origin',(-4.66204490261456,-1.5692190524323,-3.18)) ;
#135436=CARTESIAN_POINT('Ctrl Pts',(-5.34460423617422,-2.02230212313483,
-6.97987524812987)) ;
#135437=CARTESIAN_POINT('Ctrl Pts',(-5.4,-2.04990938338631,-6.97983624572347)) ;
#135438=CARTESIAN_POINT('Ctrl Pts',(-5.4,-2.11180321723903,-6.97975033111957)) ;
#135439=CARTESIAN_POINT('Ctrl Pts',(-5.34461954754097,-2.02234798681676,
-7.00615385528167)) ;
#135440=CARTESIAN_POINT('Ctrl Pts',(-5.4,-2.04997459329993,-7.01432433515999)) ;
#135441=CARTESIAN_POINT('Ctrl Pts',(-5.4,-2.1118797455067,-7.03234231302605)) ;
#135442=CARTESIAN_POINT('Ctrl Pts',(-5.33978950165958,-2.00789652656155,
-7.03213503498038)) ;
#135443=CARTESIAN_POINT('Ctrl Pts',(-5.4,-2.02908601268746,-7.04863348546835)) ;
#135444=CARTESIAN_POINT('Ctrl Pts',(-5.4,-2.08777005652399,-7.08433878736396)) ;
#135445=CARTESIAN_POINT('Ctrl Pts',(-5.32318090226693,-1.9581752705225,
-7.06921550273187)) ;
#135446=CARTESIAN_POINT('Ctrl Pts',(-5.4,-1.9652731017248,-7.08783661624714)) ;
#135447=CARTESIAN_POINT('Ctrl Pts',(-5.4,-2.00485091174287,-7.15850392511066)) ;
#135448=CARTESIAN_POINT('Ctrl Pts',(-5.31153957531165,-1.92331224822997,
-7.08001353231107)) ;
#135449=CARTESIAN_POINT('Ctrl Pts',(-5.39999999999998,-1.92148676945294,
-7.091022107462)) ;
#135450=CARTESIAN_POINT('Ctrl Pts',(-5.4,-1.94671708614657,-7.18006828697155)) ;
#135451=CARTESIAN_POINT('Ctrl Pts',(-5.29976814257747,-1.88802911972918,
-7.08000017262218)) ;
#135452=CARTESIAN_POINT('Ctrl Pts',(-5.4,-1.88802831720456,-7.07976740645702)) ;
#135453=CARTESIAN_POINT('Ctrl Pts',(-5.4,-1.88791746283072,-7.17999983753763)) ;
#135454=CARTESIAN_POINT('Origin',(-5.30000000000007,-1.88819660112522,-6.98000000000015)) ;
#135455=CARTESIAN_POINT('Origin',(-4.66204490261456,3.21928058320648,-6.98)) ;
#135456=CARTESIAN_POINT('Origin',(-4.66204490261456,3.21928058320648,-6.98)) ;
#135457=CARTESIAN_POINT('Origin',(0.175392621986784,-0.95,-4.36248472823589)) ;
#135458=CARTESIAN_POINT('Origin',(-3.37639320225,-0.95,-3.49427041564467)) ;
#135459=CARTESIAN_POINT('Origin',(-3.32804538583365,-0.902219294041845,
-3.50608877076867)) ;
#135460=CARTESIAN_POINT('Origin',(-3.46583592134999,-0.971114561800017,
-3.47240663986467)) ;
#135461=CARTESIAN_POINT('Origin',(-3.24472135955,-0.860557280900019,-6.98)) ;
#135462=CARTESIAN_POINT('Origin',(-4.66204490261456,-1.5692190524323,-6.98)) ;
#135463=CARTESIAN_POINT('Origin',(-4.66204490261456,1.95,-6.98)) ;
#135464=CARTESIAN_POINT('Origin',(-4.66204490261456,-1.5692190524323,-6.98)) ;
#135465=CARTESIAN_POINT('Ctrl Pts',(-3.4211145618,-1.06055728090001,-3.47240663986467)) ;
#135466=CARTESIAN_POINT('Ctrl Pts',(-3.40394191641935,-1.05197095820969,
-3.38459197598638)) ;
#135467=CARTESIAN_POINT('Ctrl Pts',(-3.44209061230229,-0.971114561800017,
-3.37526673921499)) ;
#135468=CARTESIAN_POINT('Ctrl Pts',(-3.40727897628736,-1.05363948814369,
-3.47917070399162)) ;
#135469=CARTESIAN_POINT('Ctrl Pts',(-3.38665319245547,-1.04670310838587,
-3.38881810851091)) ;
#135470=CARTESIAN_POINT('Ctrl Pts',(-3.4144159452097,-0.957277229261617,
-3.38203165783763)) ;
#135471=CARTESIAN_POINT('Ctrl Pts',(-3.3918627446443,-1.05,-3.4867075282519)) ;
#135472=CARTESIAN_POINT('Ctrl Pts',(-3.36870744055525,-1.04639008266724,
-3.39320484786425)) ;
#135473=CARTESIAN_POINT('Ctrl Pts',(-3.38358960366098,-0.950000000886305,
-3.38956698577176)) ;
#135474=CARTESIAN_POINT('Ctrl Pts',(-3.37639320225,-1.05,-3.49427041564467)) ;
#135475=CARTESIAN_POINT('Ctrl Pts',(-3.3526478932023,-1.05,-3.39713051499499)) ;
#135476=CARTESIAN_POINT('Ctrl Pts',(-3.3526478932023,-0.95,-3.39713051499499)) ;
#135477=CARTESIAN_POINT('Origin',(-3.37639320224939,-1.15000000000261,-3.494270415645)) ;
#135478=CARTESIAN_POINT('Origin',(-4.66204490261456,-1.5692190524323,-6.98)) ;
#135479=CARTESIAN_POINT('Origin',(-4.66204490261456,-1.5692190524323,-6.98)) ;
#135480=CARTESIAN_POINT('Origin',(-3.37639320225,-1.15,-5.08)) ;
#135481=CARTESIAN_POINT('Origin',(-3.37639320224947,-1.15000000000223,-6.6657295843551)) ;
#135482=CARTESIAN_POINT('Origin',(-1.50751564693271,0.00804557540861825,
-6.2088928486111)) ;
#135483=CARTESIAN_POINT('Origin',(-3.46583592134999,-0.971114561800017,
-6.68759336013533)) ;
#135484=CARTESIAN_POINT('Ctrl Pts',(-3.37639320225,-1.05,-6.66572958435533)) ;
#135485=CARTESIAN_POINT('Ctrl Pts',(-3.3526478932023,-1.05,-6.76286948500501)) ;
#135486=CARTESIAN_POINT('Ctrl Pts',(-3.3526478932023,-0.95,-6.76286948500501)) ;
#135487=CARTESIAN_POINT('Ctrl Pts',(-3.39186274464432,-1.05,-6.67329247174809)) ;
#135488=CARTESIAN_POINT('Ctrl Pts',(-3.36870744055522,-1.04639008266724,
-6.76679515213572)) ;
#135489=CARTESIAN_POINT('Ctrl Pts',(-3.38358960366098,-0.950000000886305,
-6.77043301422824)) ;
#135490=CARTESIAN_POINT('Ctrl Pts',(-3.40727897628736,-1.05363948814369,
-6.68082929600838)) ;
#135491=CARTESIAN_POINT('Ctrl Pts',(-3.38665319245551,-1.04670310838583,
-6.7711818914891)) ;
#135492=CARTESIAN_POINT('Ctrl Pts',(-3.4144159452097,-0.957277229261612,
-6.77796834216237)) ;
#135493=CARTESIAN_POINT('Ctrl Pts',(-3.4211145618,-1.06055728090001,-6.68759336013533)) ;
#135494=CARTESIAN_POINT('Ctrl Pts',(-3.40394191641936,-1.05197095820969,
-6.77540802401362)) ;
#135495=CARTESIAN_POINT('Ctrl Pts',(-3.4420906123023,-0.971114561800017,
-6.78473326078501)) ;
#135496=CARTESIAN_POINT('Origin',(-3.37639320225,-0.95,-6.66572958435533)) ;
#135497=CARTESIAN_POINT('Origin',(0.175392621986784,-0.95,-5.79751527176412)) ;
#135498=CARTESIAN_POINT('Origin',(12.7,2.65,-2.54)) ;
#135499=CARTESIAN_POINT('Origin',(12.8,2.65,-6.57304604217164)) ;
#135500=CARTESIAN_POINT('',(4.57524318173533,2.73534903669982,-6.52093518020973)) ;
#135501=CARTESIAN_POINT('Origin',(4.65232986199931,2.66527023615902,-6.56875421118371)) ;
#135502=CARTESIAN_POINT('Ctrl Pts',(4.57524318173533,2.73534903669982,-6.52093518020973)) ;
#135503=CARTESIAN_POINT('Ctrl Pts',(4.5761458558036,2.73452842391049,-6.51959115118323)) ;
#135504=CARTESIAN_POINT('Ctrl Pts',(4.57705238626145,2.73367683201792,-6.51826812933933)) ;
#135505=CARTESIAN_POINT('Ctrl Pts',(4.5779495181309,2.73280244902547,-6.51697684888884)) ;
#135506=CARTESIAN_POINT('Ctrl Pts',(4.58144263576941,2.72939790755534,-6.51194905456846)) ;
#135507=CARTESIAN_POINT('Ctrl Pts',(4.58496694799996,2.72549786515169,-6.50716994451779)) ;
#135508=CARTESIAN_POINT('Ctrl Pts',(4.5881567005692,2.72107165565026,-6.50269819385252)) ;
#135509=CARTESIAN_POINT('Ctrl Pts',(4.59069123847483,2.7175546443724,-6.49914499612962)) ;
#135510=CARTESIAN_POINT('Ctrl Pts',(4.59301454561858,2.71370459823898,-6.49578631272419)) ;
#135511=CARTESIAN_POINT('Ctrl Pts',(4.5949431309995,2.70950205848694,-6.49267499616739)) ;
#135512=CARTESIAN_POINT('Ctrl Pts',(4.59651854606294,2.70606910472946,-6.49013343642149)) ;
#135513=CARTESIAN_POINT('Ctrl Pts',(4.59783685868319,2.70233705077427,-6.48771608615717)) ;
#135514=CARTESIAN_POINT('Ctrl Pts',(4.59873118971422,2.69838744820002,-6.48553230121235)) ;
#135515=CARTESIAN_POINT('Ctrl Pts',(4.59916508318198,2.6964712597891,-6.48447281653647)) ;
#135516=CARTESIAN_POINT('Ctrl Pts',(4.59949917984822,2.69450444432188,-6.48346779888203)) ;
#135517=CARTESIAN_POINT('Ctrl Pts',(4.5997144226265,2.69249922659198,-6.48252634409943)) ;
#135518=CARTESIAN_POINT('Ctrl Pts',(4.59990113259977,2.6907598225955,-6.48170968953523)) ;
#135519=CARTESIAN_POINT('Ctrl Pts',(4.6,2.68896788689974,-6.48093031221453)) ;
#135520=CARTESIAN_POINT('Ctrl Pts',(4.6,2.68715716172261,-6.48020561276333)) ;
#135521=CARTESIAN_POINT('Origin',(4.5,2.1,-6.46195395782836)) ;
#135522=CARTESIAN_POINT('Origin',(4.6,2.1,-6.46195395782836)) ;
#135523=CARTESIAN_POINT('Origin',(12.7,2.1,-6.46195395782836)) ;
#135524=CARTESIAN_POINT('Origin',(12.7,2.76643989873054,-6.55363939238321)) ;
#135525=CARTESIAN_POINT('Origin',(12.7,2.13287979746107,-6.65923274259479)) ;
#135526=CARTESIAN_POINT('Origin',(4.4,2.72431432344521,-5.08)) ;
#135527=CARTESIAN_POINT('Ctrl Pts',(4.48762159086959,2.77250619842349,-3.69117568174948)) ;
#135528=CARTESIAN_POINT('Ctrl Pts',(4.48806820038223,2.77169418112776,-3.69383556708983)) ;
#135529=CARTESIAN_POINT('Ctrl Pts',(4.48852084821546,2.77084293101113,-3.69648271501847)) ;
#135530=CARTESIAN_POINT('Ctrl Pts',(4.49012932137855,2.76769877392855,-3.70576300952075)) ;
#135531=CARTESIAN_POINT('Ctrl Pts',(4.49131046584975,2.76517764467227,-3.71234413170349)) ;
#135532=CARTESIAN_POINT('Ctrl Pts',(4.49351977821778,2.75978760391028,-3.72463528016215)) ;
#135533=CARTESIAN_POINT('Ctrl Pts',(4.49455195297829,2.7569765375012,-3.73036774060142)) ;
#135534=CARTESIAN_POINT('Ctrl Pts',(4.49620670090467,2.75163165728869,-3.73994332160334)) ;
#135535=CARTESIAN_POINT('Ctrl Pts',(4.49686252944493,2.74924176842721,-3.74386402620338)) ;
#135536=CARTESIAN_POINT('Ctrl Pts',(4.49822764032851,2.74331716058949,-3.75264463163475)) ;
#135537=CARTESIAN_POINT('Ctrl Pts',(4.49890203357906,2.73961076902702,-3.75748650016056)) ;
#135538=CARTESIAN_POINT('Ctrl Pts',(4.49975897856022,2.73206576252675,-3.7658277784398)) ;
#135539=CARTESIAN_POINT('Ctrl Pts',(4.5,2.72833175948613,-3.76941900229181)) ;
#135540=CARTESIAN_POINT('Ctrl Pts',(4.5,2.72431432344521,-3.77263481664499)) ;
#135541=CARTESIAN_POINT('Ctrl Pts',(4.5,2.72431432344521,-6.38736518335501)) ;
#135542=CARTESIAN_POINT('Ctrl Pts',(4.5,2.7290466915143,-6.39115327531367)) ;
#135543=CARTESIAN_POINT('Ctrl Pts',(4.49966645684473,2.73338556955559,-6.39546141017606)) ;
#135544=CARTESIAN_POINT('Ctrl Pts',(4.49869539480393,2.74072289096378,-6.40398024143747)) ;
#135545=CARTESIAN_POINT('Ctrl Pts',(4.49811062025687,2.74382502998085,-6.40810805965865)) ;
#135546=CARTESIAN_POINT('Ctrl Pts',(4.49664125196625,2.75020211699687,-6.41755926494058)) ;
#135547=CARTESIAN_POINT('Ctrl Pts',(4.49570721389711,2.75339870015141,-6.42301039031934)) ;
#135548=CARTESIAN_POINT('Ctrl Pts',(4.49363760641477,2.75952863263949,-6.43475170518696)) ;
#135549=CARTESIAN_POINT('Ctrl Pts',(4.49249077386342,2.76240287369074,-6.44107122583083)) ;
#135550=CARTESIAN_POINT('Ctrl Pts',(4.49055019898872,2.76677757270139,-6.45191412562089)) ;
#135551=CARTESIAN_POINT('Ctrl Pts',(4.48975662823143,2.76842729450635,-6.45638729192264)) ;
#135552=CARTESIAN_POINT('Ctrl Pts',(4.4885208482156,2.77084293101086,-6.46351728498073)) ;
#135553=CARTESIAN_POINT('Ctrl Pts',(4.48806820038252,2.77169418112725,-6.46616443290854)) ;
#135554=CARTESIAN_POINT('Ctrl Pts',(4.48762159086959,2.77250619842348,-6.46882431824782)) ;
#135555=CARTESIAN_POINT('Origin',(4.6,2.1,-5.08)) ;
#135556=CARTESIAN_POINT('Origin',(4.6,2.1,-3.69804604217164)) ;
#135557=CARTESIAN_POINT('Origin',(4.6,2.1,-6.46195395782836)) ;
#135558=CARTESIAN_POINT('Origin',(12.7,2.1,-6.46195395782836)) ;
#135559=CARTESIAN_POINT('Origin',(12.7,1.9,-6.46195395782836)) ;
#135560=CARTESIAN_POINT('Origin',(4.5,2.65,-3.58695395782836)) ;
#135561=CARTESIAN_POINT('',(4.6,2.68715716172261,-3.67979438723668)) ;
#135562=CARTESIAN_POINT('',(4.57524318173443,2.73534903670064,-3.63906481978892)) ;
#135563=CARTESIAN_POINT('Ctrl Pts',(4.6,2.68715716172261,-3.67979438723667)) ;
#135564=CARTESIAN_POINT('Ctrl Pts',(4.6,2.69106036671413,-3.67823222277847)) ;
#135565=CARTESIAN_POINT('Ctrl Pts',(4.59952510519173,2.69488861888989,-3.67640970947469)) ;
#135566=CARTESIAN_POINT('Ctrl Pts',(4.59869497748254,2.69852743640772,-3.674390151225)) ;
#135567=CARTESIAN_POINT('Ctrl Pts',(4.59815316003464,2.70090246232129,-3.67307200236113)) ;
#135568=CARTESIAN_POINT('Ctrl Pts',(4.59746001108778,2.70319720658047,-3.6716709680452)) ;
#135569=CARTESIAN_POINT('Ctrl Pts',(4.59664880273703,2.70538659711789,-3.6702145418985)) ;
#135570=CARTESIAN_POINT('Ctrl Pts',(4.59612777291939,2.70679281754376,-3.66927909609234)) ;
#135571=CARTESIAN_POINT('Ctrl Pts',(4.59555051815356,2.70817855133085,-3.66830492990722)) ;
#135572=CARTESIAN_POINT('Ctrl Pts',(4.59494172533681,2.70950512149367,-3.66732273606981)) ;
#135573=CARTESIAN_POINT('Ctrl Pts',(4.59250947890861,2.71480502887016,-3.66339867949904)) ;
#135574=CARTESIAN_POINT('Ctrl Pts',(4.5894485781299,2.71954517005253,-3.65908233758082)) ;
#135575=CARTESIAN_POINT('Ctrl Pts',(4.58612768646811,2.7237636121892,-3.65447380318364)) ;
#135576=CARTESIAN_POINT('Ctrl Pts',(4.58350334758173,2.7270972414872,-3.65083190297747)) ;
#135577=CARTESIAN_POINT('Ctrl Pts',(4.58071664514661,2.73010548898776,-3.6470059959315)) ;
#135578=CARTESIAN_POINT('Ctrl Pts',(4.5779495181309,2.73280244902547,-3.64302315111117)) ;
#135579=CARTESIAN_POINT('Ctrl Pts',(4.57705238626115,2.73367683201821,-3.64173187066025)) ;
#135580=CARTESIAN_POINT('Ctrl Pts',(4.576145855803,2.73452842391106,-3.64040884881589)) ;
#135581=CARTESIAN_POINT('Ctrl Pts',(4.57524318173443,2.73534903670064,-3.63906481978892)) ;
#135582=CARTESIAN_POINT('Origin',(4.65232986200049,2.66527023615798,-3.5912457888159)) ;
#135583=CARTESIAN_POINT('Origin',(4.6,2.65,-3.58695395782836)) ;
#135584=CARTESIAN_POINT('Origin',(12.7,1.9,-6.58)) ;
#135585=CARTESIAN_POINT('Origin',(12.7,2.01643989873054,-3.48136060761679)) ;
#135586=CARTESIAN_POINT('Origin',(-3.65,10.7,-4.33)) ;
#135587=CARTESIAN_POINT('Origin',(-3.65,10.7,-4.33)) ;
#135588=CARTESIAN_POINT('Origin',(-3.65,10.7,-4.33)) ;
#135589=CARTESIAN_POINT('Origin',(0.,10.7,-4.33)) ;
#135590=CARTESIAN_POINT('Origin',(-2.9,10.7,-4.33)) ;
#135591=CARTESIAN_POINT('Origin',(-3.65,10.7,-5.08)) ;
#135592=CARTESIAN_POINT('Origin',(-3.65,10.7,-5.83)) ;
#135593=CARTESIAN_POINT('Origin',(-2.9,10.7,-4.33)) ;
#135594=CARTESIAN_POINT('Origin',(-2.9,10.7,-4.33)) ;
#135595=CARTESIAN_POINT('Origin',(-3.65,10.7,-5.83)) ;
#135596=CARTESIAN_POINT('Origin',(-3.65,10.7,-5.83)) ;
#135597=CARTESIAN_POINT('Origin',(-2.9,10.7,-5.08)) ;
#135598=CARTESIAN_POINT('Origin',(-2.9,10.7,-5.83)) ;
#135599=CARTESIAN_POINT('Origin',(0.,10.7,-5.83)) ;
#135600=CARTESIAN_POINT('Origin',(-2.9,10.7,-5.83)) ;
#135601=CARTESIAN_POINT('Origin',(-2.9,10.7,-5.83)) ;
#135602=CARTESIAN_POINT('Origin',(-3.05,-3.95,-4.08)) ;
#135603=CARTESIAN_POINT('Origin',(-3.05,-3.95,-5.98)) ;
#135604=CARTESIAN_POINT('Origin',(-3.05,-3.95,-4.18)) ;
#135605=CARTESIAN_POINT('Origin',(-3.25,-3.95,-4.18)) ;
#135606=CARTESIAN_POINT('Origin',(-3.25,-3.95,-3.98)) ;
#135607=CARTESIAN_POINT('Origin',(-3.25,-3.95,-4.18)) ;
#135608=CARTESIAN_POINT('Origin',(-3.25,-3.95,-5.98)) ;
#135609=CARTESIAN_POINT('Origin',(-3.25,-3.95,-5.98)) ;
#135610=CARTESIAN_POINT('Origin',(-3.25,-3.95,-6.18)) ;
#135611=CARTESIAN_POINT('Origin',(-4.4,-3.95,-3.98)) ;
#135612=CARTESIAN_POINT('Origin',(-4.3,-3.95,-3.98)) ;
#135613=CARTESIAN_POINT('Origin',(-3.25,-3.9,-4.18)) ;
#135614=CARTESIAN_POINT('Origin',(-3.25,-3.85,-4.18)) ;
#135615=CARTESIAN_POINT('Origin',(-3.25,-3.85,-5.08)) ;
#135616=CARTESIAN_POINT('Origin',(-3.25,-3.85,-5.98)) ;
#135617=CARTESIAN_POINT('Origin',(-3.25,-3.85,-4.18)) ;
#135618=CARTESIAN_POINT('Origin',(-3.25,-3.9,-5.98)) ;
#135619=CARTESIAN_POINT('Origin',(-3.25,-3.85,-5.98)) ;
#135620=CARTESIAN_POINT('Origin',(-4.4,-3.95,-6.18)) ;
#135621=CARTESIAN_POINT('Origin',(-4.3,-3.95,-6.18)) ;
#135622=CARTESIAN_POINT('Origin',(-4.5,-3.95,-4.08)) ;
#135623=CARTESIAN_POINT('Origin',(-4.5,-3.95,-4.18)) ;
#135624=CARTESIAN_POINT('Origin',(-4.5,-3.95,-5.98)) ;
#135625=CARTESIAN_POINT('Origin',(-4.3,-3.95,-4.18)) ;
#135626=CARTESIAN_POINT('Origin',(-4.3,-3.95,-4.18)) ;
#135627=CARTESIAN_POINT('Origin',(-3.25,-3.85,-4.18)) ;
#135628=CARTESIAN_POINT('Origin',(-3.25,-3.85,-4.18)) ;
#135629=CARTESIAN_POINT('Origin',(-3.25,-3.85,-5.98)) ;
#135630=CARTESIAN_POINT('Origin',(-3.25,-3.85,-5.98)) ;
#135631=CARTESIAN_POINT('Origin',(-4.3,-3.95,-5.98)) ;
#135632=CARTESIAN_POINT('Origin',(-4.3,-3.95,-5.98)) ;
#135633=CARTESIAN_POINT('Origin',(-4.3,-3.9,-4.18)) ;
#135634=CARTESIAN_POINT('Origin',(-4.3,-3.85,-4.18)) ;
#135635=CARTESIAN_POINT('Origin',(-1.56125112837913E-16,-3.85,-4.18)) ;
#135636=CARTESIAN_POINT('Origin',(-4.3,-3.85,-4.18)) ;
#135637=CARTESIAN_POINT('Origin',(-1.56125112837913E-16,-3.85,-5.98)) ;
#135638=CARTESIAN_POINT('Origin',(-4.3,-3.85,-5.98)) ;
#135639=CARTESIAN_POINT('Origin',(-4.3,-3.9,-5.98)) ;
#135640=CARTESIAN_POINT('Origin',(-4.3,-3.85,-5.98)) ;
#135641=CARTESIAN_POINT('Origin',(-4.3,-3.85,-4.18)) ;
#135642=CARTESIAN_POINT('Origin',(-4.3,-3.85,-4.18)) ;
#135643=CARTESIAN_POINT('Origin',(-4.3,-3.85,-5.98)) ;
#135644=CARTESIAN_POINT('Origin',(-4.3,-3.85,-5.98)) ;
#135645=CARTESIAN_POINT('Origin',(-4.3,-3.85,-5.08)) ;
#135646=CARTESIAN_POINT('Origin',(-4.,10.85,-6.08)) ;
#135647=CARTESIAN_POINT('Origin',(-4.,10.85,-5.98)) ;
#135648=CARTESIAN_POINT('Origin',(-4.,10.85,-4.18)) ;
#135649=CARTESIAN_POINT('Origin',(-3.8,10.85,-4.18)) ;
#135650=CARTESIAN_POINT('Origin',(-3.8,10.85,-3.98)) ;
#135651=CARTESIAN_POINT('Origin',(-3.8,10.85,-4.18)) ;
#135652=CARTESIAN_POINT('Origin',(-3.8,10.85,-5.98)) ;
#135653=CARTESIAN_POINT('Origin',(-3.8,10.85,-5.98)) ;
#135654=CARTESIAN_POINT('Origin',(-3.8,10.85,-6.18)) ;
#135655=CARTESIAN_POINT('Origin',(-3.9,10.85,-3.98)) ;
#135656=CARTESIAN_POINT('Origin',(-2.75,10.85,-3.98)) ;
#135657=CARTESIAN_POINT('Origin',(-3.8,10.8,-4.18)) ;
#135658=CARTESIAN_POINT('Origin',(-3.8,10.75,-4.18)) ;
#135659=CARTESIAN_POINT('Origin',(-3.8,10.75,-5.08)) ;
#135660=CARTESIAN_POINT('Origin',(-3.8,10.75,-5.98)) ;
#135661=CARTESIAN_POINT('Origin',(-3.8,10.75,-4.18)) ;
#135662=CARTESIAN_POINT('Origin',(-3.8,10.8,-5.98)) ;
#135663=CARTESIAN_POINT('Origin',(-3.8,10.75,-5.98)) ;
#135664=CARTESIAN_POINT('Origin',(-3.9,10.85,-6.18)) ;
#135665=CARTESIAN_POINT('Origin',(-2.75,10.85,-6.18)) ;
#135666=CARTESIAN_POINT('Origin',(-2.55,10.85,-6.08)) ;
#135667=CARTESIAN_POINT('Origin',(-2.55,10.85,-4.18)) ;
#135668=CARTESIAN_POINT('Origin',(-2.55,10.85,-5.98)) ;
#135669=CARTESIAN_POINT('Origin',(-2.75,10.85,-4.18)) ;
#135670=CARTESIAN_POINT('Origin',(-2.75,10.85,-4.18)) ;
#135671=CARTESIAN_POINT('Origin',(-3.8,10.75,-4.18)) ;
#135672=CARTESIAN_POINT('Origin',(-3.8,10.75,-4.18)) ;
#135673=CARTESIAN_POINT('Origin',(-3.8,10.75,-5.98)) ;
#135674=CARTESIAN_POINT('Origin',(-3.8,10.75,-5.98)) ;
#135675=CARTESIAN_POINT('Origin',(-2.75,10.85,-5.98)) ;
#135676=CARTESIAN_POINT('Origin',(-2.75,10.85,-5.98)) ;
#135677=CARTESIAN_POINT('Origin',(-2.75,10.8,-4.18)) ;
#135678=CARTESIAN_POINT('Origin',(-2.75,10.75,-4.18)) ;
#135679=CARTESIAN_POINT('Origin',(1.56125112837912E-16,10.75,-4.18)) ;
#135680=CARTESIAN_POINT('Origin',(-2.75,10.75,-4.18)) ;
#135681=CARTESIAN_POINT('Origin',(-1.56125112837913E-16,10.75,-5.98)) ;
#135682=CARTESIAN_POINT('Origin',(-2.75,10.75,-5.98)) ;
#135683=CARTESIAN_POINT('Origin',(-2.75,10.8,-5.98)) ;
#135684=CARTESIAN_POINT('Origin',(-2.75,10.75,-5.98)) ;
#135685=CARTESIAN_POINT('Origin',(-2.75,10.75,-4.18)) ;
#135686=CARTESIAN_POINT('Origin',(-2.75,10.75,-4.18)) ;
#135687=CARTESIAN_POINT('Origin',(-2.75,10.75,-5.98)) ;
#135688=CARTESIAN_POINT('Origin',(-2.75,10.75,-5.98)) ;
#135689=CARTESIAN_POINT('Origin',(-2.75,10.75,-5.08)) ;
#135690=CARTESIAN_POINT('Origin',(4.6,0.,-5.08)) ;
#135691=CARTESIAN_POINT('Ctrl Pts',(4.5,-2.7,-3.55684537882722)) ;
#135692=CARTESIAN_POINT('Ctrl Pts',(4.5,-2.71827986285823,-3.63196473917507)) ;
#135693=CARTESIAN_POINT('Ctrl Pts',(4.50597963419107,-2.73556801027185,
-3.70673986045281)) ;
#135694=CARTESIAN_POINT('Ctrl Pts',(4.52394923367545,-2.75977758633329,
-3.81843683402156)) ;
#135695=CARTESIAN_POINT('Ctrl Pts',(4.53141024883993,-2.76757607569523,
-3.85568328239029)) ;
#135696=CARTESIAN_POINT('Ctrl Pts',(4.54734065524866,-2.77857284247615,
-3.91016568958296)) ;
#135697=CARTESIAN_POINT('Ctrl Pts',(4.55339248498575,-2.78214991573955,
-3.92823827441494)) ;
#135698=CARTESIAN_POINT('Ctrl Pts',(4.56567492147095,-2.787183259287,-3.95414672186072)) ;
#135699=CARTESIAN_POINT('Ctrl Pts',(4.5702469143305,-2.78880341224557,-3.96257260505082)) ;
#135700=CARTESIAN_POINT('Ctrl Pts',(4.58215938980081,-2.79169669265294,
-3.97774347988509)) ;
#135701=CARTESIAN_POINT('Ctrl Pts',(4.59005470866978,-2.79310344827587,
-3.98520635404226)) ;
#135702=CARTESIAN_POINT('Ctrl Pts',(4.6,-2.79310344827586,-3.98520635404223)) ;
#135703=CARTESIAN_POINT('Origin',(4.6,-2.4,-3.11785831296514)) ;
#135704=CARTESIAN_POINT('Origin',(4.6,-2.4,-3.11785831296514)) ;
#135705=CARTESIAN_POINT('Origin',(4.6,-2.4,-3.11785831296514)) ;
#135706=CARTESIAN_POINT('Origin',(0.584645609909622,-2.4,-3.11785831296514)) ;
#135707=CARTESIAN_POINT('Origin',(12.7,-2.4,-3.11785831296514)) ;
#135708=CARTESIAN_POINT('Origin',(12.7,-2.4,-3.11785831296514)) ;
#135709=CARTESIAN_POINT('Origin',(12.7,-2.24516129032258,-3.24444809922546)) ;
#135710=CARTESIAN_POINT('Origin',(12.7,0.,-5.08)) ;
#135711=CARTESIAN_POINT('Origin',(12.7,-2.24516129032258,-6.91555190077455)) ;
#135712=CARTESIAN_POINT('Origin',(12.7,-2.2,-2.54)) ;
#135713=CARTESIAN_POINT('Origin',(12.7,-2.2,-7.04214168703486)) ;
#135714=CARTESIAN_POINT('Origin',(12.7,-2.4,-7.04214168703486)) ;
#135715=CARTESIAN_POINT('Origin',(12.7,-2.4,-7.04214168703486)) ;
#135716=CARTESIAN_POINT('Origin',(0.584645609909622,-2.4,-7.04214168703486)) ;
#135717=CARTESIAN_POINT('Origin',(4.6,-2.4,-7.04214168703486)) ;
#135718=CARTESIAN_POINT('Origin',(4.6,-2.4,-2.54)) ;
#135719=CARTESIAN_POINT('Origin',(4.6,-2.4,-7.04214168703486)) ;
#135720=CARTESIAN_POINT('Origin',(4.6,-2.4,-7.04214168703486)) ;
#135721=CARTESIAN_POINT('Origin',(4.6,-2.4,-7.04214168703486)) ;
#135722=CARTESIAN_POINT('Origin',(4.6,0.,-5.08)) ;
#135723=CARTESIAN_POINT('Ctrl Pts',(4.6,-2.79310344827586,-6.17479364595777)) ;
#135724=CARTESIAN_POINT('Ctrl Pts',(4.59007568892311,-2.79310344827586,
-6.17479364595777)) ;
#135725=CARTESIAN_POINT('Ctrl Pts',(4.5821920763724,-2.79170232102182,-6.18222674227604)) ;
#135726=CARTESIAN_POINT('Ctrl Pts',(4.57028631514659,-2.78881527838255,
-6.19736543899001)) ;
#135727=CARTESIAN_POINT('Ctrl Pts',(4.56571532154372,-2.78719767797524,
-6.20577848858353)) ;
#135728=CARTESIAN_POINT('Ctrl Pts',(4.55343865632726,-2.78217307830036,
-6.23164363330887)) ;
#135729=CARTESIAN_POINT('Ctrl Pts',(4.54738888873344,-2.77860151743012,
-6.24969008596606)) ;
#135730=CARTESIAN_POINT('Ctrl Pts',(4.53146440752601,-2.76762263748299,
-6.3040903156831)) ;
#135731=CARTESIAN_POINT('Ctrl Pts',(4.52400917967609,-2.75984503873828,
-6.34124550630579)) ;
#135732=CARTESIAN_POINT('Ctrl Pts',(4.50599905604505,-2.7356206423885,-6.45303013546926)) ;
#135733=CARTESIAN_POINT('Ctrl Pts',(4.5,-2.71826422026483,-6.5280995425769)) ;
#135734=CARTESIAN_POINT('Ctrl Pts',(4.5,-2.7,-6.60315462117279)) ;
#135735=CARTESIAN_POINT('Origin',(-0.362523114814661,9.05,-5.24904730469628)) ;
#135736=CARTESIAN_POINT('Origin',(0.36252311481466,9.05,-4.91095269530372)) ;
#135737=CARTESIAN_POINT('Origin',(-1.31845674202095,9.85,-3.67228134223507)) ;
#135738=CARTESIAN_POINT('Origin',(-0.230887397576972,9.85,-3.16513942814623)) ;
#135739=CARTESIAN_POINT('Origin',(4.6,2.1,-3.69804604217164)) ;
#135740=CARTESIAN_POINT('Origin',(4.6,2.1,-3.69804604217164)) ;
#135741=CARTESIAN_POINT('Origin',(4.6,0.280857398566761,-3.39485560859943)) ;
#135742=CARTESIAN_POINT('Origin',(4.6,2.61712020253893,-3.78423274259479)) ;
#135743=CARTESIAN_POINT('Origin',(4.6,2.65,-3.58695395782836)) ;
#135744=CARTESIAN_POINT('Origin',(4.6,2.72431432344521,-3.77263481664499)) ;
#135745=CARTESIAN_POINT('Ctrl Pts',(4.48762159086906,2.77250619842445,-3.69117568174961)) ;
#135746=CARTESIAN_POINT('Ctrl Pts',(4.51316716229105,2.72605970493114,-3.65423879419716)) ;
#135747=CARTESIAN_POINT('Ctrl Pts',(4.57527453405851,2.73535372386122,-3.63905715319801)) ;
#135748=CARTESIAN_POINT('Ctrl Pts',(4.49363662433156,2.76156977394745,-3.72699959247169)) ;
#135749=CARTESIAN_POINT('Ctrl Pts',(4.5146945995807,2.70766535161869,-3.67620084739329)) ;
#135750=CARTESIAN_POINT('Ctrl Pts',(4.58732693581885,2.72440392220678,-3.65699504123406)) ;
#135751=CARTESIAN_POINT('Ctrl Pts',(4.5,2.7448843843803,-3.75616921606616)) ;
#135752=CARTESIAN_POINT('Ctrl Pts',(4.50856472873626,2.6903148207967,-3.67849111370471)) ;
#135753=CARTESIAN_POINT('Ctrl Pts',(4.60003980620507,2.70775073269832,-3.67155231137473)) ;
#135754=CARTESIAN_POINT('Ctrl Pts',(4.5,2.72431432344521,-3.77263481664499)) ;
#135755=CARTESIAN_POINT('Ctrl Pts',(4.5,2.68714136424467,-3.6797549158517)) ;
#135756=CARTESIAN_POINT('Ctrl Pts',(4.60004250625998,2.68715716507935,-3.6797943956238)) ;
#135757=CARTESIAN_POINT('Origin',(4.57524318173443,2.82069807340128,-3.69117568174948)) ;
#135758=CARTESIAN_POINT('Ctrl Pts',(4.47150553123747,2.80180812502279,-3.58695395782836)) ;
#135759=CARTESIAN_POINT('Ctrl Pts',(4.5,2.75,-3.58695395782836)) ;
#135760=CARTESIAN_POINT('Ctrl Pts',(4.55912712210514,2.75,-3.58695395782836)) ;
#135761=CARTESIAN_POINT('Ctrl Pts',(4.47150553186688,2.8018081238784,-3.62357447273468)) ;
#135762=CARTESIAN_POINT('Ctrl Pts',(4.50000000073523,2.74999999866316,-3.61125808426874)) ;
#135763=CARTESIAN_POINT('Ctrl Pts',(4.5591271227348,2.75,-3.60527204575928)) ;
#135764=CARTESIAN_POINT('Ctrl Pts',(4.47712448971608,2.79159183687985,-3.65991653735233)) ;
#135765=CARTESIAN_POINT('Ctrl Pts',(4.50480340096852,2.74126654369363,-3.63553795099809)) ;
#135766=CARTESIAN_POINT('Ctrl Pts',(4.56473907811158,2.74489822224645,-3.62342482158227)) ;
#135767=CARTESIAN_POINT('Ctrl Pts',(4.48762159086676,2.77250619842407,-3.69117568174948)) ;
#135768=CARTESIAN_POINT('Ctrl Pts',(4.51315802400618,2.72607631998876,-3.6542520074343)) ;
#135769=CARTESIAN_POINT('Ctrl Pts',(4.57524318173443,2.73534903670064,-3.63906481978892)) ;
#135770=CARTESIAN_POINT('Origin',(4.55912712210514,2.85,-2.54)) ;
#135771=CARTESIAN_POINT('Origin',(4.55912712210514,2.85,-6.57304604217164)) ;
#135772=CARTESIAN_POINT('Ctrl Pts',(4.48762159086767,2.77250619842243,-6.46882431824783)) ;
#135773=CARTESIAN_POINT('Ctrl Pts',(4.51315802400691,2.72607631998743,-6.50574799256407)) ;
#135774=CARTESIAN_POINT('Ctrl Pts',(4.57524318173533,2.73534903669982,-6.52093518020973)) ;
#135775=CARTESIAN_POINT('Ctrl Pts',(4.47712448971641,2.79159183687925,-6.50008346264559)) ;
#135776=CARTESIAN_POINT('Ctrl Pts',(4.50480340096881,2.74126654369309,-6.52446204900054)) ;
#135777=CARTESIAN_POINT('Ctrl Pts',(4.5647390781119,2.74489822224615,-6.53657517841669)) ;
#135778=CARTESIAN_POINT('Ctrl Pts',(4.47150553186688,2.8018081238784,-6.53642552726426)) ;
#135779=CARTESIAN_POINT('Ctrl Pts',(4.50000000073523,2.74999999866316,-6.54874191573054)) ;
#135780=CARTESIAN_POINT('Ctrl Pts',(4.5591271227348,2.75,-6.55472795424019)) ;
#135781=CARTESIAN_POINT('Ctrl Pts',(4.47150553123747,2.80180812502279,-6.57304604217164)) ;
#135782=CARTESIAN_POINT('Ctrl Pts',(4.5,2.75,-6.57304604217164)) ;
#135783=CARTESIAN_POINT('Ctrl Pts',(4.55912712210513,2.75,-6.57304604217164)) ;
#135784=CARTESIAN_POINT('Origin',(4.57524318173533,2.82069807339964,-6.46882431824783)) ;
#135785=CARTESIAN_POINT('Ctrl Pts',(4.57527448145475,2.73535371598842,-6.52094283394186)) ;
#135786=CARTESIAN_POINT('Ctrl Pts',(4.51316714695682,2.72605973281053,-6.50576118362915)) ;
#135787=CARTESIAN_POINT('Ctrl Pts',(4.48762159086951,2.77250619842363,-6.4688243182477)) ;
#135788=CARTESIAN_POINT('Ctrl Pts',(4.58732687742635,2.72440390874892,-6.50300494332462)) ;
#135789=CARTESIAN_POINT('Ctrl Pts',(4.51469458626358,2.70766538570653,-6.48379912048174)) ;
#135790=CARTESIAN_POINT('Ctrl Pts',(4.49363662433187,2.76156977394665,-6.4330004075269)) ;
#135791=CARTESIAN_POINT('Ctrl Pts',(4.60003973844304,2.7077507197818,-6.48844768348498)) ;
#135792=CARTESIAN_POINT('Ctrl Pts',(4.50856472285793,2.69031485824819,-6.48150883298403)) ;
#135793=CARTESIAN_POINT('Ctrl Pts',(4.5,2.74488438437979,-6.40383078393338)) ;
#135794=CARTESIAN_POINT('Ctrl Pts',(4.60004243494347,2.6871571650681,-6.48020560440432)) ;
#135795=CARTESIAN_POINT('Ctrl Pts',(4.5,2.68714139075513,-6.48024501790961)) ;
#135796=CARTESIAN_POINT('Ctrl Pts',(4.5,2.72431432344521,-6.38736518335501)) ;
#135797=CARTESIAN_POINT('Origin',(4.6,0.280857398566761,-6.76514439140057)) ;
#135798=CARTESIAN_POINT('Origin',(4.6,2.1,-6.46195395782836)) ;
#135799=CARTESIAN_POINT('Origin',(4.6,2.1,-6.46195395782836)) ;
#135800=CARTESIAN_POINT('Origin',(4.6,0.,-5.08)) ;
#135801=CARTESIAN_POINT('',(4.5,-2.9,-5.08000000000385)) ;
#135802=CARTESIAN_POINT('',(4.57439618084313,-2.80937499999937,-6.12279586712545)) ;
#135803=CARTESIAN_POINT('Ctrl Pts',(4.5,-2.9,-5.08000000000385)) ;
#135804=CARTESIAN_POINT('Ctrl Pts',(4.5,-2.9000000234111,-5.25617626257029)) ;
#135805=CARTESIAN_POINT('Ctrl Pts',(4.49893459747296,-2.89187728142186,
-5.43229382255519)) ;
#135806=CARTESIAN_POINT('Ctrl Pts',(4.50498172725087,-2.86839426105774,
-5.69494327688717)) ;
#135807=CARTESIAN_POINT('Ctrl Pts',(4.50826226558342,-2.85869729223562,
-5.78228702711349)) ;
#135808=CARTESIAN_POINT('Ctrl Pts',(4.52028413974051,-2.84160518746962,
-5.9128409654328)) ;
#135809=CARTESIAN_POINT('Ctrl Pts',(4.52545003690602,-2.8354696349403,-5.95636311362202)) ;
#135810=CARTESIAN_POINT('Ctrl Pts',(4.53741870680498,-2.82581179679252,
-6.02063945501075)) ;
#135811=CARTESIAN_POINT('Ctrl Pts',(4.54209540184575,-2.82251395224859,
-6.04192001826058)) ;
#135812=CARTESIAN_POINT('Ctrl Pts',(4.55451190949429,-2.81582803324483,
-6.0838742105328)) ;
#135813=CARTESIAN_POINT('Ctrl Pts',(4.56139306411848,-2.8124020390272,-6.10474353182486)) ;
#135814=CARTESIAN_POINT('Ctrl Pts',(4.57439618084313,-2.80937499999937,
-6.12279586712545)) ;
#135815=CARTESIAN_POINT('Ctrl Pts',(4.57439618084313,-2.80937499999937,
-6.12279586712545)) ;
#135816=CARTESIAN_POINT('Ctrl Pts',(4.57788811720513,-2.80856205104935,
-6.12764388459131)) ;
#135817=CARTESIAN_POINT('Ctrl Pts',(4.58132110715667,-2.80743849592502,
-6.1326543114198)) ;
#135818=CARTESIAN_POINT('Ctrl Pts',(4.58591063786564,-2.80541025280315,
-6.14006834915985)) ;
#135819=CARTESIAN_POINT('Ctrl Pts',(4.58721694730501,-2.80476695238161,
-6.14226832508376)) ;
#135820=CARTESIAN_POINT('Ctrl Pts',(4.5887449802686,-2.80393035430395,-6.14497171464085)) ;
#135821=CARTESIAN_POINT('Ctrl Pts',(4.58900094431508,-2.8037870887984,-6.14542942337304)) ;
#135822=CARTESIAN_POINT('Ctrl Pts',(4.58924476828968,-2.80364801935069,
-6.14586949326005)) ;
#135823=CARTESIAN_POINT('Ctrl Pts',(4.58924931741448,-2.80364542371033,
-6.1458777053493)) ;
#135824=CARTESIAN_POINT('Ctrl Pts',(4.59158188358133,-2.80231401319274,
-6.15008924012213)) ;
#135825=CARTESIAN_POINT('Ctrl Pts',(4.59377134212491,-2.800813098491,-6.15443839239641)) ;
#135826=CARTESIAN_POINT('Ctrl Pts',(4.59570408210448,-2.79909049146271,
-6.1591378632085)) ;
#135827=CARTESIAN_POINT('Ctrl Pts',(4.59570848738489,-2.79908656285628,
-6.15914857957787)) ;
#135828=CARTESIAN_POINT('Ctrl Pts',(4.59603576097761,-2.79879453264351,
-6.15994507543617)) ;
#135829=CARTESIAN_POINT('Ctrl Pts',(4.59633794834607,-2.79851279959495,
-6.16070652531885)) ;
#135830=CARTESIAN_POINT('Ctrl Pts',(4.59727216584803,-2.79759800070516,
-6.16316063340996)) ;
#135831=CARTESIAN_POINT('Ctrl Pts',(4.59785661125443,-2.79695684051616,
-6.16485291560937)) ;
#135832=CARTESIAN_POINT('Ctrl Pts',(4.59875882816121,-2.79580092267551,
-6.16786832422156)) ;
#135833=CARTESIAN_POINT('Ctrl Pts',(4.59910960512328,-2.79529211440566,
-6.16918449921755)) ;
#135834=CARTESIAN_POINT('Ctrl Pts',(4.59950074890552,-2.79458032370897,
-6.17101507841206)) ;
#135835=CARTESIAN_POINT('Ctrl Pts',(4.59959271145697,-2.79439474074568,
-6.17149484058078)) ;
#135836=CARTESIAN_POINT('Ctrl Pts',(4.59970479219924,-2.79411978912796,
-6.1722025710462)) ;
#135837=CARTESIAN_POINT('Ctrl Pts',(4.59973686334512,-2.79403231884249,
-6.17242726844519)) ;
#135838=CARTESIAN_POINT('Ctrl Pts',(4.59980956306601,-2.79380428276742,
-6.17301082640206)) ;
#135839=CARTESIAN_POINT('Ctrl Pts',(4.59984405921136,-2.79366555090846,
-6.17336897900421)) ;
#135840=CARTESIAN_POINT('Ctrl Pts',(4.59992170638736,-2.79338632637293,
-6.1740824135446)) ;
#135841=CARTESIAN_POINT('Ctrl Pts',(4.59995882625634,-2.79324305250059,
-6.17443747925646)) ;
#135842=CARTESIAN_POINT('Ctrl Pts',(4.59999999999999,-2.79310344827586,
-6.17479364595777)) ;
#135843=CARTESIAN_POINT('',(4.57439618084271,-2.80937499999947,-4.03720413287514)) ;
#135844=CARTESIAN_POINT('Ctrl Pts',(4.59999999999999,-2.79310344827586,
-3.98520635404223)) ;
#135845=CARTESIAN_POINT('Ctrl Pts',(4.59995895305209,-2.79324111387631,
-3.98556200704419)) ;
#135846=CARTESIAN_POINT('Ctrl Pts',(4.59992125133673,-2.79338175512528,
-3.98591664999517)) ;
#135847=CARTESIAN_POINT('Ctrl Pts',(4.59984242179761,-2.79365985893298,
-3.98662721825472)) ;
#135848=CARTESIAN_POINT('Ctrl Pts',(4.5998070294299,-2.79379858543765,-3.98698190400296)) ;
#135849=CARTESIAN_POINT('Ctrl Pts',(4.59973261548695,-2.79401893257626,
-3.98754582127962)) ;
#135850=CARTESIAN_POINT('Ctrl Pts',(4.59970092564442,-2.79410050108421,
-3.98775470445263)) ;
#135851=CARTESIAN_POINT('Ctrl Pts',(4.59958060815603,-2.79437456977472,
-3.98845707425772)) ;
#135852=CARTESIAN_POINT('Ctrl Pts',(4.59947821517875,-2.79456857658396,
-3.98895509538074)) ;
#135853=CARTESIAN_POINT('Ctrl Pts',(4.5990597198479,-2.79527981802028,-3.99078506438848)) ;
#135854=CARTESIAN_POINT('Ctrl Pts',(4.59869396429225,-2.79579226918927,
-3.99211140120008)) ;
#135855=CARTESIAN_POINT('Ctrl Pts',(4.59768320083749,-2.79706868650734,
-3.99544407389333)) ;
#135856=CARTESIAN_POINT('Ctrl Pts',(4.59698254015873,-2.79783590182173,
-3.99747319966267)) ;
#135857=CARTESIAN_POINT('Ctrl Pts',(4.5959970522588,-2.79876532988113,-3.99998468423847)) ;
#135858=CARTESIAN_POINT('Ctrl Pts',(4.59580678362761,-2.7989396411024,-4.00045810500393)) ;
#135859=CARTESIAN_POINT('Ctrl Pts',(4.59367882781298,-2.80083904916685,
-4.00564491199709)) ;
#135860=CARTESIAN_POINT('Ctrl Pts',(4.5915070708769,-2.80233337893514,-4.00997932770411)) ;
#135861=CARTESIAN_POINT('Ctrl Pts',(4.58628071719241,-2.80532570224267,
-4.01945146742912)) ;
#135862=CARTESIAN_POINT('Ctrl Pts',(4.58313959595723,-2.80673110767403,
-4.02451024806553)) ;
#135863=CARTESIAN_POINT('Ctrl Pts',(4.57802611146349,-2.80844040952811,
-4.03209635749153)) ;
#135864=CARTESIAN_POINT('Ctrl Pts',(4.57624387811654,-2.80894486836994,
-4.03463895934158)) ;
#135865=CARTESIAN_POINT('Ctrl Pts',(4.57439618084271,-2.80937499999947,
-4.03720413287514)) ;
#135866=CARTESIAN_POINT('Ctrl Pts',(4.57439618084271,-2.80937499999947,
-4.03720413287514)) ;
#135867=CARTESIAN_POINT('Ctrl Pts',(4.56149777794589,-2.81237766235467,
-4.0551110931668)) ;
#135868=CARTESIAN_POINT('Ctrl Pts',(4.55451596106519,-2.81582788236477,
-4.07612624229681)) ;
#135869=CARTESIAN_POINT('Ctrl Pts',(4.54213610452188,-2.82249001163036,
-4.11792835962828)) ;
#135870=CARTESIAN_POINT('Ctrl Pts',(4.53742891479326,-2.82580422498964,
-4.139310967236)) ;
#135871=CARTESIAN_POINT('Ctrl Pts',(4.52545161424301,-2.8354670333868,-4.20361794379489)) ;
#135872=CARTESIAN_POINT('Ctrl Pts',(4.52032009146395,-2.84156292603926,
-4.24685657347849)) ;
#135873=CARTESIAN_POINT('Ctrl Pts',(4.50830110904356,-2.85862448221642,
-4.37711642595738)) ;
#135874=CARTESIAN_POINT('Ctrl Pts',(4.50499166750953,-2.86836219567853,
-4.4647300385823)) ;
#135875=CARTESIAN_POINT('Ctrl Pts',(4.49892845988062,-2.8918880660271,-4.72776299683786)) ;
#135876=CARTESIAN_POINT('Ctrl Pts',(4.49999999999475,-2.89999999999869,
-4.90383009011776)) ;
#135877=CARTESIAN_POINT('Ctrl Pts',(4.5,-2.9,-5.08000000000385)) ;
#135878=CARTESIAN_POINT('Ctrl Pts',(4.40227435089071,-2.79999990867355,
-3.48940069288197)) ;
#135879=CARTESIAN_POINT('Ctrl Pts',(4.51828879250213,-2.80015667527382,
-3.49878556679245)) ;
#135880=CARTESIAN_POINT('Ctrl Pts',(4.50118227077258,-2.68533700727783,
-3.49797110744947)) ;
#135881=CARTESIAN_POINT('Ctrl Pts',(4.39419482113924,-2.79999992837382,
-3.60368769966904)) ;
#135882=CARTESIAN_POINT('Ctrl Pts',(4.48571792501736,-2.80010751836586,
-3.5826713667507)) ;
#135883=CARTESIAN_POINT('Ctrl Pts',(4.49717570077251,-2.71006921719236,
-3.5970318982145)) ;
#135884=CARTESIAN_POINT('Ctrl Pts',(4.40636790575267,-2.79999994706265,
-3.71490890735437)) ;
#135885=CARTESIAN_POINT('Ctrl Pts',(4.47481046024545,-2.80007242131916,
-3.69332242779908)) ;
#135886=CARTESIAN_POINT('Ctrl Pts',(4.50328131876401,-2.73353293829097,
-3.69702587481009)) ;
#135887=CARTESIAN_POINT('Ctrl Pts',(4.45479736994228,-2.79999997092221,
-3.86507366547108)) ;
#135888=CARTESIAN_POINT('Ctrl Pts',(4.49869786247045,-2.80003603117403,
-3.84627924349579)) ;
#135889=CARTESIAN_POINT('Ctrl Pts',(4.52748687875413,-2.76348976047509,
-3.8362891728587)) ;
#135890=CARTESIAN_POINT('Ctrl Pts',(4.47221929614095,-2.79999997745988,
-3.90730406022327)) ;
#135891=CARTESIAN_POINT('Ctrl Pts',(4.50880556767615,-2.8000272573648,-3.88827484828593)) ;
#135892=CARTESIAN_POINT('Ctrl Pts',(4.53619137795527,-2.77169834185705,
-3.87598368236757)) ;
#135893=CARTESIAN_POINT('Ctrl Pts',(4.50882352800135,-2.7999999860536,-3.96428434960906)) ;
#135894=CARTESIAN_POINT('Ctrl Pts',(4.53367802911271,-2.80001636071784,
-3.94535870242034)) ;
#135895=CARTESIAN_POINT('Ctrl Pts',(4.55447319025662,-2.78248861123826,
-3.93009568142552)) ;
#135896=CARTESIAN_POINT('Ctrl Pts',(4.52308919141482,-2.79999998878206,
-3.98266256169107)) ;
#135897=CARTESIAN_POINT('Ctrl Pts',(4.5436396263862,-2.80001303821803,-3.96372615017167)) ;
#135898=CARTESIAN_POINT('Ctrl Pts',(4.56159739427506,-2.78591449131414,
-3.9476542708947)) ;
#135899=CARTESIAN_POINT('Ctrl Pts',(4.57467506176496,-2.79999999510246,
-4.02569650839937)) ;
#135900=CARTESIAN_POINT('Ctrl Pts',(4.58062405303292,-2.80000557393877,
-4.0063341632778)) ;
#135901=CARTESIAN_POINT('Ctrl Pts',(4.58735613403294,-2.79385049254304,
-3.98891981499328)) ;
#135902=CARTESIAN_POINT('Ctrl Pts',(4.62437069655631,-2.79999999703807,
-4.03953134305988)) ;
#135903=CARTESIAN_POINT('Ctrl Pts',(4.6182737266188,-2.80000334969057,-4.02093404548721)) ;
#135904=CARTESIAN_POINT('Ctrl Pts',(4.61212682540737,-2.79628090446616,
-4.00240281421806)) ;
#135905=CARTESIAN_POINT('Ctrl Pts',(4.67161368302049,-2.79999998860619,
-3.98078982676581)) ;
#135906=CARTESIAN_POINT('Ctrl Pts',(4.6540701010266,-2.80001325705919,-3.96046373959001)) ;
#135907=CARTESIAN_POINT('Ctrl Pts',(4.63587130780629,-2.78569367459204,
-3.94562812959451)) ;
#135908=CARTESIAN_POINT('Ctrl Pts',(4.54879236204369,-2.8,-4.0035655563675)) ;
#135909=CARTESIAN_POINT('Ctrl Pts',(4.55448837802407,-2.7999999999815,-4.00117882091359)) ;
#135910=CARTESIAN_POINT('Ctrl Pts',(4.56021842726647,-2.79959150783236,
-3.998839542734)) ;
#135911=CARTESIAN_POINT('Ctrl Pts',(4.56730671985029,-2.79865167182169,
-3.99597888386339)) ;
#135912=CARTESIAN_POINT('Ctrl Pts',(4.56847770958292,-2.79848295770254,
-3.99550732683466)) ;
#135913=CARTESIAN_POINT('Ctrl Pts',(4.57107523099021,-2.79808046368154,
-3.99446296289698)) ;
#135914=CARTESIAN_POINT('Ctrl Pts',(4.5725009361248,-2.79784058543152,-3.99388964302801)) ;
#135915=CARTESIAN_POINT('Ctrl Pts',(4.5764383594612,-2.79713266293194,-3.99231368646489)) ;
#135916=CARTESIAN_POINT('Ctrl Pts',(4.57879956048961,-2.79666132938901,
-3.99137580039693)) ;
#135917=CARTESIAN_POINT('Ctrl Pts',(4.58293855712953,-2.79579586318667,
-3.98976081592963)) ;
#135918=CARTESIAN_POINT('Ctrl Pts',(4.58471363403686,-2.79540911153441,
-3.98907461719119)) ;
#135919=CARTESIAN_POINT('Ctrl Pts',(4.58699082729421,-2.79492697681981,
-3.98824452926203)) ;
#135920=CARTESIAN_POINT('Ctrl Pts',(4.58739952300692,-2.79484234870239,
-3.9881019268464)) ;
#135921=CARTESIAN_POINT('Ctrl Pts',(4.58871515235486,-2.79457617288695,
-3.98766112910085)) ;
#135922=CARTESIAN_POINT('Ctrl Pts',(4.58961690596145,-2.7944024780556,-3.98738498699949)) ;
#135923=CARTESIAN_POINT('Ctrl Pts',(4.5910537506587,-2.79414748185764,-3.98698298181791)) ;
#135924=CARTESIAN_POINT('Ctrl Pts',(4.5915530390955,-2.79406229662442,-3.98684924350712)) ;
#135925=CARTESIAN_POINT('Ctrl Pts',(4.59245965385669,-2.79391282221553,
-3.98661259411486)) ;
#135926=CARTESIAN_POINT('Ctrl Pts',(4.59286388425105,-2.79384761399903,
-3.98650842178452)) ;
#135927=CARTESIAN_POINT('Ctrl Pts',(4.59368973959981,-2.79370598615371,
-3.98626767265165)) ;
#135928=CARTESIAN_POINT('Ctrl Pts',(4.59407665941124,-2.79363973714592,
-3.98615152123316)) ;
#135929=CARTESIAN_POINT('Ctrl Pts',(4.59444371287733,-2.79357284110655,
-3.98602679272788)) ;
#135930=CARTESIAN_POINT('Ctrl Pts',(4.5944889025916,-2.79356452972317,-3.98601115819951)) ;
#135931=CARTESIAN_POINT('Ctrl Pts',(4.59470842334911,-2.79352377141065,
-3.98593382545217)) ;
#135932=CARTESIAN_POINT('Ctrl Pts',(4.59483598733269,-2.79349361011836,
-3.98587233148411)) ;
#135933=CARTESIAN_POINT('Ctrl Pts',(4.59514620525224,-2.7934297131363,-3.9857459400492)) ;
#135934=CARTESIAN_POINT('Ctrl Pts',(4.59533334275102,-2.79339696908416,
-3.9856838378534)) ;
#135935=CARTESIAN_POINT('Ctrl Pts',(4.59563785533348,-2.79335634095568,
-3.98561299034027)) ;
#135936=CARTESIAN_POINT('Ctrl Pts',(4.59571710962763,-2.79334654412182,
-3.98559639128765)) ;
#135937=CARTESIAN_POINT('Ctrl Pts',(4.59594411915587,-2.79332043135007,
-3.9855533496182)) ;
#135938=CARTESIAN_POINT('Ctrl Pts',(4.59600288191153,-2.79330503361987,
-3.98553395124079)) ;
#135939=CARTESIAN_POINT('Ctrl Pts',(4.59613307952174,-2.79327450473787,
-3.98549928051942)) ;
#135940=CARTESIAN_POINT('Ctrl Pts',(4.59620389659312,-2.7932597078882,-3.98548500605855)) ;
#135941=CARTESIAN_POINT('Ctrl Pts',(4.59651192984772,-2.79322709231927,
-3.98545027786287)) ;
#135942=CARTESIAN_POINT('Ctrl Pts',(4.59679543741297,-2.79320989448354,
-3.98542934418241)) ;
#135943=CARTESIAN_POINT('Ctrl Pts',(4.59784475938523,-2.793166495242,-3.9853578835066)) ;
#135944=CARTESIAN_POINT('Ctrl Pts',(4.59874915064779,-2.79313948637392,
-3.98529926431075)) ;
#135945=CARTESIAN_POINT('Ctrl Pts',(4.59999999999999,-2.79310344827586,
-3.98520635404223)) ;
#135946=CARTESIAN_POINT('Origin',(4.4,-2.7,-2.54)) ;
#135947=CARTESIAN_POINT('Origin',(4.4,-2.7,-6.60315462117279)) ;
#135948=CARTESIAN_POINT('Ctrl Pts',(4.5011795914298,-2.68531903459929,-6.66202902017229)) ;
#135949=CARTESIAN_POINT('Ctrl Pts',(4.51828670358941,-2.8,-6.66121382514058)) ;
#135950=CARTESIAN_POINT('Ctrl Pts',(4.40240952225579,-2.8,-6.67058837211076)) ;
#135951=CARTESIAN_POINT('Ctrl Pts',(4.49717774927193,-2.71005310920068,
-6.56296553236259)) ;
#135952=CARTESIAN_POINT('Ctrl Pts',(4.48574628541085,-2.8,-6.5773148520404)) ;
#135953=CARTESIAN_POINT('Ctrl Pts',(4.39431668173578,-2.8,-6.5563402695083)) ;
#135954=CARTESIAN_POINT('Ctrl Pts',(4.50328690685191,-2.73351987602563,
-6.46297339786193)) ;
#135955=CARTESIAN_POINT('Ctrl Pts',(4.47485145549548,-2.8,-6.46667669574134)) ;
#135956=CARTESIAN_POINT('Ctrl Pts',(4.40646789472124,-2.8,-6.44512261863839)) ;
#135957=CARTESIAN_POINT('Ctrl Pts',(4.52749311797091,-2.76348183928881,
-6.3237129921595)) ;
#135958=CARTESIAN_POINT('Ctrl Pts',(4.49873206155793,-2.8,-6.31373309530699)) ;
#135959=CARTESIAN_POINT('Ctrl Pts',(4.4548681704377,-2.8,-6.29495664336612)) ;
#135960=CARTESIAN_POINT('Ctrl Pts',(4.53619745972499,-2.77169205010107,
-6.28401904718521)) ;
#135961=CARTESIAN_POINT('Ctrl Pts',(4.5088366481667,-2.79999999999999,-6.27173943817213)) ;
#135962=CARTESIAN_POINT('Ctrl Pts',(4.47227975612147,-2.8,-6.25272738460372)) ;
#135963=CARTESIAN_POINT('Ctrl Pts',(4.55447795090009,-2.78248459830339,
-6.22990781273338)) ;
#135964=CARTESIAN_POINT('Ctrl Pts',(4.53370055749884,-2.8,-6.21465791836995)) ;
#135965=CARTESIAN_POINT('Ctrl Pts',(4.50886586566854,-2.8,-6.19574788827224)) ;
#135966=CARTESIAN_POINT('Ctrl Pts',(4.56160154376424,-2.78591123334062,
-6.21234944281567)) ;
#135967=CARTESIAN_POINT('Ctrl Pts',(4.54365878772218,-2.8,-6.19629106645425)) ;
#135968=CARTESIAN_POINT('Ctrl Pts',(4.52312452397684,-2.8,-6.17736999548674)) ;
#135969=CARTESIAN_POINT('Ctrl Pts',(4.58735772267364,-2.79384903998488,
-6.17108429439849)) ;
#135970=CARTESIAN_POINT('Ctrl Pts',(4.58063087367386,-2.8,-6.15368396338089)) ;
#135971=CARTESIAN_POINT('Ctrl Pts',(4.57468550767192,-2.8,-6.13433748660569)) ;
#135972=CARTESIAN_POINT('Ctrl Pts',(4.61212536563475,-2.79628002040286,
-6.15760158659528)) ;
#135973=CARTESIAN_POINT('Ctrl Pts',(4.61826745782994,-2.80000000000005,
-6.13908487937516)) ;
#135974=CARTESIAN_POINT('Ctrl Pts',(4.62435992349563,-2.8,-6.12050151732127)) ;
#135975=CARTESIAN_POINT('Ctrl Pts',(4.63586710715934,-2.78569036914635,
-6.21437529467588)) ;
#135976=CARTESIAN_POINT('Ctrl Pts',(4.65405106945717,-2.79999999999983,
-6.19955252388527)) ;
#135977=CARTESIAN_POINT('Ctrl Pts',(4.67158355065755,-2.8,-6.17924507978128)) ;
#135978=CARTESIAN_POINT('Ctrl Pts',(4.59999999999999,-2.79310344827586,
-6.17479364595777)) ;
#135979=CARTESIAN_POINT('Ctrl Pts',(4.59840954578197,-2.79314968944989,
-6.17467567269119)) ;
#135980=CARTESIAN_POINT('Ctrl Pts',(4.59737383489067,-2.79318159606221,
-6.17461332397164)) ;
#135981=CARTESIAN_POINT('Ctrl Pts',(4.59650507521635,-2.79322931786013,
-6.17455037725996)) ;
#135982=CARTESIAN_POINT('Ctrl Pts',(4.59632758424294,-2.79324472590583,
-6.17453457917666)) ;
#135983=CARTESIAN_POINT('Ctrl Pts',(4.59611847210841,-2.79327477162037,
-6.17450475657722)) ;
#135984=CARTESIAN_POINT('Ctrl Pts',(4.59606489504923,-2.79328892979787,
-6.17449102658529)) ;
#135985=CARTESIAN_POINT('Ctrl Pts',(4.59594601677692,-2.79331605564258,
-6.17445911449494)) ;
#135986=CARTESIAN_POINT('Ctrl Pts',(4.59588597444855,-2.7933285533825,-6.17444265618345)) ;
#135987=CARTESIAN_POINT('Ctrl Pts',(4.59549967474364,-2.79337285752324,
-6.17437027876054)) ;
#135988=CARTESIAN_POINT('Ctrl Pts',(4.59527331486237,-2.79340622385959,
-6.17431008070831)) ;
#135989=CARTESIAN_POINT('Ctrl Pts',(4.59493201239529,-2.79346950514991,
-6.17418704029369)) ;
#135990=CARTESIAN_POINT('Ctrl Pts',(4.59480393230128,-2.79349821606423,
-6.17412847427896)) ;
#135991=CARTESIAN_POINT('Ctrl Pts',(4.59460326813595,-2.79353924388982,
-6.17404763514903)) ;
#135992=CARTESIAN_POINT('Ctrl Pts',(4.59455075953096,-2.79354963432651,
-6.17402742767144)) ;
#135993=CARTESIAN_POINT('Ctrl Pts',(4.59417008680874,-2.79361944405452,
-6.17389559371762)) ;
#135994=CARTESIAN_POINT('Ctrl Pts',(4.5937774209655,-2.79368602572532,-6.17377734615548)) ;
#135995=CARTESIAN_POINT('Ctrl Pts',(4.59289939109634,-2.7938335466559,-6.17352541902409)) ;
#135996=CARTESIAN_POINT('Ctrl Pts',(4.59245006584786,-2.79390305456782,
-6.17341603619897)) ;
#135997=CARTESIAN_POINT('Ctrl Pts',(4.59099552519191,-2.79413629528614,
-6.17305685240917)) ;
#135998=CARTESIAN_POINT('Ctrl Pts',(4.5900219788148,-2.79430302757335,-6.17280637017571)) ;
#135999=CARTESIAN_POINT('Ctrl Pts',(4.58861122644573,-2.79456793455722,
-6.17239213656651)) ;
#136000=CARTESIAN_POINT('Ctrl Pts',(4.58817904894346,-2.79465210327464,
-6.17225852343037)) ;
#136001=CARTESIAN_POINT('Ctrl Pts',(4.58736872283365,-2.79481449815582,
-6.17199418358962)) ;
#136002=CARTESIAN_POINT('Ctrl Pts',(4.58699491219413,-2.79489135860975,
-6.17186658235812)) ;
#136003=CARTESIAN_POINT('Ctrl Pts',(4.58468897497186,-2.79537899446709,
-6.17103519061958)) ;
#136004=CARTESIAN_POINT('Ctrl Pts',(4.58290717718701,-2.79577019617637,
-6.1703420642284)) ;
#136005=CARTESIAN_POINT('Ctrl Pts',(4.57867627871777,-2.79666451416568,
-6.16867078828749)) ;
#136006=CARTESIAN_POINT('Ctrl Pts',(4.57626321554132,-2.79715040843618,
-6.16768776514285)) ;
#136007=CARTESIAN_POINT('Ctrl Pts',(4.57243386308706,-2.79784156172336,
-6.1661367865103)) ;
#136008=CARTESIAN_POINT('Ctrl Pts',(4.57107519984216,-2.79807176647234,
-6.16558402144498)) ;
#136009=CARTESIAN_POINT('Ctrl Pts',(4.56513452430488,-2.79900074294388,
-6.16316939035812)) ;
#136010=CARTESIAN_POINT('Ctrl Pts',(4.56062162665774,-2.79951267011375,
-6.1613309293496)) ;
#136011=CARTESIAN_POINT('Ctrl Pts',(4.55365420596667,-2.79992470862866,
-6.1584610302785)) ;
#136012=CARTESIAN_POINT('Ctrl Pts',(4.55124660967284,-2.79999983267432,
-6.15746323925077)) ;
#136013=CARTESIAN_POINT('Ctrl Pts',(4.54880051362943,-2.79999999972164,
-6.15643786073294)) ;
#136014=CARTESIAN_POINT('Ctrl Pts',(4.54879236166275,-2.8,-4.00356555651516)) ;
#136015=CARTESIAN_POINT('Ctrl Pts',(4.5622387183224,-2.79999999999679,-4.02123152627487)) ;
#136016=CARTESIAN_POINT('Ctrl Pts',(4.57442182196495,-2.80939476060287,
-4.03723782046681)) ;
#136017=CARTESIAN_POINT('Ctrl Pts',(4.5555684251759,-2.79999999999889,-4.00072506404886)) ;
#136018=CARTESIAN_POINT('Ctrl Pts',(4.56783337210915,-2.80040661803735,
-4.01618630155189)) ;
#136019=CARTESIAN_POINT('Ctrl Pts',(4.5796182352237,-2.80818164104597,-4.03001834132724)) ;
#136020=CARTESIAN_POINT('Ctrl Pts',(4.5623898283162,-2.79942602551759,-3.99795285151707)) ;
#136021=CARTESIAN_POINT('Ctrl Pts',(4.57357810388183,-2.80014618986472,
-4.01093107214122)) ;
#136022=CARTESIAN_POINT('Ctrl Pts',(4.58462643299474,-2.80630261261112,
-4.02252327116488)) ;
#136023=CARTESIAN_POINT('Ctrl Pts',(4.57328757735257,-2.7977370397245,-3.99356999795014)) ;
#136024=CARTESIAN_POINT('Ctrl Pts',(4.58237922839514,-2.79856394574987,
-4.00226640893136)) ;
#136025=CARTESIAN_POINT('Ctrl Pts',(4.59151541127592,-2.80237286596199,
-4.01008300288058)) ;
#136026=CARTESIAN_POINT('Ctrl Pts',(4.57700059755674,-2.7970371466716,-3.99207607634203)) ;
#136027=CARTESIAN_POINT('Ctrl Pts',(4.58532305318676,-2.79784352093717,
-3.99926254300445)) ;
#136028=CARTESIAN_POINT('Ctrl Pts',(4.59370961102545,-2.80088045369937,
-4.00574551418945)) ;
#136029=CARTESIAN_POINT('Ctrl Pts',(4.58319893207066,-2.79574016930783,
-3.98965467052114)) ;
#136030=CARTESIAN_POINT('Ctrl Pts',(4.5899041610924,-2.79637293360539,-3.99433035456225)) ;
#136031=CARTESIAN_POINT('Ctrl Pts',(4.59665800356695,-2.79825577077759,
-3.99858194486972)) ;
#136032=CARTESIAN_POINT('Ctrl Pts',(4.58534994317986,-2.79526732601294,
-3.98881886188718)) ;
#136033=CARTESIAN_POINT('Ctrl Pts',(4.59144552977844,-2.79581844972913,
-3.99262003661071)) ;
#136034=CARTESIAN_POINT('Ctrl Pts',(4.59758018705035,-2.79731769672697,
-3.99608858039389)) ;
#136035=CARTESIAN_POINT('Ctrl Pts',(4.58899927751306,-2.79450268149332,
-3.98751730126711)) ;
#136036=CARTESIAN_POINT('Ctrl Pts',(4.59386223202754,-2.79488630507105,
-3.98994951703029)) ;
#136037=CARTESIAN_POINT('Ctrl Pts',(4.59874684688641,-2.79582009356912,
-3.99218136524475)) ;
#136038=CARTESIAN_POINT('Ctrl Pts',(4.59026755692872,-2.79423885380164,
-3.98707439958004)) ;
#136039=CARTESIAN_POINT('Ctrl Pts',(4.59467706068312,-2.79455862385202,
-3.98904054333606)) ;
#136040=CARTESIAN_POINT('Ctrl Pts',(4.59910266898803,-2.79530499526365,
-3.99084863990216)) ;
#136041=CARTESIAN_POINT('Ctrl Pts',(4.59257623319513,-2.79382131826659,
-3.98638413144999)) ;
#136042=CARTESIAN_POINT('Ctrl Pts',(4.59605751036344,-2.79403163929513,
-3.98762276103362)) ;
#136043=CARTESIAN_POINT('Ctrl Pts',(4.59954701072604,-2.79449510806573,
-3.98876576681697)) ;
#136044=CARTESIAN_POINT('Ctrl Pts',(4.59342976933297,-2.79367543507711,
-3.98614453745337)) ;
#136045=CARTESIAN_POINT('Ctrl Pts',(4.59655016100493,-2.79384713427256,
-3.98713488953029)) ;
#136046=CARTESIAN_POINT('Ctrl Pts',(4.59967640178298,-2.79421605292372,
-3.98805021393703)) ;
#136047=CARTESIAN_POINT('Ctrl Pts',(4.59428414179641,-2.79346156087783,
-3.98570693618526)) ;
#136048=CARTESIAN_POINT('Ctrl Pts',(4.59704519451433,-2.79355469746529,
-3.98637363574795)) ;
#136049=CARTESIAN_POINT('Ctrl Pts',(4.5998104157401,-2.79379877456676,-3.98698237127069)) ;
#136050=CARTESIAN_POINT('Ctrl Pts',(4.59432658472652,-2.7933916625364,-3.98553381814949)) ;
#136051=CARTESIAN_POINT('Ctrl Pts',(4.59708408719785,-2.79345234504014,
-3.98610907664628)) ;
#136052=CARTESIAN_POINT('Ctrl Pts',(4.59984563524626,-2.79366003518351,
-3.98662765435266)) ;
#136053=CARTESIAN_POINT('Ctrl Pts',(4.59537197237733,-2.79324260992761,
-3.98528726159385)) ;
#136054=CARTESIAN_POINT('Ctrl Pts',(4.59764722167537,-2.79326383513929,
-3.985620961855)) ;
#136055=CARTESIAN_POINT('Ctrl Pts',(4.59992475053754,-2.79338190759658,
-3.98591703064758)) ;
#136056=CARTESIAN_POINT('Ctrl Pts',(4.59364183392371,-2.79313407032025,
-3.98528447884512)) ;
#136057=CARTESIAN_POINT('Ctrl Pts',(4.59684754854893,-2.79327107597597,
-3.9856389310452)) ;
#136058=CARTESIAN_POINT('Ctrl Pts',(4.59996664298755,-2.79324102308607,
-3.98556177368153)) ;
#136059=CARTESIAN_POINT('Ctrl Pts',(4.59999999999999,-2.79310344827586,
-3.98520635404223)) ;
#136060=CARTESIAN_POINT('Ctrl Pts',(4.59999999999999,-2.79310344827586,
-3.98520635404223)) ;
#136061=CARTESIAN_POINT('Ctrl Pts',(4.59999999999999,-2.79310344827586,
-3.98520635404223)) ;
#136062=CARTESIAN_POINT('Origin',(4.54879236168542,-2.9,-4.00356555651607)) ;
#136063=CARTESIAN_POINT('Ctrl Pts',(4.39959973407451,-2.8,-5.19059224280254)) ;
#136064=CARTESIAN_POINT('Ctrl Pts',(4.49922290141885,-2.8,-5.19010524833144)) ;
#136065=CARTESIAN_POINT('Ctrl Pts',(4.49980764094185,-2.8996950427638,-5.19060804589504)) ;
#136066=CARTESIAN_POINT('Ctrl Pts',(4.40142712570759,-2.8,-4.96953389600773)) ;
#136067=CARTESIAN_POINT('Ctrl Pts',(4.50593622119654,-2.8,-4.96604801346827)) ;
#136068=CARTESIAN_POINT('Ctrl Pts',(4.50067611734351,-2.90411960318543,
-4.96965028712544)) ;
#136069=CARTESIAN_POINT('Ctrl Pts',(4.39573539165433,-2.8,-4.74762254178847)) ;
#136070=CARTESIAN_POINT('Ctrl Pts',(4.49039105203448,-2.8,-4.76644486600883)) ;
#136071=CARTESIAN_POINT('Ctrl Pts',(4.49793210898572,-2.89506044297348,
-4.74659283506961)) ;
#136072=CARTESIAN_POINT('Ctrl Pts',(4.41164816536272,-2.8,-4.43449214865647)) ;
#136073=CARTESIAN_POINT('Ctrl Pts',(4.48203507549538,-2.8,-4.44300753838916)) ;
#136074=CARTESIAN_POINT('Ctrl Pts',(4.50604587949365,-2.86657833599734,
-4.44179163345507)) ;
#136075=CARTESIAN_POINT('Ctrl Pts',(4.41940490599913,-2.8,-4.34215713199869)) ;
#136076=CARTESIAN_POINT('Ctrl Pts',(4.48133975791573,-2.8,-4.35332746373866)) ;
#136077=CARTESIAN_POINT('Ctrl Pts',(4.50997623336228,-2.85625883833136,
-4.35306464323898)) ;
#136078=CARTESIAN_POINT('Ctrl Pts',(4.4457743437364,-2.8,-4.20702065882598)) ;
#136079=CARTESIAN_POINT('Ctrl Pts',(4.49360122670478,-2.8,-4.21933058766783)) ;
#136080=CARTESIAN_POINT('Ctrl Pts',(4.52318558604184,-2.83896465559566,
-4.22548504243761)) ;
#136081=CARTESIAN_POINT('Ctrl Pts',(4.45692583760035,-2.8,-4.16247689305276)) ;
#136082=CARTESIAN_POINT('Ctrl Pts',(4.49949391572668,-2.8,-4.17605430264613)) ;
#136083=CARTESIAN_POINT('Ctrl Pts',(4.52876348458385,-2.8328925815763,-4.18380298860427)) ;
#136084=CARTESIAN_POINT('Ctrl Pts',(4.50378503771654,-2.8,-4.04107591625834)) ;
#136085=CARTESIAN_POINT('Ctrl Pts',(4.52873519606808,-2.8,-4.05992534227479)) ;
#136086=CARTESIAN_POINT('Ctrl Pts',(4.55214466721903,-2.81552005845344,
-4.07122486980161)) ;
#136087=CARTESIAN_POINT('Ctrl Pts',(4.5471442379016,-2.8,-3.9622684950464)) ;
#136088=CARTESIAN_POINT('Ctrl Pts',(4.55761617337291,-2.8,-3.98320656418789)) ;
#136089=CARTESIAN_POINT('Ctrl Pts',(4.5725958481338,-2.80338245043785,-4.00123859518852)) ;
#136090=CARTESIAN_POINT('Ctrl Pts',(4.67762904165661,-2.8,-3.97149504479684)) ;
#136091=CARTESIAN_POINT('Ctrl Pts',(4.66093484725016,-2.8,-3.98706706583889)) ;
#136092=CARTESIAN_POINT('Ctrl Pts',(4.64133868807469,-2.80368623369366,
-4.00468800638713)) ;
#136093=CARTESIAN_POINT('Origin',(4.4,-2.9,-5.08000000000385)) ;
#136094=CARTESIAN_POINT('Ctrl Pts',(4.72172783566997,-2.8000000024879,-6.18036295491321)) ;
#136095=CARTESIAN_POINT('Ctrl Pts',(4.69645430307969,-2.7999966052579,-6.16707004731005)) ;
#136096=CARTESIAN_POINT('Ctrl Pts',(4.66463283185045,-2.80454824226947,
-6.14949036829302)) ;
#136097=CARTESIAN_POINT('Ctrl Pts',(4.55709227475159,-2.80000000030524,
-6.21599643631003)) ;
#136098=CARTESIAN_POINT('Ctrl Pts',(4.56399237478705,-2.79999958643656,
-6.19395937920066)) ;
#136099=CARTESIAN_POINT('Ctrl Pts',(4.57729370999481,-2.80055804294518,
-6.1751759050806)) ;
#136100=CARTESIAN_POINT('Ctrl Pts',(4.50667826286322,-2.80000000784871,
-6.12661464799816)) ;
#136101=CARTESIAN_POINT('Ctrl Pts',(4.53037382014979,-2.79998899178918,
-6.1070846001167)) ;
#136102=CARTESIAN_POINT('Ctrl Pts',(4.55348183854644,-2.81434699509192,
-6.09594660411389)) ;
#136103=CARTESIAN_POINT('Ctrl Pts',(4.45692280158724,-2.80000001789831,
-5.99764221828758)) ;
#136104=CARTESIAN_POINT('Ctrl Pts',(4.49938029267375,-2.79997354447564,
-5.98409988800932)) ;
#136105=CARTESIAN_POINT('Ctrl Pts',(4.52864149761209,-2.83271033979016,
-5.9763290620799)) ;
#136106=CARTESIAN_POINT('Ctrl Pts',(4.44554661086163,-2.80000002126189,
-5.95237744001399)) ;
#136107=CARTESIAN_POINT('Ctrl Pts',(4.49333665154859,-2.7999679796365,-5.9400969398739)) ;
#136108=CARTESIAN_POINT('Ctrl Pts',(4.52295544156363,-2.83885474437132,
-5.93396785822799)) ;
#136109=CARTESIAN_POINT('Ctrl Pts',(4.41903322104337,-2.8000000307772,-5.81589479757718)) ;
#136110=CARTESIAN_POINT('Ctrl Pts',(4.48100616080251,-2.79995095769182,
-5.80473000402043)) ;
#136111=CARTESIAN_POINT('Ctrl Pts',(4.50969337368906,-2.85623179093886,
-5.80506962360893)) ;
#136112=CARTESIAN_POINT('Ctrl Pts',(4.41147189908671,-2.8000000363501,-5.72424159004355)) ;
#136113=CARTESIAN_POINT('Ctrl Pts',(4.48178828424061,-2.79993989905029,
-5.71578914920562)) ;
#136114=CARTESIAN_POINT('Ctrl Pts',(4.50589025525746,-2.86640526991155,
-5.71696815120114)) ;
#136115=CARTESIAN_POINT('Ctrl Pts',(4.39523119070919,-2.80000005228414,
-5.40317951983274)) ;
#136116=CARTESIAN_POINT('Ctrl Pts',(4.4903383634593,-2.79990261688304,-5.38307413166043)) ;
#136117=CARTESIAN_POINT('Ctrl Pts',(4.49769757367178,-2.8954773795302,-5.40433321576157)) ;
#136118=CARTESIAN_POINT('Ctrl Pts',(4.40178225889351,-2.80000005718968,
-5.17262397828535)) ;
#136119=CARTESIAN_POINT('Ctrl Pts',(4.50681341018205,-2.79988784121843,
-5.17705819882443)) ;
#136120=CARTESIAN_POINT('Ctrl Pts',(4.50092255053473,-2.90441958896115,
-5.17244069603922)) ;
#136121=CARTESIAN_POINT('Ctrl Pts',(4.39924589760307,-2.80000005405718,
-4.94303116887986)) ;
#136122=CARTESIAN_POINT('Ctrl Pts',(4.49795607191426,-2.79989746608216,
-4.94392293749601)) ;
#136123=CARTESIAN_POINT('Ctrl Pts',(4.49968270404899,-2.89870974459585,
-4.94302849459147)) ;
#136124=CARTESIAN_POINT('Origin',(4.54879236168626,-2.9,-6.15643444348457)) ;
#136125=CARTESIAN_POINT('Ctrl Pts',(4.57442492185553,-2.809397151199,-6.12275810686208)) ;
#136126=CARTESIAN_POINT('Ctrl Pts',(4.56210583156796,-2.79989612750329,
-6.13894306178873)) ;
#136127=CARTESIAN_POINT('Ctrl Pts',(4.54850917782856,-2.80000109307748,
-6.15680649348806)) ;
#136128=CARTESIAN_POINT('Ctrl Pts',(4.57959763980855,-2.80818914940071,
-6.12994530049546)) ;
#136129=CARTESIAN_POINT('Ctrl Pts',(4.56768008075465,-2.80031924975227,
-6.14394104572909)) ;
#136130=CARTESIAN_POINT('Ctrl Pts',(4.55527876038347,-2.79999229227378,
-6.15958997638679)) ;
#136131=CARTESIAN_POINT('Ctrl Pts',(4.58464248447265,-2.80630474344638,
-6.13748431263835)) ;
#136132=CARTESIAN_POINT('Ctrl Pts',(4.57346944634371,-2.80008318972134,
-6.14920129105219)) ;
#136133=CARTESIAN_POINT('Ctrl Pts',(4.56216307187793,-2.79941338753917,
-6.16232809153347)) ;
#136134=CARTESIAN_POINT('Ctrl Pts',(4.59159231899494,-2.80232720646228,
-6.15005636929591)) ;
#136135=CARTESIAN_POINT('Ctrl Pts',(4.58237910662986,-2.79850221241048,
-6.15791493625778)) ;
#136136=CARTESIAN_POINT('Ctrl Pts',(4.57321634584968,-2.79769868647539,
-6.16666448649469)) ;
#136137=CARTESIAN_POINT('Ctrl Pts',(4.59378564167737,-2.8008235544484,-6.15441458376545)) ;
#136138=CARTESIAN_POINT('Ctrl Pts',(4.58533966160572,-2.79778056279966,
-6.16091806944782)) ;
#136139=CARTESIAN_POINT('Ctrl Pts',(4.57696130093819,-2.79699227428059,
-6.16813207403618)) ;
#136140=CARTESIAN_POINT('Ctrl Pts',(4.59669734138576,-2.79821861236081,
-6.16151744690911)) ;
#136141=CARTESIAN_POINT('Ctrl Pts',(4.58989502505308,-2.79633072300511,
-6.16578370298497)) ;
#136142=CARTESIAN_POINT('Ctrl Pts',(4.58314295739387,-2.79570785369251,
-6.17047890318142)) ;
#136143=CARTESIAN_POINT('Ctrl Pts',(4.59760632414568,-2.79728965034655,
-6.16398524662906)) ;
#136144=CARTESIAN_POINT('Ctrl Pts',(4.59142619397023,-2.79578507327358,
-6.16746789372295)) ;
#136145=CARTESIAN_POINT('Ctrl Pts',(4.58528630332434,-2.79524119148169,
-6.17128737837496)) ;
#136146=CARTESIAN_POINT('Ctrl Pts',(4.59875741430933,-2.79580683383093,
-6.16785300449597)) ;
#136147=CARTESIAN_POINT('Ctrl Pts',(4.59383193680337,-2.79486773439436,
-6.17009800553386)) ;
#136148=CARTESIAN_POINT('Ctrl Pts',(4.58892874314203,-2.79448758877844,
-6.17254647301294)) ;
#136149=CARTESIAN_POINT('Ctrl Pts',(4.59910834609947,-2.79529718130591,
-6.16917149930145)) ;
#136150=CARTESIAN_POINT('Ctrl Pts',(4.59464343907623,-2.79454543406795,
-6.17099269585011)) ;
#136151=CARTESIAN_POINT('Ctrl Pts',(4.59019511689903,-2.79422790851556,
-6.17297467120907)) ;
#136152=CARTESIAN_POINT('Ctrl Pts',(4.59954688679867,-2.79449699552073,
-6.17122938465871)) ;
#136153=CARTESIAN_POINT('Ctrl Pts',(4.59601732089134,-2.79402779797774,
-6.17238633635183)) ;
#136154=CARTESIAN_POINT('Ctrl Pts',(4.59249627585269,-2.79381771894921,
-6.17364111416749)) ;
#136155=CARTESIAN_POINT('Ctrl Pts',(4.59967529310588,-2.79422450025963,
-6.17193546456122)) ;
#136156=CARTESIAN_POINT('Ctrl Pts',(4.59651100242293,-2.79384821317134,
-6.17286441087348)) ;
#136157=CARTESIAN_POINT('Ctrl Pts',(4.59335287412397,-2.79367727499394,
-6.17387144765739)) ;
#136158=CARTESIAN_POINT('Ctrl Pts',(4.59980981518572,-2.79380630943631,
-6.17300564521014)) ;
#136159=CARTESIAN_POINT('Ctrl Pts',(4.59701056623719,-2.79355888022806,
-6.17362493503647)) ;
#136160=CARTESIAN_POINT('Ctrl Pts',(4.59421559911326,-2.79346462438277,
-6.17430302898986)) ;
#136161=CARTESIAN_POINT('Ctrl Pts',(4.59984534134842,-2.79366726490194,
-6.17336460674889)) ;
#136162=CARTESIAN_POINT('Ctrl Pts',(4.59705039509826,-2.79345667046144,
-6.17389173939615)) ;
#136163=CARTESIAN_POINT('Ctrl Pts',(4.59425962044003,-2.79339574833516,
-6.17447656370425)) ;
#136164=CARTESIAN_POINT('Ctrl Pts',(4.59992484646001,-2.7933873519883,-6.17407980383996)) ;
#136165=CARTESIAN_POINT('Ctrl Pts',(4.5976165286321,-2.7932668237374,-6.17438058953102)) ;
#136166=CARTESIAN_POINT('Ctrl Pts',(4.59531061070858,-2.79324678512396,
-6.17472041373345)) ;
#136167=CARTESIAN_POINT('Ctrl Pts',(4.59996721368508,-2.79324340897637,
-6.17443656979399)) ;
#136168=CARTESIAN_POINT('Ctrl Pts',(4.59680854952868,-2.79327323421044,
-6.17436047786158)) ;
#136169=CARTESIAN_POINT('Ctrl Pts',(4.59356174266137,-2.79313094944462,
-6.17472348332067)) ;
#136170=CARTESIAN_POINT('Ctrl Pts',(4.59999999999999,-2.79310344827586,
-6.17479364595777)) ;
#136171=CARTESIAN_POINT('Ctrl Pts',(4.59999999999999,-2.79310344827586,
-6.17479364595777)) ;
#136172=CARTESIAN_POINT('Ctrl Pts',(4.59999999999999,-2.79310344827586,
-6.17479364595777)) ;
#136173=CARTESIAN_POINT('Origin',(8.6,4.09462794777298,-2.775)) ;
#136174=CARTESIAN_POINT('Origin',(8.6,4.09462794777298,-2.775)) ;
#136175=CARTESIAN_POINT('Origin',(8.6,4.09462794777298,-2.775)) ;
#136176=CARTESIAN_POINT('Origin',(8.6,4.09462794777298,-1.475)) ;
#136177=CARTESIAN_POINT('Origin',(8.6,4.09462794777298,-1.475)) ;
#136178=CARTESIAN_POINT('Origin',(8.6,4.09462794777298,-1.475)) ;
#136179=CARTESIAN_POINT('Origin',(8.6,3.95,-2.775)) ;
#136180=CARTESIAN_POINT('Origin',(8.6,3.95,-2.775)) ;
#136181=CARTESIAN_POINT('Origin',(8.6,4.09462794777298,-2.775)) ;
#136182=CARTESIAN_POINT('Origin',(7.25334304318326,5.40585602606554,-2.775)) ;
#136183=CARTESIAN_POINT('Origin',(7.25334304318326,5.40585602606554,-1.475)) ;
#136184=CARTESIAN_POINT('Origin',(7.25334304318326,5.40585602606554,-1.475)) ;
#136185=CARTESIAN_POINT('Origin',(8.6,5.40585602606554,-1.475)) ;
#136186=CARTESIAN_POINT('Origin',(8.6,3.95,-1.475)) ;
#136187=CARTESIAN_POINT('Origin',(8.6,3.95,-2.775)) ;
#136188=CARTESIAN_POINT('Origin',(8.6,3.95,-2.775)) ;
#136189=CARTESIAN_POINT('Origin',(7.25334304318326,5.40585602606554,-2.775)) ;
#136190=CARTESIAN_POINT('Origin',(7.25334304318326,5.40585602606554,-2.775)) ;
#136191=CARTESIAN_POINT('Origin',(7.25334304318326,5.40585602606554,-1.475)) ;
#136192=CARTESIAN_POINT('Origin',(7.25334304318326,5.40585602606554,-1.475)) ;
#136193=CARTESIAN_POINT('Origin',(8.6,3.95,-1.475)) ;
#136194=CARTESIAN_POINT('Origin',(8.6,3.95,-1.475)) ;
#136195=CARTESIAN_POINT('Origin',(7.36677829147199,4.5782099492339,-2.775)) ;
#136196=CARTESIAN_POINT('Origin',(7.36677829147199,4.5782099492339,-2.775)) ;
#136197=CARTESIAN_POINT('Origin',(7.25334304318326,5.40585602606554,-2.775)) ;
#136198=CARTESIAN_POINT('Ctrl Pts',(4.03523814377473,5.98727788898885,-2.775)) ;
#136199=CARTESIAN_POINT('Ctrl Pts',(4.03523814427722,5.98727788891385,-2.82947128016675)) ;
#136200=CARTESIAN_POINT('Ctrl Pts',(4.04195902792202,5.94024173112809,-2.875)) ;
#136201=CARTESIAN_POINT('Ctrl Pts',(4.05,5.88396692803319,-2.875)) ;
#136202=CARTESIAN_POINT('Origin',(4.05,6.08618232569815,-2.875)) ;
#136203=CARTESIAN_POINT('Origin',(4.05,6.08618232569815,-1.475)) ;
#136204=CARTESIAN_POINT('Origin',(4.05,6.08618232569815,-2.775)) ;
#136205=CARTESIAN_POINT('Origin',(7.25334304318326,5.40585602606554,-1.475)) ;
#136206=CARTESIAN_POINT('Ctrl Pts',(4.05,5.88396692803319,-1.375)) ;
#136207=CARTESIAN_POINT('Ctrl Pts',(4.04195902792202,5.94024173112809,-1.375)) ;
#136208=CARTESIAN_POINT('Ctrl Pts',(4.03523814427722,5.98727788891385,-1.42052871983325)) ;
#136209=CARTESIAN_POINT('Ctrl Pts',(4.03523814377473,5.98727788898885,-1.475)) ;
#136210=CARTESIAN_POINT('Origin',(6.94197060168454,4.79460933256464,-1.475)) ;
#136211=CARTESIAN_POINT('Origin',(7.36677829147199,4.5782099492339,-1.475)) ;
#136212=CARTESIAN_POINT('Origin',(7.27599715910381,4.4,-2.775)) ;
#136213=CARTESIAN_POINT('Origin',(7.27599715910381,4.6,-2.775)) ;
#136214=CARTESIAN_POINT('Ctrl Pts',(3.95,6.08618232569815,-2.775)) ;
#136215=CARTESIAN_POINT('Ctrl Pts',(3.95,6.,-2.775)) ;
#136216=CARTESIAN_POINT('Ctrl Pts',(4.03523814377473,5.98727788898885,-2.775)) ;
#136217=CARTESIAN_POINT('Ctrl Pts',(3.95,6.08618232225605,-2.88394256277222)) ;
#136218=CARTESIAN_POINT('Ctrl Pts',(3.95,5.99999999675454,-2.838335940386)) ;
#136219=CARTESIAN_POINT('Ctrl Pts',(4.03523814427722,5.98727788891385,-2.82947128016675)) ;
#136220=CARTESIAN_POINT('Ctrl Pts',(3.95,5.99411624638818,-2.97499999670621)) ;
#136221=CARTESIAN_POINT('Ctrl Pts',(3.94999999999981,5.93865134487241,-2.88281389783655)) ;
#136222=CARTESIAN_POINT('Ctrl Pts',(4.04195902792202,5.94024173112809,-2.875)) ;
#136223=CARTESIAN_POINT('Ctrl Pts',(3.95,5.88396692803319,-2.975)) ;
#136224=CARTESIAN_POINT('Ctrl Pts',(3.95,5.8839669280332,-2.875)) ;
#136225=CARTESIAN_POINT('Ctrl Pts',(4.05,5.88396692803319,-2.875)) ;
#136226=CARTESIAN_POINT('Origin',(4.05,5.88396692803319,-2.975)) ;
#136227=CARTESIAN_POINT('Ctrl Pts',(3.95,5.88396692803319,-1.275)) ;
#136228=CARTESIAN_POINT('Ctrl Pts',(3.95,5.8839669280332,-1.375)) ;
#136229=CARTESIAN_POINT('Ctrl Pts',(4.05,5.88396692803319,-1.375)) ;
#136230=CARTESIAN_POINT('Ctrl Pts',(3.95,5.99411624638819,-1.27500000329373)) ;
#136231=CARTESIAN_POINT('Ctrl Pts',(3.95,5.9386513448724,-1.36718610216324)) ;
#136232=CARTESIAN_POINT('Ctrl Pts',(4.04195902792202,5.94024173112809,-1.375)) ;
#136233=CARTESIAN_POINT('Ctrl Pts',(3.95,6.08618232225605,-1.36605743722782)) ;
#136234=CARTESIAN_POINT('Ctrl Pts',(3.95,5.99999999675454,-1.41166405961416)) ;
#136235=CARTESIAN_POINT('Ctrl Pts',(4.03523814427722,5.98727788891385,-1.42052871983325)) ;
#136236=CARTESIAN_POINT('Ctrl Pts',(3.95,6.08618232569815,-1.475)) ;
#136237=CARTESIAN_POINT('Ctrl Pts',(3.95,6.,-1.475)) ;
#136238=CARTESIAN_POINT('Ctrl Pts',(4.03523814377473,5.98727788898885,-1.475)) ;
#136239=CARTESIAN_POINT('Origin',(4.05,5.88396692803319,-1.275)) ;
#136240=CARTESIAN_POINT('Origin',(7.27599715910381,4.4,-1.475)) ;
#136241=CARTESIAN_POINT('Origin',(7.27599715910381,4.6,-1.475)) ;
#136242=CARTESIAN_POINT('Origin',(3.95,4.6,-2.775)) ;
#136243=CARTESIAN_POINT('Origin',(4.05,4.6,-2.775)) ;
#136244=CARTESIAN_POINT('Origin',(4.05,3.75,-2.975)) ;
#136245=CARTESIAN_POINT('Origin',(4.05,4.6,-2.975)) ;
#136246=CARTESIAN_POINT('Origin',(4.05,5.40585602606554,-1.275)) ;
#136247=CARTESIAN_POINT('Origin',(4.05,4.6,-1.275)) ;
#136248=CARTESIAN_POINT('Origin',(7.25334304318326,4.6,-1.475)) ;
#136249=CARTESIAN_POINT('Origin',(4.05,4.6,-1.475)) ;
#136250=CARTESIAN_POINT('Origin',(4.05,4.6,-2.775)) ;
#136251=CARTESIAN_POINT('Origin',(4.05,4.4,-2.775)) ;
#136252=CARTESIAN_POINT('Origin',(4.05,4.6,-1.475)) ;
#136253=CARTESIAN_POINT('Origin',(4.05,4.4,-1.475)) ;
#136254=CARTESIAN_POINT('Origin',(4.05,4.4,2.54)) ;
#136255=CARTESIAN_POINT('Origin',(4.6,2.65,-16.7330460421716)) ;
#136256=CARTESIAN_POINT('',(4.5,2.61712020253893,-16.5357672574052)) ;
#136257=CARTESIAN_POINT('',(4.5,2.72431432344521,-16.547365183355)) ;
#136258=CARTESIAN_POINT('Origin',(4.5,2.65,-16.7330460421716)) ;
#136259=CARTESIAN_POINT('',(4.6,2.63356010126946,-16.6344066497884)) ;
#136260=CARTESIAN_POINT('Origin',(4.6,2.61712020253893,-16.5357672574052)) ;
#136261=CARTESIAN_POINT('',(4.6,2.68715716172261,-16.6402056127633)) ;
#136262=CARTESIAN_POINT('Origin',(4.6,2.65,-16.7330460421716)) ;
#136263=CARTESIAN_POINT('Origin',(4.6,2.72431432344521,-16.547365183355)) ;
#136264=CARTESIAN_POINT('Origin',(0.,10.85,-15.24)) ;
#136265=CARTESIAN_POINT('',(-2.44929359829471E-16,10.95,-13.24)) ;
#136266=CARTESIAN_POINT('Origin',(0.,10.95,-15.24)) ;
#136267=CARTESIAN_POINT('',(-2.32682891837997E-16,10.85,-13.34)) ;
#136268=CARTESIAN_POINT('Origin',(-2.44929359829471E-16,10.85,-13.24)) ;
#136269=CARTESIAN_POINT('',(2.32682891837997E-16,10.85,-17.14)) ;
#136270=CARTESIAN_POINT('Origin',(0.,10.85,-15.24)) ;
#136271=CARTESIAN_POINT('Origin',(0.,10.85,-15.24)) ;
#136272=CARTESIAN_POINT('Origin',(11.0914213562373,0.,-15.24)) ;
#136273=CARTESIAN_POINT('',(11.0207106781187,-1.80110112442985E-16,-13.7692893218813)) ;
#136274=CARTESIAN_POINT('Origin',(11.0207106781187,0.,-15.24)) ;
#136275=CARTESIAN_POINT('',(11.0914213562373,-1.83697019872103E-16,-13.74)) ;
#136276=CARTESIAN_POINT('Origin',(11.0914213562373,-1.7145055188063E-16,
-13.84)) ;
#136277=CARTESIAN_POINT('Origin',(11.0914213562373,0.,-15.24)) ;
#136278=CARTESIAN_POINT('Origin',(12.7,0.,-15.24)) ;
#136279=CARTESIAN_POINT('',(12.8,-1.95943487863577E-16,-16.84)) ;
#136280=CARTESIAN_POINT('Origin',(12.8,0.,-15.24)) ;
#136281=CARTESIAN_POINT('',(12.7,-1.83697019872103E-16,-16.74)) ;
#136282=CARTESIAN_POINT('Origin',(12.7,-1.95943487863577E-16,-16.84)) ;
#136283=CARTESIAN_POINT('',(12.7,1.83697019872103E-16,-13.74)) ;
#136284=CARTESIAN_POINT('Origin',(12.7,0.,-15.24)) ;
#136285=CARTESIAN_POINT('Origin',(12.7,0.,-15.24)) ;
#136286=CARTESIAN_POINT('Origin',(12.7,2.1,-13.8580460421716)) ;
#136287=CARTESIAN_POINT('',(12.7,2.,-13.8580460421716)) ;
#136288=CARTESIAN_POINT('',(12.7,2.11643989873054,-13.7594066497884)) ;
#136289=CARTESIAN_POINT('Origin',(12.7,2.1,-13.8580460421716)) ;
#136290=CARTESIAN_POINT('',(12.8,2.13287979746107,-13.6607672574052)) ;
#136291=CARTESIAN_POINT('Origin',(12.7,2.13287979746107,-13.6607672574052)) ;
#136292=CARTESIAN_POINT('',(12.8,1.9,-13.8580460421716)) ;
#136293=CARTESIAN_POINT('Origin',(12.8,2.1,-13.8580460421716)) ;
#136294=CARTESIAN_POINT('Origin',(12.7,1.9,-13.8580460421716)) ;
#136295=CARTESIAN_POINT('Origin',(12.7,2.65,-13.7469539578284)) ;
#136296=CARTESIAN_POINT('',(12.7,2.63356010126947,-13.8455933502116)) ;
#136297=CARTESIAN_POINT('',(12.7,2.75,-13.7469539578284)) ;
#136298=CARTESIAN_POINT('Origin',(12.7,2.65,-13.7469539578284)) ;
#136299=CARTESIAN_POINT('',(12.8,2.65,-13.7469539578284)) ;
#136300=CARTESIAN_POINT('Origin',(12.7,2.65,-13.7469539578284)) ;
#136301=CARTESIAN_POINT('Origin',(12.7,2.65,-13.7469539578284)) ;
#136302=CARTESIAN_POINT('Origin',(4.5,2.1,-13.8580460421716)) ;
#136303=CARTESIAN_POINT('',(4.6,2.,-13.8580460421716)) ;
#136304=CARTESIAN_POINT('',(12.8,2.,-13.8580460421716)) ;
#136305=CARTESIAN_POINT('',(4.6,2.11643989873054,-13.7594066497884)) ;
#136306=CARTESIAN_POINT('Origin',(4.6,2.1,-13.8580460421716)) ;
#136307=CARTESIAN_POINT('',(4.5,2.11643989873054,-13.7594066497884)) ;
#136308=CARTESIAN_POINT('Origin',(12.7,2.65,-16.7330460421716)) ;
#136309=CARTESIAN_POINT('',(12.8,2.65,-16.7330460421716)) ;
#136310=CARTESIAN_POINT('',(12.7,2.63356010126947,-16.6344066497884)) ;
#136311=CARTESIAN_POINT('Origin',(12.7,2.65,-16.7330460421716)) ;
#136312=CARTESIAN_POINT('',(12.7,2.75,-16.7330460421716)) ;
#136313=CARTESIAN_POINT('Origin',(12.7,2.65,-16.7330460421716)) ;
#136314=CARTESIAN_POINT('Origin',(12.7,2.65,-16.7330460421716)) ;
#136315=CARTESIAN_POINT('Origin',(11.05,0.,-15.24)) ;
#136316=CARTESIAN_POINT('',(10.3,-9.18485099360511E-17,-14.49)) ;
#136317=CARTESIAN_POINT('Origin',(10.3,0.,-15.24)) ;
#136318=CARTESIAN_POINT('',(11.05,-1.83697019872103E-16,-13.74)) ;
#136319=CARTESIAN_POINT('Origin',(11.05,0.,-15.24)) ;
#136320=CARTESIAN_POINT('',(11.05,-1.83697019872103E-16,-13.74)) ;
#136321=CARTESIAN_POINT('Origin',(0.,9.95,-15.24)) ;
#136322=CARTESIAN_POINT('',(0.218101234104781,9.95,-17.1274405558009)) ;
#136323=CARTESIAN_POINT('',(-2.32682891837997E-16,9.95,-17.14)) ;
#136324=CARTESIAN_POINT('Origin',(0.,9.95,-15.24)) ;
#136325=CARTESIAN_POINT('',(0.321518176280636,9.85,-17.1125987456797)) ;
#136326=CARTESIAN_POINT('Ctrl Pts',(0.21810123410477,9.95,-17.1274405558009)) ;
#136327=CARTESIAN_POINT('Ctrl Pts',(0.231193919344567,9.95,-17.1259276441493)) ;
#136328=CARTESIAN_POINT('Ctrl Pts',(0.245192892440011,9.94751445938575,
-17.1241565825739)) ;
#136329=CARTESIAN_POINT('Ctrl Pts',(0.270990685773149,9.93716996065971,
-17.1206215789467)) ;
#136330=CARTESIAN_POINT('Ctrl Pts',(0.282791986325031,9.92931613918426,
-17.1188607093668)) ;
#136331=CARTESIAN_POINT('Ctrl Pts',(0.300953024019383,9.91135900604096,
-17.1160350266619)) ;
#136332=CARTESIAN_POINT('Ctrl Pts',(0.308688523153902,9.90025653083842,
-17.114762561801)) ;
#136333=CARTESIAN_POINT('Ctrl Pts',(0.318969164829191,9.87583423571802,
-17.1130429866749)) ;
#136334=CARTESIAN_POINT('Ctrl Pts',(0.321518176280625,9.86251584266313,
-17.1125987456797)) ;
#136335=CARTESIAN_POINT('Ctrl Pts',(0.321518176280625,9.85,-17.1125987456797)) ;
#136336=CARTESIAN_POINT('',(0.321518176280636,9.05,-17.1125987456797)) ;
#136337=CARTESIAN_POINT('',(0.321518176280636,8.95,-17.1125987456797)) ;
#136338=CARTESIAN_POINT('',(0.422455466606969,8.95,-17.0924393050067)) ;
#136339=CARTESIAN_POINT('Ctrl Pts',(0.321518176280627,9.05,-17.1125987456797)) ;
#136340=CARTESIAN_POINT('Ctrl Pts',(0.321518176280627,9.03744936090869,
-17.1125987456797)) ;
#136341=CARTESIAN_POINT('Ctrl Pts',(0.324085473150902,9.02409774280079,
-17.1121645622427)) ;
#136342=CARTESIAN_POINT('Ctrl Pts',(0.334387313650431,8.99960748025859,
-17.1103498579077)) ;
#136343=CARTESIAN_POINT('Ctrl Pts',(0.34212249945656,8.98846937989492,-17.1089656420615)) ;
#136344=CARTESIAN_POINT('Ctrl Pts',(0.360004521225388,8.97064401154629,
-17.1056049780795)) ;
#136345=CARTESIAN_POINT('Ctrl Pts',(0.371447108749463,8.96285745107738,
-17.1033820840476)) ;
#136346=CARTESIAN_POINT('Ctrl Pts',(0.39637397952969,8.95253508546271,-17.0982373032789)) ;
#136347=CARTESIAN_POINT('Ctrl Pts',(0.409857901997321,8.95,-17.0953122250646)) ;
#136348=CARTESIAN_POINT('Ctrl Pts',(0.422455466606959,8.95,-17.0924393050067)) ;
#136349=CARTESIAN_POINT('',(1.14750169623629,8.95,-16.7543446956142)) ;
#136350=CARTESIAN_POINT('Origin',(0.,8.95,-15.24)) ;
#136351=CARTESIAN_POINT('',(1.22782596331729,9.05,-16.689980483939)) ;
#136352=CARTESIAN_POINT('Ctrl Pts',(1.1475016962363,8.95,-16.7543446956142)) ;
#136353=CARTESIAN_POINT('Ctrl Pts',(1.15780003912543,8.95,-16.7465410786649)) ;
#136354=CARTESIAN_POINT('Ctrl Pts',(1.16870807732935,8.95253508546271,-16.7380919988207)) ;
#136355=CARTESIAN_POINT('Ctrl Pts',(1.18867189173409,8.96285745107738,-16.7223039093078)) ;
#136356=CARTESIAN_POINT('Ctrl Pts',(1.19772988083811,8.97064401154629,-16.7149672274615)) ;
#136357=CARTESIAN_POINT('Ctrl Pts',(1.21179864083582,8.98846937989492,-16.7034289972216)) ;
#136358=CARTESIAN_POINT('Ctrl Pts',(1.21783109328768,8.99960748025859,-16.6983932579134)) ;
#136359=CARTESIAN_POINT('Ctrl Pts',(1.22584313288947,9.02409774280079,-16.6916680597067)) ;
#136360=CARTESIAN_POINT('Ctrl Pts',(1.22782596331729,9.03744936090869,-16.689980483939)) ;
#136361=CARTESIAN_POINT('Ctrl Pts',(1.22782596331729,9.05,-16.689980483939)) ;
#136362=CARTESIAN_POINT('',(1.22782596331729,9.85,-16.689980483939)) ;
#136363=CARTESIAN_POINT('',(1.22782596331729,8.95,-16.689980483939)) ;
#136364=CARTESIAN_POINT('',(1.30567057854876,9.95,-16.6202986417121)) ;
#136365=CARTESIAN_POINT('Ctrl Pts',(1.2278259633173,9.85,-16.689980483939)) ;
#136366=CARTESIAN_POINT('Ctrl Pts',(1.2278259633173,9.85579162428539,-16.689980483939)) ;
#136367=CARTESIAN_POINT('Ctrl Pts',(1.22822745887819,9.86162764920013,-16.6896405714653)) ;
#136368=CARTESIAN_POINT('Ctrl Pts',(1.22902753823172,9.86736607146311,-16.6889619546779)) ;
#136369=CARTESIAN_POINT('Ctrl Pts',(1.22973095933686,9.87241123018667,-16.6883653221458)) ;
#136370=CARTESIAN_POINT('Ctrl Pts',(1.23074168751921,9.87738020477702,-16.6875074302535)) ;
#136371=CARTESIAN_POINT('Ctrl Pts',(1.23203099150183,9.88218322835582,-16.6864092214793)) ;
#136372=CARTESIAN_POINT('Ctrl Pts',(1.23351897101726,9.88772637473068,-16.6851417840233)) ;
#136373=CARTESIAN_POINT('Ctrl Pts',(1.2354014557903,9.89313280655104,-16.6835343365783)) ;
#136374=CARTESIAN_POINT('Ctrl Pts',(1.23763252770622,9.89827011881554,-16.6816189827484)) ;
#136375=CARTESIAN_POINT('Ctrl Pts',(1.23953000874363,9.90263929783464,-16.6799900134865)) ;
#136376=CARTESIAN_POINT('Ctrl Pts',(1.24167862345461,9.90681364346946,-16.6781390311988)) ;
#136377=CARTESIAN_POINT('Ctrl Pts',(1.24403025306867,9.91072825704925,-16.6761019216791)) ;
#136378=CARTESIAN_POINT('Ctrl Pts',(1.24687926059923,9.91547082513965,-16.6736339563467)) ;
#136379=CARTESIAN_POINT('Ctrl Pts',(1.25006974298106,9.91990270163234,-16.6708551265321)) ;
#136380=CARTESIAN_POINT('Ctrl Pts',(1.2535194093265,9.92391762881321,-16.6678266146309)) ;
#136381=CARTESIAN_POINT('Ctrl Pts',(1.25634620505522,9.92720762206749,-16.665344929839)) ;
#136382=CARTESIAN_POINT('Ctrl Pts',(1.25934609941473,9.93021806933732,-16.6626963101588)) ;
#136383=CARTESIAN_POINT('Ctrl Pts',(1.26246241000316,9.93291206679729,-16.6599255837293)) ;
#136384=CARTESIAN_POINT('Ctrl Pts',(1.26649145911189,9.93639511117203,-16.6563433371803)) ;
#136385=CARTESIAN_POINT('Ctrl Pts',(1.27077652588474,9.93940081548805,-16.6525022625241)) ;
#136386=CARTESIAN_POINT('Ctrl Pts',(1.27520851369617,9.94185862744775,-16.6484896739102)) ;
#136387=CARTESIAN_POINT('Ctrl Pts',(1.27864718185097,9.94376558208659,-16.6453764070711)) ;
#136388=CARTESIAN_POINT('Ctrl Pts',(1.28217366418729,9.94534362661778,-16.6421604997622)) ;
#136389=CARTESIAN_POINT('Ctrl Pts',(1.28573335778226,9.94658081625577,-16.6388887492202)) ;
#136390=CARTESIAN_POINT('Ctrl Pts',(1.29026904082682,9.94815721599755,-16.6347199568611)) ;
#136391=CARTESIAN_POINT('Ctrl Pts',(1.29492021413416,9.9491996901822,-16.6304036518226)) ;
#136392=CARTESIAN_POINT('Ctrl Pts',(1.29957290046268,9.9496832238817,-16.6260412243875)) ;
#136393=CARTESIAN_POINT('Ctrl Pts',(1.30160833994481,9.94989475836166,-16.6241327662598)) ;
#136394=CARTESIAN_POINT('Ctrl Pts',(1.30364403319568,9.95,-16.6222156186355)) ;
#136395=CARTESIAN_POINT('Ctrl Pts',(1.30567057854874,9.95,-16.6202986417121)) ;
#136396=CARTESIAN_POINT('',(-0.218101234104782,9.95,-13.3525594441991)) ;
#136397=CARTESIAN_POINT('Origin',(0.,9.95,-15.24)) ;
#136398=CARTESIAN_POINT('',(-0.321518176280637,9.85,-13.3674012543203)) ;
#136399=CARTESIAN_POINT('Ctrl Pts',(-0.218101234104768,9.95,-13.3525594441991)) ;
#136400=CARTESIAN_POINT('Ctrl Pts',(-0.231193919344566,9.95,-13.3540723558507)) ;
#136401=CARTESIAN_POINT('Ctrl Pts',(-0.245192892440009,9.94751445938575,
-13.3558434174261)) ;
#136402=CARTESIAN_POINT('Ctrl Pts',(-0.270990685773146,9.93716996065971,
-13.3593784210533)) ;
#136403=CARTESIAN_POINT('Ctrl Pts',(-0.282791986325029,9.92931613918426,
-13.3611392906332)) ;
#136404=CARTESIAN_POINT('Ctrl Pts',(-0.300953024019382,9.91135900604096,
-13.3639649733381)) ;
#136405=CARTESIAN_POINT('Ctrl Pts',(-0.308688523153901,9.90025653083842,
-13.365237438199)) ;
#136406=CARTESIAN_POINT('Ctrl Pts',(-0.31896916482919,9.87583423571802,
-13.3669570133251)) ;
#136407=CARTESIAN_POINT('Ctrl Pts',(-0.321518176280622,9.86251584266313,
-13.3674012543203)) ;
#136408=CARTESIAN_POINT('Ctrl Pts',(-0.321518176280622,9.85,-13.3674012543203)) ;
#136409=CARTESIAN_POINT('',(-0.321518176280637,9.05,-13.3674012543203)) ;
#136410=CARTESIAN_POINT('',(-0.321518176280637,8.95,-13.3674012543203)) ;
#136411=CARTESIAN_POINT('',(-0.422455466606969,8.95,-13.3875606949933)) ;
#136412=CARTESIAN_POINT('Ctrl Pts',(-0.321518176280627,9.05,-13.3674012543203)) ;
#136413=CARTESIAN_POINT('Ctrl Pts',(-0.321518176280627,9.03744936090869,
-13.3674012543203)) ;
#136414=CARTESIAN_POINT('Ctrl Pts',(-0.324085473150903,9.02409774280079,
-13.3678354377573)) ;
#136415=CARTESIAN_POINT('Ctrl Pts',(-0.334387313650432,8.99960748025859,
-13.3696501420923)) ;
#136416=CARTESIAN_POINT('Ctrl Pts',(-0.342122499456561,8.98846937989492,
-13.3710343579385)) ;
#136417=CARTESIAN_POINT('Ctrl Pts',(-0.360004521225389,8.97064401154629,
-13.3743950219205)) ;
#136418=CARTESIAN_POINT('Ctrl Pts',(-0.371447108749464,8.96285745107738,
-13.3766179159524)) ;
#136419=CARTESIAN_POINT('Ctrl Pts',(-0.396373979529691,8.95253508546271,
-13.3817626967211)) ;
#136420=CARTESIAN_POINT('Ctrl Pts',(-0.409857901997322,8.95,-13.3846877749354)) ;
#136421=CARTESIAN_POINT('Ctrl Pts',(-0.42245546660696,8.95,-13.3875606949933)) ;
#136422=CARTESIAN_POINT('',(-1.14750169623629,8.95,-13.7256553043858)) ;
#136423=CARTESIAN_POINT('Origin',(0.,8.95,-15.24)) ;
#136424=CARTESIAN_POINT('',(-1.22782596331729,9.05,-13.790019516061)) ;
#136425=CARTESIAN_POINT('Ctrl Pts',(-1.1475016962363,8.95,-13.7256553043858)) ;
#136426=CARTESIAN_POINT('Ctrl Pts',(-1.15780003912543,8.95,-13.7334589213351)) ;
#136427=CARTESIAN_POINT('Ctrl Pts',(-1.16870807732935,8.95253508546271,
-13.7419080011793)) ;
#136428=CARTESIAN_POINT('Ctrl Pts',(-1.18867189173409,8.96285745107738,
-13.7576960906922)) ;
#136429=CARTESIAN_POINT('Ctrl Pts',(-1.19772988083812,8.97064401154629,
-13.7650327725385)) ;
#136430=CARTESIAN_POINT('Ctrl Pts',(-1.21179864083582,8.98846937989492,
-13.7765710027784)) ;
#136431=CARTESIAN_POINT('Ctrl Pts',(-1.21783109328768,8.99960748025859,
-13.7816067420866)) ;
#136432=CARTESIAN_POINT('Ctrl Pts',(-1.22584313288947,9.02409774280079,
-13.7883319402933)) ;
#136433=CARTESIAN_POINT('Ctrl Pts',(-1.22782596331729,9.03744936090869,
-13.790019516061)) ;
#136434=CARTESIAN_POINT('Ctrl Pts',(-1.22782596331729,9.05,-13.790019516061)) ;
#136435=CARTESIAN_POINT('',(-1.22782596331729,9.85,-13.790019516061)) ;
#136436=CARTESIAN_POINT('',(-1.22782596331729,8.95,-13.790019516061)) ;
#136437=CARTESIAN_POINT('',(-1.30567057854876,9.95,-13.8597013582879)) ;
#136438=CARTESIAN_POINT('Ctrl Pts',(-1.2278259633173,9.85,-13.790019516061)) ;
#136439=CARTESIAN_POINT('Ctrl Pts',(-1.2278259633173,9.85579162428539,-13.790019516061)) ;
#136440=CARTESIAN_POINT('Ctrl Pts',(-1.22822745887819,9.86162764920014,
-13.7903594285347)) ;
#136441=CARTESIAN_POINT('Ctrl Pts',(-1.22902753823172,9.86736607146313,
-13.7910380453221)) ;
#136442=CARTESIAN_POINT('Ctrl Pts',(-1.22973095933686,9.87241123018668,
-13.7916346778542)) ;
#136443=CARTESIAN_POINT('Ctrl Pts',(-1.23074168751921,9.87738020477702,
-13.7924925697465)) ;
#136444=CARTESIAN_POINT('Ctrl Pts',(-1.23203099150183,9.88218322835582,
-13.7935907785207)) ;
#136445=CARTESIAN_POINT('Ctrl Pts',(-1.23351897101726,9.88772637473068,
-13.7948582159767)) ;
#136446=CARTESIAN_POINT('Ctrl Pts',(-1.23540145579029,9.89313280655104,
-13.7964656634217)) ;
#136447=CARTESIAN_POINT('Ctrl Pts',(-1.23763252770621,9.89827011881554,
-13.7983810172516)) ;
#136448=CARTESIAN_POINT('Ctrl Pts',(-1.23953000874362,9.90263929783464,
-13.8000099865135)) ;
#136449=CARTESIAN_POINT('Ctrl Pts',(-1.24167862345461,9.90681364346945,
-13.8018609688012)) ;
#136450=CARTESIAN_POINT('Ctrl Pts',(-1.24403025306867,9.91072825704925,
-13.8038980783209)) ;
#136451=CARTESIAN_POINT('Ctrl Pts',(-1.24687926059924,9.91547082513966,
-13.8063660436533)) ;
#136452=CARTESIAN_POINT('Ctrl Pts',(-1.25006974298107,9.91990270163235,
-13.8091448734679)) ;
#136453=CARTESIAN_POINT('Ctrl Pts',(-1.25351940932651,9.92391762881324,
-13.8121733853692)) ;
#136454=CARTESIAN_POINT('Ctrl Pts',(-1.25634620505522,9.92720762206753,
-13.8146550701611)) ;
#136455=CARTESIAN_POINT('Ctrl Pts',(-1.25934609941473,9.93021806933732,
-13.8173036898412)) ;
#136456=CARTESIAN_POINT('Ctrl Pts',(-1.26246241000317,9.93291206679729,
-13.8200744162707)) ;
#136457=CARTESIAN_POINT('Ctrl Pts',(-1.26649145911189,9.93639511117203,
-13.8236566628197)) ;
#136458=CARTESIAN_POINT('Ctrl Pts',(-1.27077652588473,9.93940081548805,
-13.827497737476)) ;
#136459=CARTESIAN_POINT('Ctrl Pts',(-1.27520851369616,9.94185862744775,
-13.8315103260898)) ;
#136460=CARTESIAN_POINT('Ctrl Pts',(-1.27864718185096,9.94376558208659,
-13.8346235929289)) ;
#136461=CARTESIAN_POINT('Ctrl Pts',(-1.28217366418729,9.94534362661778,
-13.8378395002378)) ;
#136462=CARTESIAN_POINT('Ctrl Pts',(-1.28573335778226,9.94658081625577,
-13.8411112507798)) ;
#136463=CARTESIAN_POINT('Ctrl Pts',(-1.29026904082682,9.94815721599755,
-13.8452800431389)) ;
#136464=CARTESIAN_POINT('Ctrl Pts',(-1.29492021413416,9.9491996901822,-13.8495963481774)) ;
#136465=CARTESIAN_POINT('Ctrl Pts',(-1.29957290046264,9.9496832238817,-13.8539587756125)) ;
#136466=CARTESIAN_POINT('Ctrl Pts',(-1.30160833994476,9.94989475836165,
-13.8558672337401)) ;
#136467=CARTESIAN_POINT('Ctrl Pts',(-1.30364403319568,9.95,-13.8577843813645)) ;
#136468=CARTESIAN_POINT('Ctrl Pts',(-1.30567057854874,9.95,-13.8597013582879)) ;
#136469=CARTESIAN_POINT('Origin',(0.,9.95,-15.24)) ;
#136470=CARTESIAN_POINT('',(-2.32682891837997E-16,9.95,-17.14)) ;
#136471=CARTESIAN_POINT('Origin',(4.6,2.65,-21.8130460421716)) ;
#136472=CARTESIAN_POINT('',(4.5,2.61712020253893,-21.6157672574052)) ;
#136473=CARTESIAN_POINT('',(4.5,2.72431432344521,-21.627365183355)) ;
#136474=CARTESIAN_POINT('Origin',(4.5,2.65,-21.8130460421716)) ;
#136475=CARTESIAN_POINT('',(4.6,2.63356010126946,-21.7144066497884)) ;
#136476=CARTESIAN_POINT('Origin',(4.6,2.61712020253893,-21.6157672574052)) ;
#136477=CARTESIAN_POINT('',(4.6,2.68715716172261,-21.7202056127633)) ;
#136478=CARTESIAN_POINT('Origin',(4.6,2.65,-21.8130460421716)) ;
#136479=CARTESIAN_POINT('Origin',(4.6,2.72431432344521,-21.627365183355)) ;
#136480=CARTESIAN_POINT('Origin',(-4.52198039027186,10.1,-17.78)) ;
#136481=CARTESIAN_POINT('',(-4.42392232270277,10.0803883864862,-22.86)) ;
#136482=CARTESIAN_POINT('',(-4.52198039027186,10.2,-22.86)) ;
#136483=CARTESIAN_POINT('Origin',(-4.52198039027186,10.1,-22.86)) ;
#136484=CARTESIAN_POINT('',(-4.42392232270277,10.0803883864862,-12.7)) ;
#136485=CARTESIAN_POINT('',(-4.42392232270277,10.0803883864862,-22.86)) ;
#136486=CARTESIAN_POINT('',(-4.52198039027186,10.2,-12.7)) ;
#136487=CARTESIAN_POINT('Origin',(-4.52198039027186,10.1,-12.7)) ;
#136488=CARTESIAN_POINT('',(-4.52198039027186,10.2,-17.78)) ;
#136489=CARTESIAN_POINT('Origin',(0.,10.85,-20.32)) ;
#136490=CARTESIAN_POINT('',(-2.44929359829471E-16,10.95,-18.32)) ;
#136491=CARTESIAN_POINT('Origin',(0.,10.95,-20.32)) ;
#136492=CARTESIAN_POINT('',(-2.32682891837997E-16,10.85,-18.42)) ;
#136493=CARTESIAN_POINT('Origin',(-2.44929359829471E-16,10.85,-18.32)) ;
#136494=CARTESIAN_POINT('',(2.32682891837997E-16,10.85,-22.22)) ;
#136495=CARTESIAN_POINT('Origin',(0.,10.85,-20.32)) ;
#136496=CARTESIAN_POINT('Origin',(0.,10.85,-20.32)) ;
#136497=CARTESIAN_POINT('Origin',(11.0914213562373,0.,-20.32)) ;
#136498=CARTESIAN_POINT('',(11.0207106781187,-1.80110112442985E-16,-18.8492893218813)) ;
#136499=CARTESIAN_POINT('Origin',(11.0207106781187,0.,-20.32)) ;
#136500=CARTESIAN_POINT('',(11.0914213562373,-1.83697019872103E-16,-18.82)) ;
#136501=CARTESIAN_POINT('Origin',(11.0914213562373,-1.7145055188063E-16,
-18.92)) ;
#136502=CARTESIAN_POINT('Origin',(11.0914213562373,0.,-20.32)) ;
#136503=CARTESIAN_POINT('Origin',(12.7,0.,-20.32)) ;
#136504=CARTESIAN_POINT('',(12.8,-1.95943487863577E-16,-21.92)) ;
#136505=CARTESIAN_POINT('Origin',(12.8,0.,-20.32)) ;
#136506=CARTESIAN_POINT('',(12.7,-1.83697019872103E-16,-21.82)) ;
#136507=CARTESIAN_POINT('Origin',(12.7,-1.95943487863577E-16,-21.92)) ;
#136508=CARTESIAN_POINT('',(12.7,1.83697019872103E-16,-18.82)) ;
#136509=CARTESIAN_POINT('Origin',(12.7,0.,-20.32)) ;
#136510=CARTESIAN_POINT('Origin',(12.7,0.,-20.32)) ;
#136511=CARTESIAN_POINT('Origin',(12.7,2.1,-18.9380460421716)) ;
#136512=CARTESIAN_POINT('',(12.7,2.,-18.9380460421716)) ;
#136513=CARTESIAN_POINT('',(12.7,2.11643989873054,-18.8394066497884)) ;
#136514=CARTESIAN_POINT('Origin',(12.7,2.1,-18.9380460421716)) ;
#136515=CARTESIAN_POINT('',(12.8,2.13287979746107,-18.7407672574052)) ;
#136516=CARTESIAN_POINT('Origin',(12.7,2.13287979746107,-18.7407672574052)) ;
#136517=CARTESIAN_POINT('',(12.8,1.9,-18.9380460421716)) ;
#136518=CARTESIAN_POINT('Origin',(12.8,2.1,-18.9380460421716)) ;
#136519=CARTESIAN_POINT('Origin',(12.7,1.9,-18.9380460421716)) ;
#136520=CARTESIAN_POINT('Origin',(12.7,2.65,-18.8269539578284)) ;
#136521=CARTESIAN_POINT('',(12.7,2.63356010126947,-18.9255933502116)) ;
#136522=CARTESIAN_POINT('',(12.7,2.75,-18.8269539578284)) ;
#136523=CARTESIAN_POINT('Origin',(12.7,2.65,-18.8269539578284)) ;
#136524=CARTESIAN_POINT('',(12.8,2.65,-18.8269539578284)) ;
#136525=CARTESIAN_POINT('Origin',(12.7,2.65,-18.8269539578284)) ;
#136526=CARTESIAN_POINT('Origin',(12.7,2.65,-18.8269539578284)) ;
#136527=CARTESIAN_POINT('Origin',(4.5,2.1,-18.9380460421716)) ;
#136528=CARTESIAN_POINT('',(4.6,2.,-18.9380460421716)) ;
#136529=CARTESIAN_POINT('',(12.8,2.,-18.9380460421716)) ;
#136530=CARTESIAN_POINT('',(4.6,2.11643989873054,-18.8394066497884)) ;
#136531=CARTESIAN_POINT('Origin',(4.6,2.1,-18.9380460421716)) ;
#136532=CARTESIAN_POINT('',(4.5,2.11643989873054,-18.8394066497884)) ;
#136533=CARTESIAN_POINT('Origin',(12.7,2.65,-21.8130460421716)) ;
#136534=CARTESIAN_POINT('',(12.8,2.65,-21.8130460421716)) ;
#136535=CARTESIAN_POINT('',(12.7,2.63356010126947,-21.7144066497884)) ;
#136536=CARTESIAN_POINT('Origin',(12.7,2.65,-21.8130460421716)) ;
#136537=CARTESIAN_POINT('',(12.7,2.75,-21.8130460421716)) ;
#136538=CARTESIAN_POINT('Origin',(12.7,2.65,-21.8130460421716)) ;
#136539=CARTESIAN_POINT('Origin',(12.7,2.65,-21.8130460421716)) ;
#136540=CARTESIAN_POINT('Origin',(11.05,0.,-20.32)) ;
#136541=CARTESIAN_POINT('',(10.3,-9.1848509936051E-17,-19.57)) ;
#136542=CARTESIAN_POINT('Origin',(10.3,0.,-20.32)) ;
#136543=CARTESIAN_POINT('',(11.05,-1.83697019872103E-16,-18.82)) ;
#136544=CARTESIAN_POINT('Origin',(11.05,0.,-20.32)) ;
#136545=CARTESIAN_POINT('',(11.05,-1.83697019872103E-16,-18.82)) ;
#136546=CARTESIAN_POINT('Origin',(0.,9.95,-20.32)) ;
#136547=CARTESIAN_POINT('',(0.218101234104781,9.95,-22.2074405558009)) ;
#136548=CARTESIAN_POINT('',(-2.32682891837997E-16,9.95,-22.22)) ;
#136549=CARTESIAN_POINT('Origin',(0.,9.95,-20.32)) ;
#136550=CARTESIAN_POINT('',(0.321518176280636,9.85,-22.1925987456797)) ;
#136551=CARTESIAN_POINT('Ctrl Pts',(0.21810123410477,9.95,-22.2074405558009)) ;
#136552=CARTESIAN_POINT('Ctrl Pts',(0.231193919344568,9.95,-22.2059276441493)) ;
#136553=CARTESIAN_POINT('Ctrl Pts',(0.245192892440011,9.94751445938575,
-22.2041565825739)) ;
#136554=CARTESIAN_POINT('Ctrl Pts',(0.270990685773149,9.93716996065971,
-22.2006215789467)) ;
#136555=CARTESIAN_POINT('Ctrl Pts',(0.282791986325031,9.92931613918426,
-22.1988607093667)) ;
#136556=CARTESIAN_POINT('Ctrl Pts',(0.300953024019383,9.91135900604096,
-22.1960350266619)) ;
#136557=CARTESIAN_POINT('Ctrl Pts',(0.308688523153903,9.90025653083842,
-22.1947625618009)) ;
#136558=CARTESIAN_POINT('Ctrl Pts',(0.318969164829192,9.87583423571802,
-22.1930429866749)) ;
#136559=CARTESIAN_POINT('Ctrl Pts',(0.321518176280625,9.86251584266313,
-22.1925987456797)) ;
#136560=CARTESIAN_POINT('Ctrl Pts',(0.321518176280625,9.85,-22.1925987456797)) ;
#136561=CARTESIAN_POINT('',(0.321518176280636,9.05,-22.1925987456797)) ;
#136562=CARTESIAN_POINT('',(0.321518176280636,8.95,-22.1925987456797)) ;
#136563=CARTESIAN_POINT('',(0.422455466606969,8.95,-22.1724393050068)) ;
#136564=CARTESIAN_POINT('Ctrl Pts',(0.321518176280626,9.05,-22.1925987456797)) ;
#136565=CARTESIAN_POINT('Ctrl Pts',(0.321518176280626,9.03744936090869,
-22.1925987456797)) ;
#136566=CARTESIAN_POINT('Ctrl Pts',(0.324085473150903,9.02409774280079,
-22.1921645622427)) ;
#136567=CARTESIAN_POINT('Ctrl Pts',(0.334387313650432,8.99960748025859,
-22.1903498579077)) ;
#136568=CARTESIAN_POINT('Ctrl Pts',(0.342122499456559,8.98846937989492,
-22.1889656420615)) ;
#136569=CARTESIAN_POINT('Ctrl Pts',(0.360004521225388,8.97064401154629,
-22.1856049780795)) ;
#136570=CARTESIAN_POINT('Ctrl Pts',(0.371447108749463,8.96285745107738,
-22.1833820840476)) ;
#136571=CARTESIAN_POINT('Ctrl Pts',(0.39637397952969,8.95253508546271,-22.1782373032789)) ;
#136572=CARTESIAN_POINT('Ctrl Pts',(0.409857901997322,8.95,-22.1753122250646)) ;
#136573=CARTESIAN_POINT('Ctrl Pts',(0.42245546660696,8.95,-22.1724393050068)) ;
#136574=CARTESIAN_POINT('',(1.14750169623629,8.95,-21.8343446956142)) ;
#136575=CARTESIAN_POINT('Origin',(0.,8.95,-20.32)) ;
#136576=CARTESIAN_POINT('',(1.22782596331729,9.05,-21.769980483939)) ;
#136577=CARTESIAN_POINT('Ctrl Pts',(1.1475016962363,8.95,-21.8343446956142)) ;
#136578=CARTESIAN_POINT('Ctrl Pts',(1.15780003912543,8.95,-21.8265410786649)) ;
#136579=CARTESIAN_POINT('Ctrl Pts',(1.16870807732935,8.95253508546271,-21.8180919988207)) ;
#136580=CARTESIAN_POINT('Ctrl Pts',(1.18867189173409,8.96285745107738,-21.8023039093078)) ;
#136581=CARTESIAN_POINT('Ctrl Pts',(1.19772988083812,8.97064401154629,-21.7949672274615)) ;
#136582=CARTESIAN_POINT('Ctrl Pts',(1.21179864083582,8.98846937989492,-21.7834289972216)) ;
#136583=CARTESIAN_POINT('Ctrl Pts',(1.21783109328768,8.99960748025859,-21.7783932579134)) ;
#136584=CARTESIAN_POINT('Ctrl Pts',(1.22584313288947,9.02409774280079,-21.7716680597067)) ;
#136585=CARTESIAN_POINT('Ctrl Pts',(1.22782596331729,9.03744936090869,-21.769980483939)) ;
#136586=CARTESIAN_POINT('Ctrl Pts',(1.22782596331729,9.05,-21.769980483939)) ;
#136587=CARTESIAN_POINT('',(1.22782596331729,9.85,-21.769980483939)) ;
#136588=CARTESIAN_POINT('',(1.22782596331729,8.95,-21.769980483939)) ;
#136589=CARTESIAN_POINT('',(1.30567057854876,9.95,-21.7002986417121)) ;
#136590=CARTESIAN_POINT('Ctrl Pts',(1.2278259633173,9.85,-21.769980483939)) ;
#136591=CARTESIAN_POINT('Ctrl Pts',(1.2278259633173,9.85579162428539,-21.769980483939)) ;
#136592=CARTESIAN_POINT('Ctrl Pts',(1.22822745887819,9.86162764920014,-21.7696405714653)) ;
#136593=CARTESIAN_POINT('Ctrl Pts',(1.22902753823172,9.86736607146312,-21.7689619546779)) ;
#136594=CARTESIAN_POINT('Ctrl Pts',(1.22973095933686,9.87241123018668,-21.7683653221458)) ;
#136595=CARTESIAN_POINT('Ctrl Pts',(1.23074168751921,9.87738020477702,-21.7675074302535)) ;
#136596=CARTESIAN_POINT('Ctrl Pts',(1.23203099150183,9.88218322835581,-21.7664092214793)) ;
#136597=CARTESIAN_POINT('Ctrl Pts',(1.23351897101726,9.88772637473068,-21.7651417840233)) ;
#136598=CARTESIAN_POINT('Ctrl Pts',(1.23540145579029,9.89313280655103,-21.7635343365783)) ;
#136599=CARTESIAN_POINT('Ctrl Pts',(1.23763252770622,9.89827011881554,-21.7616189827484)) ;
#136600=CARTESIAN_POINT('Ctrl Pts',(1.23953000874363,9.90263929783464,-21.7599900134865)) ;
#136601=CARTESIAN_POINT('Ctrl Pts',(1.24167862345461,9.90681364346946,-21.7581390311988)) ;
#136602=CARTESIAN_POINT('Ctrl Pts',(1.24403025306867,9.91072825704926,-21.7561019216791)) ;
#136603=CARTESIAN_POINT('Ctrl Pts',(1.24687926059923,9.91547082513965,-21.7536339563467)) ;
#136604=CARTESIAN_POINT('Ctrl Pts',(1.25006974298107,9.91990270163235,-21.7508551265321)) ;
#136605=CARTESIAN_POINT('Ctrl Pts',(1.2535194093265,9.92391762881322,-21.7478266146309)) ;
#136606=CARTESIAN_POINT('Ctrl Pts',(1.25634620505521,9.92720762206752,-21.7453449298389)) ;
#136607=CARTESIAN_POINT('Ctrl Pts',(1.25934609941473,9.93021806933731,-21.7426963101588)) ;
#136608=CARTESIAN_POINT('Ctrl Pts',(1.26246241000317,9.93291206679729,-21.7399255837293)) ;
#136609=CARTESIAN_POINT('Ctrl Pts',(1.26649145911189,9.93639511117203,-21.7363433371803)) ;
#136610=CARTESIAN_POINT('Ctrl Pts',(1.27077652588473,9.93940081548805,-21.732502262524)) ;
#136611=CARTESIAN_POINT('Ctrl Pts',(1.27520851369616,9.94185862744774,-21.7284896739102)) ;
#136612=CARTESIAN_POINT('Ctrl Pts',(1.27864718185096,9.94376558208659,-21.7253764070711)) ;
#136613=CARTESIAN_POINT('Ctrl Pts',(1.28217366418729,9.94534362661778,-21.7221604997622)) ;
#136614=CARTESIAN_POINT('Ctrl Pts',(1.28573335778226,9.94658081625576,-21.7188887492202)) ;
#136615=CARTESIAN_POINT('Ctrl Pts',(1.29026904082681,9.94815721599754,-21.7147199568612)) ;
#136616=CARTESIAN_POINT('Ctrl Pts',(1.29492021413415,9.9491996901822,-21.7104036518226)) ;
#136617=CARTESIAN_POINT('Ctrl Pts',(1.29957290046262,9.9496832238817,-21.7060412243876)) ;
#136618=CARTESIAN_POINT('Ctrl Pts',(1.30160833994475,9.94989475836165,-21.7041327662599)) ;
#136619=CARTESIAN_POINT('Ctrl Pts',(1.30364403319562,9.95,-21.7022156186355)) ;
#136620=CARTESIAN_POINT('Ctrl Pts',(1.30567057854874,9.95,-21.7002986417121)) ;
#136621=CARTESIAN_POINT('',(-0.218101234104782,9.95,-18.4325594441991)) ;
#136622=CARTESIAN_POINT('Origin',(0.,9.95,-20.32)) ;
#136623=CARTESIAN_POINT('',(-0.321518176280637,9.85,-18.4474012543203)) ;
#136624=CARTESIAN_POINT('Ctrl Pts',(-0.218101234104768,9.95,-18.4325594441991)) ;
#136625=CARTESIAN_POINT('Ctrl Pts',(-0.231193919344566,9.95,-18.4340723558507)) ;
#136626=CARTESIAN_POINT('Ctrl Pts',(-0.245192892440009,9.94751445938575,
-18.4358434174261)) ;
#136627=CARTESIAN_POINT('Ctrl Pts',(-0.270990685773147,9.93716996065971,
-18.4393784210533)) ;
#136628=CARTESIAN_POINT('Ctrl Pts',(-0.282791986325029,9.92931613918426,
-18.4411392906332)) ;
#136629=CARTESIAN_POINT('Ctrl Pts',(-0.300953024019382,9.91135900604096,
-18.4439649733381)) ;
#136630=CARTESIAN_POINT('Ctrl Pts',(-0.308688523153901,9.90025653083842,
-18.445237438199)) ;
#136631=CARTESIAN_POINT('Ctrl Pts',(-0.31896916482919,9.87583423571802,
-18.4469570133251)) ;
#136632=CARTESIAN_POINT('Ctrl Pts',(-0.321518176280622,9.86251584266313,
-18.4474012543203)) ;
#136633=CARTESIAN_POINT('Ctrl Pts',(-0.321518176280622,9.85,-18.4474012543203)) ;
#136634=CARTESIAN_POINT('',(-0.321518176280637,9.05,-18.4474012543203)) ;
#136635=CARTESIAN_POINT('',(-0.321518176280637,8.95,-18.4474012543203)) ;
#136636=CARTESIAN_POINT('',(-0.422455466606969,8.95,-18.4675606949933)) ;
#136637=CARTESIAN_POINT('Ctrl Pts',(-0.321518176280627,9.05,-18.4474012543203)) ;
#136638=CARTESIAN_POINT('Ctrl Pts',(-0.321518176280627,9.03744936090869,
-18.4474012543203)) ;
#136639=CARTESIAN_POINT('Ctrl Pts',(-0.324085473150904,9.02409774280079,
-18.4478354377573)) ;
#136640=CARTESIAN_POINT('Ctrl Pts',(-0.334387313650432,8.99960748025859,
-18.4496501420923)) ;
#136641=CARTESIAN_POINT('Ctrl Pts',(-0.34212249945656,8.98846937989492,
-18.4510343579385)) ;
#136642=CARTESIAN_POINT('Ctrl Pts',(-0.360004521225388,8.97064401154629,
-18.4543950219205)) ;
#136643=CARTESIAN_POINT('Ctrl Pts',(-0.371447108749464,8.96285745107739,
-18.4566179159524)) ;
#136644=CARTESIAN_POINT('Ctrl Pts',(-0.39637397952969,8.95253508546271,
-18.4617626967211)) ;
#136645=CARTESIAN_POINT('Ctrl Pts',(-0.409857901997323,8.95,-18.4646877749354)) ;
#136646=CARTESIAN_POINT('Ctrl Pts',(-0.42245546660696,8.95,-18.4675606949932)) ;
#136647=CARTESIAN_POINT('',(-1.14750169623629,8.95,-18.8056553043858)) ;
#136648=CARTESIAN_POINT('Origin',(0.,8.95,-20.32)) ;
#136649=CARTESIAN_POINT('',(-1.22782596331729,9.05,-18.870019516061)) ;
#136650=CARTESIAN_POINT('Ctrl Pts',(-1.1475016962363,8.95,-18.8056553043858)) ;
#136651=CARTESIAN_POINT('Ctrl Pts',(-1.15780003912543,8.95,-18.8134589213351)) ;
#136652=CARTESIAN_POINT('Ctrl Pts',(-1.16870807732935,8.95253508546271,
-18.8219080011793)) ;
#136653=CARTESIAN_POINT('Ctrl Pts',(-1.18867189173409,8.96285745107739,
-18.8376960906922)) ;
#136654=CARTESIAN_POINT('Ctrl Pts',(-1.19772988083812,8.97064401154629,
-18.8450327725385)) ;
#136655=CARTESIAN_POINT('Ctrl Pts',(-1.21179864083582,8.98846937989492,
-18.8565710027784)) ;
#136656=CARTESIAN_POINT('Ctrl Pts',(-1.21783109328768,8.99960748025859,
-18.8616067420866)) ;
#136657=CARTESIAN_POINT('Ctrl Pts',(-1.22584313288947,9.02409774280079,
-18.8683319402933)) ;
#136658=CARTESIAN_POINT('Ctrl Pts',(-1.22782596331729,9.03744936090869,
-18.870019516061)) ;
#136659=CARTESIAN_POINT('Ctrl Pts',(-1.22782596331729,9.05,-18.870019516061)) ;
#136660=CARTESIAN_POINT('',(-1.22782596331729,9.85,-18.870019516061)) ;
#136661=CARTESIAN_POINT('',(-1.22782596331729,8.95,-18.870019516061)) ;
#136662=CARTESIAN_POINT('',(-1.30567057854876,9.95,-18.9397013582879)) ;
#136663=CARTESIAN_POINT('Ctrl Pts',(-1.2278259633173,9.85,-18.870019516061)) ;
#136664=CARTESIAN_POINT('Ctrl Pts',(-1.2278259633173,9.85579162428539,-18.870019516061)) ;
#136665=CARTESIAN_POINT('Ctrl Pts',(-1.22822745887819,9.86162764920014,
-18.8703594285347)) ;
#136666=CARTESIAN_POINT('Ctrl Pts',(-1.22902753823172,9.86736607146313,
-18.8710380453221)) ;
#136667=CARTESIAN_POINT('Ctrl Pts',(-1.22973095933686,9.87241123018668,
-18.8716346778542)) ;
#136668=CARTESIAN_POINT('Ctrl Pts',(-1.23074168751921,9.87738020477702,
-18.8724925697465)) ;
#136669=CARTESIAN_POINT('Ctrl Pts',(-1.23203099150183,9.88218322835581,
-18.8735907785207)) ;
#136670=CARTESIAN_POINT('Ctrl Pts',(-1.23351897101725,9.88772637473067,
-18.8748582159767)) ;
#136671=CARTESIAN_POINT('Ctrl Pts',(-1.23540145579029,9.89313280655104,
-18.8764656634217)) ;
#136672=CARTESIAN_POINT('Ctrl Pts',(-1.23763252770621,9.89827011881553,
-18.8783810172516)) ;
#136673=CARTESIAN_POINT('Ctrl Pts',(-1.23953000874362,9.90263929783464,
-18.8800099865135)) ;
#136674=CARTESIAN_POINT('Ctrl Pts',(-1.24167862345461,9.90681364346945,
-18.8818609688012)) ;
#136675=CARTESIAN_POINT('Ctrl Pts',(-1.24403025306867,9.91072825704926,
-18.8838980783209)) ;
#136676=CARTESIAN_POINT('Ctrl Pts',(-1.24687926059923,9.91547082513966,
-18.8863660436533)) ;
#136677=CARTESIAN_POINT('Ctrl Pts',(-1.25006974298107,9.91990270163235,
-18.8891448734679)) ;
#136678=CARTESIAN_POINT('Ctrl Pts',(-1.2535194093265,9.92391762881323,-18.8921733853691)) ;
#136679=CARTESIAN_POINT('Ctrl Pts',(-1.25634620505522,9.92720762206752,
-18.8946550701611)) ;
#136680=CARTESIAN_POINT('Ctrl Pts',(-1.25934609941473,9.93021806933732,
-18.8973036898412)) ;
#136681=CARTESIAN_POINT('Ctrl Pts',(-1.26246241000317,9.93291206679729,
-18.9000744162707)) ;
#136682=CARTESIAN_POINT('Ctrl Pts',(-1.26649145911189,9.93639511117203,
-18.9036566628197)) ;
#136683=CARTESIAN_POINT('Ctrl Pts',(-1.27077652588473,9.93940081548805,
-18.907497737476)) ;
#136684=CARTESIAN_POINT('Ctrl Pts',(-1.27520851369617,9.94185862744775,
-18.9115103260898)) ;
#136685=CARTESIAN_POINT('Ctrl Pts',(-1.27864718185097,9.94376558208659,
-18.9146235929289)) ;
#136686=CARTESIAN_POINT('Ctrl Pts',(-1.28217366418729,9.94534362661778,
-18.9178395002378)) ;
#136687=CARTESIAN_POINT('Ctrl Pts',(-1.28573335778226,9.94658081625577,
-18.9211112507798)) ;
#136688=CARTESIAN_POINT('Ctrl Pts',(-1.29026904082681,9.94815721599754,
-18.9252800431388)) ;
#136689=CARTESIAN_POINT('Ctrl Pts',(-1.29492021413408,9.94919969018218,
-18.9295963481773)) ;
#136690=CARTESIAN_POINT('Ctrl Pts',(-1.29957290046257,9.94968322388169,
-18.9339587756124)) ;
#136691=CARTESIAN_POINT('Ctrl Pts',(-1.30160833994473,9.94989475836165,
-18.9358672337401)) ;
#136692=CARTESIAN_POINT('Ctrl Pts',(-1.30364403319561,9.95,-18.9377843813644)) ;
#136693=CARTESIAN_POINT('Ctrl Pts',(-1.30567057854874,9.95,-18.9397013582879)) ;
#136694=CARTESIAN_POINT('Origin',(0.,9.95,-20.32)) ;
#136695=CARTESIAN_POINT('',(-2.32682891837997E-16,9.95,-22.22)) ;
#136696=CARTESIAN_POINT('Origin',(3.95,3.75,-17.78)) ;
#136697=CARTESIAN_POINT('',(3.95,6.92431432344521,-22.86)) ;
#136698=CARTESIAN_POINT('',(3.95,6.92431432344521,-12.7)) ;
#136699=CARTESIAN_POINT('',(3.95,6.92431432344521,-17.78)) ;
#136700=CARTESIAN_POINT('',(3.95,3.77568567655479,-12.7)) ;
#136701=CARTESIAN_POINT('',(3.95,3.75,-12.7)) ;
#136702=CARTESIAN_POINT('',(3.95,3.77568567655479,-22.86)) ;
#136703=CARTESIAN_POINT('',(3.95,3.77568567655479,-22.86)) ;
#136704=CARTESIAN_POINT('',(3.95,3.75,-22.86)) ;
#136705=CARTESIAN_POINT('',(3.95,4.6,-17.345)) ;
#136706=CARTESIAN_POINT('',(3.95,4.4,-17.545)) ;
#136707=CARTESIAN_POINT('Origin',(3.95,4.6,-17.545)) ;
#136708=CARTESIAN_POINT('',(3.95,5.88396692803319,-17.345)) ;
#136709=CARTESIAN_POINT('',(3.95,3.75,-17.345)) ;
#136710=CARTESIAN_POINT('',(3.95,6.08618232569815,-17.545)) ;
#136711=CARTESIAN_POINT('Ctrl Pts',(3.95,6.08618232569815,-17.545)) ;
#136712=CARTESIAN_POINT('Ctrl Pts',(3.95,6.08618232225605,-17.4360574372282)) ;
#136713=CARTESIAN_POINT('Ctrl Pts',(3.95,5.9941162463882,-17.3450000032932)) ;
#136714=CARTESIAN_POINT('Ctrl Pts',(3.95,5.88396692803319,-17.345)) ;
#136715=CARTESIAN_POINT('',(3.95,6.08618232569815,-18.845)) ;
#136716=CARTESIAN_POINT('',(3.95,6.08618232569815,-17.78)) ;
#136717=CARTESIAN_POINT('',(3.95,5.88396692803319,-19.045)) ;
#136718=CARTESIAN_POINT('Ctrl Pts',(3.95,5.88396692803319,-19.045)) ;
#136719=CARTESIAN_POINT('Ctrl Pts',(3.95,5.9941162463882,-19.0449999967068)) ;
#136720=CARTESIAN_POINT('Ctrl Pts',(3.95,6.08618232225605,-18.9539425627718)) ;
#136721=CARTESIAN_POINT('Ctrl Pts',(3.95,6.08618232569815,-18.845)) ;
#136722=CARTESIAN_POINT('',(3.95,4.6,-19.045)) ;
#136723=CARTESIAN_POINT('',(3.95,4.5,-19.045)) ;
#136724=CARTESIAN_POINT('',(3.95,4.4,-18.845)) ;
#136725=CARTESIAN_POINT('Origin',(3.95,4.6,-18.845)) ;
#136726=CARTESIAN_POINT('',(3.95,4.4,-17.78)) ;
#136727=CARTESIAN_POINT('Origin',(3.4,7.95,-17.78)) ;
#136728=CARTESIAN_POINT('',(3.,7.95,-22.36)) ;
#136729=CARTESIAN_POINT('',(3.34087287789487,7.95,-22.36)) ;
#136730=CARTESIAN_POINT('',(3.4,7.95,-22.36)) ;
#136731=CARTESIAN_POINT('',(3.,7.95,-12.7)) ;
#136732=CARTESIAN_POINT('',(3.,7.95,-17.78)) ;
#136733=CARTESIAN_POINT('',(3.34087287789487,7.95,-12.7)) ;
#136734=CARTESIAN_POINT('',(3.4,7.95,-12.7)) ;
#136735=CARTESIAN_POINT('',(3.34087287789487,7.95,-17.78)) ;
#136736=CARTESIAN_POINT('Origin',(2.9,7.95,-17.78)) ;
#136737=CARTESIAN_POINT('',(2.9,9.85,-22.36)) ;
#136738=CARTESIAN_POINT('',(2.9,8.05,-22.36)) ;
#136739=CARTESIAN_POINT('',(2.9,7.825,-22.36)) ;
#136740=CARTESIAN_POINT('',(2.9,9.85,-12.7)) ;
#136741=CARTESIAN_POINT('',(2.9,9.85,-17.78)) ;
#136742=CARTESIAN_POINT('',(2.9,8.05,-12.7)) ;
#136743=CARTESIAN_POINT('',(2.9,7.95,-12.7)) ;
#136744=CARTESIAN_POINT('',(2.9,8.05,-22.86)) ;
#136745=CARTESIAN_POINT('Origin',(2.9,9.95,-17.78)) ;
#136746=CARTESIAN_POINT('',(3.3,9.95,-22.36)) ;
#136747=CARTESIAN_POINT('',(3.,9.95,-22.36)) ;
#136748=CARTESIAN_POINT('',(2.9,9.95,-22.36)) ;
#136749=CARTESIAN_POINT('',(3.3,9.95,-12.7)) ;
#136750=CARTESIAN_POINT('',(3.3,9.95,-17.78)) ;
#136751=CARTESIAN_POINT('',(3.,9.95,-12.7)) ;
#136752=CARTESIAN_POINT('',(2.9,9.95,-12.7)) ;
#136753=CARTESIAN_POINT('',(3.,9.95,-22.86)) ;
#136754=CARTESIAN_POINT('Origin',(3.3,10.05,-17.78)) ;
#136755=CARTESIAN_POINT('',(3.4,10.05,-22.36)) ;
#136756=CARTESIAN_POINT('Origin',(3.3,10.05,-22.36)) ;
#136757=CARTESIAN_POINT('',(3.4,10.05,-12.7)) ;
#136758=CARTESIAN_POINT('',(3.4,10.05,-17.78)) ;
#136759=CARTESIAN_POINT('Origin',(3.3,10.05,-12.7)) ;
#136760=CARTESIAN_POINT('Origin',(3.,9.85,-17.78)) ;
#136761=CARTESIAN_POINT('Origin',(3.,9.85,-22.36)) ;
#136762=CARTESIAN_POINT('Origin',(3.,9.85,-12.7)) ;
#136763=CARTESIAN_POINT('Origin',(3.,8.05,-17.78)) ;
#136764=CARTESIAN_POINT('Origin',(3.,8.05,-22.36)) ;
#136765=CARTESIAN_POINT('Origin',(3.,8.05,-12.7)) ;
#136766=CARTESIAN_POINT('Origin',(3.34087287789487,7.85,-17.78)) ;
#136767=CARTESIAN_POINT('',(3.4,7.93064727789309,-22.86)) ;
#136768=CARTESIAN_POINT('',(3.42849446876253,7.89819187497721,-22.86)) ;
#136769=CARTESIAN_POINT('Origin',(3.34087287789487,7.85,-22.86)) ;
#136770=CARTESIAN_POINT('',(3.4,7.93064727789309,-22.36)) ;
#136771=CARTESIAN_POINT('',(3.4,7.93064727789309,-17.78)) ;
#136772=CARTESIAN_POINT('Origin',(3.34087287789487,7.85,-22.36)) ;
#136773=CARTESIAN_POINT('',(3.42849446876253,7.89819187497721,-12.7)) ;
#136774=CARTESIAN_POINT('Origin',(3.34087287789487,7.85,-12.7)) ;
#136775=CARTESIAN_POINT('',(3.42849446876253,7.89819187497721,-17.78)) ;
#136776=CARTESIAN_POINT('Origin',(4.5,-2.8,-17.78)) ;
#136777=CARTESIAN_POINT('',(4.5,-2.4,-22.2821416870349)) ;
#136778=CARTESIAN_POINT('',(4.5,-2.7,-21.8431546211728)) ;
#136779=CARTESIAN_POINT('Origin',(4.5,0.,-20.32)) ;
#136780=CARTESIAN_POINT('',(4.5,-2.7,-22.86)) ;
#136781=CARTESIAN_POINT('',(4.5,-2.7,-17.78)) ;
#136782=CARTESIAN_POINT('',(4.5,-2.4,-22.86)) ;
#136783=CARTESIAN_POINT('',(4.5,-2.8,-22.86)) ;
#136784=CARTESIAN_POINT('',(4.5,-2.4,-22.2461360284258)) ;
#136785=CARTESIAN_POINT('Origin',(4.5,-2.3,-17.78)) ;
#136786=CARTESIAN_POINT('',(12.7,-2.3,-18.3578583129651)) ;
#136787=CARTESIAN_POINT('',(12.7,-2.3,-17.2021416870349)) ;
#136788=CARTESIAN_POINT('',(12.7,-2.3,-17.78)) ;
#136789=CARTESIAN_POINT('',(4.6,-2.3,-17.2021416870349)) ;
#136790=CARTESIAN_POINT('',(4.5,-2.3,-17.2021416870349)) ;
#136791=CARTESIAN_POINT('',(4.6,-2.3,-18.3578583129651)) ;
#136792=CARTESIAN_POINT('',(4.6,-2.3,-18.3938639715742)) ;
#136793=CARTESIAN_POINT('',(4.5,-2.3,-18.3578583129651)) ;
#136794=CARTESIAN_POINT('Origin',(12.8,2.75,-17.78)) ;
#136795=CARTESIAN_POINT('',(12.7,2.75,-22.86)) ;
#136796=CARTESIAN_POINT('',(4.55912712210514,2.75,-22.86)) ;
#136797=CARTESIAN_POINT('',(12.8,2.75,-22.86)) ;
#136798=CARTESIAN_POINT('',(4.55912712210513,2.75,-21.8130460421716)) ;
#136799=CARTESIAN_POINT('',(4.55912712210514,2.75,-21.8130460421716)) ;
#136800=CARTESIAN_POINT('',(12.8,2.75,-21.8130460421716)) ;
#136801=CARTESIAN_POINT('',(12.7,2.75,-17.78)) ;
#136802=CARTESIAN_POINT('Origin',(0.,9.95,-20.32)) ;
#136803=CARTESIAN_POINT('',(0.230887397576971,9.95,-22.2348605718538)) ;
#136804=CARTESIAN_POINT('Origin',(12.8,-2.3,-17.78)) ;
#136805=CARTESIAN_POINT('',(12.8,-2.3359925337019,-17.9959552022114)) ;
#136806=CARTESIAN_POINT('',(12.8,2.65,-17.78)) ;
#136807=CARTESIAN_POINT('',(12.8,2.13287979746107,-16.8192327425948)) ;
#136808=CARTESIAN_POINT('',(12.8,-1.51220874991811,-17.4267475004913)) ;
#136809=CARTESIAN_POINT('',(12.8,1.9,-16.6219539578284)) ;
#136810=CARTESIAN_POINT('Origin',(12.8,2.1,-16.6219539578284)) ;
#136811=CARTESIAN_POINT('',(12.8,1.9,-12.7)) ;
#136812=CARTESIAN_POINT('',(12.8,-2.3359925337019,-12.9159552022114)) ;
#136813=CARTESIAN_POINT('',(12.8,2.65,-12.7)) ;
#136814=CARTESIAN_POINT('',(12.8,2.65,-12.7)) ;
#136815=CARTESIAN_POINT('',(12.8,-2.2,-12.7)) ;
#136816=CARTESIAN_POINT('',(12.8,-2.3,-12.7)) ;
#136817=CARTESIAN_POINT('',(12.8,-2.2,-13.2778583129651)) ;
#136818=CARTESIAN_POINT('',(12.8,-2.2,-12.7)) ;
#136819=CARTESIAN_POINT('',(12.8,-2.24516129032258,-13.4044480992255)) ;
#136820=CARTESIAN_POINT('Origin',(12.8,-2.4,-13.2778583129651)) ;
#136821=CARTESIAN_POINT('',(12.8,-2.24516129032258,-17.0755519007745)) ;
#136822=CARTESIAN_POINT('Origin',(12.8,0.,-15.24)) ;
#136823=CARTESIAN_POINT('',(12.8,-2.2,-17.2021416870349)) ;
#136824=CARTESIAN_POINT('Origin',(12.8,-2.4,-17.2021416870349)) ;
#136825=CARTESIAN_POINT('',(12.8,-2.2,-18.3578583129651)) ;
#136826=CARTESIAN_POINT('',(12.8,-2.2,-17.78)) ;
#136827=CARTESIAN_POINT('',(12.8,-2.24516129032258,-18.4844480992255)) ;
#136828=CARTESIAN_POINT('Origin',(12.8,-2.4,-18.3578583129651)) ;
#136829=CARTESIAN_POINT('',(12.8,-2.24516129032258,-22.1555519007745)) ;
#136830=CARTESIAN_POINT('Origin',(12.8,0.,-20.32)) ;
#136831=CARTESIAN_POINT('',(12.8,-2.2,-22.2821416870349)) ;
#136832=CARTESIAN_POINT('Origin',(12.8,-2.4,-22.2821416870349)) ;
#136833=CARTESIAN_POINT('',(12.8,-2.2,-22.86)) ;
#136834=CARTESIAN_POINT('',(12.8,-2.2,-17.78)) ;
#136835=CARTESIAN_POINT('',(12.8,2.65,-22.86)) ;
#136836=CARTESIAN_POINT('',(12.8,-2.3,-22.86)) ;
#136837=CARTESIAN_POINT('',(12.8,2.65,-17.78)) ;
#136838=CARTESIAN_POINT('',(12.8,2.13287979746107,-21.8992327425948)) ;
#136839=CARTESIAN_POINT('',(12.8,-1.51220874991811,-22.5067475004913)) ;
#136840=CARTESIAN_POINT('',(12.8,1.9,-21.7019539578284)) ;
#136841=CARTESIAN_POINT('Origin',(12.8,2.1,-21.7019539578284)) ;
#136842=CARTESIAN_POINT('',(12.8,1.9,-17.78)) ;
#136843=CARTESIAN_POINT('Origin',(12.8,2.75,-17.78)) ;
#136844=CARTESIAN_POINT('',(4.55912712210513,2.75,-18.8269539578284)) ;
#136845=CARTESIAN_POINT('',(12.8,2.75,-18.8269539578284)) ;
#136846=CARTESIAN_POINT('',(4.55912712210513,2.75,-16.7330460421716)) ;
#136847=CARTESIAN_POINT('',(4.55912712210514,2.75,-17.78)) ;
#136848=CARTESIAN_POINT('',(12.8,2.75,-16.7330460421716)) ;
#136849=CARTESIAN_POINT('',(12.7,2.75,-17.78)) ;
#136850=CARTESIAN_POINT('Origin',(4.5,2.75,-17.78)) ;
#136851=CARTESIAN_POINT('',(3.96237840913234,3.72749380157757,-22.86)) ;
#136852=CARTESIAN_POINT('',(3.96237840913234,3.72749380157757,-12.7)) ;
#136853=CARTESIAN_POINT('',(3.96237840913234,3.72749380157757,-17.78)) ;
#136854=CARTESIAN_POINT('',(4.47150553123747,2.80180812502278,-12.7)) ;
#136855=CARTESIAN_POINT('',(4.5,2.75,-12.7)) ;
#136856=CARTESIAN_POINT('',(4.47150553123747,2.80180812502279,-13.7469539578284)) ;
#136857=CARTESIAN_POINT('',(4.47150553123747,2.80180812502278,-13.7469539578284)) ;
#136858=CARTESIAN_POINT('',(4.48762159086767,2.77250619842243,-13.8511756817495)) ;
#136859=CARTESIAN_POINT('Origin',(4.56263299594724,2.63612182555043,-13.7566002940964)) ;
#136860=CARTESIAN_POINT('',(4.48762159086767,2.77250619842243,-16.6288243182478)) ;
#136861=CARTESIAN_POINT('',(4.48762159086767,2.77250619842243,-12.7)) ;
#136862=CARTESIAN_POINT('',(4.47150553123747,2.80180812502279,-16.7330460421716)) ;
#136863=CARTESIAN_POINT('Origin',(4.56263299597154,2.63612182550629,-16.723399705895)) ;
#136864=CARTESIAN_POINT('',(4.47150553123747,2.80180812502279,-18.8269539578284)) ;
#136865=CARTESIAN_POINT('',(4.47150553123747,2.80180812502278,-18.8269539578284)) ;
#136866=CARTESIAN_POINT('',(4.48762159086767,2.77250619842243,-18.9311756817495)) ;
#136867=CARTESIAN_POINT('Origin',(4.56263299594023,2.63612182556322,-18.836600294098)) ;
#136868=CARTESIAN_POINT('',(4.48762159086767,2.77250619842243,-21.7088243182478)) ;
#136869=CARTESIAN_POINT('',(4.48762159086767,2.77250619842243,-17.78)) ;
#136870=CARTESIAN_POINT('',(4.47150553123747,2.80180812502279,-21.8130460421716)) ;
#136871=CARTESIAN_POINT('Origin',(4.56263299597011,2.63612182550888,-21.8033997058945)) ;
#136872=CARTESIAN_POINT('',(4.47150553123747,2.80180812502278,-22.86)) ;
#136873=CARTESIAN_POINT('',(4.47150553123747,2.80180812502278,-22.86)) ;
#136874=CARTESIAN_POINT('',(4.5,2.75,-22.86)) ;
#136875=CARTESIAN_POINT('Origin',(3.95,6.95,-17.78)) ;
#136876=CARTESIAN_POINT('',(3.93762159086767,6.97250619842243,-22.86)) ;
#136877=CARTESIAN_POINT('',(3.95,6.95,-22.86)) ;
#136878=CARTESIAN_POINT('',(3.93762159086767,6.97250619842243,-12.7)) ;
#136879=CARTESIAN_POINT('',(3.95,6.95,-12.7)) ;
#136880=CARTESIAN_POINT('',(3.93762159086767,6.97250619842243,-17.78)) ;
#136881=CARTESIAN_POINT('Origin',(3.4,9.95,-17.78)) ;
#136882=CARTESIAN_POINT('',(3.4,10.85,-22.86)) ;
#136883=CARTESIAN_POINT('',(3.4,9.95,-22.86)) ;
#136884=CARTESIAN_POINT('',(3.4,10.85,-12.7)) ;
#136885=CARTESIAN_POINT('',(3.4,10.85,-17.78)) ;
#136886=CARTESIAN_POINT('',(3.4,9.95,-12.7)) ;
#136887=CARTESIAN_POINT('',(3.4,7.825,-22.36)) ;
#136888=CARTESIAN_POINT('Origin',(3.4,10.95,-17.78)) ;
#136889=CARTESIAN_POINT('',(3.3,10.95,-22.86)) ;
#136890=CARTESIAN_POINT('',(-4.8,10.95,-22.86)) ;
#136891=CARTESIAN_POINT('',(3.4,10.95,-22.86)) ;
#136892=CARTESIAN_POINT('',(-4.8,10.95,-12.7)) ;
#136893=CARTESIAN_POINT('',(-4.8,10.95,-17.78)) ;
#136894=CARTESIAN_POINT('',(3.3,10.95,-12.7)) ;
#136895=CARTESIAN_POINT('',(3.4,10.95,-12.7)) ;
#136896=CARTESIAN_POINT('',(3.3,10.95,-17.78)) ;
#136897=CARTESIAN_POINT('',(-2.55,10.95,-16.14)) ;
#136898=CARTESIAN_POINT('',(-2.75,10.95,-16.34)) ;
#136899=CARTESIAN_POINT('Origin',(-2.75,10.95,-16.14)) ;
#136900=CARTESIAN_POINT('',(-2.55,10.95,-14.34)) ;
#136901=CARTESIAN_POINT('',(-2.55,10.95,-12.7)) ;
#136902=CARTESIAN_POINT('',(-2.75,10.95,-14.14)) ;
#136903=CARTESIAN_POINT('Origin',(-2.75,10.95,-14.34)) ;
#136904=CARTESIAN_POINT('',(-3.8,10.95,-14.14)) ;
#136905=CARTESIAN_POINT('',(3.4,10.95,-14.14)) ;
#136906=CARTESIAN_POINT('',(-4.,10.95,-14.34)) ;
#136907=CARTESIAN_POINT('Origin',(-3.8,10.95,-14.34)) ;
#136908=CARTESIAN_POINT('',(-4.,10.95,-16.14)) ;
#136909=CARTESIAN_POINT('',(-4.,10.95,-12.7)) ;
#136910=CARTESIAN_POINT('',(-3.8,10.95,-16.34)) ;
#136911=CARTESIAN_POINT('Origin',(-3.8,10.95,-16.14)) ;
#136912=CARTESIAN_POINT('',(3.4,10.95,-16.34)) ;
#136913=CARTESIAN_POINT('',(-2.55,10.95,-21.22)) ;
#136914=CARTESIAN_POINT('',(-2.75,10.95,-21.42)) ;
#136915=CARTESIAN_POINT('Origin',(-2.75,10.95,-21.22)) ;
#136916=CARTESIAN_POINT('',(-2.55,10.95,-19.42)) ;
#136917=CARTESIAN_POINT('',(-2.55,10.95,-17.78)) ;
#136918=CARTESIAN_POINT('',(-2.75,10.95,-19.22)) ;
#136919=CARTESIAN_POINT('Origin',(-2.75,10.95,-19.42)) ;
#136920=CARTESIAN_POINT('',(-3.8,10.95,-19.22)) ;
#136921=CARTESIAN_POINT('',(3.4,10.95,-19.22)) ;
#136922=CARTESIAN_POINT('',(-4.,10.95,-19.42)) ;
#136923=CARTESIAN_POINT('Origin',(-3.8,10.95,-19.42)) ;
#136924=CARTESIAN_POINT('',(-4.,10.95,-21.22)) ;
#136925=CARTESIAN_POINT('',(-4.,10.95,-17.78)) ;
#136926=CARTESIAN_POINT('',(-3.8,10.95,-21.42)) ;
#136927=CARTESIAN_POINT('Origin',(-3.8,10.95,-21.22)) ;
#136928=CARTESIAN_POINT('',(3.4,10.95,-21.42)) ;
#136929=CARTESIAN_POINT('Origin',(-4.9,10.95,-17.78)) ;
#136930=CARTESIAN_POINT('',(-4.9,10.85,-22.86)) ;
#136931=CARTESIAN_POINT('',(-4.9,10.3,-22.86)) ;
#136932=CARTESIAN_POINT('',(-4.9,10.95,-22.86)) ;
#136933=CARTESIAN_POINT('',(-4.9,10.3,-12.7)) ;
#136934=CARTESIAN_POINT('',(-4.9,10.3,-17.78)) ;
#136935=CARTESIAN_POINT('',(-4.9,10.85,-12.7)) ;
#136936=CARTESIAN_POINT('',(-4.9,10.95,-12.7)) ;
#136937=CARTESIAN_POINT('',(-4.9,10.85,-17.78)) ;
#136938=CARTESIAN_POINT('Origin',(-4.9,10.2,-17.78)) ;
#136939=CARTESIAN_POINT('',(-4.8,10.2,-22.86)) ;
#136940=CARTESIAN_POINT('',(-4.9,10.2,-22.86)) ;
#136941=CARTESIAN_POINT('',(-4.8,10.2,-12.7)) ;
#136942=CARTESIAN_POINT('',(-4.9,10.2,-12.7)) ;
#136943=CARTESIAN_POINT('',(-4.8,10.2,-17.78)) ;
#136944=CARTESIAN_POINT('Origin',(-4.4,10.2,-17.78)) ;
#136945=CARTESIAN_POINT('',(-5.39805806756909,5.20970966215454,-22.86)) ;
#136946=CARTESIAN_POINT('',(-4.4,10.2,-22.86)) ;
#136947=CARTESIAN_POINT('',(-5.39805806756909,5.20970966215454,-12.7)) ;
#136948=CARTESIAN_POINT('',(-5.39805806756909,5.20970966215454,-17.78)) ;
#136949=CARTESIAN_POINT('',(-4.4,10.2,-12.7)) ;
#136950=CARTESIAN_POINT('Origin',(-5.4,5.2,-17.78)) ;
#136951=CARTESIAN_POINT('',(-5.4,5.19009804864072,-22.86)) ;
#136952=CARTESIAN_POINT('',(-5.4,-3.95,-22.86)) ;
#136953=CARTESIAN_POINT('',(-5.4,5.2,-22.86)) ;
#136954=CARTESIAN_POINT('',(-5.4,-3.95,-12.7)) ;
#136955=CARTESIAN_POINT('',(-5.4,-3.95,-17.78)) ;
#136956=CARTESIAN_POINT('',(-5.4,5.19009804864072,-12.7)) ;
#136957=CARTESIAN_POINT('',(-5.4,5.2,-12.7)) ;
#136958=CARTESIAN_POINT('',(-5.4,5.19009804864072,-17.78)) ;
#136959=CARTESIAN_POINT('',(-5.4,4.23801993223491,-17.14)) ;
#136960=CARTESIAN_POINT('',(-5.4,4.23801993223491,-13.34)) ;
#136961=CARTESIAN_POINT('',(-5.4,4.23801993223491,-13.24)) ;
#136962=CARTESIAN_POINT('',(-5.4,3.9369800677651,-13.14)) ;
#136963=CARTESIAN_POINT('Ctrl Pts',(-5.4,4.23801993223491,-13.34)) ;
#136964=CARTESIAN_POINT('Ctrl Pts',(-5.4,4.23801992976516,-13.2874931280902)) ;
#136965=CARTESIAN_POINT('Ctrl Pts',(-5.4,4.20557579169425,-13.2356025737683)) ;
#136966=CARTESIAN_POINT('Ctrl Pts',(-5.4,4.09411900298411,-13.1615547137571)) ;
#136967=CARTESIAN_POINT('Ctrl Pts',(-5.4,4.0160133758189,-13.1400000004813)) ;
#136968=CARTESIAN_POINT('Ctrl Pts',(-5.4,3.9369800677651,-13.14)) ;
#136969=CARTESIAN_POINT('',(-5.4,-1.88819660112502,-13.14)) ;
#136970=CARTESIAN_POINT('',(-5.4,-2.05,-13.14)) ;
#136971=CARTESIAN_POINT('',(-5.4,-2.11180339887499,-13.34)) ;
#136972=CARTESIAN_POINT('Ctrl Pts',(-5.4,-2.11180339887499,-13.34)) ;
#136973=CARTESIAN_POINT('Ctrl Pts',(-5.4,-2.11180339704051,-13.2874931601087)) ;
#136974=CARTESIAN_POINT('Ctrl Pts',(-5.4,-2.0877044485962,-13.2356025311215)) ;
#136975=CARTESIAN_POINT('Ctrl Pts',(-5.4,-2.00491651967066,-13.1615547564039)) ;
#136976=CARTESIAN_POINT('Ctrl Pts',(-5.4,-1.946901032774,-13.1400000011741)) ;
#136977=CARTESIAN_POINT('Ctrl Pts',(-5.4,-1.88819660112501,-13.14)) ;
#136978=CARTESIAN_POINT('',(-5.4,-2.11180339887499,-17.14)) ;
#136979=CARTESIAN_POINT('',(-5.4,-2.11180339887499,-17.24)) ;
#136980=CARTESIAN_POINT('',(-5.4,-1.88819660112501,-17.34)) ;
#136981=CARTESIAN_POINT('Ctrl Pts',(-5.4,-1.88819660112501,-17.34)) ;
#136982=CARTESIAN_POINT('Ctrl Pts',(-5.4,-1.946901032774,-17.3399999988261)) ;
#136983=CARTESIAN_POINT('Ctrl Pts',(-5.4,-2.00491651967066,-17.3184452435961)) ;
#136984=CARTESIAN_POINT('Ctrl Pts',(-5.4,-2.0877044485962,-17.2443974688785)) ;
#136985=CARTESIAN_POINT('Ctrl Pts',(-5.4,-2.11180339704051,-17.1925068398913)) ;
#136986=CARTESIAN_POINT('Ctrl Pts',(-5.4,-2.11180339887499,-17.14)) ;
#136987=CARTESIAN_POINT('',(-5.4,3.9369800677651,-17.34)) ;
#136988=CARTESIAN_POINT('',(-5.4,4.20000000000001,-17.34)) ;
#136989=CARTESIAN_POINT('Ctrl Pts',(-5.4,3.9369800677651,-17.34)) ;
#136990=CARTESIAN_POINT('Ctrl Pts',(-5.4,4.01601337581888,-17.3399999995189)) ;
#136991=CARTESIAN_POINT('Ctrl Pts',(-5.4,4.09411900298413,-17.3184452862429)) ;
#136992=CARTESIAN_POINT('Ctrl Pts',(-5.4,4.20557579169423,-17.2443974262317)) ;
#136993=CARTESIAN_POINT('Ctrl Pts',(-5.4,4.23801992976516,-17.1925068719098)) ;
#136994=CARTESIAN_POINT('Ctrl Pts',(-5.4,4.23801993223491,-17.14)) ;
#136995=CARTESIAN_POINT('',(-5.4,4.23801993223491,-22.22)) ;
#136996=CARTESIAN_POINT('',(-5.4,4.23801993223491,-18.42)) ;
#136997=CARTESIAN_POINT('',(-5.4,4.23801993223491,-18.32)) ;
#136998=CARTESIAN_POINT('',(-5.4,3.9369800677651,-18.22)) ;
#136999=CARTESIAN_POINT('Ctrl Pts',(-5.4,4.23801993223491,-18.42)) ;
#137000=CARTESIAN_POINT('Ctrl Pts',(-5.4,4.23801992976516,-18.3674931280903)) ;
#137001=CARTESIAN_POINT('Ctrl Pts',(-5.4,4.20557579169425,-18.3156025737682)) ;
#137002=CARTESIAN_POINT('Ctrl Pts',(-5.4,4.09411900298411,-18.2415547137572)) ;
#137003=CARTESIAN_POINT('Ctrl Pts',(-5.4,4.0160133758189,-18.2200000004811)) ;
#137004=CARTESIAN_POINT('Ctrl Pts',(-5.4,3.9369800677651,-18.22)) ;
#137005=CARTESIAN_POINT('',(-5.4,-1.88819660112502,-18.22)) ;
#137006=CARTESIAN_POINT('',(-5.4,-2.05,-18.22)) ;
#137007=CARTESIAN_POINT('',(-5.4,-2.11180339887499,-18.42)) ;
#137008=CARTESIAN_POINT('Ctrl Pts',(-5.4,-2.11180339887499,-18.42)) ;
#137009=CARTESIAN_POINT('Ctrl Pts',(-5.4,-2.11180339704051,-18.3674931601087)) ;
#137010=CARTESIAN_POINT('Ctrl Pts',(-5.4,-2.0877044485962,-18.3156025311215)) ;
#137011=CARTESIAN_POINT('Ctrl Pts',(-5.4,-2.00491651967066,-18.2415547564039)) ;
#137012=CARTESIAN_POINT('Ctrl Pts',(-5.4,-1.946901032774,-18.2200000011739)) ;
#137013=CARTESIAN_POINT('Ctrl Pts',(-5.4,-1.88819660112502,-18.22)) ;
#137014=CARTESIAN_POINT('',(-5.4,-2.11180339887499,-22.22)) ;
#137015=CARTESIAN_POINT('',(-5.4,-2.11180339887499,-22.32)) ;
#137016=CARTESIAN_POINT('',(-5.4,-1.88819660112501,-22.42)) ;
#137017=CARTESIAN_POINT('Ctrl Pts',(-5.4,-1.88819660112501,-22.42)) ;
#137018=CARTESIAN_POINT('Ctrl Pts',(-5.4,-1.946901032774,-22.4199999988261)) ;
#137019=CARTESIAN_POINT('Ctrl Pts',(-5.4,-2.00491651967066,-22.3984452435961)) ;
#137020=CARTESIAN_POINT('Ctrl Pts',(-5.4,-2.0877044485962,-22.3243974688785)) ;
#137021=CARTESIAN_POINT('Ctrl Pts',(-5.4,-2.11180339704051,-22.2725068398913)) ;
#137022=CARTESIAN_POINT('Ctrl Pts',(-5.4,-2.11180339887499,-22.22)) ;
#137023=CARTESIAN_POINT('',(-5.4,3.9369800677651,-22.42)) ;
#137024=CARTESIAN_POINT('',(-5.4,4.20000000000001,-22.42)) ;
#137025=CARTESIAN_POINT('Ctrl Pts',(-5.4,3.9369800677651,-22.42)) ;
#137026=CARTESIAN_POINT('Ctrl Pts',(-5.4,4.01601337581889,-22.4199999995189)) ;
#137027=CARTESIAN_POINT('Ctrl Pts',(-5.4,4.09411900298413,-22.3984452862429)) ;
#137028=CARTESIAN_POINT('Ctrl Pts',(-5.4,4.20557579169423,-22.3243974262317)) ;
#137029=CARTESIAN_POINT('Ctrl Pts',(-5.4,4.23801992976516,-22.2725068719098)) ;
#137030=CARTESIAN_POINT('Ctrl Pts',(-5.4,4.23801993223491,-22.22)) ;
#137031=CARTESIAN_POINT('Origin',(-5.4,-4.05,-17.78)) ;
#137032=CARTESIAN_POINT('',(-5.3,-4.05,-22.86)) ;
#137033=CARTESIAN_POINT('',(3.5,-4.05,-22.86)) ;
#137034=CARTESIAN_POINT('',(-5.4,-4.05,-22.86)) ;
#137035=CARTESIAN_POINT('',(3.5,-4.05,-12.7)) ;
#137036=CARTESIAN_POINT('',(3.5,-4.05,-17.78)) ;
#137037=CARTESIAN_POINT('',(-5.3,-4.05,-12.7)) ;
#137038=CARTESIAN_POINT('',(-5.4,-4.05,-12.7)) ;
#137039=CARTESIAN_POINT('',(-5.3,-4.05,-17.78)) ;
#137040=CARTESIAN_POINT('',(-4.5,-4.05,-16.14)) ;
#137041=CARTESIAN_POINT('',(-4.3,-4.05,-16.34)) ;
#137042=CARTESIAN_POINT('Origin',(-4.3,-4.05,-16.14)) ;
#137043=CARTESIAN_POINT('',(-4.5,-4.05,-14.34)) ;
#137044=CARTESIAN_POINT('',(-4.5,-4.05,-12.7)) ;
#137045=CARTESIAN_POINT('',(-4.3,-4.05,-14.14)) ;
#137046=CARTESIAN_POINT('Origin',(-4.3,-4.05,-14.34)) ;
#137047=CARTESIAN_POINT('',(-3.25,-4.05,-14.14)) ;
#137048=CARTESIAN_POINT('',(-5.4,-4.05,-14.14)) ;
#137049=CARTESIAN_POINT('',(-3.05,-4.05,-14.34)) ;
#137050=CARTESIAN_POINT('Origin',(-3.25,-4.05,-14.34)) ;
#137051=CARTESIAN_POINT('',(-3.05,-4.05,-16.14)) ;
#137052=CARTESIAN_POINT('',(-3.05,-4.05,-12.7)) ;
#137053=CARTESIAN_POINT('',(-3.25,-4.05,-16.34)) ;
#137054=CARTESIAN_POINT('Origin',(-3.25,-4.05,-16.14)) ;
#137055=CARTESIAN_POINT('',(-5.4,-4.05,-16.34)) ;
#137056=CARTESIAN_POINT('',(-4.5,-4.05,-21.22)) ;
#137057=CARTESIAN_POINT('',(-4.3,-4.05,-21.42)) ;
#137058=CARTESIAN_POINT('Origin',(-4.3,-4.05,-21.22)) ;
#137059=CARTESIAN_POINT('',(-4.5,-4.05,-19.42)) ;
#137060=CARTESIAN_POINT('',(-4.5,-4.05,-17.78)) ;
#137061=CARTESIAN_POINT('',(-4.3,-4.05,-19.22)) ;
#137062=CARTESIAN_POINT('Origin',(-4.3,-4.05,-19.42)) ;
#137063=CARTESIAN_POINT('',(-3.25,-4.05,-19.22)) ;
#137064=CARTESIAN_POINT('',(-5.4,-4.05,-19.22)) ;
#137065=CARTESIAN_POINT('',(-3.05,-4.05,-19.42)) ;
#137066=CARTESIAN_POINT('Origin',(-3.25,-4.05,-19.42)) ;
#137067=CARTESIAN_POINT('',(-3.05,-4.05,-21.22)) ;
#137068=CARTESIAN_POINT('',(-3.05,-4.05,-17.78)) ;
#137069=CARTESIAN_POINT('',(-3.25,-4.05,-21.42)) ;
#137070=CARTESIAN_POINT('Origin',(-3.25,-4.05,-21.22)) ;
#137071=CARTESIAN_POINT('',(-5.4,-4.05,-21.42)) ;
#137072=CARTESIAN_POINT('Origin',(3.6,-4.05,-17.78)) ;
#137073=CARTESIAN_POINT('',(3.6,-3.95,-22.86)) ;
#137074=CARTESIAN_POINT('',(3.6,-2.9,-22.86)) ;
#137075=CARTESIAN_POINT('',(3.6,-4.05,-22.86)) ;
#137076=CARTESIAN_POINT('',(3.6,-2.9,-12.7)) ;
#137077=CARTESIAN_POINT('',(3.6,-2.9,-17.78)) ;
#137078=CARTESIAN_POINT('',(3.6,-3.95,-12.7)) ;
#137079=CARTESIAN_POINT('',(3.6,-4.05,-12.7)) ;
#137080=CARTESIAN_POINT('',(3.6,-3.95,-17.78)) ;
#137081=CARTESIAN_POINT('Origin',(3.6,-2.8,-17.78)) ;
#137082=CARTESIAN_POINT('',(4.4,-2.8,-21.8431546211728)) ;
#137083=CARTESIAN_POINT('',(4.54880051362942,-2.79999999972164,-21.3964378607329)) ;
#137084=CARTESIAN_POINT('Ctrl Pts',(4.4,-2.8,-21.8431546211728)) ;
#137085=CARTESIAN_POINT('Ctrl Pts',(4.40001102013631,-2.8,-21.8064400198503)) ;
#137086=CARTESIAN_POINT('Ctrl Pts',(4.40220140384643,-2.79999999812164,
-21.7700681661022)) ;
#137087=CARTESIAN_POINT('Ctrl Pts',(4.4066417499365,-2.79999999722267,-21.7340727380016)) ;
#137088=CARTESIAN_POINT('Ctrl Pts',(4.41108209602656,-2.79999999632371,
-21.6980773099009)) ;
#137089=CARTESIAN_POINT('Ctrl Pts',(4.41777240449682,-2.79999999692353,
-21.6624583074478)) ;
#137090=CARTESIAN_POINT('Ctrl Pts',(4.42678327415264,-2.79999999844302,
-21.6272494087151)) ;
#137091=CARTESIAN_POINT('Ctrl Pts',(4.42864654535147,-2.79999999875722,
-21.6199688986803)) ;
#137092=CARTESIAN_POINT('Ctrl Pts',(4.43060908636135,-2.79999999907333,
-21.6127059171117)) ;
#137093=CARTESIAN_POINT('Ctrl Pts',(4.43267155768737,-2.79999999933983,
-21.6054607590652)) ;
#137094=CARTESIAN_POINT('Ctrl Pts',(4.4352900037877,-2.79999999967816,-21.5962625435099)) ;
#137095=CARTESIAN_POINT('Ctrl Pts',(4.4380733085653,-2.79999999966609,-21.5870911025424)) ;
#137096=CARTESIAN_POINT('Ctrl Pts',(4.44102157277561,-2.79999999954234,
-21.5779480782015)) ;
#137097=CARTESIAN_POINT('Ctrl Pts',(4.45046499569139,-2.79999999914597,
-21.548662559869)) ;
#137098=CARTESIAN_POINT('Ctrl Pts',(4.46157908226631,-2.7999999950538,-21.5197202134932)) ;
#137099=CARTESIAN_POINT('Ctrl Pts',(4.47540732315414,-2.79999999166095,
-21.4922492625065)) ;
#137100=CARTESIAN_POINT('Ctrl Pts',(4.47702479055524,-2.79999999126409,
-21.4890360289464)) ;
#137101=CARTESIAN_POINT('Ctrl Pts',(4.47867903313991,-2.79999999107055,
-21.4858427221255)) ;
#137102=CARTESIAN_POINT('Ctrl Pts',(4.4803718748147,-2.79999999105954,-21.482671097194)) ;
#137103=CARTESIAN_POINT('Ctrl Pts',(4.48545039983907,-2.79999999102651,
-21.4731562223995)) ;
#137104=CARTESIAN_POINT('Ctrl Pts',(4.49087631667452,-2.79999999265304,
-21.4638364846097)) ;
#137105=CARTESIAN_POINT('Ctrl Pts',(4.49669887079745,-2.79999999431461,
-21.4547592728789)) ;
#137106=CARTESIAN_POINT('Ctrl Pts',(4.50888705006192,-2.79999999779274,
-21.4357582157035)) ;
#137107=CARTESIAN_POINT('Ctrl Pts',(4.52313265843749,-2.79999999982394,
-21.41737449918)) ;
#137108=CARTESIAN_POINT('Ctrl Pts',(4.54066913339539,-2.79999999997241,
-21.4027304219711)) ;
#137109=CARTESIAN_POINT('Ctrl Pts',(4.54329026609835,-2.79999999999461,
-21.400541608668)) ;
#137110=CARTESIAN_POINT('Ctrl Pts',(4.5460045281952,-2.8,-21.3984393445787)) ;
#137111=CARTESIAN_POINT('Ctrl Pts',(4.54880363749517,-2.8,-21.396450206041)) ;
#137112=CARTESIAN_POINT('',(4.4,-2.8,-20.3200000000039)) ;
#137113=CARTESIAN_POINT('Ctrl Pts',(4.54879236168152,-2.8,-21.39643444348)) ;
#137114=CARTESIAN_POINT('Ctrl Pts',(4.51096310105345,-2.8,-21.3676409078196)) ;
#137115=CARTESIAN_POINT('Ctrl Pts',(4.49022331291407,-2.8,-21.3238291192761)) ;
#137116=CARTESIAN_POINT('Ctrl Pts',(4.45698031182017,-2.8,-21.2376238713958)) ;
#137117=CARTESIAN_POINT('Ctrl Pts',(4.44561000227039,-2.8,-21.1923611449586)) ;
#137118=CARTESIAN_POINT('Ctrl Pts',(4.41911102299977,-2.8,-21.0558807916569)) ;
#137119=CARTESIAN_POINT('Ctrl Pts',(4.41155688769424,-2.8,-20.964231375192)) ;
#137120=CARTESIAN_POINT('Ctrl Pts',(4.39763503647248,-2.8,-20.688710456933)) ;
#137121=CARTESIAN_POINT('Ctrl Pts',(4.4,-2.8,-20.5042606621178)) ;
#137122=CARTESIAN_POINT('Ctrl Pts',(4.4,-2.8,-20.3200000000039)) ;
#137123=CARTESIAN_POINT('',(4.54879236179094,-2.79999999953044,-19.2435655565041)) ;
#137124=CARTESIAN_POINT('Ctrl Pts',(4.4,-2.8,-20.3200000000039)) ;
#137125=CARTESIAN_POINT('Ctrl Pts',(4.4,-2.8,-20.1354847183429)) ;
#137126=CARTESIAN_POINT('Ctrl Pts',(4.39760751905643,-2.8,-19.9507836732851)) ;
#137127=CARTESIAN_POINT('Ctrl Pts',(4.40696794948104,-2.8,-19.7665893237033)) ;
#137128=CARTESIAN_POINT('Ctrl Pts',(4.41164816469334,-2.8,-19.6744921489124)) ;
#137129=CARTESIAN_POINT('Ctrl Pts',(4.41940496802384,-2.80000000000001,
-19.5821571435008)) ;
#137130=CARTESIAN_POINT('Ctrl Pts',(4.43698455094239,-2.8,-19.4920661537484)) ;
#137131=CARTESIAN_POINT('Ctrl Pts',(4.44577434240167,-2.8,-19.4470206588722)) ;
#137132=CARTESIAN_POINT('Ctrl Pts',(4.456925956929,-2.80000000000001,-19.4024769174896)) ;
#137133=CARTESIAN_POINT('Ctrl Pts',(4.47366127850408,-2.8,-19.3591194060904)) ;
#137134=CARTESIAN_POINT('Ctrl Pts',(4.47575319370098,-2.8,-19.3536997171655)) ;
#137135=CARTESIAN_POINT('Ctrl Pts',(4.47791173590511,-2.79999999997843,
-19.3482741547806)) ;
#137136=CARTESIAN_POINT('Ctrl Pts',(4.48016062485992,-2.80000000010461,
-19.3428732875221)) ;
#137137=CARTESIAN_POINT('Ctrl Pts',(4.48803173620173,-2.80000000054624,
-19.3239702521172)) ;
#137138=CARTESIAN_POINT('Ctrl Pts',(4.49700942865457,-2.80000000534986,
-19.3053696658144)) ;
#137139=CARTESIAN_POINT('Ctrl Pts',(4.50810946414921,-2.80000000469598,
-19.2883816651393)) ;
#137140=CARTESIAN_POINT('Ctrl Pts',(4.51435323411495,-2.80000000432818,
-19.2788259147596)) ;
#137141=CARTESIAN_POINT('Ctrl Pts',(4.52126852668377,-2.80000000204489,
-19.2697803965514)) ;
#137142=CARTESIAN_POINT('Ctrl Pts',(4.5290361256546,-2.80000000089509,-19.2614782866676)) ;
#137143=CARTESIAN_POINT('Ctrl Pts',(4.5320568585877,-2.80000000044794,-19.2582496883795)) ;
#137144=CARTESIAN_POINT('Ctrl Pts',(4.53520648971123,-2.80000000018876,
-19.2551335191281)) ;
#137145=CARTESIAN_POINT('Ctrl Pts',(4.53849565154303,-2.80000000008376,
-19.252143492806)) ;
#137146=CARTESIAN_POINT('Ctrl Pts',(4.54178481337482,-2.79999999997876,
-19.2491534664838)) ;
#137147=CARTESIAN_POINT('Ctrl Pts',(4.54521363891049,-2.8,-19.2462897578219)) ;
#137148=CARTESIAN_POINT('Ctrl Pts',(4.5487923616809,-2.8,-19.2435655565195)) ;
#137149=CARTESIAN_POINT('',(4.4,-2.8,-18.7968453788272)) ;
#137150=CARTESIAN_POINT('Ctrl Pts',(4.54879236168109,-2.79999999812176,
-19.2435655565192)) ;
#137151=CARTESIAN_POINT('Ctrl Pts',(4.54599316991904,-2.79999999835896,
-19.2415756143354)) ;
#137152=CARTESIAN_POINT('Ctrl Pts',(4.54327885465676,-2.7999999985882,-19.2394726568399)) ;
#137153=CARTESIAN_POINT('Ctrl Pts',(4.52311604063302,-2.80000000023132,
-19.2226310596931)) ;
#137154=CARTESIAN_POINT('Ctrl Pts',(4.5088678063233,-2.80000000100533,-19.2042421996431)) ;
#137155=CARTESIAN_POINT('Ctrl Pts',(4.48892103801306,-2.79999999510252,
-19.1731290218304)) ;
#137156=CARTESIAN_POINT('Ctrl Pts',(4.48186523313292,-2.7999999909955,-19.1605832050237)) ;
#137157=CARTESIAN_POINT('Ctrl Pts',(4.46162186753409,-2.79999997126272,
-19.1202567139418)) ;
#137158=CARTESIAN_POINT('Ctrl Pts',(4.45052849087263,-2.7999999685384,-19.0913189617092)) ;
#137159=CARTESIAN_POINT('Ctrl Pts',(4.43813540717736,-2.79999997674815,
-19.0529060591291)) ;
#137160=CARTESIAN_POINT('Ctrl Pts',(4.43535270120343,-2.79999997903695,
-19.0437502640508)) ;
#137161=CARTESIAN_POINT('Ctrl Pts',(4.41677772587598,-2.79999999273252,
-18.9786688014867)) ;
#137162=CARTESIAN_POINT('Ctrl Pts',(4.40678488790793,-2.79999999887621,
-18.9217195184934)) ;
#137163=CARTESIAN_POINT('Ctrl Pts',(4.40081887576499,-2.80000000006435,
-18.8416198967613)) ;
#137164=CARTESIAN_POINT('Ctrl Pts',(4.4,-2.8,-18.8193018981784)) ;
#137165=CARTESIAN_POINT('Ctrl Pts',(4.4,-2.8,-18.7968453788272)) ;
#137166=CARTESIAN_POINT('',(4.4,-2.8,-16.7631546211728)) ;
#137167=CARTESIAN_POINT('',(4.4,-2.8,-17.78)) ;
#137168=CARTESIAN_POINT('',(4.54880051362942,-2.79999999972164,-16.3164378607329)) ;
#137169=CARTESIAN_POINT('Ctrl Pts',(4.4,-2.8,-16.7631546211728)) ;
#137170=CARTESIAN_POINT('Ctrl Pts',(4.40001102013631,-2.8,-16.7264400198511)) ;
#137171=CARTESIAN_POINT('Ctrl Pts',(4.40220140384633,-2.79999999812164,
-16.6900681661039)) ;
#137172=CARTESIAN_POINT('Ctrl Pts',(4.40664174993619,-2.79999999722267,
-16.6540727380041)) ;
#137173=CARTESIAN_POINT('Ctrl Pts',(4.41108209602605,-2.79999999632371,
-16.6180773099042)) ;
#137174=CARTESIAN_POINT('Ctrl Pts',(4.41777240449601,-2.79999999692353,
-16.5824583074518)) ;
#137175=CARTESIAN_POINT('Ctrl Pts',(4.42678327415141,-2.79999999844302,
-16.5472494087199)) ;
#137176=CARTESIAN_POINT('Ctrl Pts',(4.42864654535061,-2.79999999875722,
-16.5399688986835)) ;
#137177=CARTESIAN_POINT('Ctrl Pts',(4.4306090863609,-2.79999999907333,-16.5327059171133)) ;
#137178=CARTESIAN_POINT('Ctrl Pts',(4.43267155768737,-2.79999999933982,
-16.5254607590652)) ;
#137179=CARTESIAN_POINT('Ctrl Pts',(4.4352900037877,-2.79999999967816,-16.5162625435099)) ;
#137180=CARTESIAN_POINT('Ctrl Pts',(4.4380733085653,-2.79999999966609,-16.5070911025424)) ;
#137181=CARTESIAN_POINT('Ctrl Pts',(4.44102157277562,-2.79999999954234,
-16.4979480782015)) ;
#137182=CARTESIAN_POINT('Ctrl Pts',(4.45046499569139,-2.79999999914597,
-16.468662559869)) ;
#137183=CARTESIAN_POINT('Ctrl Pts',(4.46157908226631,-2.79999999505379,
-16.4397202134932)) ;
#137184=CARTESIAN_POINT('Ctrl Pts',(4.47540732315414,-2.79999999166095,
-16.4122492625065)) ;
#137185=CARTESIAN_POINT('Ctrl Pts',(4.47702479055524,-2.79999999126409,
-16.4090360289464)) ;
#137186=CARTESIAN_POINT('Ctrl Pts',(4.47867903313991,-2.79999999107055,
-16.4058427221255)) ;
#137187=CARTESIAN_POINT('Ctrl Pts',(4.4803718748147,-2.79999999105954,-16.402671097194)) ;
#137188=CARTESIAN_POINT('Ctrl Pts',(4.48545039983907,-2.79999999102651,
-16.3931562223995)) ;
#137189=CARTESIAN_POINT('Ctrl Pts',(4.49087631667452,-2.79999999265304,
-16.3838364846097)) ;
#137190=CARTESIAN_POINT('Ctrl Pts',(4.49669887079745,-2.79999999431461,
-16.3747592728789)) ;
#137191=CARTESIAN_POINT('Ctrl Pts',(4.50888705006192,-2.79999999779274,
-16.3557582157035)) ;
#137192=CARTESIAN_POINT('Ctrl Pts',(4.52313265843749,-2.79999999982394,
-16.33737449918)) ;
#137193=CARTESIAN_POINT('Ctrl Pts',(4.54066913339539,-2.79999999997241,
-16.3227304219711)) ;
#137194=CARTESIAN_POINT('Ctrl Pts',(4.54329026609835,-2.7999999999946,-16.320541608668)) ;
#137195=CARTESIAN_POINT('Ctrl Pts',(4.5460045281952,-2.8,-16.3184393445787)) ;
#137196=CARTESIAN_POINT('Ctrl Pts',(4.54880363749517,-2.8,-16.316450206041)) ;
#137197=CARTESIAN_POINT('',(4.4,-2.8,-15.2400000000038)) ;
#137198=CARTESIAN_POINT('Ctrl Pts',(4.54879236168152,-2.8,-16.31643444348)) ;
#137199=CARTESIAN_POINT('Ctrl Pts',(4.51096310105345,-2.8,-16.2876409078196)) ;
#137200=CARTESIAN_POINT('Ctrl Pts',(4.49022331291407,-2.8,-16.2438291192761)) ;
#137201=CARTESIAN_POINT('Ctrl Pts',(4.45698031182017,-2.8,-16.1576238713958)) ;
#137202=CARTESIAN_POINT('Ctrl Pts',(4.44561000227039,-2.8,-16.1123611449586)) ;
#137203=CARTESIAN_POINT('Ctrl Pts',(4.41911102299977,-2.8,-15.9758807916569)) ;
#137204=CARTESIAN_POINT('Ctrl Pts',(4.41155688769424,-2.8,-15.8842313751921)) ;
#137205=CARTESIAN_POINT('Ctrl Pts',(4.39763503647248,-2.8,-15.608710456933)) ;
#137206=CARTESIAN_POINT('Ctrl Pts',(4.4,-2.8,-15.4242606621178)) ;
#137207=CARTESIAN_POINT('Ctrl Pts',(4.4,-2.8,-15.2400000000038)) ;
#137208=CARTESIAN_POINT('',(4.54879236179093,-2.79999999953044,-14.1635655565041)) ;
#137209=CARTESIAN_POINT('Ctrl Pts',(4.4,-2.8,-15.2400000000038)) ;
#137210=CARTESIAN_POINT('Ctrl Pts',(4.4,-2.8,-15.0554847183429)) ;
#137211=CARTESIAN_POINT('Ctrl Pts',(4.39760751905643,-2.8,-14.8707836732851)) ;
#137212=CARTESIAN_POINT('Ctrl Pts',(4.40696794948104,-2.8,-14.6865893237033)) ;
#137213=CARTESIAN_POINT('Ctrl Pts',(4.41164816469334,-2.8,-14.5944921489124)) ;
#137214=CARTESIAN_POINT('Ctrl Pts',(4.41940496802384,-2.80000000000001,
-14.5021571435008)) ;
#137215=CARTESIAN_POINT('Ctrl Pts',(4.43698455094237,-2.8,-14.4120661537484)) ;
#137216=CARTESIAN_POINT('Ctrl Pts',(4.44577434240165,-2.8,-14.3670206588722)) ;
#137217=CARTESIAN_POINT('Ctrl Pts',(4.456925956929,-2.80000000000001,-14.3224769174896)) ;
#137218=CARTESIAN_POINT('Ctrl Pts',(4.47366127850409,-2.8,-14.2791194060904)) ;
#137219=CARTESIAN_POINT('Ctrl Pts',(4.47575319370098,-2.8,-14.2736997171655)) ;
#137220=CARTESIAN_POINT('Ctrl Pts',(4.47791173590511,-2.79999999997843,
-14.2682741547806)) ;
#137221=CARTESIAN_POINT('Ctrl Pts',(4.48016062485991,-2.80000000010461,
-14.2628732875221)) ;
#137222=CARTESIAN_POINT('Ctrl Pts',(4.48803173620173,-2.80000000054624,
-14.2439702521172)) ;
#137223=CARTESIAN_POINT('Ctrl Pts',(4.49700942865457,-2.80000000534986,
-14.2253696658144)) ;
#137224=CARTESIAN_POINT('Ctrl Pts',(4.50810946414921,-2.80000000469598,
-14.2083816651393)) ;
#137225=CARTESIAN_POINT('Ctrl Pts',(4.51435323411495,-2.80000000432818,
-14.1988259147596)) ;
#137226=CARTESIAN_POINT('Ctrl Pts',(4.52126852668377,-2.80000000204489,
-14.1897803965514)) ;
#137227=CARTESIAN_POINT('Ctrl Pts',(4.5290361256546,-2.80000000089509,-14.1814782866676)) ;
#137228=CARTESIAN_POINT('Ctrl Pts',(4.5320568585877,-2.80000000044794,-14.1782496883795)) ;
#137229=CARTESIAN_POINT('Ctrl Pts',(4.53520648971123,-2.80000000018876,
-14.1751335191281)) ;
#137230=CARTESIAN_POINT('Ctrl Pts',(4.53849565154302,-2.80000000008376,
-14.1721434928059)) ;
#137231=CARTESIAN_POINT('Ctrl Pts',(4.54178481337482,-2.79999999997876,
-14.1691534664838)) ;
#137232=CARTESIAN_POINT('Ctrl Pts',(4.54521363891049,-2.8,-14.1662897578218)) ;
#137233=CARTESIAN_POINT('Ctrl Pts',(4.54879236168087,-2.8,-14.1635655565195)) ;
#137234=CARTESIAN_POINT('',(4.4,-2.8,-13.7168453788272)) ;
#137235=CARTESIAN_POINT('Ctrl Pts',(4.54879236168109,-2.79999999812176,
-14.1635655565192)) ;
#137236=CARTESIAN_POINT('Ctrl Pts',(4.54599316991904,-2.79999999835896,
-14.1615756143355)) ;
#137237=CARTESIAN_POINT('Ctrl Pts',(4.54327885465676,-2.7999999985882,-14.1594726568399)) ;
#137238=CARTESIAN_POINT('Ctrl Pts',(4.52311604063302,-2.80000000023133,
-14.1426310596931)) ;
#137239=CARTESIAN_POINT('Ctrl Pts',(4.5088678063233,-2.80000000100534,-14.1242421996432)) ;
#137240=CARTESIAN_POINT('Ctrl Pts',(4.48892103801306,-2.79999999510253,
-14.0931290218304)) ;
#137241=CARTESIAN_POINT('Ctrl Pts',(4.48186523313291,-2.79999999099551,
-14.0805832050237)) ;
#137242=CARTESIAN_POINT('Ctrl Pts',(4.46162186753409,-2.79999997126272,
-14.0402567139419)) ;
#137243=CARTESIAN_POINT('Ctrl Pts',(4.45052849087263,-2.7999999685384,-14.0113189617092)) ;
#137244=CARTESIAN_POINT('Ctrl Pts',(4.43813540717736,-2.79999997674815,
-13.9729060591291)) ;
#137245=CARTESIAN_POINT('Ctrl Pts',(4.43535270120344,-2.79999997903695,
-13.9637502640508)) ;
#137246=CARTESIAN_POINT('Ctrl Pts',(4.4167777258757,-2.79999999273252,-13.8986688014857)) ;
#137247=CARTESIAN_POINT('Ctrl Pts',(4.40678488790757,-2.79999999887621,
-13.8417195184913)) ;
#137248=CARTESIAN_POINT('Ctrl Pts',(4.40081887576491,-2.80000000006435,
-13.7616198967592)) ;
#137249=CARTESIAN_POINT('Ctrl Pts',(4.4,-2.8,-13.7393018981773)) ;
#137250=CARTESIAN_POINT('Ctrl Pts',(4.4,-2.8,-13.7168453788272)) ;
#137251=CARTESIAN_POINT('',(4.4,-2.8,-12.7)) ;
#137252=CARTESIAN_POINT('',(4.4,-2.8,-12.7)) ;
#137253=CARTESIAN_POINT('',(3.7,-2.8,-12.7)) ;
#137254=CARTESIAN_POINT('',(3.6,-2.8,-12.7)) ;
#137255=CARTESIAN_POINT('',(3.7,-2.8,-22.86)) ;
#137256=CARTESIAN_POINT('',(3.7,-2.8,-22.86)) ;
#137257=CARTESIAN_POINT('',(4.4,-2.8,-22.86)) ;
#137258=CARTESIAN_POINT('',(3.6,-2.8,-22.86)) ;
#137259=CARTESIAN_POINT('',(4.4,-2.8,-17.78)) ;
#137260=CARTESIAN_POINT('Origin',(4.5,-2.8,-17.78)) ;
#137261=CARTESIAN_POINT('',(4.5,-2.4,-18.3578583129651)) ;
#137262=CARTESIAN_POINT('',(4.5,-2.4,-17.2021416870349)) ;
#137263=CARTESIAN_POINT('',(4.5,-2.4,-17.78)) ;
#137264=CARTESIAN_POINT('',(4.5,-2.7,-16.7631546211728)) ;
#137265=CARTESIAN_POINT('Origin',(4.5,0.,-15.24)) ;
#137266=CARTESIAN_POINT('',(4.5,-2.7,-18.7968453788272)) ;
#137267=CARTESIAN_POINT('',(4.5,-2.7,-17.78)) ;
#137268=CARTESIAN_POINT('Origin',(4.5,0.,-20.32)) ;
#137269=CARTESIAN_POINT('Origin',(4.5,-2.3,-17.78)) ;
#137270=CARTESIAN_POINT('',(12.7,-2.3,-22.2821416870349)) ;
#137271=CARTESIAN_POINT('',(4.6,-2.3,-22.2821416870349)) ;
#137272=CARTESIAN_POINT('',(4.5,-2.3,-22.2821416870349)) ;
#137273=CARTESIAN_POINT('',(4.6,-2.3,-22.86)) ;
#137274=CARTESIAN_POINT('',(4.6,-2.3,-22.86)) ;
#137275=CARTESIAN_POINT('',(12.7,-2.3,-22.86)) ;
#137276=CARTESIAN_POINT('',(4.5,-2.3,-22.86)) ;
#137277=CARTESIAN_POINT('',(12.7,-2.3,-17.78)) ;
#137278=CARTESIAN_POINT('Origin',(0.,0.,-22.86)) ;
#137279=CARTESIAN_POINT('Origin',(3.3,10.85,-22.86)) ;
#137280=CARTESIAN_POINT('Origin',(3.85,6.92431432344521,-22.86)) ;
#137281=CARTESIAN_POINT('Origin',(4.05,3.77568567655479,-22.86)) ;
#137282=CARTESIAN_POINT('Origin',(4.55912712210514,2.85,-22.86)) ;
#137283=CARTESIAN_POINT('Origin',(12.7,2.65,-22.86)) ;
#137284=CARTESIAN_POINT('Origin',(12.7,-2.2,-22.86)) ;
#137285=CARTESIAN_POINT('Origin',(4.6,-2.4,-22.86)) ;
#137286=CARTESIAN_POINT('Origin',(4.4,-2.7,-22.86)) ;
#137287=CARTESIAN_POINT('Origin',(3.7,-2.9,-22.86)) ;
#137288=CARTESIAN_POINT('Origin',(3.5,-3.95,-22.86)) ;
#137289=CARTESIAN_POINT('Origin',(-5.3,-3.95,-22.86)) ;
#137290=CARTESIAN_POINT('Origin',(-5.3,5.19009804864072,-22.86)) ;
#137291=CARTESIAN_POINT('Origin',(-4.8,10.3,-22.86)) ;
#137292=CARTESIAN_POINT('Origin',(-4.8,10.85,-22.86)) ;
#137293=CARTESIAN_POINT('Origin',(-4.65,1.95,-22.32)) ;
#137294=CARTESIAN_POINT('',(-4.66204490261456,3.21928058320648,-22.32)) ;
#137295=CARTESIAN_POINT('',(-5.3,3.9369800677651,-22.32)) ;
#137296=CARTESIAN_POINT('',(-5.47474093186837,4.13356361611701,-22.32)) ;
#137297=CARTESIAN_POINT('',(-5.3,-1.88819660112501,-22.32)) ;
#137298=CARTESIAN_POINT('',(-5.3,-2.05,-22.32)) ;
#137299=CARTESIAN_POINT('',(-4.66204490261456,-1.5692190524323,-22.32)) ;
#137300=CARTESIAN_POINT('',(-4.69472135955,-1.58555728090001,-22.32)) ;
#137301=CARTESIAN_POINT('',(-4.66204490261456,3.35625,-22.32)) ;
#137302=CARTESIAN_POINT('Origin',(-5.4,1.95,-18.32)) ;
#137303=CARTESIAN_POINT('',(-4.66204490261456,-1.5692190524323,-18.32)) ;
#137304=CARTESIAN_POINT('',(-5.3,-1.88819660112502,-18.32)) ;
#137305=CARTESIAN_POINT('',(-5.44472135955,-1.96055728090001,-18.32)) ;
#137306=CARTESIAN_POINT('',(-5.3,3.9369800677651,-18.32)) ;
#137307=CARTESIAN_POINT('',(-5.3,4.20000000000001,-18.32)) ;
#137308=CARTESIAN_POINT('',(-4.66204490261456,3.21928058320648,-18.32)) ;
#137309=CARTESIAN_POINT('',(-4.72474093186837,3.28981361611701,-18.32)) ;
#137310=CARTESIAN_POINT('',(-4.66204490261456,-1.67500000000001,-18.32)) ;
#137311=CARTESIAN_POINT('Origin',(-4.65,1.95,-18.32)) ;
#137312=CARTESIAN_POINT('',(-3.33134808452128,1.85,-18.6423371348948)) ;
#137313=CARTESIAN_POINT('',(-3.48082994825801,1.91712723223402,-18.6057971237592)) ;
#137314=CARTESIAN_POINT('Origin',(-3.34328863644916,2.02341244982155,-18.6394183333124)) ;
#137315=CARTESIAN_POINT('',(-2.4,1.85,-18.87)) ;
#137316=CARTESIAN_POINT('',(-4.65,1.85,-18.32)) ;
#137317=CARTESIAN_POINT('',(-2.4,-0.95,-18.87)) ;
#137318=CARTESIAN_POINT('',(-2.4,1.95,-18.87)) ;
#137319=CARTESIAN_POINT('',(-3.3526478932023,-0.95,-18.637130514995)) ;
#137320=CARTESIAN_POINT('',(-3.39999999999998,-0.95,-18.6255555555556)) ;
#137321=CARTESIAN_POINT('',(-3.44209061230229,-0.971114561800017,-18.615266739215)) ;
#137322=CARTESIAN_POINT('Origin',(-3.36201220558082,-1.11033257691485,-18.634841460858)) ;
#137323=CARTESIAN_POINT('',(-4.63829959356686,-1.5692190524323,-18.3228600993503)) ;
#137324=CARTESIAN_POINT('',(-4.68814869588294,-1.59414360359034,-18.3106747632286)) ;
#137325=CARTESIAN_POINT('',(-4.63829959356686,3.21928058320648,-18.3228600993503)) ;
#137326=CARTESIAN_POINT('',(-4.63829959356686,3.35625,-18.3228600993503)) ;
#137327=CARTESIAN_POINT('',(-3.45989661114215,1.89357722797868,-18.6109141617208)) ;
#137328=CARTESIAN_POINT('Origin',(-2.4,1.95,-18.87)) ;
#137329=CARTESIAN_POINT('',(-2.4,1.85,-21.77)) ;
#137330=CARTESIAN_POINT('',(-2.4,-0.95,-21.77)) ;
#137331=CARTESIAN_POINT('',(-2.4,1.95,-21.77)) ;
#137332=CARTESIAN_POINT('',(-2.4,-1.05,-21.667055690472)) ;
#137333=CARTESIAN_POINT('Origin',(-2.4,-0.950000000000066,-21.6670556904721)) ;
#137334=CARTESIAN_POINT('',(-2.4,-1.05,-18.972944309528)) ;
#137335=CARTESIAN_POINT('',(-2.4,-1.05,-18.87)) ;
#137336=CARTESIAN_POINT('Origin',(-2.4,-0.949999999999802,-18.9729443095282)) ;
#137337=CARTESIAN_POINT('',(-2.4,1.95,-18.972944309528)) ;
#137338=CARTESIAN_POINT('Origin',(-2.4,1.84999999999981,-18.9729443095282)) ;
#137339=CARTESIAN_POINT('',(-2.4,1.95,-21.667055690472)) ;
#137340=CARTESIAN_POINT('',(-2.4,1.95,-18.87)) ;
#137341=CARTESIAN_POINT('Origin',(-2.4,1.85000000000024,-21.6670556904722)) ;
#137342=CARTESIAN_POINT('Origin',(-2.4,1.95,-21.77)) ;
#137343=CARTESIAN_POINT('',(-3.3526478932023,-0.95,-22.002869485005)) ;
#137344=CARTESIAN_POINT('',(-3.44209061230229,-0.971114561800017,-22.024733260785)) ;
#137345=CARTESIAN_POINT('Origin',(-3.36201220558296,-1.11033257690641,-22.0051585391426)) ;
#137346=CARTESIAN_POINT('',(-2.4,-0.95,-21.77)) ;
#137347=CARTESIAN_POINT('',(-3.33134808452128,1.85,-21.9976628651052)) ;
#137348=CARTESIAN_POINT('',(-2.4,1.85,-21.77)) ;
#137349=CARTESIAN_POINT('',(-3.48082994825801,1.91712723223402,-22.0342028762408)) ;
#137350=CARTESIAN_POINT('Origin',(-3.34328863644886,2.0234124498222,-22.0005816666875)) ;
#137351=CARTESIAN_POINT('',(-4.63829959356686,3.21928058320648,-22.3171399006497)) ;
#137352=CARTESIAN_POINT('',(-4.70989661114216,3.29982722797869,-22.3346413938348)) ;
#137353=CARTESIAN_POINT('',(-4.63829959356686,-1.5692190524323,-22.3171399006497)) ;
#137354=CARTESIAN_POINT('',(-4.63829959356686,-1.67500000000001,-22.3171399006497)) ;
#137355=CARTESIAN_POINT('',(-3.43814869588292,-0.969143603590331,-22.0237696812158)) ;
#137356=CARTESIAN_POINT('Origin',(0.,1.95,-20.32)) ;
#137357=CARTESIAN_POINT('',(-3.35509339356897,1.95,-18.7394770355445)) ;
#137358=CARTESIAN_POINT('',(0.175392621986784,1.95,-19.6024847282359)) ;
#137359=CARTESIAN_POINT('',(-3.35509339356897,1.95,-21.9005229644555)) ;
#137360=CARTESIAN_POINT('',(-3.35509339356897,1.95,-22.0144444444444)) ;
#137361=CARTESIAN_POINT('',(0.175392621986784,1.95,-21.0375152717641)) ;
#137362=CARTESIAN_POINT('Origin',(0.,-1.05,-20.32)) ;
#137363=CARTESIAN_POINT('',(-3.37639320225,-1.05,-21.9057295843553)) ;
#137364=CARTESIAN_POINT('',(-3.42374530904768,-1.05,-21.9173045437948)) ;
#137365=CARTESIAN_POINT('',(-3.37639320225,-1.05,-18.7342704156447)) ;
#137366=CARTESIAN_POINT('',(-3.37639320225,-1.05,-20.32)) ;
#137367=CARTESIAN_POINT('',(-2.4237453090477,-1.05,-18.9671399006497)) ;
#137368=CARTESIAN_POINT('Origin',(-3.39999999999998,-1.05,-20.32)) ;
#137369=CARTESIAN_POINT('',(-3.4211145618,-1.06055728090001,-18.7124066398647)) ;
#137370=CARTESIAN_POINT('',(-3.4211145618,-1.06055728090001,-21.9275933601353)) ;
#137371=CARTESIAN_POINT('',(-3.4211145618,-1.06055728090001,-20.32)) ;
#137372=CARTESIAN_POINT('',(-4.61732354306457,-1.65866177153229,-22.22)) ;
#137373=CARTESIAN_POINT('',(-4.66717264538064,-1.68358632269033,-22.2321853361217)) ;
#137374=CARTESIAN_POINT('',(-5.34472135954999,-2.022360679775,-22.22)) ;
#137375=CARTESIAN_POINT('',(-5.4,-2.05,-22.22)) ;
#137376=CARTESIAN_POINT('',(-5.34472135954999,-2.022360679775,-18.42)) ;
#137377=CARTESIAN_POINT('',(-5.34472135954999,-2.022360679775,-18.32)) ;
#137378=CARTESIAN_POINT('',(-4.61732354306457,-1.65866177153229,-18.42)) ;
#137379=CARTESIAN_POINT('',(-4.65,-1.67500000000001,-18.42)) ;
#137380=CARTESIAN_POINT('',(-3.41717264538063,-1.05858632269032,-18.7133702194339)) ;
#137381=CARTESIAN_POINT('Origin',(-5.4,4.20000000000001,-17.78)) ;
#137382=CARTESIAN_POINT('',(-5.37474093186837,4.17158354835192,-18.42)) ;
#137383=CARTESIAN_POINT('',(-5.37474093186837,4.17158354835192,-22.22)) ;
#137384=CARTESIAN_POINT('',(-5.37474093186837,4.17158354835192,-22.32)) ;
#137385=CARTESIAN_POINT('',(-4.58730397074619,3.28571696708947,-22.22)) ;
#137386=CARTESIAN_POINT('',(-4.65,3.35625,-22.22)) ;
#137387=CARTESIAN_POINT('',(-3.42983432543734,1.98356361611701,-21.9370629755912)) ;
#137388=CARTESIAN_POINT('',(-3.40890098832149,1.96001361186167,-21.9319459376295)) ;
#137389=CARTESIAN_POINT('',(-3.42983432543734,1.98356361611701,-18.7029370244088)) ;
#137390=CARTESIAN_POINT('',(-3.42983432543734,1.98356361611701,-18.6255555555556)) ;
#137391=CARTESIAN_POINT('',(-4.58730397074619,3.28571696708947,-18.42)) ;
#137392=CARTESIAN_POINT('',(-4.65890098832149,3.36626361186168,-18.4024985068149)) ;
#137393=CARTESIAN_POINT('',(-5.4,4.20000000000001,-18.42)) ;
#137394=CARTESIAN_POINT('Origin',(-3.15,-3.9,-19.32)) ;
#137395=CARTESIAN_POINT('',(-3.15,-3.95,-19.42)) ;
#137396=CARTESIAN_POINT('',(-3.15,-3.85,-19.42)) ;
#137397=CARTESIAN_POINT('',(-3.15,-3.75,-19.42)) ;
#137398=CARTESIAN_POINT('',(-3.15,-3.85,-21.22)) ;
#137399=CARTESIAN_POINT('',(-3.15,-3.85,-19.32)) ;
#137400=CARTESIAN_POINT('',(-3.15,-3.95,-21.22)) ;
#137401=CARTESIAN_POINT('',(-3.15,-4.05,-21.22)) ;
#137402=CARTESIAN_POINT('',(-3.15,-3.95,-19.32)) ;
#137403=CARTESIAN_POINT('Origin',(-4.4,-3.9,-21.32)) ;
#137404=CARTESIAN_POINT('',(-3.25,-3.85,-21.32)) ;
#137405=CARTESIAN_POINT('',(-4.3,-3.85,-21.32)) ;
#137406=CARTESIAN_POINT('',(-4.4,-3.85,-21.32)) ;
#137407=CARTESIAN_POINT('',(-4.3,-3.95,-21.32)) ;
#137408=CARTESIAN_POINT('',(-4.3,-4.05,-21.32)) ;
#137409=CARTESIAN_POINT('',(-3.25,-3.95,-21.32)) ;
#137410=CARTESIAN_POINT('',(-4.4,-3.95,-21.32)) ;
#137411=CARTESIAN_POINT('',(-3.25,-3.75,-21.32)) ;
#137412=CARTESIAN_POINT('Origin',(-4.4,-3.9,-19.32)) ;
#137413=CARTESIAN_POINT('',(-4.4,-3.85,-21.22)) ;
#137414=CARTESIAN_POINT('',(-4.4,-3.85,-19.42)) ;
#137415=CARTESIAN_POINT('',(-4.4,-3.85,-19.32)) ;
#137416=CARTESIAN_POINT('',(-4.4,-3.95,-19.42)) ;
#137417=CARTESIAN_POINT('',(-4.4,-4.05,-19.42)) ;
#137418=CARTESIAN_POINT('',(-4.4,-3.95,-21.22)) ;
#137419=CARTESIAN_POINT('',(-4.4,-3.95,-19.32)) ;
#137420=CARTESIAN_POINT('',(-4.4,-3.75,-21.22)) ;
#137421=CARTESIAN_POINT('Origin',(-4.4,-3.9,-19.32)) ;
#137422=CARTESIAN_POINT('',(-4.3,-3.95,-19.32)) ;
#137423=CARTESIAN_POINT('',(-4.3,-3.85,-19.32)) ;
#137424=CARTESIAN_POINT('',(-4.3,-3.75,-19.32)) ;
#137425=CARTESIAN_POINT('',(-3.25,-3.85,-19.32)) ;
#137426=CARTESIAN_POINT('',(-4.4,-3.85,-19.32)) ;
#137427=CARTESIAN_POINT('',(-3.25,-3.95,-19.32)) ;
#137428=CARTESIAN_POINT('',(-3.25,-4.05,-19.32)) ;
#137429=CARTESIAN_POINT('',(-4.4,-3.95,-19.32)) ;
#137430=CARTESIAN_POINT('Origin',(0.,-3.75,-20.32)) ;
#137431=CARTESIAN_POINT('',(-3.25,-3.75,-19.42)) ;
#137432=CARTESIAN_POINT('',(-4.3,-3.75,-19.42)) ;
#137433=CARTESIAN_POINT('',(-1.56125112837913E-16,-3.75,-19.42)) ;
#137434=CARTESIAN_POINT('',(-4.3,-3.75,-21.22)) ;
#137435=CARTESIAN_POINT('',(-4.3,-3.75,-20.32)) ;
#137436=CARTESIAN_POINT('',(-3.25,-3.75,-21.22)) ;
#137437=CARTESIAN_POINT('',(-1.56125112837913E-16,-3.75,-21.22)) ;
#137438=CARTESIAN_POINT('',(-3.25,-3.75,-20.32)) ;
#137439=CARTESIAN_POINT('',(-4.15,-3.75,-21.17)) ;
#137440=CARTESIAN_POINT('',(-3.4,-3.75,-21.17)) ;
#137441=CARTESIAN_POINT('',(-4.15,-3.75,-21.17)) ;
#137442=CARTESIAN_POINT('',(-4.25,-3.75,-21.07)) ;
#137443=CARTESIAN_POINT('Origin',(-4.15,-3.75,-21.07)) ;
#137444=CARTESIAN_POINT('',(-4.25,-3.75,-19.57)) ;
#137445=CARTESIAN_POINT('',(-4.25,-3.75,-19.57)) ;
#137446=CARTESIAN_POINT('',(-4.15,-3.75,-19.47)) ;
#137447=CARTESIAN_POINT('Origin',(-4.15,-3.75,-19.57)) ;
#137448=CARTESIAN_POINT('',(-3.4,-3.75,-19.47)) ;
#137449=CARTESIAN_POINT('',(-3.4,-3.75,-19.47)) ;
#137450=CARTESIAN_POINT('',(-3.3,-3.75,-19.57)) ;
#137451=CARTESIAN_POINT('Origin',(-3.4,-3.75,-19.57)) ;
#137452=CARTESIAN_POINT('',(-3.3,-3.75,-21.07)) ;
#137453=CARTESIAN_POINT('',(-3.3,-3.75,-21.07)) ;
#137454=CARTESIAN_POINT('Origin',(-3.4,-3.75,-21.07)) ;
#137455=CARTESIAN_POINT('Origin',(-3.4,-3.75,-21.07)) ;
#137456=CARTESIAN_POINT('',(-3.4,-3.9,-21.17)) ;
#137457=CARTESIAN_POINT('',(-3.3,-3.9,-21.07)) ;
#137458=CARTESIAN_POINT('Origin',(-3.4,-3.9,-21.07)) ;
#137459=CARTESIAN_POINT('',(-3.4,-3.75,-21.17)) ;
#137460=CARTESIAN_POINT('',(-3.3,-3.75,-21.07)) ;
#137461=CARTESIAN_POINT('Origin',(-4.15,-3.75,-21.17)) ;
#137462=CARTESIAN_POINT('',(-4.15,-3.9,-21.17)) ;
#137463=CARTESIAN_POINT('',(-4.15,-3.9,-21.17)) ;
#137464=CARTESIAN_POINT('',(-4.15,-3.75,-21.17)) ;
#137465=CARTESIAN_POINT('Origin',(-4.15,-3.75,-21.07)) ;
#137466=CARTESIAN_POINT('',(-4.25,-3.9,-21.07)) ;
#137467=CARTESIAN_POINT('Origin',(-4.15,-3.9,-21.07)) ;
#137468=CARTESIAN_POINT('',(-4.25,-3.75,-21.07)) ;
#137469=CARTESIAN_POINT('Origin',(-4.25,-3.75,-19.57)) ;
#137470=CARTESIAN_POINT('',(-4.25,-3.9,-19.57)) ;
#137471=CARTESIAN_POINT('',(-4.25,-3.9,-19.57)) ;
#137472=CARTESIAN_POINT('',(-4.25,-3.75,-19.57)) ;
#137473=CARTESIAN_POINT('Origin',(-4.15,-3.75,-19.57)) ;
#137474=CARTESIAN_POINT('',(-4.15,-3.9,-19.47)) ;
#137475=CARTESIAN_POINT('Origin',(-4.15,-3.9,-19.57)) ;
#137476=CARTESIAN_POINT('',(-4.15,-3.75,-19.47)) ;
#137477=CARTESIAN_POINT('Origin',(-3.4,-3.75,-19.47)) ;
#137478=CARTESIAN_POINT('',(-3.4,-3.9,-19.47)) ;
#137479=CARTESIAN_POINT('',(-3.4,-3.9,-19.47)) ;
#137480=CARTESIAN_POINT('',(-3.4,-3.75,-19.47)) ;
#137481=CARTESIAN_POINT('Origin',(-3.4,-3.75,-19.57)) ;
#137482=CARTESIAN_POINT('',(-3.3,-3.9,-19.57)) ;
#137483=CARTESIAN_POINT('Origin',(-3.4,-3.9,-19.57)) ;
#137484=CARTESIAN_POINT('',(-3.3,-3.75,-19.57)) ;
#137485=CARTESIAN_POINT('Origin',(-3.3,-3.75,-21.07)) ;
#137486=CARTESIAN_POINT('',(-3.3,-3.9,-21.07)) ;
#137487=CARTESIAN_POINT('Origin',(0.,-3.9,-20.32)) ;
#137488=CARTESIAN_POINT('Origin',(0.,9.95,-20.32)) ;
#137489=CARTESIAN_POINT('',(-0.230887397576972,9.95,-18.4051394281462)) ;
#137490=CARTESIAN_POINT('Origin',(-0.321518176280637,8.95,-18.4474012543203)) ;
#137491=CARTESIAN_POINT('',(-0.321518176280637,9.05,-18.4474012543203)) ;
#137492=CARTESIAN_POINT('',(1.22782596331729,9.85,-21.769980483939)) ;
#137493=CARTESIAN_POINT('Origin',(-1.22782596331729,8.95,-18.870019516061)) ;
#137494=CARTESIAN_POINT('',(-1.22782596331729,9.05,-18.870019516061)) ;
#137495=CARTESIAN_POINT('',(-1.22782596331729,9.85,-18.870019516061)) ;
#137496=CARTESIAN_POINT('Origin',(0.,8.95,-20.32)) ;
#137497=CARTESIAN_POINT('',(-0.362523114814661,8.95,-20.4890473046963)) ;
#137498=CARTESIAN_POINT('',(0.36252311481466,8.95,-20.1509526953037)) ;
#137499=CARTESIAN_POINT('Origin',(-2.65,10.8,-21.32)) ;
#137500=CARTESIAN_POINT('',(-2.65,10.75,-21.22)) ;
#137501=CARTESIAN_POINT('',(-2.65,10.75,-19.42)) ;
#137502=CARTESIAN_POINT('',(-2.65,10.75,-21.32)) ;
#137503=CARTESIAN_POINT('',(-2.65,10.85,-19.42)) ;
#137504=CARTESIAN_POINT('',(-2.65,10.95,-19.42)) ;
#137505=CARTESIAN_POINT('',(-2.65,10.85,-21.22)) ;
#137506=CARTESIAN_POINT('',(-2.65,10.85,-21.32)) ;
#137507=CARTESIAN_POINT('',(-2.65,10.65,-21.22)) ;
#137508=CARTESIAN_POINT('Origin',(-3.9,10.8,-19.32)) ;
#137509=CARTESIAN_POINT('',(-2.75,10.85,-19.32)) ;
#137510=CARTESIAN_POINT('',(-2.75,10.75,-19.32)) ;
#137511=CARTESIAN_POINT('',(-2.75,10.65,-19.32)) ;
#137512=CARTESIAN_POINT('',(-3.8,10.75,-19.32)) ;
#137513=CARTESIAN_POINT('',(-3.9,10.75,-19.32)) ;
#137514=CARTESIAN_POINT('',(-3.8,10.85,-19.32)) ;
#137515=CARTESIAN_POINT('',(-3.8,10.95,-19.32)) ;
#137516=CARTESIAN_POINT('',(-3.9,10.85,-19.32)) ;
#137517=CARTESIAN_POINT('Origin',(-3.9,10.8,-21.32)) ;
#137518=CARTESIAN_POINT('',(-3.9,10.85,-19.42)) ;
#137519=CARTESIAN_POINT('',(-3.9,10.75,-19.42)) ;
#137520=CARTESIAN_POINT('',(-3.9,10.65,-19.42)) ;
#137521=CARTESIAN_POINT('',(-3.9,10.75,-21.22)) ;
#137522=CARTESIAN_POINT('',(-3.9,10.75,-21.32)) ;
#137523=CARTESIAN_POINT('',(-3.9,10.85,-21.22)) ;
#137524=CARTESIAN_POINT('',(-3.9,10.95,-21.22)) ;
#137525=CARTESIAN_POINT('',(-3.9,10.85,-21.32)) ;
#137526=CARTESIAN_POINT('Origin',(-3.9,10.8,-21.32)) ;
#137527=CARTESIAN_POINT('',(-3.8,10.75,-21.32)) ;
#137528=CARTESIAN_POINT('',(-2.75,10.75,-21.32)) ;
#137529=CARTESIAN_POINT('',(-3.9,10.75,-21.32)) ;
#137530=CARTESIAN_POINT('',(-2.75,10.85,-21.32)) ;
#137531=CARTESIAN_POINT('',(-2.75,10.95,-21.32)) ;
#137532=CARTESIAN_POINT('',(-3.8,10.85,-21.32)) ;
#137533=CARTESIAN_POINT('',(-3.9,10.85,-21.32)) ;
#137534=CARTESIAN_POINT('',(-3.8,10.65,-21.32)) ;
#137535=CARTESIAN_POINT('Origin',(0.,10.65,-20.32)) ;
#137536=CARTESIAN_POINT('',(-3.8,10.65,-19.42)) ;
#137537=CARTESIAN_POINT('',(-2.75,10.65,-19.42)) ;
#137538=CARTESIAN_POINT('',(1.56125112837912E-16,10.65,-19.42)) ;
#137539=CARTESIAN_POINT('',(-2.75,10.65,-21.22)) ;
#137540=CARTESIAN_POINT('',(-2.75,10.65,-20.32)) ;
#137541=CARTESIAN_POINT('',(-3.8,10.65,-21.22)) ;
#137542=CARTESIAN_POINT('',(-1.56125112837913E-16,10.65,-21.22)) ;
#137543=CARTESIAN_POINT('',(-3.8,10.65,-20.32)) ;
#137544=CARTESIAN_POINT('',(-3.65,10.65,-19.47)) ;
#137545=CARTESIAN_POINT('',(-2.9,10.65,-19.47)) ;
#137546=CARTESIAN_POINT('',(-3.65,10.65,-19.47)) ;
#137547=CARTESIAN_POINT('',(-3.75,10.65,-19.57)) ;
#137548=CARTESIAN_POINT('Origin',(-3.65,10.65,-19.57)) ;
#137549=CARTESIAN_POINT('',(-3.75,10.65,-21.07)) ;
#137550=CARTESIAN_POINT('',(-3.75,10.65,-21.07)) ;
#137551=CARTESIAN_POINT('',(-3.65,10.65,-21.17)) ;
#137552=CARTESIAN_POINT('Origin',(-3.65,10.65,-21.07)) ;
#137553=CARTESIAN_POINT('',(-2.9,10.65,-21.17)) ;
#137554=CARTESIAN_POINT('',(-2.9,10.65,-21.17)) ;
#137555=CARTESIAN_POINT('',(-2.8,10.65,-21.07)) ;
#137556=CARTESIAN_POINT('Origin',(-2.9,10.65,-21.07)) ;
#137557=CARTESIAN_POINT('',(-2.8,10.65,-19.57)) ;
#137558=CARTESIAN_POINT('',(-2.8,10.65,-19.57)) ;
#137559=CARTESIAN_POINT('Origin',(-2.9,10.65,-19.57)) ;
#137560=CARTESIAN_POINT('Origin',(-2.9,10.65,-19.57)) ;
#137561=CARTESIAN_POINT('',(-2.8,10.7,-19.57)) ;
#137562=CARTESIAN_POINT('',(-2.8,10.65,-19.57)) ;
#137563=CARTESIAN_POINT('',(-2.9,10.7,-19.47)) ;
#137564=CARTESIAN_POINT('Origin',(-2.9,10.7,-19.57)) ;
#137565=CARTESIAN_POINT('',(-2.9,10.65,-19.47)) ;
#137566=CARTESIAN_POINT('Origin',(-3.65,10.65,-19.47)) ;
#137567=CARTESIAN_POINT('',(-3.65,10.7,-19.47)) ;
#137568=CARTESIAN_POINT('',(-3.65,10.7,-19.47)) ;
#137569=CARTESIAN_POINT('',(-3.65,10.65,-19.47)) ;
#137570=CARTESIAN_POINT('Origin',(-3.65,10.65,-19.57)) ;
#137571=CARTESIAN_POINT('',(-3.75,10.7,-19.57)) ;
#137572=CARTESIAN_POINT('Origin',(-3.65,10.7,-19.57)) ;
#137573=CARTESIAN_POINT('',(-3.75,10.65,-19.57)) ;
#137574=CARTESIAN_POINT('Origin',(-3.75,10.65,-21.07)) ;
#137575=CARTESIAN_POINT('',(-3.75,10.7,-21.07)) ;
#137576=CARTESIAN_POINT('',(-3.75,10.7,-21.07)) ;
#137577=CARTESIAN_POINT('',(-3.75,10.65,-21.07)) ;
#137578=CARTESIAN_POINT('Origin',(-3.65,10.65,-21.07)) ;
#137579=CARTESIAN_POINT('',(-3.65,10.7,-21.17)) ;
#137580=CARTESIAN_POINT('Origin',(-3.65,10.7,-21.07)) ;
#137581=CARTESIAN_POINT('',(-3.65,10.65,-21.17)) ;
#137582=CARTESIAN_POINT('Origin',(-2.9,10.65,-21.17)) ;
#137583=CARTESIAN_POINT('',(-2.9,10.7,-21.17)) ;
#137584=CARTESIAN_POINT('',(-2.9,10.7,-21.17)) ;
#137585=CARTESIAN_POINT('',(-2.9,10.65,-21.17)) ;
#137586=CARTESIAN_POINT('Origin',(-2.9,10.65,-21.07)) ;
#137587=CARTESIAN_POINT('',(-2.8,10.7,-21.07)) ;
#137588=CARTESIAN_POINT('Origin',(-2.9,10.7,-21.07)) ;
#137589=CARTESIAN_POINT('',(-2.8,10.65,-21.07)) ;
#137590=CARTESIAN_POINT('Origin',(-2.8,10.65,-19.57)) ;
#137591=CARTESIAN_POINT('',(-2.8,10.7,-19.57)) ;
#137592=CARTESIAN_POINT('Origin',(0.,10.8,-20.32)) ;
#137593=CARTESIAN_POINT('',(-3.65,10.8,-19.57)) ;
#137594=CARTESIAN_POINT('',(-2.9,10.8,-19.57)) ;
#137595=CARTESIAN_POINT('',(0.,10.8,-19.57)) ;
#137596=CARTESIAN_POINT('',(-2.9,10.8,-21.07)) ;
#137597=CARTESIAN_POINT('',(-2.9,10.8,-20.32)) ;
#137598=CARTESIAN_POINT('',(-3.65,10.8,-21.07)) ;
#137599=CARTESIAN_POINT('',(0.,10.8,-21.07)) ;
#137600=CARTESIAN_POINT('',(-3.65,10.8,-20.32)) ;
#137601=CARTESIAN_POINT('Origin',(4.5,2.75,-21.695)) ;
#137602=CARTESIAN_POINT('',(4.5,2.63356010126946,-21.7144066497884)) ;
#137603=CARTESIAN_POINT('',(4.6,2.11643989873054,-21.8005933502116)) ;
#137604=CARTESIAN_POINT('',(4.6,2.11643989873054,-21.8005933502116)) ;
#137605=CARTESIAN_POINT('',(12.7,2.11643989873054,-21.8005933502116)) ;
#137606=CARTESIAN_POINT('',(12.8,2.11643989873054,-21.8005933502116)) ;
#137607=CARTESIAN_POINT('',(12.7,2.75,-21.695)) ;
#137608=CARTESIAN_POINT('Origin',(4.5,2.,-21.82)) ;
#137609=CARTESIAN_POINT('',(4.6,2.,-21.7019539578284)) ;
#137610=CARTESIAN_POINT('',(4.6,2.,-18.82)) ;
#137611=CARTESIAN_POINT('',(12.7,2.,-21.7019539578284)) ;
#137612=CARTESIAN_POINT('',(12.7,2.,-21.82)) ;
#137613=CARTESIAN_POINT('',(4.5,2.,-21.7019539578284)) ;
#137614=CARTESIAN_POINT('Origin',(4.5,2.,-18.82)) ;
#137615=CARTESIAN_POINT('',(4.6,2.63356010126946,-18.9255933502116)) ;
#137616=CARTESIAN_POINT('',(4.6,2.63356010126947,-18.9255933502116)) ;
#137617=CARTESIAN_POINT('',(4.5,2.63356010126946,-18.9255933502116)) ;
#137618=CARTESIAN_POINT('',(12.7,2.,-18.82)) ;
#137619=CARTESIAN_POINT('Origin',(4.5,0.,-20.32)) ;
#137620=CARTESIAN_POINT('',(4.5,2.72431432344521,-19.012634816645)) ;
#137621=CARTESIAN_POINT('',(4.5,2.72431432344521,-20.32)) ;
#137622=CARTESIAN_POINT('',(4.5,2.61712020253893,-19.0242327425948)) ;
#137623=CARTESIAN_POINT('Origin',(4.5,2.65,-18.8269539578284)) ;
#137624=CARTESIAN_POINT('',(4.5,2.1,-18.9380460421716)) ;
#137625=CARTESIAN_POINT('',(4.5,2.1,-18.9380460421716)) ;
#137626=CARTESIAN_POINT('',(4.5,2.1,-21.7019539578284)) ;
#137627=CARTESIAN_POINT('',(4.5,2.1,-21.82)) ;
#137628=CARTESIAN_POINT('',(4.5,2.61712020253893,-21.6157672574052)) ;
#137629=CARTESIAN_POINT('Origin',(10.3,0.,-20.32)) ;
#137630=CARTESIAN_POINT('Origin',(0.584645609909621,0.,-20.32)) ;
#137631=CARTESIAN_POINT('',(4.6,-2.32258064516129,-18.4211532060953)) ;
#137632=CARTESIAN_POINT('',(4.6,-2.79310344827574,-19.2252063540419)) ;
#137633=CARTESIAN_POINT('Origin',(4.6,0.,-20.32)) ;
#137634=CARTESIAN_POINT('',(4.6,-2.79310344827574,-21.4147936459581)) ;
#137635=CARTESIAN_POINT('Origin',(4.6,0.,-20.32)) ;
#137636=CARTESIAN_POINT('',(4.6,-2.32258064516129,-22.2188467939047)) ;
#137637=CARTESIAN_POINT('Origin',(4.6,0.,-20.32)) ;
#137638=CARTESIAN_POINT('',(12.7,-2.32258064516129,-22.2188467939047)) ;
#137639=CARTESIAN_POINT('',(0.584645609909621,-2.32258064516129,-22.2188467939047)) ;
#137640=CARTESIAN_POINT('',(12.7,-2.32258064516129,-18.4211532060953)) ;
#137641=CARTESIAN_POINT('Origin',(12.7,0.,-20.32)) ;
#137642=CARTESIAN_POINT('',(0.584645609909621,-2.32258064516129,-18.4211532060953)) ;
#137643=CARTESIAN_POINT('Ctrl Pts',(-5.37474093186837,4.17158354835192,
-18.42)) ;
#137644=CARTESIAN_POINT('Ctrl Pts',(-5.4,4.2,-18.42)) ;
#137645=CARTESIAN_POINT('Ctrl Pts',(-5.4,4.23801993223491,-18.42)) ;
#137646=CARTESIAN_POINT('Ctrl Pts',(-5.37474093064202,4.17158354697228,
-18.3937465640611)) ;
#137647=CARTESIAN_POINT('Ctrl Pts',(-5.4,4.19999999724801,-18.382481412799)) ;
#137648=CARTESIAN_POINT('Ctrl Pts',(-5.4,4.23801992976516,-18.3674931280903)) ;
#137649=CARTESIAN_POINT('Ctrl Pts',(-5.36668583490659,4.14629949399949,
-18.3678012868841)) ;
#137650=CARTESIAN_POINT('Ctrl Pts',(-5.4,4.16739198385624,-18.3446678350657)) ;
#137651=CARTESIAN_POINT('Ctrl Pts',(-5.4,4.20557579169425,-18.3156025737682)) ;
#137652=CARTESIAN_POINT('Ctrl Pts',(-5.33901380460605,4.05944006555652,
-18.3307773568786)) ;
#137653=CARTESIAN_POINT('Ctrl Pts',(-5.4,4.06625640449639,-18.3031326366143)) ;
#137654=CARTESIAN_POINT('Ctrl Pts',(-5.4,4.09411900298411,-18.2415547137572)) ;
#137655=CARTESIAN_POINT('Ctrl Pts',(-5.31962206268972,3.99857154231908,
-18.32)) ;
#137656=CARTESIAN_POINT('Ctrl Pts',(-5.4,3.99346933127516,-18.3020035074265)) ;
#137657=CARTESIAN_POINT('Ctrl Pts',(-5.4,4.0160133758189,-18.2200000004811)) ;
#137658=CARTESIAN_POINT('Ctrl Pts',(-5.3,3.9369800677651,-18.32)) ;
#137659=CARTESIAN_POINT('Ctrl Pts',(-5.4,3.9369800677651,-18.32)) ;
#137660=CARTESIAN_POINT('Ctrl Pts',(-5.4,3.9369800677651,-18.22)) ;
#137661=CARTESIAN_POINT('Origin',(-5.3,4.23801993223491,-18.42)) ;
#137662=CARTESIAN_POINT('Ctrl Pts',(-5.3,3.9369800677651,-18.32)) ;
#137663=CARTESIAN_POINT('Ctrl Pts',(-5.31962206268972,3.99857154231908,
-18.32)) ;
#137664=CARTESIAN_POINT('Ctrl Pts',(-5.33901380460605,4.05944006555653,
-18.3307773568786)) ;
#137665=CARTESIAN_POINT('Ctrl Pts',(-5.36668583490659,4.14629949399949,
-18.3678012868841)) ;
#137666=CARTESIAN_POINT('Ctrl Pts',(-5.37474093064202,4.17158354697228,
-18.3937465640611)) ;
#137667=CARTESIAN_POINT('Ctrl Pts',(-5.37474093186837,4.17158354835192,
-18.42)) ;
#137668=CARTESIAN_POINT('Origin',(-5.3,3.9369800677651,-18.22)) ;
#137669=CARTESIAN_POINT('Origin',(-4.6737453090477,1.85,-18.4171399006497)) ;
#137670=CARTESIAN_POINT('Origin',(-3.35509339356897,1.85,-18.7394770355445)) ;
#137671=CARTESIAN_POINT('Ctrl Pts',(-3.35509339356897,1.95,-18.7394770355445)) ;
#137672=CARTESIAN_POINT('Ctrl Pts',(-3.33134808452128,1.95,-18.6423371348948)) ;
#137673=CARTESIAN_POINT('Ctrl Pts',(-3.33134808452128,1.85,-18.6423371348948)) ;
#137674=CARTESIAN_POINT('Ctrl Pts',(-3.38343213690424,1.95,-18.7256225388029)) ;
#137675=CARTESIAN_POINT('Ctrl Pts',(-3.36046743872486,1.94345445676968,
-18.6352190705343)) ;
#137676=CARTESIAN_POINT('Ctrl Pts',(-3.38803897426452,1.85000000162387,
-18.6284793618465)) ;
#137677=CARTESIAN_POINT('Ctrl Pts',(-3.41101314049054,1.96238978305186,
-18.7121384929161)) ;
#137678=CARTESIAN_POINT('Ctrl Pts',(-3.39538881861725,1.95068928167331,
-18.6266827332266)) ;
#137679=CARTESIAN_POINT('Ctrl Pts',(-3.44316973238528,1.87475949194142,
-18.6150029543058)) ;
#137680=CARTESIAN_POINT('Ctrl Pts',(-3.42983432543734,1.98356361611701,
-18.7029370244088)) ;
#137681=CARTESIAN_POINT('Ctrl Pts',(-3.42093333711585,1.97355000425533,
-18.6204385175939)) ;
#137682=CARTESIAN_POINT('Ctrl Pts',(-3.48082994825801,1.91712723223402,
-18.6057971237592)) ;
#137683=CARTESIAN_POINT('Origin',(-3.50457525730571,1.91712723223402,-18.7029370244088)) ;
#137684=CARTESIAN_POINT('Origin',(-3.36128627567715,2.03621361435819,-18.7364494043352)) ;
#137685=CARTESIAN_POINT('Origin',(-4.05330900605469,2.53445269957662,-18.568802108048)) ;
#137686=CARTESIAN_POINT('Origin',(-4.66204490261456,3.21928058320648,-18.42)) ;
#137687=CARTESIAN_POINT('Origin',(-4.35749955255802,2.87666706439287,-18.42)) ;
#137688=CARTESIAN_POINT('Origin',(-4.66204490261456,3.21928058320648,-18.42)) ;
#137689=CARTESIAN_POINT('Origin',(-5.3,5.2,-18.22)) ;
#137690=CARTESIAN_POINT('Origin',(-5.3,-1.88819660112502,-18.22)) ;
#137691=CARTESIAN_POINT('Origin',(-5.3,4.23801993223491,-17.78)) ;
#137692=CARTESIAN_POINT('Origin',(-5.3,4.23801993223491,-22.22)) ;
#137693=CARTESIAN_POINT('Origin',(-3.35509339356897,2.05,-20.32)) ;
#137694=CARTESIAN_POINT('Origin',(-3.36128627567707,2.03621361435845,-21.9035505956648)) ;
#137695=CARTESIAN_POINT('Origin',(-2.4237453090477,1.85,-21.6728600993503)) ;
#137696=CARTESIAN_POINT('Origin',(-3.35509339356897,1.85,-21.9005229644555)) ;
#137697=CARTESIAN_POINT('Origin',(-4.66204490261456,3.21928058320648,-18.42)) ;
#137698=CARTESIAN_POINT('Origin',(-4.66204490261456,3.21928058320648,-18.42)) ;
#137699=CARTESIAN_POINT('Ctrl Pts',(-5.29976814257746,-1.88802911972918,
-18.3199998273778)) ;
#137700=CARTESIAN_POINT('Ctrl Pts',(-5.4,-1.88802831720455,-18.320232593543)) ;
#137701=CARTESIAN_POINT('Ctrl Pts',(-5.4,-1.88791746283071,-18.2200001624624)) ;
#137702=CARTESIAN_POINT('Ctrl Pts',(-5.31153957531163,-1.92331224822996,
-18.3199864676889)) ;
#137703=CARTESIAN_POINT('Ctrl Pts',(-5.4,-1.92148676945281,-18.3089778925376)) ;
#137704=CARTESIAN_POINT('Ctrl Pts',(-5.4,-1.94671708614657,-18.2199317130282)) ;
#137705=CARTESIAN_POINT('Ctrl Pts',(-5.32318090226694,-1.9581752705225,
-18.3307844972681)) ;
#137706=CARTESIAN_POINT('Ctrl Pts',(-5.4,-1.96527310172481,-18.3121633837529)) ;
#137707=CARTESIAN_POINT('Ctrl Pts',(-5.4,-2.00485091174287,-18.2414960748893)) ;
#137708=CARTESIAN_POINT('Ctrl Pts',(-5.33978950165956,-2.00789652656154,
-18.3678649650196)) ;
#137709=CARTESIAN_POINT('Ctrl Pts',(-5.4,-2.02908601268745,-18.3513665145317)) ;
#137710=CARTESIAN_POINT('Ctrl Pts',(-5.4,-2.087770056524,-18.3156612126361)) ;
#137711=CARTESIAN_POINT('Ctrl Pts',(-5.34461954754097,-2.02234798681676,
-18.3938461447183)) ;
#137712=CARTESIAN_POINT('Ctrl Pts',(-5.4,-2.04997459329993,-18.38567566484)) ;
#137713=CARTESIAN_POINT('Ctrl Pts',(-5.4,-2.1118797455067,-18.3676576869739)) ;
#137714=CARTESIAN_POINT('Ctrl Pts',(-5.34460423617422,-2.02230212313483,
-18.4201247518701)) ;
#137715=CARTESIAN_POINT('Ctrl Pts',(-5.4,-2.04990938338631,-18.4201637542765)) ;
#137716=CARTESIAN_POINT('Ctrl Pts',(-5.4,-2.11180321723903,-18.4202496688804)) ;
#137717=CARTESIAN_POINT('Origin',(-5.29999999999992,-1.88819660112476,-18.4200000000002)) ;
#137718=CARTESIAN_POINT('Origin',(-5.3,-2.11180339887499,-18.42)) ;
#137719=CARTESIAN_POINT('Ctrl Pts',(-5.3,3.9369800677651,-22.32)) ;
#137720=CARTESIAN_POINT('Ctrl Pts',(-5.4,3.9369800677651,-22.32)) ;
#137721=CARTESIAN_POINT('Ctrl Pts',(-5.4,3.9369800677651,-22.42)) ;
#137722=CARTESIAN_POINT('Ctrl Pts',(-5.31962206268973,3.99857154231912,
-22.32)) ;
#137723=CARTESIAN_POINT('Ctrl Pts',(-5.40000000000063,3.993469331275,-22.3379964925736)) ;
#137724=CARTESIAN_POINT('Ctrl Pts',(-5.4,4.01601337581889,-22.4199999995189)) ;
#137725=CARTESIAN_POINT('Ctrl Pts',(-5.33901380460613,4.05944006555646,
-22.3092226431215)) ;
#137726=CARTESIAN_POINT('Ctrl Pts',(-5.40000000000006,4.06625640449647,
-22.3368673633861)) ;
#137727=CARTESIAN_POINT('Ctrl Pts',(-5.4,4.09411900298413,-22.3984452862429)) ;
#137728=CARTESIAN_POINT('Ctrl Pts',(-5.36668583490652,4.14629949399955,
-22.2721987131158)) ;
#137729=CARTESIAN_POINT('Ctrl Pts',(-5.39999999999995,4.16739198385616,
-22.295332164934)) ;
#137730=CARTESIAN_POINT('Ctrl Pts',(-5.4,4.20557579169423,-22.3243974262317)) ;
#137731=CARTESIAN_POINT('Ctrl Pts',(-5.37474093064202,4.17158354697228,
-22.246253435939)) ;
#137732=CARTESIAN_POINT('Ctrl Pts',(-5.4,4.19999999724801,-22.2575185872012)) ;
#137733=CARTESIAN_POINT('Ctrl Pts',(-5.4,4.23801992976516,-22.2725068719098)) ;
#137734=CARTESIAN_POINT('Ctrl Pts',(-5.37474093186837,4.17158354835192,
-22.22)) ;
#137735=CARTESIAN_POINT('Ctrl Pts',(-5.4,4.2,-22.22)) ;
#137736=CARTESIAN_POINT('Ctrl Pts',(-5.4,4.23801993223491,-22.22)) ;
#137737=CARTESIAN_POINT('Origin',(-5.3,3.9369800677651,-22.42)) ;
#137738=CARTESIAN_POINT('Ctrl Pts',(-5.37474093186837,4.17158354835192,
-22.22)) ;
#137739=CARTESIAN_POINT('Ctrl Pts',(-5.37474093064202,4.17158354697228,
-22.246253435939)) ;
#137740=CARTESIAN_POINT('Ctrl Pts',(-5.36668583490652,4.14629949399955,
-22.2721987131158)) ;
#137741=CARTESIAN_POINT('Ctrl Pts',(-5.33901380460613,4.05944006555646,
-22.3092226431215)) ;
#137742=CARTESIAN_POINT('Ctrl Pts',(-5.31962206268973,3.99857154231912,
-22.32)) ;
#137743=CARTESIAN_POINT('Ctrl Pts',(-5.3,3.9369800677651,-22.32)) ;
#137744=CARTESIAN_POINT('Ctrl Pts',(-3.42983432543734,1.98356361611701,
-21.9370629755912)) ;
#137745=CARTESIAN_POINT('Ctrl Pts',(-3.42093333711585,1.97355000425533,
-22.0195614824061)) ;
#137746=CARTESIAN_POINT('Ctrl Pts',(-3.48082994825801,1.91712723223402,
-22.0342028762409)) ;
#137747=CARTESIAN_POINT('Ctrl Pts',(-3.41101314049054,1.96238978305186,
-21.9278615070839)) ;
#137748=CARTESIAN_POINT('Ctrl Pts',(-3.39538881861725,1.95068928167332,
-22.0133172667734)) ;
#137749=CARTESIAN_POINT('Ctrl Pts',(-3.44316973238529,1.87475949194142,
-22.0249970456942)) ;
#137750=CARTESIAN_POINT('Ctrl Pts',(-3.38343213690425,1.95,-21.9143774611971)) ;
#137751=CARTESIAN_POINT('Ctrl Pts',(-3.36046743872486,1.94345445676967,
-22.0047809294657)) ;
#137752=CARTESIAN_POINT('Ctrl Pts',(-3.38803897426451,1.85000000162387,
-22.0115206381536)) ;
#137753=CARTESIAN_POINT('Ctrl Pts',(-3.35509339356897,1.95,-21.9005229644555)) ;
#137754=CARTESIAN_POINT('Ctrl Pts',(-3.33134808452128,1.95,-21.9976628651052)) ;
#137755=CARTESIAN_POINT('Ctrl Pts',(-3.33134808452128,1.85,-21.9976628651052)) ;
#137756=CARTESIAN_POINT('Origin',(-3.50457525730571,1.91712723223402,-21.9370629755912)) ;
#137757=CARTESIAN_POINT('Origin',(-4.66204490261456,1.95,-18.42)) ;
#137758=CARTESIAN_POINT('Origin',(-4.66204490261456,-1.5692190524323,-18.42)) ;
#137759=CARTESIAN_POINT('Origin',(-3.84472135955,-1.16055728090002,-18.42)) ;
#137760=CARTESIAN_POINT('Origin',(-4.66204490261456,-1.5692190524323,-18.42)) ;
#137761=CARTESIAN_POINT('Origin',(-5.3,-2.11180339887499,-17.78)) ;
#137762=CARTESIAN_POINT('Origin',(-5.3,-2.11180339887499,-22.22)) ;
#137763=CARTESIAN_POINT('Origin',(-5.3,1.95,-22.42)) ;
#137764=CARTESIAN_POINT('Origin',(-5.3,-1.88819660112501,-22.42)) ;
#137765=CARTESIAN_POINT('Origin',(-4.0264650697994,2.50425327128942,-22.22)) ;
#137766=CARTESIAN_POINT('Origin',(-4.66204490261456,3.21928058320648,-22.22)) ;
#137767=CARTESIAN_POINT('Origin',(-3.02790825149799,1.38087685070033,-21.8205443741715)) ;
#137768=CARTESIAN_POINT('Origin',(-4.66204490261456,3.21928058320648,-22.22)) ;
#137769=CARTESIAN_POINT('Origin',(-4.66204490261456,-1.5692190524323,-18.42)) ;
#137770=CARTESIAN_POINT('Origin',(-4.66204490261456,-1.5692190524323,-18.42)) ;
#137771=CARTESIAN_POINT('Ctrl Pts',(-5.34460423617422,-2.02230212313483,
-22.2198752481299)) ;
#137772=CARTESIAN_POINT('Ctrl Pts',(-5.4,-2.0499093833863,-22.2198362457235)) ;
#137773=CARTESIAN_POINT('Ctrl Pts',(-5.4,-2.11180321723903,-22.2197503311196)) ;
#137774=CARTESIAN_POINT('Ctrl Pts',(-5.34461954754096,-2.02234798681675,
-22.2461538552817)) ;
#137775=CARTESIAN_POINT('Ctrl Pts',(-5.4,-2.04997459329993,-22.25432433516)) ;
#137776=CARTESIAN_POINT('Ctrl Pts',(-5.4,-2.11187974550671,-22.2723423130261)) ;
#137777=CARTESIAN_POINT('Ctrl Pts',(-5.33978950165955,-2.00789652656154,
-22.2721350349804)) ;
#137778=CARTESIAN_POINT('Ctrl Pts',(-5.4,-2.02908601268745,-22.2886334854683)) ;
#137779=CARTESIAN_POINT('Ctrl Pts',(-5.4,-2.087770056524,-22.3243387873639)) ;
#137780=CARTESIAN_POINT('Ctrl Pts',(-5.32318090226694,-1.9581752705225,
-22.3092155027319)) ;
#137781=CARTESIAN_POINT('Ctrl Pts',(-5.4,-1.96527310172481,-22.3278366162471)) ;
#137782=CARTESIAN_POINT('Ctrl Pts',(-5.4,-2.00485091174287,-22.3985039251107)) ;
#137783=CARTESIAN_POINT('Ctrl Pts',(-5.31153957531164,-1.92331224822995,
-22.3200135323111)) ;
#137784=CARTESIAN_POINT('Ctrl Pts',(-5.39999999999961,-1.9214867694528,
-22.3310221074624)) ;
#137785=CARTESIAN_POINT('Ctrl Pts',(-5.4,-1.94671708614656,-22.4200682869718)) ;
#137786=CARTESIAN_POINT('Ctrl Pts',(-5.29976814257746,-1.88802911972917,
-22.3200001726222)) ;
#137787=CARTESIAN_POINT('Ctrl Pts',(-5.4,-1.88802831720455,-22.319767406457)) ;
#137788=CARTESIAN_POINT('Ctrl Pts',(-5.4,-1.8879174628307,-22.4199998375376)) ;
#137789=CARTESIAN_POINT('Origin',(-5.30000000000006,-1.88819660112518,-22.2200000000001)) ;
#137790=CARTESIAN_POINT('Origin',(-4.66204490261456,3.21928058320648,-22.22)) ;
#137791=CARTESIAN_POINT('Origin',(-4.66204490261456,3.21928058320648,-22.22)) ;
#137792=CARTESIAN_POINT('Origin',(0.175392621986784,-0.95,-19.6024847282359)) ;
#137793=CARTESIAN_POINT('Origin',(-3.37639320225,-0.95,-18.7342704156447)) ;
#137794=CARTESIAN_POINT('Origin',(-3.32804538583365,-0.902219294041845,
-18.7460887707687)) ;
#137795=CARTESIAN_POINT('Origin',(-3.46583592134999,-0.971114561800017,
-18.7124066398647)) ;
#137796=CARTESIAN_POINT('Origin',(-3.24472135955,-0.860557280900019,-22.22)) ;
#137797=CARTESIAN_POINT('Origin',(-4.66204490261456,-1.5692190524323,-22.22)) ;
#137798=CARTESIAN_POINT('Origin',(-4.66204490261456,1.95,-22.22)) ;
#137799=CARTESIAN_POINT('Origin',(-4.66204490261456,-1.5692190524323,-22.22)) ;
#137800=CARTESIAN_POINT('Ctrl Pts',(-3.4211145618,-1.06055728090001,-18.7124066398647)) ;
#137801=CARTESIAN_POINT('Ctrl Pts',(-3.40394191641935,-1.05197095820969,
-18.6245919759864)) ;
#137802=CARTESIAN_POINT('Ctrl Pts',(-3.44209061230229,-0.971114561800017,
-18.615266739215)) ;
#137803=CARTESIAN_POINT('Ctrl Pts',(-3.40727897628737,-1.05363948814369,
-18.7191707039916)) ;
#137804=CARTESIAN_POINT('Ctrl Pts',(-3.38665319245551,-1.04670310838585,
-18.628818108511)) ;
#137805=CARTESIAN_POINT('Ctrl Pts',(-3.4144159452097,-0.957277229261615,
-18.6220316578376)) ;
#137806=CARTESIAN_POINT('Ctrl Pts',(-3.39186274464434,-1.05,-18.726707528252)) ;
#137807=CARTESIAN_POINT('Ctrl Pts',(-3.36870744055528,-1.04639008266723,
-18.6332048478644)) ;
#137808=CARTESIAN_POINT('Ctrl Pts',(-3.38358960366097,-0.950000000886305,
-18.6295669857718)) ;
#137809=CARTESIAN_POINT('Ctrl Pts',(-3.37639320225,-1.05,-18.7342704156447)) ;
#137810=CARTESIAN_POINT('Ctrl Pts',(-3.3526478932023,-1.05,-18.637130514995)) ;
#137811=CARTESIAN_POINT('Ctrl Pts',(-3.3526478932023,-0.95,-18.637130514995)) ;
#137812=CARTESIAN_POINT('Origin',(-3.37639320224972,-1.15000000000083,-18.7342704156448)) ;
#137813=CARTESIAN_POINT('Origin',(-4.66204490261456,-1.5692190524323,-22.22)) ;
#137814=CARTESIAN_POINT('Origin',(-4.66204490261456,-1.5692190524323,-22.22)) ;
#137815=CARTESIAN_POINT('Origin',(-3.37639320225,-1.15,-20.32)) ;
#137816=CARTESIAN_POINT('Origin',(-3.37639320224994,-1.14999999999955,-21.9057295843552)) ;
#137817=CARTESIAN_POINT('Origin',(-1.50751564693271,0.00804557540861825,
-21.4488928486111)) ;
#137818=CARTESIAN_POINT('Origin',(-3.46583592134999,-0.971114561800017,
-21.9275933601353)) ;
#137819=CARTESIAN_POINT('Ctrl Pts',(-3.37639320225,-1.05,-21.9057295843553)) ;
#137820=CARTESIAN_POINT('Ctrl Pts',(-3.3526478932023,-1.05,-22.002869485005)) ;
#137821=CARTESIAN_POINT('Ctrl Pts',(-3.3526478932023,-0.95,-22.002869485005)) ;
#137822=CARTESIAN_POINT('Ctrl Pts',(-3.39186274464434,-1.05,-21.913292471748)) ;
#137823=CARTESIAN_POINT('Ctrl Pts',(-3.36870744055537,-1.04639008266721,
-22.0067951521356)) ;
#137824=CARTESIAN_POINT('Ctrl Pts',(-3.38358960366096,-0.950000000886305,
-22.0104330142282)) ;
#137825=CARTESIAN_POINT('Ctrl Pts',(-3.40727897628737,-1.0536394881437,
-21.9208292960084)) ;
#137826=CARTESIAN_POINT('Ctrl Pts',(-3.3866531924554,-1.04670310838598,
-22.011181891489)) ;
#137827=CARTESIAN_POINT('Ctrl Pts',(-3.41441594520971,-0.95727722926162,
-22.0179683421624)) ;
#137828=CARTESIAN_POINT('Ctrl Pts',(-3.4211145618,-1.06055728090001,-21.9275933601353)) ;
#137829=CARTESIAN_POINT('Ctrl Pts',(-3.40394191641936,-1.05197095820968,
-22.0154080240136)) ;
#137830=CARTESIAN_POINT('Ctrl Pts',(-3.44209061230229,-0.971114561800017,
-22.024733260785)) ;
#137831=CARTESIAN_POINT('Origin',(-3.37639320225,-0.95,-21.9057295843553)) ;
#137832=CARTESIAN_POINT('Origin',(0.175392621986784,-0.95,-21.0375152717641)) ;
#137833=CARTESIAN_POINT('Origin',(12.7,2.65,-17.78)) ;
#137834=CARTESIAN_POINT('Origin',(12.8,2.65,-21.8130460421716)) ;
#137835=CARTESIAN_POINT('',(4.57524318173533,2.73534903669982,-21.7609351802097)) ;
#137836=CARTESIAN_POINT('Origin',(4.65232986201019,2.66527023614907,-21.8087542111864)) ;
#137837=CARTESIAN_POINT('Ctrl Pts',(4.57524318173533,2.73534903669982,-21.7609351802097)) ;
#137838=CARTESIAN_POINT('Ctrl Pts',(4.5761458558036,2.73452842391049,-21.7595911511832)) ;
#137839=CARTESIAN_POINT('Ctrl Pts',(4.57705238626145,2.73367683201793,-21.7582681293393)) ;
#137840=CARTESIAN_POINT('Ctrl Pts',(4.5779495181309,2.73280244902548,-21.7569768488888)) ;
#137841=CARTESIAN_POINT('Ctrl Pts',(4.58144263576929,2.72939790755547,-21.7519490545686)) ;
#137842=CARTESIAN_POINT('Ctrl Pts',(4.58496694799971,2.72549786515197,-21.7471699445181)) ;
#137843=CARTESIAN_POINT('Ctrl Pts',(4.58815670056887,2.72107165565075,-21.742698193853)) ;
#137844=CARTESIAN_POINT('Ctrl Pts',(4.59069123847463,2.71755464437276,-21.7391449961299)) ;
#137845=CARTESIAN_POINT('Ctrl Pts',(4.59301454561849,2.71370459823918,-21.7357863127243)) ;
#137846=CARTESIAN_POINT('Ctrl Pts',(4.5949431309995,2.70950205848694,-21.7326749961674)) ;
#137847=CARTESIAN_POINT('Ctrl Pts',(4.59651854606295,2.70606910472943,-21.7301334364214)) ;
#137848=CARTESIAN_POINT('Ctrl Pts',(4.59783685868322,2.70233705077422,-21.7277160861571)) ;
#137849=CARTESIAN_POINT('Ctrl Pts',(4.59873118971424,2.69838744819993,-21.7255323012123)) ;
#137850=CARTESIAN_POINT('Ctrl Pts',(4.59916508318198,2.69647125978905,-21.7244728165364)) ;
#137851=CARTESIAN_POINT('Ctrl Pts',(4.59949917984823,2.69450444432188,-21.723467798882)) ;
#137852=CARTESIAN_POINT('Ctrl Pts',(4.5997144226265,2.692499226592,-21.7225263440994)) ;
#137853=CARTESIAN_POINT('Ctrl Pts',(4.59990113259977,2.69075982259552,-21.7217096895352)) ;
#137854=CARTESIAN_POINT('Ctrl Pts',(4.6,2.68896788689974,-21.7209303122145)) ;
#137855=CARTESIAN_POINT('Ctrl Pts',(4.6,2.68715716172261,-21.7202056127633)) ;
#137856=CARTESIAN_POINT('Origin',(4.5,2.1,-21.7019539578284)) ;
#137857=CARTESIAN_POINT('Origin',(4.6,2.1,-21.7019539578284)) ;
#137858=CARTESIAN_POINT('Origin',(12.7,2.1,-21.7019539578284)) ;
#137859=CARTESIAN_POINT('Origin',(12.7,2.76643989873054,-21.7936393923832)) ;
#137860=CARTESIAN_POINT('Origin',(12.7,2.13287979746107,-21.8992327425948)) ;
#137861=CARTESIAN_POINT('Origin',(4.4,2.72431432344521,-20.32)) ;
#137862=CARTESIAN_POINT('Ctrl Pts',(4.48762159086959,2.77250619842349,-18.9311756817495)) ;
#137863=CARTESIAN_POINT('Ctrl Pts',(4.48806820038223,2.77169418112776,-18.9338355670898)) ;
#137864=CARTESIAN_POINT('Ctrl Pts',(4.48852084821546,2.77084293101113,-18.9364827150185)) ;
#137865=CARTESIAN_POINT('Ctrl Pts',(4.49012932137854,2.76769877392856,-18.9457630095207)) ;
#137866=CARTESIAN_POINT('Ctrl Pts',(4.49131046584974,2.76517764467229,-18.9523441317034)) ;
#137867=CARTESIAN_POINT('Ctrl Pts',(4.49351977821776,2.75978760391035,-18.964635280162)) ;
#137868=CARTESIAN_POINT('Ctrl Pts',(4.49455195297826,2.75697653750129,-18.9703677406012)) ;
#137869=CARTESIAN_POINT('Ctrl Pts',(4.49620670090465,2.75163165728877,-18.9799433216032)) ;
#137870=CARTESIAN_POINT('Ctrl Pts',(4.49686252944492,2.74924176842725,-18.9838640262033)) ;
#137871=CARTESIAN_POINT('Ctrl Pts',(4.49822764032847,2.74331716058964,-18.9926446316345)) ;
#137872=CARTESIAN_POINT('Ctrl Pts',(4.498902033579,2.73961076902736,-18.9974865001601)) ;
#137873=CARTESIAN_POINT('Ctrl Pts',(4.4997589785602,2.73206576252715,-19.0058277784394)) ;
#137874=CARTESIAN_POINT('Ctrl Pts',(4.5,2.72833175948635,-19.0094190022917)) ;
#137875=CARTESIAN_POINT('Ctrl Pts',(4.5,2.72431432344521,-19.012634816645)) ;
#137876=CARTESIAN_POINT('Ctrl Pts',(4.5,2.72431432344521,-21.627365183355)) ;
#137877=CARTESIAN_POINT('Ctrl Pts',(4.5,2.72904669151417,-21.6311532753136)) ;
#137878=CARTESIAN_POINT('Ctrl Pts',(4.49966645684475,2.73338556955535,-21.6354614101758)) ;
#137879=CARTESIAN_POINT('Ctrl Pts',(4.49869539480396,2.74072289096357,-21.6439802414372)) ;
#137880=CARTESIAN_POINT('Ctrl Pts',(4.49811062025689,2.74382502998075,-21.6481080596585)) ;
#137881=CARTESIAN_POINT('Ctrl Pts',(4.49664125196625,2.75020211699685,-21.6575592649405)) ;
#137882=CARTESIAN_POINT('Ctrl Pts',(4.49570721389712,2.75339870015137,-21.6630103903193)) ;
#137883=CARTESIAN_POINT('Ctrl Pts',(4.49363760641479,2.75952863263943,-21.6747517051868)) ;
#137884=CARTESIAN_POINT('Ctrl Pts',(4.49249077386344,2.76240287369067,-21.6810712258307)) ;
#137885=CARTESIAN_POINT('Ctrl Pts',(4.49055019898874,2.76677757270135,-21.6919141256208)) ;
#137886=CARTESIAN_POINT('Ctrl Pts',(4.48975662823144,2.76842729450632,-21.6963872919226)) ;
#137887=CARTESIAN_POINT('Ctrl Pts',(4.4885208482156,2.77084293101086,-21.7035172849807)) ;
#137888=CARTESIAN_POINT('Ctrl Pts',(4.48806820038251,2.77169418112725,-21.7061644329085)) ;
#137889=CARTESIAN_POINT('Ctrl Pts',(4.48762159086959,2.77250619842348,-21.7088243182478)) ;
#137890=CARTESIAN_POINT('Origin',(4.6,2.1,-20.32)) ;
#137891=CARTESIAN_POINT('Origin',(4.6,2.1,-18.9380460421716)) ;
#137892=CARTESIAN_POINT('Origin',(4.6,2.1,-21.7019539578284)) ;
#137893=CARTESIAN_POINT('Origin',(12.7,2.1,-21.7019539578284)) ;
#137894=CARTESIAN_POINT('Origin',(12.7,1.9,-21.7019539578284)) ;
#137895=CARTESIAN_POINT('Origin',(12.7,2.65,-17.78)) ;
#137896=CARTESIAN_POINT('Origin',(4.5,2.65,-18.8269539578284)) ;
#137897=CARTESIAN_POINT('',(4.6,2.68715716172261,-18.9197943872367)) ;
#137898=CARTESIAN_POINT('',(4.57524318173443,2.73534903670064,-18.8790648197889)) ;
#137899=CARTESIAN_POINT('Ctrl Pts',(4.6,2.68715716172262,-18.9197943872367)) ;
#137900=CARTESIAN_POINT('Ctrl Pts',(4.6,2.6910603667141,-18.9182322227785)) ;
#137901=CARTESIAN_POINT('Ctrl Pts',(4.59952510519174,2.6948886188898,-18.9164097094748)) ;
#137902=CARTESIAN_POINT('Ctrl Pts',(4.59869497748257,2.69852743640759,-18.9143901512251)) ;
#137903=CARTESIAN_POINT('Ctrl Pts',(4.59815316003467,2.70090246232122,-18.9130720023612)) ;
#137904=CARTESIAN_POINT('Ctrl Pts',(4.5974600110878,2.70319720658043,-18.9116709680453)) ;
#137905=CARTESIAN_POINT('Ctrl Pts',(4.59664880273703,2.70538659711789,-18.9102145418985)) ;
#137906=CARTESIAN_POINT('Ctrl Pts',(4.59612777291939,2.70679281754375,-18.9092790960924)) ;
#137907=CARTESIAN_POINT('Ctrl Pts',(4.59555051815356,2.70817855133089,-18.9083049299072)) ;
#137908=CARTESIAN_POINT('Ctrl Pts',(4.59494172533681,2.70950512149371,-18.9073227360698)) ;
#137909=CARTESIAN_POINT('Ctrl Pts',(4.59250947890868,2.71480502887002,-18.9033986794992)) ;
#137910=CARTESIAN_POINT('Ctrl Pts',(4.58944857813008,2.71954517005227,-18.8990823375811)) ;
#137911=CARTESIAN_POINT('Ctrl Pts',(4.5861276864684,2.72376361218885,-18.8944738031841)) ;
#137912=CARTESIAN_POINT('Ctrl Pts',(4.58350334758193,2.72709724148698,-18.8908319029778)) ;
#137913=CARTESIAN_POINT('Ctrl Pts',(4.58071664514671,2.73010548898765,-18.8870059959317)) ;
#137914=CARTESIAN_POINT('Ctrl Pts',(4.5779495181309,2.73280244902546,-18.8830231511112)) ;
#137915=CARTESIAN_POINT('Ctrl Pts',(4.57705238626115,2.7336768320182,-18.8817318706603)) ;
#137916=CARTESIAN_POINT('Ctrl Pts',(4.57614585580299,2.73452842391107,-18.8804088488159)) ;
#137917=CARTESIAN_POINT('Ctrl Pts',(4.57524318173444,2.73534903670067,-18.8790648197889)) ;
#137918=CARTESIAN_POINT('Origin',(4.65232986199444,2.66527023616352,-18.8312457888174)) ;
#137919=CARTESIAN_POINT('Origin',(4.6,2.65,-18.8269539578284)) ;
#137920=CARTESIAN_POINT('Origin',(12.7,1.9,-21.82)) ;
#137921=CARTESIAN_POINT('Origin',(12.7,2.01643989873054,-18.7213606076168)) ;
#137922=CARTESIAN_POINT('Origin',(-3.65,10.7,-19.57)) ;
#137923=CARTESIAN_POINT('Origin',(-3.65,10.7,-19.57)) ;
#137924=CARTESIAN_POINT('Origin',(-3.65,10.7,-19.57)) ;
#137925=CARTESIAN_POINT('Origin',(0.,10.7,-19.57)) ;
#137926=CARTESIAN_POINT('Origin',(-2.9,10.7,-19.57)) ;
#137927=CARTESIAN_POINT('Origin',(-3.65,10.7,-20.32)) ;
#137928=CARTESIAN_POINT('Origin',(-3.65,10.7,-21.07)) ;
#137929=CARTESIAN_POINT('Origin',(-2.9,10.7,-19.57)) ;
#137930=CARTESIAN_POINT('Origin',(-2.9,10.7,-19.57)) ;
#137931=CARTESIAN_POINT('Origin',(-3.65,10.7,-21.07)) ;
#137932=CARTESIAN_POINT('Origin',(-3.65,10.7,-21.07)) ;
#137933=CARTESIAN_POINT('Origin',(-2.9,10.7,-20.32)) ;
#137934=CARTESIAN_POINT('Origin',(-2.9,10.7,-21.07)) ;
#137935=CARTESIAN_POINT('Origin',(0.,10.7,-21.07)) ;
#137936=CARTESIAN_POINT('Origin',(-2.9,10.7,-21.07)) ;
#137937=CARTESIAN_POINT('Origin',(-2.9,10.7,-21.07)) ;
#137938=CARTESIAN_POINT('Origin',(-3.05,-3.95,-19.32)) ;
#137939=CARTESIAN_POINT('Origin',(-3.05,-3.95,-21.22)) ;
#137940=CARTESIAN_POINT('Origin',(-3.05,-3.95,-19.42)) ;
#137941=CARTESIAN_POINT('Origin',(-3.25,-3.95,-19.42)) ;
#137942=CARTESIAN_POINT('Origin',(-3.25,-3.95,-19.22)) ;
#137943=CARTESIAN_POINT('Origin',(-3.25,-3.95,-19.42)) ;
#137944=CARTESIAN_POINT('Origin',(-3.25,-3.95,-21.22)) ;
#137945=CARTESIAN_POINT('Origin',(-3.25,-3.95,-21.22)) ;
#137946=CARTESIAN_POINT('Origin',(-3.25,-3.95,-21.42)) ;
#137947=CARTESIAN_POINT('Origin',(-4.4,-3.95,-19.22)) ;
#137948=CARTESIAN_POINT('Origin',(-4.3,-3.95,-19.22)) ;
#137949=CARTESIAN_POINT('Origin',(-3.25,-3.9,-19.42)) ;
#137950=CARTESIAN_POINT('Origin',(-3.25,-3.85,-19.42)) ;
#137951=CARTESIAN_POINT('Origin',(-3.25,-3.85,-20.32)) ;
#137952=CARTESIAN_POINT('Origin',(-3.25,-3.85,-21.22)) ;
#137953=CARTESIAN_POINT('Origin',(-3.25,-3.85,-19.42)) ;
#137954=CARTESIAN_POINT('Origin',(-3.25,-3.9,-21.22)) ;
#137955=CARTESIAN_POINT('Origin',(-3.25,-3.85,-21.22)) ;
#137956=CARTESIAN_POINT('Origin',(-4.4,-3.95,-21.42)) ;
#137957=CARTESIAN_POINT('Origin',(-4.3,-3.95,-21.42)) ;
#137958=CARTESIAN_POINT('Origin',(-4.5,-3.95,-19.32)) ;
#137959=CARTESIAN_POINT('Origin',(-4.5,-3.95,-19.42)) ;
#137960=CARTESIAN_POINT('Origin',(-4.5,-3.95,-21.22)) ;
#137961=CARTESIAN_POINT('Origin',(-4.3,-3.95,-19.42)) ;
#137962=CARTESIAN_POINT('Origin',(-4.3,-3.95,-19.42)) ;
#137963=CARTESIAN_POINT('Origin',(-3.25,-3.85,-19.42)) ;
#137964=CARTESIAN_POINT('Origin',(-3.25,-3.85,-19.42)) ;
#137965=CARTESIAN_POINT('Origin',(-3.25,-3.85,-21.22)) ;
#137966=CARTESIAN_POINT('Origin',(-3.25,-3.85,-21.22)) ;
#137967=CARTESIAN_POINT('Origin',(-4.3,-3.95,-21.22)) ;
#137968=CARTESIAN_POINT('Origin',(-4.3,-3.95,-21.22)) ;
#137969=CARTESIAN_POINT('Origin',(-4.3,-3.9,-19.42)) ;
#137970=CARTESIAN_POINT('Origin',(-4.3,-3.85,-19.42)) ;
#137971=CARTESIAN_POINT('Origin',(-1.56125112837913E-16,-3.85,-19.42)) ;
#137972=CARTESIAN_POINT('Origin',(-4.3,-3.85,-19.42)) ;
#137973=CARTESIAN_POINT('Origin',(-1.56125112837913E-16,-3.85,-21.22)) ;
#137974=CARTESIAN_POINT('Origin',(-4.3,-3.85,-21.22)) ;
#137975=CARTESIAN_POINT('Origin',(-4.3,-3.9,-21.22)) ;
#137976=CARTESIAN_POINT('Origin',(-4.3,-3.85,-21.22)) ;
#137977=CARTESIAN_POINT('Origin',(-4.3,-3.85,-19.42)) ;
#137978=CARTESIAN_POINT('Origin',(-4.3,-3.85,-19.42)) ;
#137979=CARTESIAN_POINT('Origin',(-4.3,-3.85,-21.22)) ;
#137980=CARTESIAN_POINT('Origin',(-4.3,-3.85,-21.22)) ;
#137981=CARTESIAN_POINT('Origin',(-4.3,-3.85,-20.32)) ;
#137982=CARTESIAN_POINT('Origin',(-4.,10.85,-21.32)) ;
#137983=CARTESIAN_POINT('Origin',(-4.,10.85,-21.22)) ;
#137984=CARTESIAN_POINT('Origin',(-4.,10.85,-19.42)) ;
#137985=CARTESIAN_POINT('Origin',(-3.8,10.85,-19.42)) ;
#137986=CARTESIAN_POINT('Origin',(-3.8,10.85,-19.22)) ;
#137987=CARTESIAN_POINT('Origin',(-3.8,10.85,-19.42)) ;
#137988=CARTESIAN_POINT('Origin',(-3.8,10.85,-21.22)) ;
#137989=CARTESIAN_POINT('Origin',(-3.8,10.85,-21.22)) ;
#137990=CARTESIAN_POINT('Origin',(-3.8,10.85,-21.42)) ;
#137991=CARTESIAN_POINT('Origin',(-3.9,10.85,-19.22)) ;
#137992=CARTESIAN_POINT('Origin',(-2.75,10.85,-19.22)) ;
#137993=CARTESIAN_POINT('Origin',(-3.8,10.8,-19.42)) ;
#137994=CARTESIAN_POINT('Origin',(-3.8,10.75,-19.42)) ;
#137995=CARTESIAN_POINT('Origin',(-3.8,10.75,-20.32)) ;
#137996=CARTESIAN_POINT('Origin',(-3.8,10.75,-21.22)) ;
#137997=CARTESIAN_POINT('Origin',(-3.8,10.75,-19.42)) ;
#137998=CARTESIAN_POINT('Origin',(-3.8,10.8,-21.22)) ;
#137999=CARTESIAN_POINT('Origin',(-3.8,10.75,-21.22)) ;
#138000=CARTESIAN_POINT('Origin',(-3.9,10.85,-21.42)) ;
#138001=CARTESIAN_POINT('Origin',(-2.75,10.85,-21.42)) ;
#138002=CARTESIAN_POINT('Origin',(-2.55,10.85,-21.32)) ;
#138003=CARTESIAN_POINT('Origin',(-2.55,10.85,-19.42)) ;
#138004=CARTESIAN_POINT('Origin',(-2.55,10.85,-21.22)) ;
#138005=CARTESIAN_POINT('Origin',(-2.75,10.85,-19.42)) ;
#138006=CARTESIAN_POINT('Origin',(-2.75,10.85,-19.42)) ;
#138007=CARTESIAN_POINT('Origin',(-3.8,10.75,-19.42)) ;
#138008=CARTESIAN_POINT('Origin',(-3.8,10.75,-19.42)) ;
#138009=CARTESIAN_POINT('Origin',(-3.8,10.75,-21.22)) ;
#138010=CARTESIAN_POINT('Origin',(-3.8,10.75,-21.22)) ;
#138011=CARTESIAN_POINT('Origin',(-2.75,10.85,-21.22)) ;
#138012=CARTESIAN_POINT('Origin',(-2.75,10.85,-21.22)) ;
#138013=CARTESIAN_POINT('Origin',(-2.75,10.8,-19.42)) ;
#138014=CARTESIAN_POINT('Origin',(-2.75,10.75,-19.42)) ;
#138015=CARTESIAN_POINT('Origin',(1.56125112837912E-16,10.75,-19.42)) ;
#138016=CARTESIAN_POINT('Origin',(-2.75,10.75,-19.42)) ;
#138017=CARTESIAN_POINT('Origin',(-1.56125112837913E-16,10.75,-21.22)) ;
#138018=CARTESIAN_POINT('Origin',(-2.75,10.75,-21.22)) ;
#138019=CARTESIAN_POINT('Origin',(-2.75,10.8,-21.22)) ;
#138020=CARTESIAN_POINT('Origin',(-2.75,10.75,-21.22)) ;
#138021=CARTESIAN_POINT('Origin',(-2.75,10.75,-19.42)) ;
#138022=CARTESIAN_POINT('Origin',(-2.75,10.75,-19.42)) ;
#138023=CARTESIAN_POINT('Origin',(-2.75,10.75,-21.22)) ;
#138024=CARTESIAN_POINT('Origin',(-2.75,10.75,-21.22)) ;
#138025=CARTESIAN_POINT('Origin',(-2.75,10.75,-20.32)) ;
#138026=CARTESIAN_POINT('Origin',(4.6,0.,-20.32)) ;
#138027=CARTESIAN_POINT('Ctrl Pts',(4.5,-2.7,-18.7968453788272)) ;
#138028=CARTESIAN_POINT('Ctrl Pts',(4.5,-2.71827986285823,-18.8719647391751)) ;
#138029=CARTESIAN_POINT('Ctrl Pts',(4.50597963419107,-2.73556801027185,
-18.9467398604528)) ;
#138030=CARTESIAN_POINT('Ctrl Pts',(4.52394923367545,-2.75977758633329,
-19.0584368340216)) ;
#138031=CARTESIAN_POINT('Ctrl Pts',(4.53141024883993,-2.76757607569523,
-19.0956832823903)) ;
#138032=CARTESIAN_POINT('Ctrl Pts',(4.54734065524867,-2.77857284247615,
-19.150165689583)) ;
#138033=CARTESIAN_POINT('Ctrl Pts',(4.55339248498576,-2.78214991573955,
-19.1682382744149)) ;
#138034=CARTESIAN_POINT('Ctrl Pts',(4.56567492147096,-2.787183259287,-19.1941467218607)) ;
#138035=CARTESIAN_POINT('Ctrl Pts',(4.5702469143305,-2.78880341224557,-19.2025726050508)) ;
#138036=CARTESIAN_POINT('Ctrl Pts',(4.58215938980081,-2.79169669265294,
-19.2177434798851)) ;
#138037=CARTESIAN_POINT('Ctrl Pts',(4.59005470866978,-2.79310344827587,
-19.2252063540423)) ;
#138038=CARTESIAN_POINT('Ctrl Pts',(4.6,-2.79310344827586,-19.2252063540422)) ;
#138039=CARTESIAN_POINT('Origin',(4.6,-2.4,-18.3578583129651)) ;
#138040=CARTESIAN_POINT('Origin',(4.6,-2.4,-17.78)) ;
#138041=CARTESIAN_POINT('Origin',(4.6,-2.4,-17.2021416870349)) ;
#138042=CARTESIAN_POINT('Origin',(4.6,-2.4,-18.3578583129651)) ;
#138043=CARTESIAN_POINT('Origin',(4.6,-2.4,-18.3578583129651)) ;
#138044=CARTESIAN_POINT('Origin',(4.6,-2.4,-18.3578583129651)) ;
#138045=CARTESIAN_POINT('Origin',(0.584645609909622,-2.4,-18.3578583129651)) ;
#138046=CARTESIAN_POINT('Origin',(12.7,-2.4,-18.3578583129651)) ;
#138047=CARTESIAN_POINT('Origin',(12.7,-2.2,-17.78)) ;
#138048=CARTESIAN_POINT('Origin',(12.7,-2.2,-17.2021416870349)) ;
#138049=CARTESIAN_POINT('Origin',(12.7,-2.2,-18.3578583129651)) ;
#138050=CARTESIAN_POINT('Origin',(12.7,-2.4,-18.3578583129651)) ;
#138051=CARTESIAN_POINT('Origin',(12.7,-2.24516129032258,-18.4844480992255)) ;
#138052=CARTESIAN_POINT('Origin',(12.7,0.,-20.32)) ;
#138053=CARTESIAN_POINT('Origin',(12.7,-2.24516129032258,-22.1555519007745)) ;
#138054=CARTESIAN_POINT('Origin',(12.7,-2.2,-17.78)) ;
#138055=CARTESIAN_POINT('Origin',(12.7,-2.2,-22.2821416870349)) ;
#138056=CARTESIAN_POINT('Origin',(12.7,-2.4,-22.2821416870349)) ;
#138057=CARTESIAN_POINT('Origin',(12.7,-2.4,-22.2821416870349)) ;
#138058=CARTESIAN_POINT('Origin',(0.584645609909622,-2.4,-22.2821416870349)) ;
#138059=CARTESIAN_POINT('Origin',(4.6,-2.4,-22.2821416870349)) ;
#138060=CARTESIAN_POINT('Origin',(4.6,-2.4,-17.78)) ;
#138061=CARTESIAN_POINT('Origin',(4.6,-2.4,-22.2821416870349)) ;
#138062=CARTESIAN_POINT('Origin',(4.6,-2.4,-22.2821416870349)) ;
#138063=CARTESIAN_POINT('Origin',(4.6,-2.4,-22.2821416870349)) ;
#138064=CARTESIAN_POINT('Origin',(4.6,0.,-20.32)) ;
#138065=CARTESIAN_POINT('Ctrl Pts',(4.6,-2.79310344827586,-21.4147936459578)) ;
#138066=CARTESIAN_POINT('Ctrl Pts',(4.59007568892311,-2.79310344827586,
-21.4147936459578)) ;
#138067=CARTESIAN_POINT('Ctrl Pts',(4.58219207637239,-2.79170232102183,
-21.422226742276)) ;
#138068=CARTESIAN_POINT('Ctrl Pts',(4.57028631514659,-2.78881527838255,
-21.43736543899)) ;
#138069=CARTESIAN_POINT('Ctrl Pts',(4.56571532154372,-2.78719767797524,
-21.4457784885835)) ;
#138070=CARTESIAN_POINT('Ctrl Pts',(4.55343865632726,-2.78217307830036,
-21.4716436333089)) ;
#138071=CARTESIAN_POINT('Ctrl Pts',(4.54738888873344,-2.77860151743012,
-21.4896900859661)) ;
#138072=CARTESIAN_POINT('Ctrl Pts',(4.53146440752602,-2.76762263748299,
-21.5440903156831)) ;
#138073=CARTESIAN_POINT('Ctrl Pts',(4.52400917967609,-2.75984503873828,
-21.5812455063058)) ;
#138074=CARTESIAN_POINT('Ctrl Pts',(4.50599905604505,-2.7356206423885,-21.6930301354693)) ;
#138075=CARTESIAN_POINT('Ctrl Pts',(4.5,-2.71826422026483,-21.7680995425769)) ;
#138076=CARTESIAN_POINT('Ctrl Pts',(4.5,-2.7,-21.8431546211728)) ;
#138077=CARTESIAN_POINT('Origin',(3.7,-2.9,-17.78)) ;
#138078=CARTESIAN_POINT('Origin',(3.7,-2.9,-12.7)) ;
#138079=CARTESIAN_POINT('Origin',(3.5,-3.95,-17.78)) ;
#138080=CARTESIAN_POINT('Origin',(3.5,-3.95,-12.7)) ;
#138081=CARTESIAN_POINT('Origin',(-5.3,-3.95,-17.78)) ;
#138082=CARTESIAN_POINT('Origin',(-5.3,-3.95,-12.7)) ;
#138083=CARTESIAN_POINT('Origin',(-5.3,5.19009804864072,-17.78)) ;
#138084=CARTESIAN_POINT('Origin',(-5.3,5.19009804864072,-12.7)) ;
#138085=CARTESIAN_POINT('Origin',(-4.8,10.3,-17.78)) ;
#138086=CARTESIAN_POINT('Origin',(-4.8,10.3,-12.7)) ;
#138087=CARTESIAN_POINT('Origin',(-4.8,10.85,-17.78)) ;
#138088=CARTESIAN_POINT('Origin',(-4.8,10.85,-12.7)) ;
#138089=CARTESIAN_POINT('Origin',(-0.362523114814661,9.05,-20.4890473046963)) ;
#138090=CARTESIAN_POINT('Origin',(0.36252311481466,9.05,-20.1509526953037)) ;
#138091=CARTESIAN_POINT('Origin',(-1.31845674202095,9.85,-18.9122813422351)) ;
#138092=CARTESIAN_POINT('Origin',(-0.230887397576972,9.85,-18.4051394281462)) ;
#138093=CARTESIAN_POINT('Origin',(3.3,10.85,-17.78)) ;
#138094=CARTESIAN_POINT('Origin',(3.3,10.85,-12.7)) ;
#138095=CARTESIAN_POINT('Origin',(3.85,6.92431432344521,-17.78)) ;
#138096=CARTESIAN_POINT('Origin',(3.85,6.92431432344521,-12.7)) ;
#138097=CARTESIAN_POINT('Origin',(4.05,3.77568567655479,-17.78)) ;
#138098=CARTESIAN_POINT('Origin',(4.05,3.77568567655479,-12.7)) ;
#138099=CARTESIAN_POINT('Origin',(4.6,2.1,-18.9380460421716)) ;
#138100=CARTESIAN_POINT('Origin',(4.6,2.1,-18.9380460421716)) ;
#138101=CARTESIAN_POINT('Origin',(4.6,0.280857398566761,-18.6348556085994)) ;
#138102=CARTESIAN_POINT('Origin',(4.6,2.61712020253893,-19.0242327425948)) ;
#138103=CARTESIAN_POINT('Origin',(4.6,2.65,-18.8269539578284)) ;
#138104=CARTESIAN_POINT('Origin',(4.6,2.72431432344521,-19.012634816645)) ;
#138105=CARTESIAN_POINT('Ctrl Pts',(4.48762159086906,2.77250619842445,-18.9311756817496)) ;
#138106=CARTESIAN_POINT('Ctrl Pts',(4.51316716229104,2.72605970493114,-18.8942387941972)) ;
#138107=CARTESIAN_POINT('Ctrl Pts',(4.57527453405851,2.73535372386122,-18.879057153198)) ;
#138108=CARTESIAN_POINT('Ctrl Pts',(4.49363662433155,2.76156977394747,-18.9669995924716)) ;
#138109=CARTESIAN_POINT('Ctrl Pts',(4.5146945995807,2.70766535161861,-18.9162008473932)) ;
#138110=CARTESIAN_POINT('Ctrl Pts',(4.58732693581885,2.72440392220678,-18.8969950412341)) ;
#138111=CARTESIAN_POINT('Ctrl Pts',(4.5,2.74488438438033,-18.9961692160663)) ;
#138112=CARTESIAN_POINT('Ctrl Pts',(4.50856472873626,2.69031482079677,-18.9184911137048)) ;
#138113=CARTESIAN_POINT('Ctrl Pts',(4.60003980620507,2.70775073269831,-18.9115523113747)) ;
#138114=CARTESIAN_POINT('Ctrl Pts',(4.5,2.72431432344521,-19.012634816645)) ;
#138115=CARTESIAN_POINT('Ctrl Pts',(4.5,2.68714136424467,-18.9197549158517)) ;
#138116=CARTESIAN_POINT('Ctrl Pts',(4.60004250625998,2.68715716507935,-18.9197943956238)) ;
#138117=CARTESIAN_POINT('Origin',(4.57524318173443,2.82069807340128,-18.9311756817495)) ;
#138118=CARTESIAN_POINT('Ctrl Pts',(4.47150553123747,2.80180812502279,-18.8269539578284)) ;
#138119=CARTESIAN_POINT('Ctrl Pts',(4.5,2.75,-18.8269539578284)) ;
#138120=CARTESIAN_POINT('Ctrl Pts',(4.55912712210514,2.75,-18.8269539578284)) ;
#138121=CARTESIAN_POINT('Ctrl Pts',(4.47150553186688,2.8018081238784,-18.8635744727347)) ;
#138122=CARTESIAN_POINT('Ctrl Pts',(4.50000000073523,2.74999999866316,-18.8512580842688)) ;
#138123=CARTESIAN_POINT('Ctrl Pts',(4.5591271227348,2.75,-18.8452720457593)) ;
#138124=CARTESIAN_POINT('Ctrl Pts',(4.47712448971608,2.79159183687986,-18.8999165373524)) ;
#138125=CARTESIAN_POINT('Ctrl Pts',(4.50480340096849,2.74126654369362,-18.8755379509981)) ;
#138126=CARTESIAN_POINT('Ctrl Pts',(4.56473907811156,2.74489822224644,-18.8634248215823)) ;
#138127=CARTESIAN_POINT('Ctrl Pts',(4.48762159086676,2.77250619842407,-18.9311756817495)) ;
#138128=CARTESIAN_POINT('Ctrl Pts',(4.51315802400618,2.72607631998876,-18.8942520074343)) ;
#138129=CARTESIAN_POINT('Ctrl Pts',(4.57524318173443,2.73534903670064,-18.8790648197889)) ;
#138130=CARTESIAN_POINT('Origin',(4.55912712210513,2.85,-18.8269539578284)) ;
#138131=CARTESIAN_POINT('Origin',(4.55912712210514,2.85,-17.78)) ;
#138132=CARTESIAN_POINT('Origin',(4.55912712210514,2.85,-16.7330460421716)) ;
#138133=CARTESIAN_POINT('Origin',(4.55912712210514,2.85,-17.78)) ;
#138134=CARTESIAN_POINT('Origin',(4.55912712210514,2.85,-21.8130460421716)) ;
#138135=CARTESIAN_POINT('Ctrl Pts',(4.48762159086766,2.77250619842243,-21.7088243182478)) ;
#138136=CARTESIAN_POINT('Ctrl Pts',(4.51315802400691,2.72607631998744,-21.7457479925641)) ;
#138137=CARTESIAN_POINT('Ctrl Pts',(4.57524318173533,2.73534903669982,-21.7609351802097)) ;
#138138=CARTESIAN_POINT('Ctrl Pts',(4.47712448971643,2.79159183687922,-21.7400834626457)) ;
#138139=CARTESIAN_POINT('Ctrl Pts',(4.50480340096883,2.74126654369304,-21.7644620490007)) ;
#138140=CARTESIAN_POINT('Ctrl Pts',(4.56473907811197,2.74489822224618,-21.7765751784167)) ;
#138141=CARTESIAN_POINT('Ctrl Pts',(4.47150553186688,2.8018081238784,-21.7764255272642)) ;
#138142=CARTESIAN_POINT('Ctrl Pts',(4.50000000073523,2.74999999866316,-21.7887419157304)) ;
#138143=CARTESIAN_POINT('Ctrl Pts',(4.5591271227348,2.75,-21.7947279542402)) ;
#138144=CARTESIAN_POINT('Ctrl Pts',(4.47150553123747,2.80180812502279,-21.8130460421716)) ;
#138145=CARTESIAN_POINT('Ctrl Pts',(4.5,2.75,-21.8130460421716)) ;
#138146=CARTESIAN_POINT('Ctrl Pts',(4.55912712210513,2.75,-21.8130460421716)) ;
#138147=CARTESIAN_POINT('Origin',(4.57524318173533,2.82069807339964,-21.7088243182478)) ;
#138148=CARTESIAN_POINT('Ctrl Pts',(4.57527448145479,2.73535371598842,-21.7609428339419)) ;
#138149=CARTESIAN_POINT('Ctrl Pts',(4.51316714695683,2.7260597328105,-21.7457611836292)) ;
#138150=CARTESIAN_POINT('Ctrl Pts',(4.48762159086951,2.77250619842363,-21.7088243182477)) ;
#138151=CARTESIAN_POINT('Ctrl Pts',(4.5873268774263,2.72440390874888,-21.7430049433246)) ;
#138152=CARTESIAN_POINT('Ctrl Pts',(4.51469458626373,2.70766538570662,-21.7237991204817)) ;
#138153=CARTESIAN_POINT('Ctrl Pts',(4.49363662433185,2.76156977394669,-21.6730004075269)) ;
#138154=CARTESIAN_POINT('Ctrl Pts',(4.60003973844309,2.70775071978185,-21.728447683485)) ;
#138155=CARTESIAN_POINT('Ctrl Pts',(4.50856472285784,2.6903148582481,-21.721508832984)) ;
#138156=CARTESIAN_POINT('Ctrl Pts',(4.5,2.74488438437978,-21.6438307839333)) ;
#138157=CARTESIAN_POINT('Ctrl Pts',(4.60004243494351,2.6871571650681,-21.7202056044043)) ;
#138158=CARTESIAN_POINT('Ctrl Pts',(4.5,2.68714139075511,-21.7202450179097)) ;
#138159=CARTESIAN_POINT('Ctrl Pts',(4.5,2.72431432344521,-21.627365183355)) ;
#138160=CARTESIAN_POINT('Origin',(4.6,0.280857398566761,-22.0051443914006)) ;
#138161=CARTESIAN_POINT('Origin',(4.6,2.1,-21.7019539578284)) ;
#138162=CARTESIAN_POINT('Origin',(4.6,2.1,-21.7019539578284)) ;
#138163=CARTESIAN_POINT('Origin',(4.6,0.,-20.32)) ;
#138164=CARTESIAN_POINT('',(4.5,-2.9,-20.3200000000039)) ;
#138165=CARTESIAN_POINT('',(4.57439618084313,-2.80937499999937,-21.3627958671254)) ;
#138166=CARTESIAN_POINT('Ctrl Pts',(4.5,-2.9,-20.3200000000039)) ;
#138167=CARTESIAN_POINT('Ctrl Pts',(4.5,-2.9000000234111,-20.4961762625703)) ;
#138168=CARTESIAN_POINT('Ctrl Pts',(4.49893459747296,-2.89187728142186,
-20.6722938225552)) ;
#138169=CARTESIAN_POINT('Ctrl Pts',(4.50498172725087,-2.86839426105774,
-20.9349432768872)) ;
#138170=CARTESIAN_POINT('Ctrl Pts',(4.50826226558342,-2.85869729223562,
-21.0222870271135)) ;
#138171=CARTESIAN_POINT('Ctrl Pts',(4.52028413974051,-2.84160518746962,
-21.1528409654328)) ;
#138172=CARTESIAN_POINT('Ctrl Pts',(4.52545003690602,-2.8354696349403,-21.196363113622)) ;
#138173=CARTESIAN_POINT('Ctrl Pts',(4.53741870680499,-2.82581179679252,
-21.2606394550108)) ;
#138174=CARTESIAN_POINT('Ctrl Pts',(4.54209540184575,-2.82251395224859,
-21.2819200182606)) ;
#138175=CARTESIAN_POINT('Ctrl Pts',(4.55451190949429,-2.81582803324483,
-21.3238742105328)) ;
#138176=CARTESIAN_POINT('Ctrl Pts',(4.56139306411848,-2.8124020390272,-21.3447435318249)) ;
#138177=CARTESIAN_POINT('Ctrl Pts',(4.57439618084313,-2.80937499999937,
-21.3627958671254)) ;
#138178=CARTESIAN_POINT('Ctrl Pts',(4.57439618084312,-2.80937499999939,
-21.3627958671254)) ;
#138179=CARTESIAN_POINT('Ctrl Pts',(4.57788811720509,-2.80856205104935,
-21.3676438845913)) ;
#138180=CARTESIAN_POINT('Ctrl Pts',(4.58132110715661,-2.80743849592504,
-21.3726543114197)) ;
#138181=CARTESIAN_POINT('Ctrl Pts',(4.58591063786558,-2.80541025280319,
-21.3800683491597)) ;
#138182=CARTESIAN_POINT('Ctrl Pts',(4.58721694730497,-2.80476695238161,
-21.3822683250837)) ;
#138183=CARTESIAN_POINT('Ctrl Pts',(4.58874498026859,-2.80393035430395,
-21.3849717146408)) ;
#138184=CARTESIAN_POINT('Ctrl Pts',(4.58900094431508,-2.80378708879839,
-21.385429423373)) ;
#138185=CARTESIAN_POINT('Ctrl Pts',(4.58924476828968,-2.80364801935069,
-21.38586949326)) ;
#138186=CARTESIAN_POINT('Ctrl Pts',(4.58924931741448,-2.80364542371033,
-21.3858777053493)) ;
#138187=CARTESIAN_POINT('Ctrl Pts',(4.59158188358133,-2.80231401319274,
-21.3900892401221)) ;
#138188=CARTESIAN_POINT('Ctrl Pts',(4.59377134212491,-2.80081309849101,
-21.3944383923964)) ;
#138189=CARTESIAN_POINT('Ctrl Pts',(4.59570408210449,-2.79909049146272,
-21.3991378632085)) ;
#138190=CARTESIAN_POINT('Ctrl Pts',(4.5957084873849,-2.79908656285629,-21.3991485795779)) ;
#138191=CARTESIAN_POINT('Ctrl Pts',(4.59603576097762,-2.79879453264352,
-21.3999450754362)) ;
#138192=CARTESIAN_POINT('Ctrl Pts',(4.59633794834607,-2.79851279959495,
-21.4007065253189)) ;
#138193=CARTESIAN_POINT('Ctrl Pts',(4.59727216584803,-2.79759800070515,
-21.40316063341)) ;
#138194=CARTESIAN_POINT('Ctrl Pts',(4.59785661125443,-2.79695684051616,
-21.4048529156094)) ;
#138195=CARTESIAN_POINT('Ctrl Pts',(4.59875882816121,-2.7958009226755,-21.4078683242216)) ;
#138196=CARTESIAN_POINT('Ctrl Pts',(4.59910960512327,-2.79529211440566,
-21.4091844992176)) ;
#138197=CARTESIAN_POINT('Ctrl Pts',(4.59950074890552,-2.79458032370895,
-21.4110150784121)) ;
#138198=CARTESIAN_POINT('Ctrl Pts',(4.59959271145697,-2.79439474074567,
-21.4114948405808)) ;
#138199=CARTESIAN_POINT('Ctrl Pts',(4.59970479219924,-2.79411978912795,
-21.4122025710462)) ;
#138200=CARTESIAN_POINT('Ctrl Pts',(4.59973686334512,-2.79403231884248,
-21.4124272684452)) ;
#138201=CARTESIAN_POINT('Ctrl Pts',(4.59980956306601,-2.7938042827674,-21.4130108264021)) ;
#138202=CARTESIAN_POINT('Ctrl Pts',(4.59984405921136,-2.79366555090847,
-21.4133689790042)) ;
#138203=CARTESIAN_POINT('Ctrl Pts',(4.59992170638736,-2.79338632637294,
-21.4140824135446)) ;
#138204=CARTESIAN_POINT('Ctrl Pts',(4.59995882625634,-2.79324305250058,
-21.4144374792565)) ;
#138205=CARTESIAN_POINT('Ctrl Pts',(4.59999999999999,-2.79310344827586,
-21.4147936459578)) ;
#138206=CARTESIAN_POINT('',(4.57439618084271,-2.80937499999947,-19.2772041328751)) ;
#138207=CARTESIAN_POINT('Ctrl Pts',(4.59999999999999,-2.79310344827586,
-19.2252063540422)) ;
#138208=CARTESIAN_POINT('Ctrl Pts',(4.59995895305209,-2.79324111387632,
-19.2255620070442)) ;
#138209=CARTESIAN_POINT('Ctrl Pts',(4.59992125133673,-2.79338175512528,
-19.2259166499952)) ;
#138210=CARTESIAN_POINT('Ctrl Pts',(4.59984242179761,-2.79365985893298,
-19.2266272182547)) ;
#138211=CARTESIAN_POINT('Ctrl Pts',(4.5998070294299,-2.79379858543765,-19.226981904003)) ;
#138212=CARTESIAN_POINT('Ctrl Pts',(4.59973261548695,-2.79401893257626,
-19.2275458212796)) ;
#138213=CARTESIAN_POINT('Ctrl Pts',(4.59970092564442,-2.7941005010842,-19.2277547044526)) ;
#138214=CARTESIAN_POINT('Ctrl Pts',(4.59958060815602,-2.79437456977472,
-19.2284570742577)) ;
#138215=CARTESIAN_POINT('Ctrl Pts',(4.59947821517874,-2.79456857658396,
-19.2289550953807)) ;
#138216=CARTESIAN_POINT('Ctrl Pts',(4.5990597198479,-2.79527981802027,-19.2307850643885)) ;
#138217=CARTESIAN_POINT('Ctrl Pts',(4.59869396429225,-2.79579226918927,
-19.2321114012001)) ;
#138218=CARTESIAN_POINT('Ctrl Pts',(4.59768320083749,-2.79706868650734,
-19.2354440738933)) ;
#138219=CARTESIAN_POINT('Ctrl Pts',(4.59698254015873,-2.79783590182173,
-19.2374731996627)) ;
#138220=CARTESIAN_POINT('Ctrl Pts',(4.5959970522588,-2.79876532988113,-19.2399846842385)) ;
#138221=CARTESIAN_POINT('Ctrl Pts',(4.59580678362761,-2.7989396411024,-19.2404581050039)) ;
#138222=CARTESIAN_POINT('Ctrl Pts',(4.59367882781298,-2.80083904916685,
-19.2456449119971)) ;
#138223=CARTESIAN_POINT('Ctrl Pts',(4.59150707087689,-2.80233337893514,
-19.2499793277041)) ;
#138224=CARTESIAN_POINT('Ctrl Pts',(4.58628071719247,-2.80532570224264,
-19.259451467429)) ;
#138225=CARTESIAN_POINT('Ctrl Pts',(4.58313959595737,-2.80673110767396,
-19.2645102480653)) ;
#138226=CARTESIAN_POINT('Ctrl Pts',(4.57802611146366,-2.80844040952806,
-19.2720963574913)) ;
#138227=CARTESIAN_POINT('Ctrl Pts',(4.57624387811663,-2.80894486836992,
-19.2746389593415)) ;
#138228=CARTESIAN_POINT('Ctrl Pts',(4.57439618084271,-2.80937499999947,
-19.2772041328751)) ;
#138229=CARTESIAN_POINT('Ctrl Pts',(4.57439618084271,-2.80937499999947,
-19.2772041328751)) ;
#138230=CARTESIAN_POINT('Ctrl Pts',(4.56149777794589,-2.81237766235467,
-19.2951110931668)) ;
#138231=CARTESIAN_POINT('Ctrl Pts',(4.55451596106519,-2.81582788236477,
-19.3161262422968)) ;
#138232=CARTESIAN_POINT('Ctrl Pts',(4.54213610452188,-2.82249001163036,
-19.3579283596283)) ;
#138233=CARTESIAN_POINT('Ctrl Pts',(4.53742891479326,-2.82580422498964,
-19.379310967236)) ;
#138234=CARTESIAN_POINT('Ctrl Pts',(4.525451614243,-2.8354670333868,-19.4436179437949)) ;
#138235=CARTESIAN_POINT('Ctrl Pts',(4.52032009146395,-2.84156292603926,
-19.4868565734785)) ;
#138236=CARTESIAN_POINT('Ctrl Pts',(4.50830110904356,-2.85862448221642,
-19.6171164259574)) ;
#138237=CARTESIAN_POINT('Ctrl Pts',(4.50499166750953,-2.86836219567853,
-19.7047300385823)) ;
#138238=CARTESIAN_POINT('Ctrl Pts',(4.49892845988062,-2.8918880660271,-19.9677629968379)) ;
#138239=CARTESIAN_POINT('Ctrl Pts',(4.49999999999474,-2.89999999999869,
-20.1438300901178)) ;
#138240=CARTESIAN_POINT('Ctrl Pts',(4.5,-2.9,-20.3200000000039)) ;
#138241=CARTESIAN_POINT('Origin',(4.4,-2.7,-17.78)) ;
#138242=CARTESIAN_POINT('Origin',(4.4,-2.7,-16.7631546211728)) ;
#138243=CARTESIAN_POINT('Origin',(4.4,-2.7,-18.7968453788272)) ;
#138244=CARTESIAN_POINT('Ctrl Pts',(4.40227435089069,-2.79999990867355,
-18.729400692882)) ;
#138245=CARTESIAN_POINT('Ctrl Pts',(4.51828879250233,-2.80015667527383,
-18.7387855667922)) ;
#138246=CARTESIAN_POINT('Ctrl Pts',(4.50118227077258,-2.68533700727761,
-18.7379711074493)) ;
#138247=CARTESIAN_POINT('Ctrl Pts',(4.39419482113923,-2.79999992837382,
-18.8436876996692)) ;
#138248=CARTESIAN_POINT('Ctrl Pts',(4.48571792501716,-2.80010751836587,
-18.822671366751)) ;
#138249=CARTESIAN_POINT('Ctrl Pts',(4.49717570077253,-2.71006921719264,
-18.8370318982147)) ;
#138250=CARTESIAN_POINT('Ctrl Pts',(4.40636790575266,-2.79999994706265,
-18.9549089073543)) ;
#138251=CARTESIAN_POINT('Ctrl Pts',(4.47481046024546,-2.80007242131916,
-18.9333224277989)) ;
#138252=CARTESIAN_POINT('Ctrl Pts',(4.50328131876399,-2.73353293829091,
-18.9370258748099)) ;
#138253=CARTESIAN_POINT('Ctrl Pts',(4.45479736994228,-2.79999997092221,
-19.1050736654711)) ;
#138254=CARTESIAN_POINT('Ctrl Pts',(4.49869786247045,-2.80003603117403,
-19.0862792434959)) ;
#138255=CARTESIAN_POINT('Ctrl Pts',(4.52748687875414,-2.7634897604751,-19.0762891728588)) ;
#138256=CARTESIAN_POINT('Ctrl Pts',(4.47221929614095,-2.79999997745988,
-19.1473040602233)) ;
#138257=CARTESIAN_POINT('Ctrl Pts',(4.50880556767619,-2.8000272573648,-19.1282748482859)) ;
#138258=CARTESIAN_POINT('Ctrl Pts',(4.53619137795526,-2.77169834185703,
-19.1159836823675)) ;
#138259=CARTESIAN_POINT('Ctrl Pts',(4.50882352800135,-2.7999999860536,-19.2042843496091)) ;
#138260=CARTESIAN_POINT('Ctrl Pts',(4.53367802911268,-2.80001636071785,
-19.1853587024204)) ;
#138261=CARTESIAN_POINT('Ctrl Pts',(4.55447319025663,-2.78248861123827,
-19.1700956814255)) ;
#138262=CARTESIAN_POINT('Ctrl Pts',(4.52308919141483,-2.79999998878206,
-19.2226625616911)) ;
#138263=CARTESIAN_POINT('Ctrl Pts',(4.54363962638622,-2.80001303821803,
-19.2037261501717)) ;
#138264=CARTESIAN_POINT('Ctrl Pts',(4.56159739427507,-2.78591449131415,
-19.1876542708947)) ;
#138265=CARTESIAN_POINT('Ctrl Pts',(4.57467506176493,-2.79999999510246,
-19.2656965083993)) ;
#138266=CARTESIAN_POINT('Ctrl Pts',(4.58062405303288,-2.80000557393877,
-19.2463341632777)) ;
#138267=CARTESIAN_POINT('Ctrl Pts',(4.58735613403293,-2.79385049254301,
-19.2289198149932)) ;
#138268=CARTESIAN_POINT('Ctrl Pts',(4.62437069655637,-2.79999999703807,
-19.2795313430603)) ;
#138269=CARTESIAN_POINT('Ctrl Pts',(4.61827372661892,-2.80000334969055,
-19.2609340454874)) ;
#138270=CARTESIAN_POINT('Ctrl Pts',(4.61212682540742,-2.79628090446614,
-19.242402814218)) ;
#138271=CARTESIAN_POINT('Ctrl Pts',(4.67161368302032,-2.7999999886062,-19.2207898267647)) ;
#138272=CARTESIAN_POINT('Ctrl Pts',(4.65407010102633,-2.80001325705931,
-19.2004637395898)) ;
#138273=CARTESIAN_POINT('Ctrl Pts',(4.63587130780619,-2.78569367459218,
-19.1856281295949)) ;
#138274=CARTESIAN_POINT('Ctrl Pts',(4.54879236204369,-2.8,-19.2435655563675)) ;
#138275=CARTESIAN_POINT('Ctrl Pts',(4.55448837802399,-2.7999999999815,-19.2411788209136)) ;
#138276=CARTESIAN_POINT('Ctrl Pts',(4.56021842726626,-2.79959150783238,
-19.2388395427341)) ;
#138277=CARTESIAN_POINT('Ctrl Pts',(4.56730671985007,-2.79865167182172,
-19.2359788838635)) ;
#138278=CARTESIAN_POINT('Ctrl Pts',(4.56847770958281,-2.79848295770256,
-19.2355073268347)) ;
#138279=CARTESIAN_POINT('Ctrl Pts',(4.5710752309902,-2.79808046368154,-19.234462962897)) ;
#138280=CARTESIAN_POINT('Ctrl Pts',(4.5725009361248,-2.79784058543152,-19.233889643028)) ;
#138281=CARTESIAN_POINT('Ctrl Pts',(4.5764383594612,-2.79713266293194,-19.2323136864649)) ;
#138282=CARTESIAN_POINT('Ctrl Pts',(4.57879956048961,-2.79666132938901,
-19.2313758003969)) ;
#138283=CARTESIAN_POINT('Ctrl Pts',(4.58293855712953,-2.79579586318667,
-19.2297608159296)) ;
#138284=CARTESIAN_POINT('Ctrl Pts',(4.58471363403687,-2.79540911153441,
-19.2290746171912)) ;
#138285=CARTESIAN_POINT('Ctrl Pts',(4.58699082729421,-2.7949269768198,-19.228244529262)) ;
#138286=CARTESIAN_POINT('Ctrl Pts',(4.58739952300692,-2.79484234870239,
-19.2281019268464)) ;
#138287=CARTESIAN_POINT('Ctrl Pts',(4.58871515235485,-2.79457617288695,
-19.2276611291009)) ;
#138288=CARTESIAN_POINT('Ctrl Pts',(4.5896169059614,-2.7944024780556,-19.2273849869995)) ;
#138289=CARTESIAN_POINT('Ctrl Pts',(4.59105375065865,-2.79414748185765,
-19.2269829818179)) ;
#138290=CARTESIAN_POINT('Ctrl Pts',(4.59155303909546,-2.79406229662442,
-19.2268492435071)) ;
#138291=CARTESIAN_POINT('Ctrl Pts',(4.59245965385668,-2.79391282221553,
-19.2266125941149)) ;
#138292=CARTESIAN_POINT('Ctrl Pts',(4.59286388425103,-2.79384761399903,
-19.2265084217845)) ;
#138293=CARTESIAN_POINT('Ctrl Pts',(4.59368973959979,-2.79370598615371,
-19.2262676726516)) ;
#138294=CARTESIAN_POINT('Ctrl Pts',(4.59407665941121,-2.79363973714592,
-19.2261515212332)) ;
#138295=CARTESIAN_POINT('Ctrl Pts',(4.5944437128773,-2.79357284110655,-19.2260267927279)) ;
#138296=CARTESIAN_POINT('Ctrl Pts',(4.59448890259158,-2.79356452972317,
-19.2260111581995)) ;
#138297=CARTESIAN_POINT('Ctrl Pts',(4.5947084233491,-2.79352377141065,-19.2259338254522)) ;
#138298=CARTESIAN_POINT('Ctrl Pts',(4.59483598733268,-2.79349361011836,
-19.2258723314841)) ;
#138299=CARTESIAN_POINT('Ctrl Pts',(4.59514620525222,-2.7934297131363,-19.2257459400492)) ;
#138300=CARTESIAN_POINT('Ctrl Pts',(4.595333342751,-2.79339696908416,-19.2256838378534)) ;
#138301=CARTESIAN_POINT('Ctrl Pts',(4.59563785533346,-2.79335634095568,
-19.2256129903403)) ;
#138302=CARTESIAN_POINT('Ctrl Pts',(4.59571710962761,-2.79334654412182,
-19.2255963912876)) ;
#138303=CARTESIAN_POINT('Ctrl Pts',(4.59594411915586,-2.79332043135007,
-19.2255533496182)) ;
#138304=CARTESIAN_POINT('Ctrl Pts',(4.59600288191152,-2.79330503361987,
-19.2255339512408)) ;
#138305=CARTESIAN_POINT('Ctrl Pts',(4.59613307952173,-2.79327450473787,
-19.2254992805194)) ;
#138306=CARTESIAN_POINT('Ctrl Pts',(4.59620389659311,-2.7932597078882,-19.2254850060586)) ;
#138307=CARTESIAN_POINT('Ctrl Pts',(4.5965119298477,-2.79322709231927,-19.2254502778629)) ;
#138308=CARTESIAN_POINT('Ctrl Pts',(4.59679543741294,-2.79320989448355,
-19.2254293441824)) ;
#138309=CARTESIAN_POINT('Ctrl Pts',(4.59784475938521,-2.793166495242,-19.2253578835066)) ;
#138310=CARTESIAN_POINT('Ctrl Pts',(4.59874915064778,-2.79313948637392,
-19.2252992643107)) ;
#138311=CARTESIAN_POINT('Ctrl Pts',(4.59999999999999,-2.79310344827586,
-19.2252063540422)) ;
#138312=CARTESIAN_POINT('Origin',(4.4,-2.7,-17.78)) ;
#138313=CARTESIAN_POINT('Origin',(4.4,-2.7,-21.8431546211728)) ;
#138314=CARTESIAN_POINT('Ctrl Pts',(4.5011795914298,-2.68531903459919,-21.9020290201724)) ;
#138315=CARTESIAN_POINT('Ctrl Pts',(4.5182867035893,-2.8,-21.9012138251407)) ;
#138316=CARTESIAN_POINT('Ctrl Pts',(4.40240952225579,-2.8,-21.9105883721108)) ;
#138317=CARTESIAN_POINT('Ctrl Pts',(4.49717774927195,-2.71005310920086,
-21.8029655323624)) ;
#138318=CARTESIAN_POINT('Ctrl Pts',(4.48574628541093,-2.8,-21.81731485204)) ;
#138319=CARTESIAN_POINT('Ctrl Pts',(4.39431668173579,-2.8,-21.7963402695081)) ;
#138320=CARTESIAN_POINT('Ctrl Pts',(4.50328690685189,-2.7335198760256,-21.7029733978621)) ;
#138321=CARTESIAN_POINT('Ctrl Pts',(4.47485145549547,-2.8,-21.7066766957415)) ;
#138322=CARTESIAN_POINT('Ctrl Pts',(4.40646789472125,-2.8,-21.6851226186384)) ;
#138323=CARTESIAN_POINT('Ctrl Pts',(4.52749311797091,-2.76348183928883,
-21.5637129921594)) ;
#138324=CARTESIAN_POINT('Ctrl Pts',(4.49873206155793,-2.8,-21.5537330953069)) ;
#138325=CARTESIAN_POINT('Ctrl Pts',(4.4548681704377,-2.8,-21.5349566433661)) ;
#138326=CARTESIAN_POINT('Ctrl Pts',(4.53619745972496,-2.77169205010104,
-21.5240190471853)) ;
#138327=CARTESIAN_POINT('Ctrl Pts',(4.50883664816672,-2.79999999999998,
-21.5117394381722)) ;
#138328=CARTESIAN_POINT('Ctrl Pts',(4.47227975612143,-2.8,-21.4927273846038)) ;
#138329=CARTESIAN_POINT('Ctrl Pts',(4.5544779509001,-2.78248459830341,-21.4699078127333)) ;
#138330=CARTESIAN_POINT('Ctrl Pts',(4.53370055749883,-2.80000000000001,
-21.4546579183699)) ;
#138331=CARTESIAN_POINT('Ctrl Pts',(4.50886586566856,-2.8,-21.4357478882722)) ;
#138332=CARTESIAN_POINT('Ctrl Pts',(4.56160154376425,-2.78591123334062,
-21.4523494428157)) ;
#138333=CARTESIAN_POINT('Ctrl Pts',(4.54365878772218,-2.8,-21.4362910664543)) ;
#138334=CARTESIAN_POINT('Ctrl Pts',(4.52312452397685,-2.8,-21.4173699954867)) ;
#138335=CARTESIAN_POINT('Ctrl Pts',(4.58735772267362,-2.79384903998488,
-21.4110842943985)) ;
#138336=CARTESIAN_POINT('Ctrl Pts',(4.58063087367386,-2.8,-21.3936839633808)) ;
#138337=CARTESIAN_POINT('Ctrl Pts',(4.5746855076719,-2.8,-21.3743374866056)) ;
#138338=CARTESIAN_POINT('Ctrl Pts',(4.61212536563479,-2.79628002040276,
-21.3976015865954)) ;
#138339=CARTESIAN_POINT('Ctrl Pts',(4.61826745782993,-2.80000000000002,
-21.3790848793757)) ;
#138340=CARTESIAN_POINT('Ctrl Pts',(4.62435992349572,-2.8,-21.3605015173211)) ;
#138341=CARTESIAN_POINT('Ctrl Pts',(4.63586710715927,-2.78569036914666,
-21.4543752946752)) ;
#138342=CARTESIAN_POINT('Ctrl Pts',(4.6540510694572,-2.79999999999994,-21.4395525238841)) ;
#138343=CARTESIAN_POINT('Ctrl Pts',(4.67158355065736,-2.8,-21.4192450797819)) ;
#138344=CARTESIAN_POINT('Ctrl Pts',(4.59999999999999,-2.79310344827586,
-21.4147936459578)) ;
#138345=CARTESIAN_POINT('Ctrl Pts',(4.59840954578207,-2.79314968944989,
-21.4146756726912)) ;
#138346=CARTESIAN_POINT('Ctrl Pts',(4.59737383489079,-2.79318159606221,
-21.4146133239717)) ;
#138347=CARTESIAN_POINT('Ctrl Pts',(4.59650507521642,-2.79322931786013,
-21.41455037726)) ;
#138348=CARTESIAN_POINT('Ctrl Pts',(4.59632758424299,-2.79324472590582,
-21.4145345791767)) ;
#138349=CARTESIAN_POINT('Ctrl Pts',(4.59611847210843,-2.79327477162037,
-21.4145047565772)) ;
#138350=CARTESIAN_POINT('Ctrl Pts',(4.59606489504924,-2.79328892979787,
-21.4144910265853)) ;
#138351=CARTESIAN_POINT('Ctrl Pts',(4.59594601677692,-2.79331605564258,
-21.414459114495)) ;
#138352=CARTESIAN_POINT('Ctrl Pts',(4.59588597444856,-2.7933285533825,-21.4144426561835)) ;
#138353=CARTESIAN_POINT('Ctrl Pts',(4.59549967474362,-2.79337285752324,
-21.4143702787605)) ;
#138354=CARTESIAN_POINT('Ctrl Pts',(4.59527331486236,-2.79340622385959,
-21.4143100807083)) ;
#138355=CARTESIAN_POINT('Ctrl Pts',(4.59493201239528,-2.79346950514991,
-21.4141870402937)) ;
#138356=CARTESIAN_POINT('Ctrl Pts',(4.59480393230127,-2.79349821606423,
-21.414128474279)) ;
#138357=CARTESIAN_POINT('Ctrl Pts',(4.59460326813593,-2.79353924388982,
-21.4140476351491)) ;
#138358=CARTESIAN_POINT('Ctrl Pts',(4.59455075953095,-2.79354963432651,
-21.4140274276715)) ;
#138359=CARTESIAN_POINT('Ctrl Pts',(4.59417008680874,-2.79361944405452,
-21.4138955937176)) ;
#138360=CARTESIAN_POINT('Ctrl Pts',(4.59377742096551,-2.79368602572532,
-21.4137773461555)) ;
#138361=CARTESIAN_POINT('Ctrl Pts',(4.59289939109635,-2.7938335466559,-21.4135254190241)) ;
#138362=CARTESIAN_POINT('Ctrl Pts',(4.59245006584786,-2.79390305456781,
-21.413416036199)) ;
#138363=CARTESIAN_POINT('Ctrl Pts',(4.59099552519241,-2.79413629528604,
-21.4130568524093)) ;
#138364=CARTESIAN_POINT('Ctrl Pts',(4.59002197881585,-2.79430302757315,
-21.412806370176)) ;
#138365=CARTESIAN_POINT('Ctrl Pts',(4.58861122644683,-2.794567934557,-21.4123921365669)) ;
#138366=CARTESIAN_POINT('Ctrl Pts',(4.58817904894403,-2.79465210327453,
-21.4122585234306)) ;
#138367=CARTESIAN_POINT('Ctrl Pts',(4.58736872283365,-2.79481449815582,
-21.4119941835896)) ;
#138368=CARTESIAN_POINT('Ctrl Pts',(4.58699491219416,-2.79489135860974,
-21.4118665823581)) ;
#138369=CARTESIAN_POINT('Ctrl Pts',(4.58468897497188,-2.79537899446709,
-21.4110351906196)) ;
#138370=CARTESIAN_POINT('Ctrl Pts',(4.58290717718701,-2.79577019617637,
-21.4103420642284)) ;
#138371=CARTESIAN_POINT('Ctrl Pts',(4.57867627871776,-2.79666451416567,
-21.4086707882875)) ;
#138372=CARTESIAN_POINT('Ctrl Pts',(4.57626321554131,-2.79715040843617,
-21.4076877651429)) ;
#138373=CARTESIAN_POINT('Ctrl Pts',(4.57243386308706,-2.79784156172336,
-21.4061367865103)) ;
#138374=CARTESIAN_POINT('Ctrl Pts',(4.57107519984217,-2.79807176647234,
-21.405584021445)) ;
#138375=CARTESIAN_POINT('Ctrl Pts',(4.56513452430471,-2.79900074294391,
-21.4031693903581)) ;
#138376=CARTESIAN_POINT('Ctrl Pts',(4.56062162665738,-2.7995126701138,-21.4013309293494)) ;
#138377=CARTESIAN_POINT('Ctrl Pts',(4.55365420596628,-2.79992470862867,
-21.3984610302783)) ;
#138378=CARTESIAN_POINT('Ctrl Pts',(4.55124660967264,-2.79999983267432,
-21.3974632392507)) ;
#138379=CARTESIAN_POINT('Ctrl Pts',(4.54880051362942,-2.79999999972164,
-21.3964378607329)) ;
#138380=CARTESIAN_POINT('Ctrl Pts',(4.54879236166274,-2.8,-19.2435655565152)) ;
#138381=CARTESIAN_POINT('Ctrl Pts',(4.5622387183224,-2.79999999999679,-19.2612315262749)) ;
#138382=CARTESIAN_POINT('Ctrl Pts',(4.57442182196495,-2.80939476060287,
-19.2772378204668)) ;
#138383=CARTESIAN_POINT('Ctrl Pts',(4.55556842517593,-2.79999999999889,
-19.2407250640489)) ;
#138384=CARTESIAN_POINT('Ctrl Pts',(4.56783337210914,-2.80040661803737,
-19.2561863015519)) ;
#138385=CARTESIAN_POINT('Ctrl Pts',(4.57961823522371,-2.80818164104597,
-19.2700183413272)) ;
#138386=CARTESIAN_POINT('Ctrl Pts',(4.56238982831618,-2.7994260255176,-19.2379528515171)) ;
#138387=CARTESIAN_POINT('Ctrl Pts',(4.57357810388182,-2.80014618986473,
-19.2509310721412)) ;
#138388=CARTESIAN_POINT('Ctrl Pts',(4.58462643299473,-2.80630261261112,
-19.2625232711649)) ;
#138389=CARTESIAN_POINT('Ctrl Pts',(4.57328757735258,-2.7977370397245,-19.2335699979501)) ;
#138390=CARTESIAN_POINT('Ctrl Pts',(4.58237922839514,-2.79856394574987,
-19.2422664089313)) ;
#138391=CARTESIAN_POINT('Ctrl Pts',(4.59151541127592,-2.80237286596198,
-19.2500830028806)) ;
#138392=CARTESIAN_POINT('Ctrl Pts',(4.57700059755675,-2.7970371466716,-19.232076076342)) ;
#138393=CARTESIAN_POINT('Ctrl Pts',(4.58532305318677,-2.79784352093717,
-19.2392625430045)) ;
#138394=CARTESIAN_POINT('Ctrl Pts',(4.59370961102545,-2.80088045369937,
-19.2457455141894)) ;
#138395=CARTESIAN_POINT('Ctrl Pts',(4.58319893207066,-2.79574016930783,
-19.2296546705211)) ;
#138396=CARTESIAN_POINT('Ctrl Pts',(4.58990416109239,-2.79637293360539,
-19.2343303545622)) ;
#138397=CARTESIAN_POINT('Ctrl Pts',(4.59665800356694,-2.79825577077759,
-19.2385819448697)) ;
#138398=CARTESIAN_POINT('Ctrl Pts',(4.58534994317985,-2.79526732601294,
-19.2288188618872)) ;
#138399=CARTESIAN_POINT('Ctrl Pts',(4.59144552977844,-2.79581844972913,
-19.2326200366107)) ;
#138400=CARTESIAN_POINT('Ctrl Pts',(4.59758018705035,-2.79731769672697,
-19.2360885803939)) ;
#138401=CARTESIAN_POINT('Ctrl Pts',(4.58899927751306,-2.79450268149332,
-19.2275173012671)) ;
#138402=CARTESIAN_POINT('Ctrl Pts',(4.59386223202754,-2.79488630507105,
-19.2299495170303)) ;
#138403=CARTESIAN_POINT('Ctrl Pts',(4.59874684688641,-2.79582009356911,
-19.2321813652447)) ;
#138404=CARTESIAN_POINT('Ctrl Pts',(4.5902675569287,-2.79423885380164,-19.22707439958)) ;
#138405=CARTESIAN_POINT('Ctrl Pts',(4.59467706068311,-2.79455862385203,
-19.2290405433361)) ;
#138406=CARTESIAN_POINT('Ctrl Pts',(4.59910266898802,-2.79530499526365,
-19.2308486399022)) ;
#138407=CARTESIAN_POINT('Ctrl Pts',(4.59257623319511,-2.79382131826659,
-19.22638413145)) ;
#138408=CARTESIAN_POINT('Ctrl Pts',(4.59605751036344,-2.79403163929514,
-19.2276227610336)) ;
#138409=CARTESIAN_POINT('Ctrl Pts',(4.59954701072604,-2.79449510806573,
-19.228765766817)) ;
#138410=CARTESIAN_POINT('Ctrl Pts',(4.59342976933296,-2.79367543507711,
-19.2261445374534)) ;
#138411=CARTESIAN_POINT('Ctrl Pts',(4.59655016100493,-2.79384713427255,
-19.2271348895303)) ;
#138412=CARTESIAN_POINT('Ctrl Pts',(4.59967640178298,-2.79421605292372,
-19.228050213937)) ;
#138413=CARTESIAN_POINT('Ctrl Pts',(4.59428414179642,-2.79346156087783,
-19.2257069361853)) ;
#138414=CARTESIAN_POINT('Ctrl Pts',(4.59704519451433,-2.79355469746529,
-19.226373635748)) ;
#138415=CARTESIAN_POINT('Ctrl Pts',(4.5998104157401,-2.79379877456676,-19.2269823712707)) ;
#138416=CARTESIAN_POINT('Ctrl Pts',(4.59432658472651,-2.7933916625364,-19.2255338181495)) ;
#138417=CARTESIAN_POINT('Ctrl Pts',(4.59708408719787,-2.79345234504014,
-19.2261090766463)) ;
#138418=CARTESIAN_POINT('Ctrl Pts',(4.59984563524626,-2.79366003518351,
-19.2266276543527)) ;
#138419=CARTESIAN_POINT('Ctrl Pts',(4.59537197237732,-2.79324260992761,
-19.2252872615938)) ;
#138420=CARTESIAN_POINT('Ctrl Pts',(4.59764722167538,-2.79326383513929,
-19.225620961855)) ;
#138421=CARTESIAN_POINT('Ctrl Pts',(4.59992475053754,-2.79338190759658,
-19.2259170306476)) ;
#138422=CARTESIAN_POINT('Ctrl Pts',(4.5936418339237,-2.79313407032025,-19.2252844788451)) ;
#138423=CARTESIAN_POINT('Ctrl Pts',(4.59684754854888,-2.79327107597598,
-19.2256389310452)) ;
#138424=CARTESIAN_POINT('Ctrl Pts',(4.59996664298755,-2.79324102308607,
-19.2255617736815)) ;
#138425=CARTESIAN_POINT('Ctrl Pts',(4.59999999999999,-2.79310344827586,
-19.2252063540422)) ;
#138426=CARTESIAN_POINT('Ctrl Pts',(4.59999999999999,-2.79310344827586,
-19.2252063540422)) ;
#138427=CARTESIAN_POINT('Ctrl Pts',(4.59999999999999,-2.79310344827586,
-19.2252063540422)) ;
#138428=CARTESIAN_POINT('Origin',(4.54879236168542,-2.9,-19.2435655565161)) ;
#138429=CARTESIAN_POINT('Ctrl Pts',(4.39959973407451,-2.8,-20.4305922428025)) ;
#138430=CARTESIAN_POINT('Ctrl Pts',(4.49922290141883,-2.8,-20.4301052483314)) ;
#138431=CARTESIAN_POINT('Ctrl Pts',(4.49980764094185,-2.89969504276379,
-20.430608045895)) ;
#138432=CARTESIAN_POINT('Ctrl Pts',(4.40142712570759,-2.8,-20.2095338960077)) ;
#138433=CARTESIAN_POINT('Ctrl Pts',(4.50593622119657,-2.8,-20.2060480134683)) ;
#138434=CARTESIAN_POINT('Ctrl Pts',(4.50067611734352,-2.90411960318544,
-20.2096502871254)) ;
#138435=CARTESIAN_POINT('Ctrl Pts',(4.39573539165433,-2.8,-19.9876225417885)) ;
#138436=CARTESIAN_POINT('Ctrl Pts',(4.49039105203437,-2.8,-20.0064448660088)) ;
#138437=CARTESIAN_POINT('Ctrl Pts',(4.49793210898571,-2.89506044297342,
-19.9865928350696)) ;
#138438=CARTESIAN_POINT('Ctrl Pts',(4.41164816536272,-2.8,-19.6744921486565)) ;
#138439=CARTESIAN_POINT('Ctrl Pts',(4.48203507549541,-2.8,-19.6830075383891)) ;
#138440=CARTESIAN_POINT('Ctrl Pts',(4.50604587949365,-2.86657833599735,
-19.6817916334551)) ;
#138441=CARTESIAN_POINT('Ctrl Pts',(4.41940490599905,-2.8,-19.5821571319988)) ;
#138442=CARTESIAN_POINT('Ctrl Pts',(4.48133975791573,-2.8,-19.5933274637386)) ;
#138443=CARTESIAN_POINT('Ctrl Pts',(4.50997623336227,-2.85625883833135,
-19.593064643239)) ;
#138444=CARTESIAN_POINT('Ctrl Pts',(4.44577434373644,-2.8,-19.4470206588259)) ;
#138445=CARTESIAN_POINT('Ctrl Pts',(4.49360122670477,-2.8,-19.4593305876678)) ;
#138446=CARTESIAN_POINT('Ctrl Pts',(4.52318558604184,-2.83896465559566,
-19.4654850424376)) ;
#138447=CARTESIAN_POINT('Ctrl Pts',(4.45692583760033,-2.8,-19.4024768930528)) ;
#138448=CARTESIAN_POINT('Ctrl Pts',(4.49949391572662,-2.8,-19.4160543026461)) ;
#138449=CARTESIAN_POINT('Ctrl Pts',(4.52876348458384,-2.83289258157629,
-19.4238029886043)) ;
#138450=CARTESIAN_POINT('Ctrl Pts',(4.50378503771657,-2.8,-19.2810759162582)) ;
#138451=CARTESIAN_POINT('Ctrl Pts',(4.52873519606818,-2.8,-19.2999253422748)) ;
#138452=CARTESIAN_POINT('Ctrl Pts',(4.55214466721903,-2.81552005845344,
-19.3112248698016)) ;
#138453=CARTESIAN_POINT('Ctrl Pts',(4.54714423790153,-2.8,-19.202268495047)) ;
#138454=CARTESIAN_POINT('Ctrl Pts',(4.55761617337286,-2.8,-19.2232065641883)) ;
#138455=CARTESIAN_POINT('Ctrl Pts',(4.57259584813385,-2.80338245043788,
-19.2412385951886)) ;
#138456=CARTESIAN_POINT('Ctrl Pts',(4.67762904165671,-2.8,-19.2114950447958)) ;
#138457=CARTESIAN_POINT('Ctrl Pts',(4.6609348472501,-2.8,-19.227067065838)) ;
#138458=CARTESIAN_POINT('Ctrl Pts',(4.64133868807456,-2.80368623369359,
-19.244688006387)) ;
#138459=CARTESIAN_POINT('Origin',(4.4,-2.9,-20.3200000000039)) ;
#138460=CARTESIAN_POINT('Ctrl Pts',(4.72172783566993,-2.8000000024879,-21.4203629549132)) ;
#138461=CARTESIAN_POINT('Ctrl Pts',(4.69645430308119,-2.79999660525783,
-21.4070700473094)) ;
#138462=CARTESIAN_POINT('Ctrl Pts',(4.66463283184998,-2.80454824226955,
-21.3894903682926)) ;
#138463=CARTESIAN_POINT('Ctrl Pts',(4.55709227475146,-2.80000000030524,
-21.45599643631)) ;
#138464=CARTESIAN_POINT('Ctrl Pts',(4.56399237478645,-2.79999958643658,
-21.4339593792008)) ;
#138465=CARTESIAN_POINT('Ctrl Pts',(4.5772937099949,-2.80055804294512,-21.4151759050809)) ;
#138466=CARTESIAN_POINT('Ctrl Pts',(4.50667826286324,-2.80000000784871,
-21.3666146479982)) ;
#138467=CARTESIAN_POINT('Ctrl Pts',(4.53037382014976,-2.79998899178916,
-21.3470846001168)) ;
#138468=CARTESIAN_POINT('Ctrl Pts',(4.55348183854635,-2.81434699509192,
-21.3359466041139)) ;
#138469=CARTESIAN_POINT('Ctrl Pts',(4.4569228015872,-2.80000001789831,-21.2376422182876)) ;
#138470=CARTESIAN_POINT('Ctrl Pts',(4.49938029267362,-2.79997354447564,
-21.2240998880093)) ;
#138471=CARTESIAN_POINT('Ctrl Pts',(4.52864149761198,-2.83271033979002,
-21.21632906208)) ;
#138472=CARTESIAN_POINT('Ctrl Pts',(4.44554661086163,-2.80000002126189,
-21.1923774400141)) ;
#138473=CARTESIAN_POINT('Ctrl Pts',(4.4933366515485,-2.7999679796365,-21.1800969398739)) ;
#138474=CARTESIAN_POINT('Ctrl Pts',(4.52295544156354,-2.83885474437117,
-21.1739678582281)) ;
#138475=CARTESIAN_POINT('Ctrl Pts',(4.4190332210433,-2.8000000307772,-21.0558947975771)) ;
#138476=CARTESIAN_POINT('Ctrl Pts',(4.48100616080231,-2.79995095769178,
-21.0447300040204)) ;
#138477=CARTESIAN_POINT('Ctrl Pts',(4.50969337368895,-2.8562317909387,-21.0450696236088)) ;
#138478=CARTESIAN_POINT('Ctrl Pts',(4.41147189908671,-2.8000000363501,-20.9642415900435)) ;
#138479=CARTESIAN_POINT('Ctrl Pts',(4.48178828424047,-2.79993989905026,
-20.9557891492056)) ;
#138480=CARTESIAN_POINT('Ctrl Pts',(4.50589025525737,-2.86640526991132,
-20.9569681512011)) ;
#138481=CARTESIAN_POINT('Ctrl Pts',(4.39523119070906,-2.80000005228416,
-20.6431795198329)) ;
#138482=CARTESIAN_POINT('Ctrl Pts',(4.49033836345893,-2.799902616883,-20.6230741316605)) ;
#138483=CARTESIAN_POINT('Ctrl Pts',(4.49769757367177,-2.89547737952995,
-20.6443332157617)) ;
#138484=CARTESIAN_POINT('Ctrl Pts',(4.40178225889352,-2.80000005718968,
-20.4126239782851)) ;
#138485=CARTESIAN_POINT('Ctrl Pts',(4.5068134101818,-2.79988784121837,-20.4170581988245)) ;
#138486=CARTESIAN_POINT('Ctrl Pts',(4.50092255053476,-2.90441958896086,
-20.4124406960391)) ;
#138487=CARTESIAN_POINT('Ctrl Pts',(4.39924589760301,-2.80000005405718,
-20.1830311688801)) ;
#138488=CARTESIAN_POINT('Ctrl Pts',(4.49795607191397,-2.79989746608212,
-20.183922937496)) ;
#138489=CARTESIAN_POINT('Ctrl Pts',(4.49968270404899,-2.89870974459557,
-20.1830284945916)) ;
#138490=CARTESIAN_POINT('Origin',(4.54879236168626,-2.9,-21.3964344434846)) ;
#138491=CARTESIAN_POINT('Ctrl Pts',(4.57442492185552,-2.80939715119899,
-21.3627581068621)) ;
#138492=CARTESIAN_POINT('Ctrl Pts',(4.56210583156797,-2.7998961275033,-21.3789430617887)) ;
#138493=CARTESIAN_POINT('Ctrl Pts',(4.54850917782858,-2.80000109307748,
-21.396806493488)) ;
#138494=CARTESIAN_POINT('Ctrl Pts',(4.57959763980855,-2.80818914940071,
-21.3699453004955)) ;
#138495=CARTESIAN_POINT('Ctrl Pts',(4.56768008075466,-2.80031924975226,
-21.3839410457291)) ;
#138496=CARTESIAN_POINT('Ctrl Pts',(4.55527876038347,-2.79999229227378,
-21.3995899763868)) ;
#138497=CARTESIAN_POINT('Ctrl Pts',(4.58464248447265,-2.80630474344638,
-21.3774843126383)) ;
#138498=CARTESIAN_POINT('Ctrl Pts',(4.57346944634373,-2.80008318972135,
-21.3892012910521)) ;
#138499=CARTESIAN_POINT('Ctrl Pts',(4.56216307187796,-2.79941338753917,
-21.4023280915335)) ;
#138500=CARTESIAN_POINT('Ctrl Pts',(4.59159231899494,-2.80232720646228,
-21.3900563692959)) ;
#138501=CARTESIAN_POINT('Ctrl Pts',(4.58237910662986,-2.79850221241048,
-21.3979149362578)) ;
#138502=CARTESIAN_POINT('Ctrl Pts',(4.57321634584969,-2.79769868647539,
-21.4066644864947)) ;
#138503=CARTESIAN_POINT('Ctrl Pts',(4.59378564167737,-2.8008235544484,-21.3944145837655)) ;
#138504=CARTESIAN_POINT('Ctrl Pts',(4.58533966160573,-2.79778056279966,
-21.4009180694478)) ;
#138505=CARTESIAN_POINT('Ctrl Pts',(4.5769613009382,-2.79699227428058,-21.4081320740362)) ;
#138506=CARTESIAN_POINT('Ctrl Pts',(4.59669734138576,-2.79821861236081,
-21.4015174469091)) ;
#138507=CARTESIAN_POINT('Ctrl Pts',(4.58989502505308,-2.79633072300511,
-21.405783702985)) ;
#138508=CARTESIAN_POINT('Ctrl Pts',(4.58314295739388,-2.79570785369251,
-21.4104789031814)) ;
#138509=CARTESIAN_POINT('Ctrl Pts',(4.59760632414569,-2.79728965034655,
-21.4039852466291)) ;
#138510=CARTESIAN_POINT('Ctrl Pts',(4.59142619397024,-2.79578507327359,
-21.4074678937229)) ;
#138511=CARTESIAN_POINT('Ctrl Pts',(4.58528630332435,-2.79524119148169,
-21.411287378375)) ;
#138512=CARTESIAN_POINT('Ctrl Pts',(4.59875741430932,-2.79580683383092,
-21.407853004496)) ;
#138513=CARTESIAN_POINT('Ctrl Pts',(4.59383193680336,-2.79486773439435,
-21.4100980055339)) ;
#138514=CARTESIAN_POINT('Ctrl Pts',(4.58892874314202,-2.79448758877844,
-21.4125464730129)) ;
#138515=CARTESIAN_POINT('Ctrl Pts',(4.59910834609946,-2.79529718130591,
-21.4091714993015)) ;
#138516=CARTESIAN_POINT('Ctrl Pts',(4.59464343907619,-2.79454543406795,
-21.4109926958501)) ;
#138517=CARTESIAN_POINT('Ctrl Pts',(4.59019511689892,-2.79422790851556,
-21.4129746712091)) ;
#138518=CARTESIAN_POINT('Ctrl Pts',(4.59954688679867,-2.79449699552073,
-21.4112293846587)) ;
#138519=CARTESIAN_POINT('Ctrl Pts',(4.59601732089137,-2.79402779797775,
-21.4123863363518)) ;
#138520=CARTESIAN_POINT('Ctrl Pts',(4.59249627585273,-2.79381771894921,
-21.4136411141675)) ;
#138521=CARTESIAN_POINT('Ctrl Pts',(4.59967529310588,-2.79422450025963,
-21.4119354645612)) ;
#138522=CARTESIAN_POINT('Ctrl Pts',(4.59651100242294,-2.79384821317134,
-21.4128644108735)) ;
#138523=CARTESIAN_POINT('Ctrl Pts',(4.593352874124,-2.79367727499394,-21.4138714476574)) ;
#138524=CARTESIAN_POINT('Ctrl Pts',(4.59980981518572,-2.79380630943631,
-21.4130056452101)) ;
#138525=CARTESIAN_POINT('Ctrl Pts',(4.59701056623719,-2.79355888022806,
-21.4136249350365)) ;
#138526=CARTESIAN_POINT('Ctrl Pts',(4.59421559911326,-2.79346462438277,
-21.4143030289899)) ;
#138527=CARTESIAN_POINT('Ctrl Pts',(4.59984534134842,-2.79366726490194,
-21.4133646067489)) ;
#138528=CARTESIAN_POINT('Ctrl Pts',(4.59705039509825,-2.79345667046144,
-21.4138917393962)) ;
#138529=CARTESIAN_POINT('Ctrl Pts',(4.59425962044002,-2.79339574833516,
-21.4144765637042)) ;
#138530=CARTESIAN_POINT('Ctrl Pts',(4.59992484646001,-2.7933873519883,-21.41407980384)) ;
#138531=CARTESIAN_POINT('Ctrl Pts',(4.59761652863209,-2.79326682373741,
-21.414380589531)) ;
#138532=CARTESIAN_POINT('Ctrl Pts',(4.59531061070857,-2.79324678512396,
-21.4147204137335)) ;
#138533=CARTESIAN_POINT('Ctrl Pts',(4.59996721368508,-2.79324340897637,
-21.414436569794)) ;
#138534=CARTESIAN_POINT('Ctrl Pts',(4.59680854952869,-2.79327323421043,
-21.4143604778616)) ;
#138535=CARTESIAN_POINT('Ctrl Pts',(4.59356174266139,-2.79313094944462,
-21.4147234833207)) ;
#138536=CARTESIAN_POINT('Ctrl Pts',(4.59999999999999,-2.79310344827586,
-21.4147936459578)) ;
#138537=CARTESIAN_POINT('Ctrl Pts',(4.59999999999999,-2.79310344827586,
-21.4147936459578)) ;
#138538=CARTESIAN_POINT('Ctrl Pts',(4.59999999999999,-2.79310344827586,
-21.4147936459578)) ;
#138539=CARTESIAN_POINT('Origin',(0.,0.,-22.36)) ;
#138540=CARTESIAN_POINT('Origin',(7.26810489940853,5.50476046277485,-18.945)) ;
#138541=CARTESIAN_POINT('',(4.03523814377473,5.98727788898885,-18.845)) ;
#138542=CARTESIAN_POINT('',(4.03523814377473,5.98727788898885,-17.545)) ;
#138543=CARTESIAN_POINT('',(4.03523814377473,5.98727788898885,-18.945)) ;
#138544=CARTESIAN_POINT('',(7.26810489940853,5.50476046277485,-17.545)) ;
#138545=CARTESIAN_POINT('',(7.26810489940853,5.50476046277485,-17.545)) ;
#138546=CARTESIAN_POINT('',(7.26810489940853,5.50476046277485,-18.845)) ;
#138547=CARTESIAN_POINT('',(7.26810489940853,5.50476046277485,-18.945)) ;
#138548=CARTESIAN_POINT('',(3.95,6.,-18.845)) ;
#138549=CARTESIAN_POINT('Origin',(7.25334304318326,5.40585602606554,-18.945)) ;
#138550=CARTESIAN_POINT('',(7.32310496992715,5.47750289324744,-17.545)) ;
#138551=CARTESIAN_POINT('Origin',(7.25334304318326,5.40585602606554,-17.545)) ;
#138552=CARTESIAN_POINT('',(7.32310496992715,5.47750289324744,-18.845)) ;
#138553=CARTESIAN_POINT('',(7.32310496992715,5.47750289324744,-18.945)) ;
#138554=CARTESIAN_POINT('Origin',(7.25334304318326,5.40585602606554,-18.845)) ;
#138555=CARTESIAN_POINT('Origin',(8.66976192674389,4.16627481495487,-18.945)) ;
#138556=CARTESIAN_POINT('',(8.66976192674389,4.16627481495487,-17.545)) ;
#138557=CARTESIAN_POINT('',(8.66976192674389,4.16627481495487,-17.545)) ;
#138558=CARTESIAN_POINT('',(8.66976192674389,4.16627481495487,-18.845)) ;
#138559=CARTESIAN_POINT('',(8.66976192674389,4.16627481495487,-18.945)) ;
#138560=CARTESIAN_POINT('',(7.32310496992715,5.47750289324744,-18.845)) ;
#138561=CARTESIAN_POINT('Origin',(8.6,4.09462794777298,-18.945)) ;
#138562=CARTESIAN_POINT('',(8.7,4.09462794777298,-17.545)) ;
#138563=CARTESIAN_POINT('Origin',(8.6,4.09462794777298,-17.545)) ;
#138564=CARTESIAN_POINT('',(8.7,4.09462794777298,-18.845)) ;
#138565=CARTESIAN_POINT('',(8.7,4.09462794777298,-18.945)) ;
#138566=CARTESIAN_POINT('Origin',(8.6,4.09462794777298,-18.845)) ;
#138567=CARTESIAN_POINT('Origin',(8.7,3.95,-18.945)) ;
#138568=CARTESIAN_POINT('',(8.7,3.95,-17.545)) ;
#138569=CARTESIAN_POINT('',(8.7,3.95,-17.545)) ;
#138570=CARTESIAN_POINT('',(8.7,3.95,-18.845)) ;
#138571=CARTESIAN_POINT('',(8.7,3.95,-18.945)) ;
#138572=CARTESIAN_POINT('',(8.7,4.09462794777298,-18.845)) ;
#138573=CARTESIAN_POINT('Origin',(8.6,3.95,-18.945)) ;
#138574=CARTESIAN_POINT('',(8.55460943381591,3.86089502538305,-17.545)) ;
#138575=CARTESIAN_POINT('Origin',(8.6,3.95,-17.545)) ;
#138576=CARTESIAN_POINT('',(8.55460943381591,3.86089502538305,-18.845)) ;
#138577=CARTESIAN_POINT('',(8.55460943381591,3.86089502538305,-18.945)) ;
#138578=CARTESIAN_POINT('Origin',(8.6,3.95,-18.845)) ;
#138579=CARTESIAN_POINT('Origin',(7.3213877252879,4.48910497461695,-18.945)) ;
#138580=CARTESIAN_POINT('',(7.3213877252879,4.48910497461695,-17.545)) ;
#138581=CARTESIAN_POINT('',(7.3213877252879,4.48910497461695,-17.545)) ;
#138582=CARTESIAN_POINT('',(7.3213877252879,4.48910497461695,-18.845)) ;
#138583=CARTESIAN_POINT('',(7.3213877252879,4.48910497461695,-18.945)) ;
#138584=CARTESIAN_POINT('',(8.55460943381591,3.86089502538305,-18.845)) ;
#138585=CARTESIAN_POINT('Origin',(7.27599715910381,4.4,-18.945)) ;
#138586=CARTESIAN_POINT('',(7.27599715910381,4.5,-17.545)) ;
#138587=CARTESIAN_POINT('Origin',(7.27599715910381,4.4,-17.545)) ;
#138588=CARTESIAN_POINT('',(7.27599715910381,4.5,-18.845)) ;
#138589=CARTESIAN_POINT('',(7.27599715910381,4.5,-18.945)) ;
#138590=CARTESIAN_POINT('Origin',(7.27599715910381,4.4,-18.845)) ;
#138591=CARTESIAN_POINT('Origin',(3.95,4.5,-18.945)) ;
#138592=CARTESIAN_POINT('',(4.05,4.5,-17.545)) ;
#138593=CARTESIAN_POINT('',(3.95,4.5,-17.545)) ;
#138594=CARTESIAN_POINT('',(4.05,4.5,-18.845)) ;
#138595=CARTESIAN_POINT('',(4.05,4.5,-18.945)) ;
#138596=CARTESIAN_POINT('',(7.27599715910381,4.5,-18.845)) ;
#138597=CARTESIAN_POINT('Origin',(7.25334304318326,5.40585602606554,-18.945)) ;
#138598=CARTESIAN_POINT('',(7.36677829147199,4.5782099492339,-18.945)) ;
#138599=CARTESIAN_POINT('',(7.27599715910381,4.6,-18.945)) ;
#138600=CARTESIAN_POINT('Origin',(7.27599715910381,4.4,-18.945)) ;
#138601=CARTESIAN_POINT('',(4.05,4.6,-18.945)) ;
#138602=CARTESIAN_POINT('',(3.95,4.6,-18.945)) ;
#138603=CARTESIAN_POINT('',(4.05,5.88396692803319,-18.945)) ;
#138604=CARTESIAN_POINT('',(4.05,6.,-18.945)) ;
#138605=CARTESIAN_POINT('',(7.25334304318326,5.40585602606554,-18.945)) ;
#138606=CARTESIAN_POINT('',(7.25334304318326,5.40585602606554,-18.945)) ;
#138607=CARTESIAN_POINT('',(8.6,4.09462794777298,-18.945)) ;
#138608=CARTESIAN_POINT('',(8.6,4.09462794777298,-18.945)) ;
#138609=CARTESIAN_POINT('',(8.6,3.95,-18.945)) ;
#138610=CARTESIAN_POINT('',(8.6,3.95,-18.945)) ;
#138611=CARTESIAN_POINT('',(7.36677829147199,4.5782099492339,-18.945)) ;
#138612=CARTESIAN_POINT('Origin',(7.25334304318326,5.40585602606554,-17.445)) ;
#138613=CARTESIAN_POINT('',(8.6,4.09462794777298,-17.445)) ;
#138614=CARTESIAN_POINT('',(7.25334304318326,5.40585602606554,-17.445)) ;
#138615=CARTESIAN_POINT('',(7.25334304318326,5.40585602606554,-17.445)) ;
#138616=CARTESIAN_POINT('',(4.05,5.88396692803319,-17.445)) ;
#138617=CARTESIAN_POINT('',(7.25334304318326,5.40585602606554,-17.445)) ;
#138618=CARTESIAN_POINT('',(4.05,4.6,-17.445)) ;
#138619=CARTESIAN_POINT('',(4.05,5.40585602606554,-17.445)) ;
#138620=CARTESIAN_POINT('',(7.27599715910381,4.6,-17.445)) ;
#138621=CARTESIAN_POINT('',(7.25334304318326,4.6,-17.445)) ;
#138622=CARTESIAN_POINT('',(7.36677829147199,4.5782099492339,-17.445)) ;
#138623=CARTESIAN_POINT('Origin',(7.27599715910381,4.4,-17.445)) ;
#138624=CARTESIAN_POINT('',(8.6,3.95,-17.445)) ;
#138625=CARTESIAN_POINT('',(6.94197060168454,4.79460933256464,-17.445)) ;
#138626=CARTESIAN_POINT('',(8.6,5.40585602606554,-17.445)) ;
#138627=CARTESIAN_POINT('Origin',(4.5,-2.3,-12.7)) ;
#138628=CARTESIAN_POINT('',(4.6,-2.3,-12.7)) ;
#138629=CARTESIAN_POINT('',(12.7,-2.3,-12.7)) ;
#138630=CARTESIAN_POINT('',(4.5,-2.3,-12.7)) ;
#138631=CARTESIAN_POINT('',(4.6,-2.3,-13.2778583129651)) ;
#138632=CARTESIAN_POINT('',(4.6,-2.3,-13.3138639715742)) ;
#138633=CARTESIAN_POINT('',(12.7,-2.3,-13.2778583129651)) ;
#138634=CARTESIAN_POINT('',(4.5,-2.3,-13.2778583129651)) ;
#138635=CARTESIAN_POINT('',(12.7,-2.3,-12.7)) ;
#138636=CARTESIAN_POINT('Origin',(0.,9.95,-15.24)) ;
#138637=CARTESIAN_POINT('',(0.230887397576971,9.95,-17.1548605718538)) ;
#138638=CARTESIAN_POINT('Origin',(12.8,2.75,-12.7)) ;
#138639=CARTESIAN_POINT('',(4.55912712210513,2.75,-13.7469539578284)) ;
#138640=CARTESIAN_POINT('',(12.8,2.75,-13.7469539578284)) ;
#138641=CARTESIAN_POINT('',(4.55912712210514,2.75,-12.7)) ;
#138642=CARTESIAN_POINT('',(4.55912712210514,2.75,-12.7)) ;
#138643=CARTESIAN_POINT('',(12.7,2.75,-12.7)) ;
#138644=CARTESIAN_POINT('',(12.8,2.75,-12.7)) ;
#138645=CARTESIAN_POINT('',(12.7,2.75,-12.7)) ;
#138646=CARTESIAN_POINT('Origin',(4.5,-2.8,-12.7)) ;
#138647=CARTESIAN_POINT('',(4.5,-2.7,-12.7)) ;
#138648=CARTESIAN_POINT('',(4.5,-2.4,-12.7)) ;
#138649=CARTESIAN_POINT('',(4.5,-2.8,-12.7)) ;
#138650=CARTESIAN_POINT('',(4.5,-2.7,-13.7168453788272)) ;
#138651=CARTESIAN_POINT('',(4.5,-2.7,-12.7)) ;
#138652=CARTESIAN_POINT('',(4.5,-2.4,-13.2778583129651)) ;
#138653=CARTESIAN_POINT('Origin',(4.5,0.,-15.24)) ;
#138654=CARTESIAN_POINT('',(4.5,-2.4,-12.7)) ;
#138655=CARTESIAN_POINT('Origin',(0.,0.,-12.7)) ;
#138656=CARTESIAN_POINT('Origin',(4.4,-2.7,-12.7)) ;
#138657=CARTESIAN_POINT('Origin',(4.6,-2.4,-12.7)) ;
#138658=CARTESIAN_POINT('Origin',(12.7,-2.2,-12.7)) ;
#138659=CARTESIAN_POINT('Origin',(12.7,2.65,-12.7)) ;
#138660=CARTESIAN_POINT('Origin',(4.55912712210514,2.85,-12.7)) ;
#138661=CARTESIAN_POINT('Origin',(-4.65,1.95,-17.24)) ;
#138662=CARTESIAN_POINT('',(-4.66204490261456,3.21928058320648,-17.24)) ;
#138663=CARTESIAN_POINT('',(-5.3,3.9369800677651,-17.24)) ;
#138664=CARTESIAN_POINT('',(-5.47474093186837,4.13356361611701,-17.24)) ;
#138665=CARTESIAN_POINT('',(-5.3,-1.88819660112501,-17.24)) ;
#138666=CARTESIAN_POINT('',(-5.3,-2.05,-17.24)) ;
#138667=CARTESIAN_POINT('',(-4.66204490261456,-1.5692190524323,-17.24)) ;
#138668=CARTESIAN_POINT('',(-4.69472135955,-1.58555728090001,-17.24)) ;
#138669=CARTESIAN_POINT('',(-4.66204490261456,3.35625,-17.24)) ;
#138670=CARTESIAN_POINT('Origin',(-5.4,1.95,-13.24)) ;
#138671=CARTESIAN_POINT('',(-4.66204490261456,-1.5692190524323,-13.24)) ;
#138672=CARTESIAN_POINT('',(-5.3,-1.88819660112502,-13.24)) ;
#138673=CARTESIAN_POINT('',(-5.44472135955,-1.96055728090001,-13.24)) ;
#138674=CARTESIAN_POINT('',(-5.3,3.9369800677651,-13.24)) ;
#138675=CARTESIAN_POINT('',(-5.3,4.20000000000001,-13.24)) ;
#138676=CARTESIAN_POINT('',(-4.66204490261456,3.21928058320648,-13.24)) ;
#138677=CARTESIAN_POINT('',(-4.72474093186837,3.28981361611701,-13.24)) ;
#138678=CARTESIAN_POINT('',(-4.66204490261456,-1.67500000000001,-13.24)) ;
#138679=CARTESIAN_POINT('Origin',(-4.65,1.95,-13.24)) ;
#138680=CARTESIAN_POINT('',(-3.33134808452128,1.85,-13.5623371348948)) ;
#138681=CARTESIAN_POINT('',(-3.48082994825801,1.91712723223402,-13.5257971237592)) ;
#138682=CARTESIAN_POINT('Origin',(-3.34328863644877,2.0234124498231,-13.5594183333125)) ;
#138683=CARTESIAN_POINT('',(-2.4,1.85,-13.79)) ;
#138684=CARTESIAN_POINT('',(-4.65,1.85,-13.24)) ;
#138685=CARTESIAN_POINT('',(-2.4,-0.95,-13.79)) ;
#138686=CARTESIAN_POINT('',(-2.4,1.95,-13.79)) ;
#138687=CARTESIAN_POINT('',(-3.3526478932023,-0.95,-13.557130514995)) ;
#138688=CARTESIAN_POINT('',(-3.39999999999998,-0.95,-13.5455555555556)) ;
#138689=CARTESIAN_POINT('',(-3.44209061230229,-0.971114561800017,-13.535266739215)) ;
#138690=CARTESIAN_POINT('Origin',(-3.36201220558139,-1.11033257691422,-13.554841460858)) ;
#138691=CARTESIAN_POINT('',(-4.63829959356686,-1.5692190524323,-13.2428600993503)) ;
#138692=CARTESIAN_POINT('',(-4.68814869588294,-1.59414360359034,-13.2306747632286)) ;
#138693=CARTESIAN_POINT('',(-4.63829959356686,3.21928058320648,-13.2428600993503)) ;
#138694=CARTESIAN_POINT('',(-4.63829959356686,3.35625,-13.2428600993503)) ;
#138695=CARTESIAN_POINT('',(-3.45989661114215,1.89357722797868,-13.5309141617208)) ;
#138696=CARTESIAN_POINT('Origin',(-2.4,1.95,-13.79)) ;
#138697=CARTESIAN_POINT('',(-2.4,1.85,-16.69)) ;
#138698=CARTESIAN_POINT('',(-2.4,-0.95,-16.69)) ;
#138699=CARTESIAN_POINT('',(-2.4,1.95,-16.69)) ;
#138700=CARTESIAN_POINT('',(-2.4,-1.05,-16.587055690472)) ;
#138701=CARTESIAN_POINT('Origin',(-2.4,-0.949999999999943,-16.5870556904719)) ;
#138702=CARTESIAN_POINT('',(-2.4,-1.05,-13.892944309528)) ;
#138703=CARTESIAN_POINT('',(-2.4,-1.05,-13.79)) ;
#138704=CARTESIAN_POINT('Origin',(-2.4,-0.949999999999926,-13.8929443095281)) ;
#138705=CARTESIAN_POINT('',(-2.4,1.95,-13.892944309528)) ;
#138706=CARTESIAN_POINT('Origin',(-2.4,1.85000000000001,-13.892944309528)) ;
#138707=CARTESIAN_POINT('',(-2.4,1.95,-16.587055690472)) ;
#138708=CARTESIAN_POINT('',(-2.4,1.95,-13.79)) ;
#138709=CARTESIAN_POINT('Origin',(-2.4,1.85000000000016,-16.5870556904722)) ;
#138710=CARTESIAN_POINT('Origin',(-2.4,1.95,-16.69)) ;
#138711=CARTESIAN_POINT('',(-3.3526478932023,-0.95,-16.922869485005)) ;
#138712=CARTESIAN_POINT('',(-3.44209061230229,-0.971114561800017,-16.944733260785)) ;
#138713=CARTESIAN_POINT('Origin',(-3.36201220558205,-1.1103325769103,-16.9251585391424)) ;
#138714=CARTESIAN_POINT('',(-2.4,-0.95,-16.69)) ;
#138715=CARTESIAN_POINT('',(-3.33134808452128,1.85,-16.9176628651052)) ;
#138716=CARTESIAN_POINT('',(-2.4,1.85,-16.69)) ;
#138717=CARTESIAN_POINT('',(-3.48082994825801,1.91712723223402,-16.9542028762408)) ;
#138718=CARTESIAN_POINT('Origin',(-3.3432886364489,2.02341244982209,-16.9205816666875)) ;
#138719=CARTESIAN_POINT('',(-4.63829959356686,3.21928058320648,-17.2371399006497)) ;
#138720=CARTESIAN_POINT('',(-4.70989661114216,3.29982722797869,-17.2546413938348)) ;
#138721=CARTESIAN_POINT('',(-4.63829959356686,-1.5692190524323,-17.2371399006497)) ;
#138722=CARTESIAN_POINT('',(-4.63829959356686,-1.67500000000001,-17.2371399006497)) ;
#138723=CARTESIAN_POINT('',(-3.43814869588292,-0.969143603590331,-16.9437696812158)) ;
#138724=CARTESIAN_POINT('Origin',(0.,1.95,-15.24)) ;
#138725=CARTESIAN_POINT('',(-3.35509339356897,1.95,-13.6594770355445)) ;
#138726=CARTESIAN_POINT('',(0.175392621986784,1.95,-14.5224847282359)) ;
#138727=CARTESIAN_POINT('',(-3.35509339356897,1.95,-16.8205229644555)) ;
#138728=CARTESIAN_POINT('',(-3.35509339356897,1.95,-16.9344444444444)) ;
#138729=CARTESIAN_POINT('',(0.175392621986784,1.95,-15.9575152717641)) ;
#138730=CARTESIAN_POINT('Origin',(0.,-1.05,-15.24)) ;
#138731=CARTESIAN_POINT('',(-3.37639320225,-1.05,-16.8257295843553)) ;
#138732=CARTESIAN_POINT('',(-3.42374530904768,-1.05,-16.8373045437948)) ;
#138733=CARTESIAN_POINT('',(-3.37639320225,-1.05,-13.6542704156447)) ;
#138734=CARTESIAN_POINT('',(-3.37639320225,-1.05,-15.24)) ;
#138735=CARTESIAN_POINT('',(-2.4237453090477,-1.05,-13.8871399006497)) ;
#138736=CARTESIAN_POINT('Origin',(-3.39999999999998,-1.05,-15.24)) ;
#138737=CARTESIAN_POINT('',(-3.4211145618,-1.06055728090001,-13.6324066398647)) ;
#138738=CARTESIAN_POINT('',(-3.4211145618,-1.06055728090001,-16.8475933601353)) ;
#138739=CARTESIAN_POINT('',(-3.4211145618,-1.06055728090001,-15.24)) ;
#138740=CARTESIAN_POINT('',(-4.61732354306457,-1.65866177153229,-17.14)) ;
#138741=CARTESIAN_POINT('',(-4.66717264538064,-1.68358632269033,-17.1521853361217)) ;
#138742=CARTESIAN_POINT('',(-5.34472135954999,-2.022360679775,-17.14)) ;
#138743=CARTESIAN_POINT('',(-5.4,-2.05,-17.14)) ;
#138744=CARTESIAN_POINT('',(-5.34472135954999,-2.022360679775,-13.34)) ;
#138745=CARTESIAN_POINT('',(-5.34472135954999,-2.022360679775,-13.24)) ;
#138746=CARTESIAN_POINT('',(-4.61732354306457,-1.65866177153229,-13.34)) ;
#138747=CARTESIAN_POINT('',(-4.65,-1.67500000000001,-13.34)) ;
#138748=CARTESIAN_POINT('',(-3.41717264538063,-1.05858632269032,-13.6333702194339)) ;
#138749=CARTESIAN_POINT('Origin',(-5.4,4.20000000000001,-12.7)) ;
#138750=CARTESIAN_POINT('',(-5.37474093186837,4.17158354835192,-13.34)) ;
#138751=CARTESIAN_POINT('',(-5.37474093186837,4.17158354835192,-17.14)) ;
#138752=CARTESIAN_POINT('',(-5.37474093186837,4.17158354835192,-17.24)) ;
#138753=CARTESIAN_POINT('',(-4.58730397074619,3.28571696708947,-17.14)) ;
#138754=CARTESIAN_POINT('',(-4.65,3.35625,-17.14)) ;
#138755=CARTESIAN_POINT('',(-3.42983432543734,1.98356361611701,-16.8570629755912)) ;
#138756=CARTESIAN_POINT('',(-3.40890098832149,1.96001361186167,-16.8519459376295)) ;
#138757=CARTESIAN_POINT('',(-3.42983432543734,1.98356361611701,-13.6229370244088)) ;
#138758=CARTESIAN_POINT('',(-3.42983432543734,1.98356361611701,-13.5455555555556)) ;
#138759=CARTESIAN_POINT('',(-4.58730397074619,3.28571696708947,-13.34)) ;
#138760=CARTESIAN_POINT('',(-4.65890098832149,3.36626361186168,-13.3224985068149)) ;
#138761=CARTESIAN_POINT('',(-5.4,4.20000000000001,-13.34)) ;
#138762=CARTESIAN_POINT('Origin',(-3.15,-3.9,-14.24)) ;
#138763=CARTESIAN_POINT('',(-3.15,-3.95,-14.34)) ;
#138764=CARTESIAN_POINT('',(-3.15,-3.85,-14.34)) ;
#138765=CARTESIAN_POINT('',(-3.15,-3.75,-14.34)) ;
#138766=CARTESIAN_POINT('',(-3.15,-3.85,-16.14)) ;
#138767=CARTESIAN_POINT('',(-3.15,-3.85,-14.24)) ;
#138768=CARTESIAN_POINT('',(-3.15,-3.95,-16.14)) ;
#138769=CARTESIAN_POINT('',(-3.15,-4.05,-16.14)) ;
#138770=CARTESIAN_POINT('',(-3.15,-3.95,-14.24)) ;
#138771=CARTESIAN_POINT('Origin',(-4.4,-3.9,-16.24)) ;
#138772=CARTESIAN_POINT('',(-3.25,-3.85,-16.24)) ;
#138773=CARTESIAN_POINT('',(-4.3,-3.85,-16.24)) ;
#138774=CARTESIAN_POINT('',(-4.4,-3.85,-16.24)) ;
#138775=CARTESIAN_POINT('',(-4.3,-3.95,-16.24)) ;
#138776=CARTESIAN_POINT('',(-4.3,-4.05,-16.24)) ;
#138777=CARTESIAN_POINT('',(-3.25,-3.95,-16.24)) ;
#138778=CARTESIAN_POINT('',(-4.4,-3.95,-16.24)) ;
#138779=CARTESIAN_POINT('',(-3.25,-3.75,-16.24)) ;
#138780=CARTESIAN_POINT('Origin',(-4.4,-3.9,-14.24)) ;
#138781=CARTESIAN_POINT('',(-4.4,-3.85,-16.14)) ;
#138782=CARTESIAN_POINT('',(-4.4,-3.85,-14.34)) ;
#138783=CARTESIAN_POINT('',(-4.4,-3.85,-14.24)) ;
#138784=CARTESIAN_POINT('',(-4.4,-3.95,-14.34)) ;
#138785=CARTESIAN_POINT('',(-4.4,-4.05,-14.34)) ;
#138786=CARTESIAN_POINT('',(-4.4,-3.95,-16.14)) ;
#138787=CARTESIAN_POINT('',(-4.4,-3.95,-14.24)) ;
#138788=CARTESIAN_POINT('',(-4.4,-3.75,-16.14)) ;
#138789=CARTESIAN_POINT('Origin',(-4.4,-3.9,-14.24)) ;
#138790=CARTESIAN_POINT('',(-4.3,-3.95,-14.24)) ;
#138791=CARTESIAN_POINT('',(-4.3,-3.85,-14.24)) ;
#138792=CARTESIAN_POINT('',(-4.3,-3.75,-14.24)) ;
#138793=CARTESIAN_POINT('',(-3.25,-3.85,-14.24)) ;
#138794=CARTESIAN_POINT('',(-4.4,-3.85,-14.24)) ;
#138795=CARTESIAN_POINT('',(-3.25,-3.95,-14.24)) ;
#138796=CARTESIAN_POINT('',(-3.25,-4.05,-14.24)) ;
#138797=CARTESIAN_POINT('',(-4.4,-3.95,-14.24)) ;
#138798=CARTESIAN_POINT('Origin',(0.,-3.75,-15.24)) ;
#138799=CARTESIAN_POINT('',(-3.25,-3.75,-14.34)) ;
#138800=CARTESIAN_POINT('',(-4.3,-3.75,-14.34)) ;
#138801=CARTESIAN_POINT('',(-1.56125112837913E-16,-3.75,-14.34)) ;
#138802=CARTESIAN_POINT('',(-4.3,-3.75,-16.14)) ;
#138803=CARTESIAN_POINT('',(-4.3,-3.75,-15.24)) ;
#138804=CARTESIAN_POINT('',(-3.25,-3.75,-16.14)) ;
#138805=CARTESIAN_POINT('',(-1.56125112837913E-16,-3.75,-16.14)) ;
#138806=CARTESIAN_POINT('',(-3.25,-3.75,-15.24)) ;
#138807=CARTESIAN_POINT('',(-4.15,-3.75,-16.09)) ;
#138808=CARTESIAN_POINT('',(-3.4,-3.75,-16.09)) ;
#138809=CARTESIAN_POINT('',(-4.15,-3.75,-16.09)) ;
#138810=CARTESIAN_POINT('',(-4.25,-3.75,-15.99)) ;
#138811=CARTESIAN_POINT('Origin',(-4.15,-3.75,-15.99)) ;
#138812=CARTESIAN_POINT('',(-4.25,-3.75,-14.49)) ;
#138813=CARTESIAN_POINT('',(-4.25,-3.75,-14.49)) ;
#138814=CARTESIAN_POINT('',(-4.15,-3.75,-14.39)) ;
#138815=CARTESIAN_POINT('Origin',(-4.15,-3.75,-14.49)) ;
#138816=CARTESIAN_POINT('',(-3.4,-3.75,-14.39)) ;
#138817=CARTESIAN_POINT('',(-3.4,-3.75,-14.39)) ;
#138818=CARTESIAN_POINT('',(-3.3,-3.75,-14.49)) ;
#138819=CARTESIAN_POINT('Origin',(-3.4,-3.75,-14.49)) ;
#138820=CARTESIAN_POINT('',(-3.3,-3.75,-15.99)) ;
#138821=CARTESIAN_POINT('',(-3.3,-3.75,-15.99)) ;
#138822=CARTESIAN_POINT('Origin',(-3.4,-3.75,-15.99)) ;
#138823=CARTESIAN_POINT('Origin',(-3.4,-3.75,-15.99)) ;
#138824=CARTESIAN_POINT('',(-3.4,-3.9,-16.09)) ;
#138825=CARTESIAN_POINT('',(-3.3,-3.9,-15.99)) ;
#138826=CARTESIAN_POINT('Origin',(-3.4,-3.9,-15.99)) ;
#138827=CARTESIAN_POINT('',(-3.4,-3.75,-16.09)) ;
#138828=CARTESIAN_POINT('',(-3.3,-3.75,-15.99)) ;
#138829=CARTESIAN_POINT('Origin',(-4.15,-3.75,-16.09)) ;
#138830=CARTESIAN_POINT('',(-4.15,-3.9,-16.09)) ;
#138831=CARTESIAN_POINT('',(-4.15,-3.9,-16.09)) ;
#138832=CARTESIAN_POINT('',(-4.15,-3.75,-16.09)) ;
#138833=CARTESIAN_POINT('Origin',(-4.15,-3.75,-15.99)) ;
#138834=CARTESIAN_POINT('',(-4.25,-3.9,-15.99)) ;
#138835=CARTESIAN_POINT('Origin',(-4.15,-3.9,-15.99)) ;
#138836=CARTESIAN_POINT('',(-4.25,-3.75,-15.99)) ;
#138837=CARTESIAN_POINT('Origin',(-4.25,-3.75,-14.49)) ;
#138838=CARTESIAN_POINT('',(-4.25,-3.9,-14.49)) ;
#138839=CARTESIAN_POINT('',(-4.25,-3.9,-14.49)) ;
#138840=CARTESIAN_POINT('',(-4.25,-3.75,-14.49)) ;
#138841=CARTESIAN_POINT('Origin',(-4.15,-3.75,-14.49)) ;
#138842=CARTESIAN_POINT('',(-4.15,-3.9,-14.39)) ;
#138843=CARTESIAN_POINT('Origin',(-4.15,-3.9,-14.49)) ;
#138844=CARTESIAN_POINT('',(-4.15,-3.75,-14.39)) ;
#138845=CARTESIAN_POINT('Origin',(-3.4,-3.75,-14.39)) ;
#138846=CARTESIAN_POINT('',(-3.4,-3.9,-14.39)) ;
#138847=CARTESIAN_POINT('',(-3.4,-3.9,-14.39)) ;
#138848=CARTESIAN_POINT('',(-3.4,-3.75,-14.39)) ;
#138849=CARTESIAN_POINT('Origin',(-3.4,-3.75,-14.49)) ;
#138850=CARTESIAN_POINT('',(-3.3,-3.9,-14.49)) ;
#138851=CARTESIAN_POINT('Origin',(-3.4,-3.9,-14.49)) ;
#138852=CARTESIAN_POINT('',(-3.3,-3.75,-14.49)) ;
#138853=CARTESIAN_POINT('Origin',(-3.3,-3.75,-15.99)) ;
#138854=CARTESIAN_POINT('',(-3.3,-3.9,-15.99)) ;
#138855=CARTESIAN_POINT('Origin',(0.,-3.9,-15.24)) ;
#138856=CARTESIAN_POINT('Origin',(0.,9.95,-15.24)) ;
#138857=CARTESIAN_POINT('',(-0.230887397576972,9.95,-13.3251394281462)) ;
#138858=CARTESIAN_POINT('Origin',(-0.321518176280637,8.95,-13.3674012543203)) ;
#138859=CARTESIAN_POINT('',(-0.321518176280637,9.05,-13.3674012543203)) ;
#138860=CARTESIAN_POINT('',(1.22782596331729,9.85,-16.689980483939)) ;
#138861=CARTESIAN_POINT('Origin',(-1.22782596331729,8.95,-13.790019516061)) ;
#138862=CARTESIAN_POINT('',(-1.22782596331729,9.05,-13.790019516061)) ;
#138863=CARTESIAN_POINT('',(-1.22782596331729,9.85,-13.790019516061)) ;
#138864=CARTESIAN_POINT('Origin',(0.,8.95,-15.24)) ;
#138865=CARTESIAN_POINT('',(-0.362523114814661,8.95,-15.4090473046963)) ;
#138866=CARTESIAN_POINT('',(0.36252311481466,8.95,-15.0709526953037)) ;
#138867=CARTESIAN_POINT('Origin',(-2.65,10.8,-16.24)) ;
#138868=CARTESIAN_POINT('',(-2.65,10.75,-16.14)) ;
#138869=CARTESIAN_POINT('',(-2.65,10.75,-14.34)) ;
#138870=CARTESIAN_POINT('',(-2.65,10.75,-16.24)) ;
#138871=CARTESIAN_POINT('',(-2.65,10.85,-14.34)) ;
#138872=CARTESIAN_POINT('',(-2.65,10.95,-14.34)) ;
#138873=CARTESIAN_POINT('',(-2.65,10.85,-16.14)) ;
#138874=CARTESIAN_POINT('',(-2.65,10.85,-16.24)) ;
#138875=CARTESIAN_POINT('',(-2.65,10.65,-16.14)) ;
#138876=CARTESIAN_POINT('Origin',(-3.9,10.8,-14.24)) ;
#138877=CARTESIAN_POINT('',(-2.75,10.85,-14.24)) ;
#138878=CARTESIAN_POINT('',(-2.75,10.75,-14.24)) ;
#138879=CARTESIAN_POINT('',(-2.75,10.65,-14.24)) ;
#138880=CARTESIAN_POINT('',(-3.8,10.75,-14.24)) ;
#138881=CARTESIAN_POINT('',(-3.9,10.75,-14.24)) ;
#138882=CARTESIAN_POINT('',(-3.8,10.85,-14.24)) ;
#138883=CARTESIAN_POINT('',(-3.8,10.95,-14.24)) ;
#138884=CARTESIAN_POINT('',(-3.9,10.85,-14.24)) ;
#138885=CARTESIAN_POINT('Origin',(-3.9,10.8,-16.24)) ;
#138886=CARTESIAN_POINT('',(-3.9,10.85,-14.34)) ;
#138887=CARTESIAN_POINT('',(-3.9,10.75,-14.34)) ;
#138888=CARTESIAN_POINT('',(-3.9,10.65,-14.34)) ;
#138889=CARTESIAN_POINT('',(-3.9,10.75,-16.14)) ;
#138890=CARTESIAN_POINT('',(-3.9,10.75,-16.24)) ;
#138891=CARTESIAN_POINT('',(-3.9,10.85,-16.14)) ;
#138892=CARTESIAN_POINT('',(-3.9,10.95,-16.14)) ;
#138893=CARTESIAN_POINT('',(-3.9,10.85,-16.24)) ;
#138894=CARTESIAN_POINT('Origin',(-3.9,10.8,-16.24)) ;
#138895=CARTESIAN_POINT('',(-3.8,10.75,-16.24)) ;
#138896=CARTESIAN_POINT('',(-2.75,10.75,-16.24)) ;
#138897=CARTESIAN_POINT('',(-3.9,10.75,-16.24)) ;
#138898=CARTESIAN_POINT('',(-2.75,10.85,-16.24)) ;
#138899=CARTESIAN_POINT('',(-2.75,10.95,-16.24)) ;
#138900=CARTESIAN_POINT('',(-3.8,10.85,-16.24)) ;
#138901=CARTESIAN_POINT('',(-3.9,10.85,-16.24)) ;
#138902=CARTESIAN_POINT('',(-3.8,10.65,-16.24)) ;
#138903=CARTESIAN_POINT('Origin',(0.,10.65,-15.24)) ;
#138904=CARTESIAN_POINT('',(-3.8,10.65,-14.34)) ;
#138905=CARTESIAN_POINT('',(-2.75,10.65,-14.34)) ;
#138906=CARTESIAN_POINT('',(1.56125112837912E-16,10.65,-14.34)) ;
#138907=CARTESIAN_POINT('',(-2.75,10.65,-16.14)) ;
#138908=CARTESIAN_POINT('',(-2.75,10.65,-15.24)) ;
#138909=CARTESIAN_POINT('',(-3.8,10.65,-16.14)) ;
#138910=CARTESIAN_POINT('',(-1.56125112837913E-16,10.65,-16.14)) ;
#138911=CARTESIAN_POINT('',(-3.8,10.65,-15.24)) ;
#138912=CARTESIAN_POINT('',(-3.65,10.65,-14.39)) ;
#138913=CARTESIAN_POINT('',(-2.9,10.65,-14.39)) ;
#138914=CARTESIAN_POINT('',(-3.65,10.65,-14.39)) ;
#138915=CARTESIAN_POINT('',(-3.75,10.65,-14.49)) ;
#138916=CARTESIAN_POINT('Origin',(-3.65,10.65,-14.49)) ;
#138917=CARTESIAN_POINT('',(-3.75,10.65,-15.99)) ;
#138918=CARTESIAN_POINT('',(-3.75,10.65,-15.99)) ;
#138919=CARTESIAN_POINT('',(-3.65,10.65,-16.09)) ;
#138920=CARTESIAN_POINT('Origin',(-3.65,10.65,-15.99)) ;
#138921=CARTESIAN_POINT('',(-2.9,10.65,-16.09)) ;
#138922=CARTESIAN_POINT('',(-2.9,10.65,-16.09)) ;
#138923=CARTESIAN_POINT('',(-2.8,10.65,-15.99)) ;
#138924=CARTESIAN_POINT('Origin',(-2.9,10.65,-15.99)) ;
#138925=CARTESIAN_POINT('',(-2.8,10.65,-14.49)) ;
#138926=CARTESIAN_POINT('',(-2.8,10.65,-14.49)) ;
#138927=CARTESIAN_POINT('Origin',(-2.9,10.65,-14.49)) ;
#138928=CARTESIAN_POINT('Origin',(-2.9,10.65,-14.49)) ;
#138929=CARTESIAN_POINT('',(-2.8,10.7,-14.49)) ;
#138930=CARTESIAN_POINT('',(-2.8,10.65,-14.49)) ;
#138931=CARTESIAN_POINT('',(-2.9,10.7,-14.39)) ;
#138932=CARTESIAN_POINT('Origin',(-2.9,10.7,-14.49)) ;
#138933=CARTESIAN_POINT('',(-2.9,10.65,-14.39)) ;
#138934=CARTESIAN_POINT('Origin',(-3.65,10.65,-14.39)) ;
#138935=CARTESIAN_POINT('',(-3.65,10.7,-14.39)) ;
#138936=CARTESIAN_POINT('',(-3.65,10.7,-14.39)) ;
#138937=CARTESIAN_POINT('',(-3.65,10.65,-14.39)) ;
#138938=CARTESIAN_POINT('Origin',(-3.65,10.65,-14.49)) ;
#138939=CARTESIAN_POINT('',(-3.75,10.7,-14.49)) ;
#138940=CARTESIAN_POINT('Origin',(-3.65,10.7,-14.49)) ;
#138941=CARTESIAN_POINT('',(-3.75,10.65,-14.49)) ;
#138942=CARTESIAN_POINT('Origin',(-3.75,10.65,-15.99)) ;
#138943=CARTESIAN_POINT('',(-3.75,10.7,-15.99)) ;
#138944=CARTESIAN_POINT('',(-3.75,10.7,-15.99)) ;
#138945=CARTESIAN_POINT('',(-3.75,10.65,-15.99)) ;
#138946=CARTESIAN_POINT('Origin',(-3.65,10.65,-15.99)) ;
#138947=CARTESIAN_POINT('',(-3.65,10.7,-16.09)) ;
#138948=CARTESIAN_POINT('Origin',(-3.65,10.7,-15.99)) ;
#138949=CARTESIAN_POINT('',(-3.65,10.65,-16.09)) ;
#138950=CARTESIAN_POINT('Origin',(-2.9,10.65,-16.09)) ;
#138951=CARTESIAN_POINT('',(-2.9,10.7,-16.09)) ;
#138952=CARTESIAN_POINT('',(-2.9,10.7,-16.09)) ;
#138953=CARTESIAN_POINT('',(-2.9,10.65,-16.09)) ;
#138954=CARTESIAN_POINT('Origin',(-2.9,10.65,-15.99)) ;
#138955=CARTESIAN_POINT('',(-2.8,10.7,-15.99)) ;
#138956=CARTESIAN_POINT('Origin',(-2.9,10.7,-15.99)) ;
#138957=CARTESIAN_POINT('',(-2.8,10.65,-15.99)) ;
#138958=CARTESIAN_POINT('Origin',(-2.8,10.65,-14.49)) ;
#138959=CARTESIAN_POINT('',(-2.8,10.7,-14.49)) ;
#138960=CARTESIAN_POINT('Origin',(0.,10.8,-15.24)) ;
#138961=CARTESIAN_POINT('',(-3.65,10.8,-14.49)) ;
#138962=CARTESIAN_POINT('',(-2.9,10.8,-14.49)) ;
#138963=CARTESIAN_POINT('',(0.,10.8,-14.49)) ;
#138964=CARTESIAN_POINT('',(-2.9,10.8,-15.99)) ;
#138965=CARTESIAN_POINT('',(-2.9,10.8,-15.24)) ;
#138966=CARTESIAN_POINT('',(-3.65,10.8,-15.99)) ;
#138967=CARTESIAN_POINT('',(0.,10.8,-15.99)) ;
#138968=CARTESIAN_POINT('',(-3.65,10.8,-15.24)) ;
#138969=CARTESIAN_POINT('Origin',(4.5,2.75,-16.615)) ;
#138970=CARTESIAN_POINT('',(4.5,2.63356010126946,-16.6344066497884)) ;
#138971=CARTESIAN_POINT('',(4.6,2.11643989873054,-16.7205933502116)) ;
#138972=CARTESIAN_POINT('',(4.6,2.11643989873054,-16.7205933502116)) ;
#138973=CARTESIAN_POINT('',(12.7,2.11643989873054,-16.7205933502116)) ;
#138974=CARTESIAN_POINT('',(12.8,2.11643989873054,-16.7205933502116)) ;
#138975=CARTESIAN_POINT('',(12.7,2.75,-16.615)) ;
#138976=CARTESIAN_POINT('Origin',(4.5,2.,-16.74)) ;
#138977=CARTESIAN_POINT('',(4.6,2.,-16.6219539578284)) ;
#138978=CARTESIAN_POINT('',(4.6,2.,-13.74)) ;
#138979=CARTESIAN_POINT('',(12.7,2.,-16.6219539578284)) ;
#138980=CARTESIAN_POINT('',(12.7,2.,-16.74)) ;
#138981=CARTESIAN_POINT('',(4.5,2.,-16.6219539578284)) ;
#138982=CARTESIAN_POINT('Origin',(4.5,2.,-13.74)) ;
#138983=CARTESIAN_POINT('',(4.6,2.63356010126946,-13.8455933502116)) ;
#138984=CARTESIAN_POINT('',(4.6,2.63356010126947,-13.8455933502116)) ;
#138985=CARTESIAN_POINT('',(4.5,2.63356010126946,-13.8455933502116)) ;
#138986=CARTESIAN_POINT('',(12.7,2.,-13.74)) ;
#138987=CARTESIAN_POINT('Origin',(4.5,0.,-15.24)) ;
#138988=CARTESIAN_POINT('',(4.5,2.72431432344521,-13.932634816645)) ;
#138989=CARTESIAN_POINT('',(4.5,2.72431432344521,-15.24)) ;
#138990=CARTESIAN_POINT('',(4.5,2.61712020253893,-13.9442327425948)) ;
#138991=CARTESIAN_POINT('Origin',(4.5,2.65,-13.7469539578284)) ;
#138992=CARTESIAN_POINT('',(4.5,2.1,-13.8580460421716)) ;
#138993=CARTESIAN_POINT('',(4.5,2.1,-13.8580460421716)) ;
#138994=CARTESIAN_POINT('',(4.5,2.1,-16.6219539578284)) ;
#138995=CARTESIAN_POINT('',(4.5,2.1,-16.74)) ;
#138996=CARTESIAN_POINT('',(4.5,2.61712020253893,-16.5357672574052)) ;
#138997=CARTESIAN_POINT('Origin',(10.3,0.,-15.24)) ;
#138998=CARTESIAN_POINT('Origin',(0.584645609909621,0.,-15.24)) ;
#138999=CARTESIAN_POINT('',(4.6,-2.32258064516129,-13.3411532060953)) ;
#139000=CARTESIAN_POINT('',(4.6,-2.79310344827574,-14.1452063540419)) ;
#139001=CARTESIAN_POINT('Origin',(4.6,0.,-15.24)) ;
#139002=CARTESIAN_POINT('',(4.6,-2.79310344827574,-16.3347936459581)) ;
#139003=CARTESIAN_POINT('Origin',(4.6,0.,-15.24)) ;
#139004=CARTESIAN_POINT('',(4.6,-2.32258064516129,-17.1388467939047)) ;
#139005=CARTESIAN_POINT('Origin',(4.6,0.,-15.24)) ;
#139006=CARTESIAN_POINT('',(12.7,-2.32258064516129,-17.1388467939047)) ;
#139007=CARTESIAN_POINT('',(0.584645609909621,-2.32258064516129,-17.1388467939047)) ;
#139008=CARTESIAN_POINT('',(12.7,-2.32258064516129,-13.3411532060953)) ;
#139009=CARTESIAN_POINT('Origin',(12.7,0.,-15.24)) ;
#139010=CARTESIAN_POINT('',(0.584645609909621,-2.32258064516129,-13.3411532060953)) ;
#139011=CARTESIAN_POINT('Ctrl Pts',(-5.37474093186837,4.17158354835192,
-13.34)) ;
#139012=CARTESIAN_POINT('Ctrl Pts',(-5.4,4.2,-13.34)) ;
#139013=CARTESIAN_POINT('Ctrl Pts',(-5.4,4.23801993223491,-13.34)) ;
#139014=CARTESIAN_POINT('Ctrl Pts',(-5.37474093064202,4.17158354697228,
-13.313746564061)) ;
#139015=CARTESIAN_POINT('Ctrl Pts',(-5.4,4.19999999724801,-13.302481412799)) ;
#139016=CARTESIAN_POINT('Ctrl Pts',(-5.4,4.23801992976516,-13.2874931280902)) ;
#139017=CARTESIAN_POINT('Ctrl Pts',(-5.36668583490655,4.14629949399955,
-13.2878012868841)) ;
#139018=CARTESIAN_POINT('Ctrl Pts',(-5.40000000000003,4.16739198385627,
-13.2646678350658)) ;
#139019=CARTESIAN_POINT('Ctrl Pts',(-5.4,4.20557579169425,-13.2356025737683)) ;
#139020=CARTESIAN_POINT('Ctrl Pts',(-5.3390138046061,4.05944006555646,-13.2507773568786)) ;
#139021=CARTESIAN_POINT('Ctrl Pts',(-5.39999999999997,4.06625640449636,
-13.2231326366142)) ;
#139022=CARTESIAN_POINT('Ctrl Pts',(-5.4,4.09411900298411,-13.1615547137571)) ;
#139023=CARTESIAN_POINT('Ctrl Pts',(-5.31962206268973,3.99857154231912,
-13.24)) ;
#139024=CARTESIAN_POINT('Ctrl Pts',(-5.4,3.99346933127521,-13.2220035074266)) ;
#139025=CARTESIAN_POINT('Ctrl Pts',(-5.4,4.0160133758189,-13.1400000004813)) ;
#139026=CARTESIAN_POINT('Ctrl Pts',(-5.3,3.9369800677651,-13.24)) ;
#139027=CARTESIAN_POINT('Ctrl Pts',(-5.4,3.9369800677651,-13.24)) ;
#139028=CARTESIAN_POINT('Ctrl Pts',(-5.4,3.9369800677651,-13.14)) ;
#139029=CARTESIAN_POINT('Origin',(-5.3,4.23801993223491,-13.34)) ;
#139030=CARTESIAN_POINT('Ctrl Pts',(-5.3,3.9369800677651,-13.24)) ;
#139031=CARTESIAN_POINT('Ctrl Pts',(-5.31962206268973,3.99857154231912,
-13.24)) ;
#139032=CARTESIAN_POINT('Ctrl Pts',(-5.3390138046061,4.05944006555646,-13.2507773568786)) ;
#139033=CARTESIAN_POINT('Ctrl Pts',(-5.36668583490655,4.14629949399955,
-13.2878012868841)) ;
#139034=CARTESIAN_POINT('Ctrl Pts',(-5.37474093064202,4.17158354697228,
-13.313746564061)) ;
#139035=CARTESIAN_POINT('Ctrl Pts',(-5.37474093186837,4.17158354835192,
-13.34)) ;
#139036=CARTESIAN_POINT('Origin',(-5.3,3.9369800677651,-13.14)) ;
#139037=CARTESIAN_POINT('Origin',(-4.6737453090477,1.85,-13.3371399006497)) ;
#139038=CARTESIAN_POINT('Origin',(-3.35509339356897,1.85,-13.6594770355445)) ;
#139039=CARTESIAN_POINT('Ctrl Pts',(-3.35509339356897,1.95,-13.6594770355445)) ;
#139040=CARTESIAN_POINT('Ctrl Pts',(-3.33134808452127,1.95,-13.5623371348948)) ;
#139041=CARTESIAN_POINT('Ctrl Pts',(-3.33134808452128,1.85,-13.5623371348948)) ;
#139042=CARTESIAN_POINT('Ctrl Pts',(-3.38343213690417,1.95,-13.6456225388028)) ;
#139043=CARTESIAN_POINT('Ctrl Pts',(-3.36046743872478,1.94345445676983,
-13.5552190705338)) ;
#139044=CARTESIAN_POINT('Ctrl Pts',(-3.38803897426454,1.85000000162387,
-13.5484793618464)) ;
#139045=CARTESIAN_POINT('Ctrl Pts',(-3.41101314049054,1.96238978305186,
-13.6321384929162)) ;
#139046=CARTESIAN_POINT('Ctrl Pts',(-3.39538881861726,1.95068928167318,
-13.5466827332267)) ;
#139047=CARTESIAN_POINT('Ctrl Pts',(-3.44316973238525,1.87475949194144,
-13.5350029543058)) ;
#139048=CARTESIAN_POINT('Ctrl Pts',(-3.42983432543734,1.98356361611701,
-13.6229370244088)) ;
#139049=CARTESIAN_POINT('Ctrl Pts',(-3.42093333711585,1.97355000425533,
-13.5404385175939)) ;
#139050=CARTESIAN_POINT('Ctrl Pts',(-3.48082994825801,1.91712723223402,
-13.5257971237592)) ;
#139051=CARTESIAN_POINT('Origin',(-3.50457525730571,1.91712723223402,-13.6229370244088)) ;
#139052=CARTESIAN_POINT('Origin',(-3.36128627567781,2.036213614357,-13.6564494043351)) ;
#139053=CARTESIAN_POINT('Origin',(-4.05330900605469,2.53445269957662,-13.488802108048)) ;
#139054=CARTESIAN_POINT('Origin',(-4.66204490261456,3.21928058320648,-13.34)) ;
#139055=CARTESIAN_POINT('Origin',(-4.35749955255802,2.87666706439287,-13.34)) ;
#139056=CARTESIAN_POINT('Origin',(-4.66204490261456,3.21928058320648,-13.34)) ;
#139057=CARTESIAN_POINT('Origin',(-5.3,5.2,-13.14)) ;
#139058=CARTESIAN_POINT('Origin',(-5.3,-1.88819660112502,-13.14)) ;
#139059=CARTESIAN_POINT('Origin',(-5.3,4.23801993223491,-12.7)) ;
#139060=CARTESIAN_POINT('Origin',(-5.3,4.23801993223491,-17.14)) ;
#139061=CARTESIAN_POINT('Origin',(-3.35509339356897,2.05,-15.24)) ;
#139062=CARTESIAN_POINT('Origin',(-3.36128627567723,2.03621361435801,-16.8235505956649)) ;
#139063=CARTESIAN_POINT('Origin',(-2.4237453090477,1.85,-16.5928600993503)) ;
#139064=CARTESIAN_POINT('Origin',(-3.35509339356897,1.85,-16.8205229644555)) ;
#139065=CARTESIAN_POINT('Origin',(-4.66204490261456,3.21928058320648,-13.34)) ;
#139066=CARTESIAN_POINT('Origin',(-4.66204490261456,3.21928058320648,-13.34)) ;
#139067=CARTESIAN_POINT('Ctrl Pts',(-5.29976814257747,-1.88802911972919,
-13.2399998273778)) ;
#139068=CARTESIAN_POINT('Ctrl Pts',(-5.4,-1.88802831720456,-13.240232593543)) ;
#139069=CARTESIAN_POINT('Ctrl Pts',(-5.4,-1.88791746283072,-13.1400001624624)) ;
#139070=CARTESIAN_POINT('Ctrl Pts',(-5.31153957531165,-1.92331224822998,
-13.2399864676889)) ;
#139071=CARTESIAN_POINT('Ctrl Pts',(-5.39999999999995,-1.92148676945297,
-13.2289778925381)) ;
#139072=CARTESIAN_POINT('Ctrl Pts',(-5.4,-1.94671708614657,-13.1399317130284)) ;
#139073=CARTESIAN_POINT('Ctrl Pts',(-5.32318090226696,-1.95817527052249,
-13.2507844972681)) ;
#139074=CARTESIAN_POINT('Ctrl Pts',(-5.4,-1.96527310172483,-13.2321633837528)) ;
#139075=CARTESIAN_POINT('Ctrl Pts',(-5.4,-2.00485091174287,-13.1614960748893)) ;
#139076=CARTESIAN_POINT('Ctrl Pts',(-5.33978950165955,-2.00789652656156,
-13.2878649650197)) ;
#139077=CARTESIAN_POINT('Ctrl Pts',(-5.4,-2.02908601268744,-13.2713665145317)) ;
#139078=CARTESIAN_POINT('Ctrl Pts',(-5.4,-2.08777005652399,-13.235661212636)) ;
#139079=CARTESIAN_POINT('Ctrl Pts',(-5.34461954754097,-2.02234798681676,
-13.3138461447183)) ;
#139080=CARTESIAN_POINT('Ctrl Pts',(-5.4,-2.04997459329993,-13.30567566484)) ;
#139081=CARTESIAN_POINT('Ctrl Pts',(-5.4,-2.1118797455067,-13.2876576869739)) ;
#139082=CARTESIAN_POINT('Ctrl Pts',(-5.34460423617423,-2.02230212313483,
-13.3401247518701)) ;
#139083=CARTESIAN_POINT('Ctrl Pts',(-5.4,-2.04990938338631,-13.3401637542765)) ;
#139084=CARTESIAN_POINT('Ctrl Pts',(-5.4,-2.11180321723903,-13.3402496688804)) ;
#139085=CARTESIAN_POINT('Origin',(-5.30000000000002,-1.88819660112506,-13.34)) ;
#139086=CARTESIAN_POINT('Origin',(-5.3,-2.11180339887499,-13.34)) ;
#139087=CARTESIAN_POINT('Ctrl Pts',(-5.3,3.9369800677651,-17.24)) ;
#139088=CARTESIAN_POINT('Ctrl Pts',(-5.4,3.9369800677651,-17.24)) ;
#139089=CARTESIAN_POINT('Ctrl Pts',(-5.4,3.9369800677651,-17.34)) ;
#139090=CARTESIAN_POINT('Ctrl Pts',(-5.31962206268973,3.99857154231911,
-17.24)) ;
#139091=CARTESIAN_POINT('Ctrl Pts',(-5.4,3.99346933127509,-17.2579964925735)) ;
#139092=CARTESIAN_POINT('Ctrl Pts',(-5.4,4.01601337581888,-17.3399999995189)) ;
#139093=CARTESIAN_POINT('Ctrl Pts',(-5.33901380460613,4.05944006555646,
-17.2292226431215)) ;
#139094=CARTESIAN_POINT('Ctrl Pts',(-5.4,4.06625640449645,-17.2568673633859)) ;
#139095=CARTESIAN_POINT('Ctrl Pts',(-5.4,4.09411900298413,-17.3184452862429)) ;
#139096=CARTESIAN_POINT('Ctrl Pts',(-5.36668583490652,4.14629949399955,
-17.1921987131158)) ;
#139097=CARTESIAN_POINT('Ctrl Pts',(-5.4,4.1673919838562,-17.2153321649341)) ;
#139098=CARTESIAN_POINT('Ctrl Pts',(-5.4,4.20557579169423,-17.2443974262317)) ;
#139099=CARTESIAN_POINT('Ctrl Pts',(-5.37474093064202,4.17158354697228,
-17.166253435939)) ;
#139100=CARTESIAN_POINT('Ctrl Pts',(-5.4,4.19999999724801,-17.1775185872011)) ;
#139101=CARTESIAN_POINT('Ctrl Pts',(-5.4,4.23801992976516,-17.1925068719098)) ;
#139102=CARTESIAN_POINT('Ctrl Pts',(-5.37474093186837,4.17158354835192,
-17.14)) ;
#139103=CARTESIAN_POINT('Ctrl Pts',(-5.4,4.2,-17.14)) ;
#139104=CARTESIAN_POINT('Ctrl Pts',(-5.4,4.23801993223491,-17.14)) ;
#139105=CARTESIAN_POINT('Origin',(-5.3,3.9369800677651,-17.34)) ;
#139106=CARTESIAN_POINT('Ctrl Pts',(-5.37474093186837,4.17158354835192,
-17.14)) ;
#139107=CARTESIAN_POINT('Ctrl Pts',(-5.37474093064202,4.17158354697228,
-17.166253435939)) ;
#139108=CARTESIAN_POINT('Ctrl Pts',(-5.36668583490652,4.14629949399955,
-17.1921987131158)) ;
#139109=CARTESIAN_POINT('Ctrl Pts',(-5.33901380460613,4.05944006555646,
-17.2292226431215)) ;
#139110=CARTESIAN_POINT('Ctrl Pts',(-5.31962206268973,3.99857154231911,
-17.24)) ;
#139111=CARTESIAN_POINT('Ctrl Pts',(-5.3,3.9369800677651,-17.24)) ;
#139112=CARTESIAN_POINT('Ctrl Pts',(-3.42983432543734,1.98356361611701,
-16.8570629755912)) ;
#139113=CARTESIAN_POINT('Ctrl Pts',(-3.42093333711585,1.97355000425533,
-16.9395614824061)) ;
#139114=CARTESIAN_POINT('Ctrl Pts',(-3.48082994825801,1.91712723223402,
-16.9542028762408)) ;
#139115=CARTESIAN_POINT('Ctrl Pts',(-3.41101314049054,1.96238978305186,
-16.8478615070839)) ;
#139116=CARTESIAN_POINT('Ctrl Pts',(-3.39538881861725,1.95068928167332,
-16.9333172667734)) ;
#139117=CARTESIAN_POINT('Ctrl Pts',(-3.44316973238528,1.87475949194142,
-16.9449970456942)) ;
#139118=CARTESIAN_POINT('Ctrl Pts',(-3.38343213690423,1.95,-16.8343774611971)) ;
#139119=CARTESIAN_POINT('Ctrl Pts',(-3.36046743872485,1.94345445676967,
-16.9247809294657)) ;
#139120=CARTESIAN_POINT('Ctrl Pts',(-3.38803897426452,1.85000000162387,
-16.9315206381536)) ;
#139121=CARTESIAN_POINT('Ctrl Pts',(-3.35509339356897,1.95,-16.8205229644555)) ;
#139122=CARTESIAN_POINT('Ctrl Pts',(-3.33134808452128,1.95,-16.9176628651052)) ;
#139123=CARTESIAN_POINT('Ctrl Pts',(-3.33134808452128,1.85,-16.9176628651052)) ;
#139124=CARTESIAN_POINT('Origin',(-3.50457525730571,1.91712723223402,-16.8570629755912)) ;
#139125=CARTESIAN_POINT('Origin',(-4.66204490261456,1.95,-13.34)) ;
#139126=CARTESIAN_POINT('Origin',(-4.66204490261456,-1.5692190524323,-13.34)) ;
#139127=CARTESIAN_POINT('Origin',(-3.84472135955,-1.16055728090002,-13.34)) ;
#139128=CARTESIAN_POINT('Origin',(-4.66204490261456,-1.5692190524323,-13.34)) ;
#139129=CARTESIAN_POINT('Origin',(-5.3,-2.11180339887499,-12.7)) ;
#139130=CARTESIAN_POINT('Origin',(-5.3,-2.11180339887499,-17.14)) ;
#139131=CARTESIAN_POINT('Origin',(-5.3,1.95,-17.34)) ;
#139132=CARTESIAN_POINT('Origin',(-5.3,-1.88819660112501,-17.34)) ;
#139133=CARTESIAN_POINT('Origin',(-4.0264650697994,2.50425327128942,-17.14)) ;
#139134=CARTESIAN_POINT('Origin',(-4.66204490261456,3.21928058320648,-17.14)) ;
#139135=CARTESIAN_POINT('Origin',(-3.02790825149799,1.38087685070033,-16.7405443741715)) ;
#139136=CARTESIAN_POINT('Origin',(-4.66204490261456,3.21928058320648,-17.14)) ;
#139137=CARTESIAN_POINT('Origin',(-4.66204490261456,-1.5692190524323,-13.34)) ;
#139138=CARTESIAN_POINT('Origin',(-4.66204490261456,-1.5692190524323,-13.34)) ;
#139139=CARTESIAN_POINT('Ctrl Pts',(-5.34460423617422,-2.02230212313483,
-17.1398752481299)) ;
#139140=CARTESIAN_POINT('Ctrl Pts',(-5.4,-2.04990938338631,-17.1398362457235)) ;
#139141=CARTESIAN_POINT('Ctrl Pts',(-5.4,-2.11180321723903,-17.1397503311196)) ;
#139142=CARTESIAN_POINT('Ctrl Pts',(-5.34461954754097,-2.02234798681675,
-17.1661538552817)) ;
#139143=CARTESIAN_POINT('Ctrl Pts',(-5.4,-2.04997459329993,-17.17432433516)) ;
#139144=CARTESIAN_POINT('Ctrl Pts',(-5.4,-2.1118797455067,-17.1923423130261)) ;
#139145=CARTESIAN_POINT('Ctrl Pts',(-5.33978950165956,-2.00789652656154,
-17.1921350349804)) ;
#139146=CARTESIAN_POINT('Ctrl Pts',(-5.4,-2.02908601268745,-17.2086334854683)) ;
#139147=CARTESIAN_POINT('Ctrl Pts',(-5.4,-2.087770056524,-17.244338787364)) ;
#139148=CARTESIAN_POINT('Ctrl Pts',(-5.32318090226695,-1.95817527052251,
-17.2292155027319)) ;
#139149=CARTESIAN_POINT('Ctrl Pts',(-5.4,-1.96527310172481,-17.2478366162471)) ;
#139150=CARTESIAN_POINT('Ctrl Pts',(-5.4,-2.00485091174287,-17.3185039251107)) ;
#139151=CARTESIAN_POINT('Ctrl Pts',(-5.31153957531164,-1.92331224822996,
-17.2400135323111)) ;
#139152=CARTESIAN_POINT('Ctrl Pts',(-5.4,-1.9214867694528,-17.2510221074624)) ;
#139153=CARTESIAN_POINT('Ctrl Pts',(-5.4,-1.94671708614657,-17.3400682869718)) ;
#139154=CARTESIAN_POINT('Ctrl Pts',(-5.29976814257746,-1.88802911972918,
-17.2400001726222)) ;
#139155=CARTESIAN_POINT('Ctrl Pts',(-5.4,-1.88802831720455,-17.239767406457)) ;
#139156=CARTESIAN_POINT('Ctrl Pts',(-5.4,-1.88791746283071,-17.3399998375376)) ;
#139157=CARTESIAN_POINT('Origin',(-5.30000000000006,-1.8881966011252,-17.1400000000001)) ;
#139158=CARTESIAN_POINT('Origin',(-4.66204490261456,3.21928058320648,-17.14)) ;
#139159=CARTESIAN_POINT('Origin',(-4.66204490261456,3.21928058320648,-17.14)) ;
#139160=CARTESIAN_POINT('Origin',(0.175392621986784,-0.95,-14.5224847282359)) ;
#139161=CARTESIAN_POINT('Origin',(-3.37639320225,-0.95,-13.6542704156447)) ;
#139162=CARTESIAN_POINT('Origin',(-3.32804538583365,-0.902219294041845,
-13.6660887707687)) ;
#139163=CARTESIAN_POINT('Origin',(-3.46583592134999,-0.971114561800017,
-13.6324066398647)) ;
#139164=CARTESIAN_POINT('Origin',(-3.24472135955,-0.860557280900019,-17.14)) ;
#139165=CARTESIAN_POINT('Origin',(-4.66204490261456,-1.5692190524323,-17.14)) ;
#139166=CARTESIAN_POINT('Origin',(-4.66204490261456,1.95,-17.14)) ;
#139167=CARTESIAN_POINT('Origin',(-4.66204490261456,-1.5692190524323,-17.14)) ;
#139168=CARTESIAN_POINT('Ctrl Pts',(-3.4211145618,-1.06055728090001,-13.6324066398647)) ;
#139169=CARTESIAN_POINT('Ctrl Pts',(-3.40394191641935,-1.05197095820969,
-13.5445919759864)) ;
#139170=CARTESIAN_POINT('Ctrl Pts',(-3.44209061230229,-0.971114561800017,
-13.535266739215)) ;
#139171=CARTESIAN_POINT('Ctrl Pts',(-3.40727897628737,-1.05363948814369,
-13.6391707039916)) ;
#139172=CARTESIAN_POINT('Ctrl Pts',(-3.38665319245543,-1.04670310838585,
-13.5488181085109)) ;
#139173=CARTESIAN_POINT('Ctrl Pts',(-3.4144159452097,-0.957277229261619,
-13.5420316578376)) ;
#139174=CARTESIAN_POINT('Ctrl Pts',(-3.39186274464429,-1.05,-13.6467075282519)) ;
#139175=CARTESIAN_POINT('Ctrl Pts',(-3.36870744055528,-1.04639008266731,
-13.5532048478642)) ;
#139176=CARTESIAN_POINT('Ctrl Pts',(-3.38358960366098,-0.950000000886305,
-13.5495669857718)) ;
#139177=CARTESIAN_POINT('Ctrl Pts',(-3.37639320225,-1.05,-13.6542704156447)) ;
#139178=CARTESIAN_POINT('Ctrl Pts',(-3.3526478932023,-1.05,-13.557130514995)) ;
#139179=CARTESIAN_POINT('Ctrl Pts',(-3.3526478932023,-0.95,-13.557130514995)) ;
#139180=CARTESIAN_POINT('Origin',(-3.37639320224937,-1.1500000000029,-13.654270415645)) ;
#139181=CARTESIAN_POINT('Origin',(-4.66204490261456,-1.5692190524323,-17.14)) ;
#139182=CARTESIAN_POINT('Origin',(-4.66204490261456,-1.5692190524323,-17.14)) ;
#139183=CARTESIAN_POINT('Origin',(-3.37639320225,-1.15,-15.24)) ;
#139184=CARTESIAN_POINT('Origin',(-3.37639320225038,-1.14999999999817,-16.8257295843555)) ;
#139185=CARTESIAN_POINT('Origin',(-1.50751564693271,0.00804557540861825,
-16.3688928486111)) ;
#139186=CARTESIAN_POINT('Origin',(-3.46583592134999,-0.971114561800017,
-16.8475933601353)) ;
#139187=CARTESIAN_POINT('Ctrl Pts',(-3.37639320225,-1.05,-16.8257295843553)) ;
#139188=CARTESIAN_POINT('Ctrl Pts',(-3.3526478932023,-1.05,-16.922869485005)) ;
#139189=CARTESIAN_POINT('Ctrl Pts',(-3.3526478932023,-0.95,-16.922869485005)) ;
#139190=CARTESIAN_POINT('Ctrl Pts',(-3.39186274464434,-1.05,-16.833292471748)) ;
#139191=CARTESIAN_POINT('Ctrl Pts',(-3.36870744055529,-1.04639008266723,
-16.9267951521356)) ;
#139192=CARTESIAN_POINT('Ctrl Pts',(-3.38358960366097,-0.950000000886305,
-16.9304330142282)) ;
#139193=CARTESIAN_POINT('Ctrl Pts',(-3.40727897628736,-1.05363948814369,
-16.8408292960084)) ;
#139194=CARTESIAN_POINT('Ctrl Pts',(-3.3866531924555,-1.04670310838586,
-16.931181891489)) ;
#139195=CARTESIAN_POINT('Ctrl Pts',(-3.4144159452097,-0.957277229261615,
-16.9379683421624)) ;
#139196=CARTESIAN_POINT('Ctrl Pts',(-3.4211145618,-1.06055728090001,-16.8475933601353)) ;
#139197=CARTESIAN_POINT('Ctrl Pts',(-3.40394191641935,-1.05197095820969,
-16.9354080240136)) ;
#139198=CARTESIAN_POINT('Ctrl Pts',(-3.44209061230229,-0.971114561800017,
-16.944733260785)) ;
#139199=CARTESIAN_POINT('Origin',(-3.37639320225,-0.95,-16.8257295843553)) ;
#139200=CARTESIAN_POINT('Origin',(0.175392621986784,-0.95,-15.9575152717641)) ;
#139201=CARTESIAN_POINT('Origin',(12.8,2.65,-16.7330460421716)) ;
#139202=CARTESIAN_POINT('',(4.57524318173533,2.73534903669982,-16.6809351802097)) ;
#139203=CARTESIAN_POINT('Origin',(4.65232986200977,2.66527023614941,-16.7287542111863)) ;
#139204=CARTESIAN_POINT('Ctrl Pts',(4.57524318173533,2.73534903669982,-16.6809351802097)) ;
#139205=CARTESIAN_POINT('Ctrl Pts',(4.5761458558036,2.73452842391049,-16.6795911511832)) ;
#139206=CARTESIAN_POINT('Ctrl Pts',(4.57705238626145,2.73367683201793,-16.6782681293393)) ;
#139207=CARTESIAN_POINT('Ctrl Pts',(4.5779495181309,2.73280244902548,-16.6769768488888)) ;
#139208=CARTESIAN_POINT('Ctrl Pts',(4.58144263576934,2.7293979075554,-16.6719490545685)) ;
#139209=CARTESIAN_POINT('Ctrl Pts',(4.58496694799982,2.72549786515183,-16.6671699445179)) ;
#139210=CARTESIAN_POINT('Ctrl Pts',(4.58815670056902,2.72107165565054,-16.6626981938528)) ;
#139211=CARTESIAN_POINT('Ctrl Pts',(4.59069123847472,2.71755464437262,-16.6591449961298)) ;
#139212=CARTESIAN_POINT('Ctrl Pts',(4.59301454561853,2.71370459823908,-16.6557863127242)) ;
#139213=CARTESIAN_POINT('Ctrl Pts',(4.5949431309995,2.70950205848695,-16.6526749961674)) ;
#139214=CARTESIAN_POINT('Ctrl Pts',(4.59651854606294,2.7060691047295,-16.6501334364215)) ;
#139215=CARTESIAN_POINT('Ctrl Pts',(4.59783685868319,2.70233705077427,-16.6477160861571)) ;
#139216=CARTESIAN_POINT('Ctrl Pts',(4.59873118971422,2.69838744820002,-16.6455323012123)) ;
#139217=CARTESIAN_POINT('Ctrl Pts',(4.59916508318197,2.6964712597891,-16.6444728165364)) ;
#139218=CARTESIAN_POINT('Ctrl Pts',(4.59949917984822,2.6945044443219,-16.643467798882)) ;
#139219=CARTESIAN_POINT('Ctrl Pts',(4.5997144226265,2.692499226592,-16.6425263440994)) ;
#139220=CARTESIAN_POINT('Ctrl Pts',(4.59990113259977,2.69075982259552,-16.6417096895352)) ;
#139221=CARTESIAN_POINT('Ctrl Pts',(4.6,2.68896788689974,-16.6409303122145)) ;
#139222=CARTESIAN_POINT('Ctrl Pts',(4.6,2.68715716172261,-16.6402056127633)) ;
#139223=CARTESIAN_POINT('Origin',(4.5,2.1,-16.6219539578284)) ;
#139224=CARTESIAN_POINT('Origin',(4.6,2.1,-16.6219539578284)) ;
#139225=CARTESIAN_POINT('Origin',(12.7,2.1,-16.6219539578284)) ;
#139226=CARTESIAN_POINT('Origin',(12.7,2.76643989873054,-16.7136393923832)) ;
#139227=CARTESIAN_POINT('Origin',(12.7,2.13287979746107,-16.8192327425948)) ;
#139228=CARTESIAN_POINT('Origin',(4.4,2.72431432344521,-15.24)) ;
#139229=CARTESIAN_POINT('Ctrl Pts',(4.48762159086959,2.77250619842349,-13.8511756817495)) ;
#139230=CARTESIAN_POINT('Ctrl Pts',(4.48806820038223,2.77169418112776,-13.8538355670898)) ;
#139231=CARTESIAN_POINT('Ctrl Pts',(4.48852084821546,2.77084293101113,-13.8564827150185)) ;
#139232=CARTESIAN_POINT('Ctrl Pts',(4.49012932137854,2.76769877392856,-13.8657630095207)) ;
#139233=CARTESIAN_POINT('Ctrl Pts',(4.49131046584974,2.76517764467229,-13.8723441317034)) ;
#139234=CARTESIAN_POINT('Ctrl Pts',(4.49351977821776,2.75978760391033,-13.884635280162)) ;
#139235=CARTESIAN_POINT('Ctrl Pts',(4.49455195297827,2.75697653750127,-13.8903677406013)) ;
#139236=CARTESIAN_POINT('Ctrl Pts',(4.49620670090465,2.75163165728875,-13.8999433216032)) ;
#139237=CARTESIAN_POINT('Ctrl Pts',(4.49686252944492,2.74924176842724,-13.9038640262033)) ;
#139238=CARTESIAN_POINT('Ctrl Pts',(4.49822764032848,2.74331716058958,-13.9126446316346)) ;
#139239=CARTESIAN_POINT('Ctrl Pts',(4.49890203357901,2.73961076902724,-13.9174865001603)) ;
#139240=CARTESIAN_POINT('Ctrl Pts',(4.49975897856021,2.73206576252701,-13.9258277784396)) ;
#139241=CARTESIAN_POINT('Ctrl Pts',(4.5,2.72833175948628,-13.9294190022917)) ;
#139242=CARTESIAN_POINT('Ctrl Pts',(4.5,2.72431432344521,-13.932634816645)) ;
#139243=CARTESIAN_POINT('Ctrl Pts',(4.5,2.72431432344521,-16.547365183355)) ;
#139244=CARTESIAN_POINT('Ctrl Pts',(4.5,2.72904669151416,-16.5511532753135)) ;
#139245=CARTESIAN_POINT('Ctrl Pts',(4.49966645684475,2.73338556955534,-16.5554614101758)) ;
#139246=CARTESIAN_POINT('Ctrl Pts',(4.49869539480397,2.74072289096356,-16.5639802414372)) ;
#139247=CARTESIAN_POINT('Ctrl Pts',(4.49811062025689,2.74382502998075,-16.5681080596585)) ;
#139248=CARTESIAN_POINT('Ctrl Pts',(4.49664125196625,2.75020211699685,-16.5775592649405)) ;
#139249=CARTESIAN_POINT('Ctrl Pts',(4.49570721389712,2.75339870015137,-16.5830103903193)) ;
#139250=CARTESIAN_POINT('Ctrl Pts',(4.49363760641479,2.75952863263942,-16.5947517051868)) ;
#139251=CARTESIAN_POINT('Ctrl Pts',(4.49249077386345,2.76240287369066,-16.6010712258307)) ;
#139252=CARTESIAN_POINT('Ctrl Pts',(4.49055019898874,2.76677757270134,-16.6119141256208)) ;
#139253=CARTESIAN_POINT('Ctrl Pts',(4.48975662823144,2.76842729450632,-16.6163872919226)) ;
#139254=CARTESIAN_POINT('Ctrl Pts',(4.4885208482156,2.77084293101086,-16.6235172849807)) ;
#139255=CARTESIAN_POINT('Ctrl Pts',(4.48806820038251,2.77169418112725,-16.6261644329085)) ;
#139256=CARTESIAN_POINT('Ctrl Pts',(4.48762159086959,2.77250619842348,-16.6288243182478)) ;
#139257=CARTESIAN_POINT('Origin',(4.6,2.1,-15.24)) ;
#139258=CARTESIAN_POINT('Origin',(4.6,2.1,-13.8580460421716)) ;
#139259=CARTESIAN_POINT('Origin',(4.6,2.1,-16.6219539578284)) ;
#139260=CARTESIAN_POINT('Origin',(12.7,2.1,-16.6219539578284)) ;
#139261=CARTESIAN_POINT('Origin',(12.7,1.9,-16.6219539578284)) ;
#139262=CARTESIAN_POINT('Origin',(12.7,2.65,-12.7)) ;
#139263=CARTESIAN_POINT('Origin',(4.5,2.65,-13.7469539578284)) ;
#139264=CARTESIAN_POINT('',(4.6,2.68715716172261,-13.8397943872367)) ;
#139265=CARTESIAN_POINT('',(4.57524318173443,2.73534903670064,-13.7990648197889)) ;
#139266=CARTESIAN_POINT('Ctrl Pts',(4.6,2.68715716172261,-13.8397943872367)) ;
#139267=CARTESIAN_POINT('Ctrl Pts',(4.6,2.69106036671411,-13.8382322227785)) ;
#139268=CARTESIAN_POINT('Ctrl Pts',(4.59952510519174,2.69488861888981,-13.8364097094748)) ;
#139269=CARTESIAN_POINT('Ctrl Pts',(4.59869497748257,2.6985274364076,-13.8343901512251)) ;
#139270=CARTESIAN_POINT('Ctrl Pts',(4.59815316003466,2.70090246232122,-13.8330720023612)) ;
#139271=CARTESIAN_POINT('Ctrl Pts',(4.5974600110878,2.70319720658043,-13.8316709680453)) ;
#139272=CARTESIAN_POINT('Ctrl Pts',(4.59664880273703,2.70538659711789,-13.8302145418985)) ;
#139273=CARTESIAN_POINT('Ctrl Pts',(4.59612777291939,2.70679281754375,-13.8292790960924)) ;
#139274=CARTESIAN_POINT('Ctrl Pts',(4.59555051815356,2.70817855133088,-13.8283049299072)) ;
#139275=CARTESIAN_POINT('Ctrl Pts',(4.59494172533681,2.7095051214937,-13.8273227360698)) ;
#139276=CARTESIAN_POINT('Ctrl Pts',(4.59250947890868,2.71480502887001,-13.8233986794992)) ;
#139277=CARTESIAN_POINT('Ctrl Pts',(4.58944857813008,2.71954517005227,-13.8190823375811)) ;
#139278=CARTESIAN_POINT('Ctrl Pts',(4.5861276864684,2.72376361218884,-13.8144738031841)) ;
#139279=CARTESIAN_POINT('Ctrl Pts',(4.58350334758194,2.72709724148698,-13.8108319029778)) ;
#139280=CARTESIAN_POINT('Ctrl Pts',(4.58071664514672,2.73010548898765,-13.8070059959317)) ;
#139281=CARTESIAN_POINT('Ctrl Pts',(4.5779495181309,2.73280244902546,-13.8030231511112)) ;
#139282=CARTESIAN_POINT('Ctrl Pts',(4.57705238626115,2.7336768320182,-13.8017318706603)) ;
#139283=CARTESIAN_POINT('Ctrl Pts',(4.576145855803,2.73452842391107,-13.8004088488159)) ;
#139284=CARTESIAN_POINT('Ctrl Pts',(4.57524318173444,2.73534903670067,-13.7990648197889)) ;
#139285=CARTESIAN_POINT('Origin',(4.65232986201396,2.66527023614562,-13.7512457888124)) ;
#139286=CARTESIAN_POINT('Origin',(4.6,2.65,-13.7469539578284)) ;
#139287=CARTESIAN_POINT('Origin',(12.7,1.9,-16.74)) ;
#139288=CARTESIAN_POINT('Origin',(12.7,2.01643989873054,-13.6413606076168)) ;
#139289=CARTESIAN_POINT('Origin',(-3.65,10.7,-14.49)) ;
#139290=CARTESIAN_POINT('Origin',(-3.65,10.7,-14.49)) ;
#139291=CARTESIAN_POINT('Origin',(-3.65,10.7,-14.49)) ;
#139292=CARTESIAN_POINT('Origin',(0.,10.7,-14.49)) ;
#139293=CARTESIAN_POINT('Origin',(-2.9,10.7,-14.49)) ;
#139294=CARTESIAN_POINT('Origin',(-3.65,10.7,-15.24)) ;
#139295=CARTESIAN_POINT('Origin',(-3.65,10.7,-15.99)) ;
#139296=CARTESIAN_POINT('Origin',(-2.9,10.7,-14.49)) ;
#139297=CARTESIAN_POINT('Origin',(-2.9,10.7,-14.49)) ;
#139298=CARTESIAN_POINT('Origin',(-3.65,10.7,-15.99)) ;
#139299=CARTESIAN_POINT('Origin',(-3.65,10.7,-15.99)) ;
#139300=CARTESIAN_POINT('Origin',(-2.9,10.7,-15.24)) ;
#139301=CARTESIAN_POINT('Origin',(-2.9,10.7,-15.99)) ;
#139302=CARTESIAN_POINT('Origin',(0.,10.7,-15.99)) ;
#139303=CARTESIAN_POINT('Origin',(-2.9,10.7,-15.99)) ;
#139304=CARTESIAN_POINT('Origin',(-2.9,10.7,-15.99)) ;
#139305=CARTESIAN_POINT('Origin',(-3.05,-3.95,-14.24)) ;
#139306=CARTESIAN_POINT('Origin',(-3.05,-3.95,-16.14)) ;
#139307=CARTESIAN_POINT('Origin',(-3.05,-3.95,-14.34)) ;
#139308=CARTESIAN_POINT('Origin',(-3.25,-3.95,-14.34)) ;
#139309=CARTESIAN_POINT('Origin',(-3.25,-3.95,-14.14)) ;
#139310=CARTESIAN_POINT('Origin',(-3.25,-3.95,-14.34)) ;
#139311=CARTESIAN_POINT('Origin',(-3.25,-3.95,-16.14)) ;
#139312=CARTESIAN_POINT('Origin',(-3.25,-3.95,-16.14)) ;
#139313=CARTESIAN_POINT('Origin',(-3.25,-3.95,-16.34)) ;
#139314=CARTESIAN_POINT('Origin',(-4.4,-3.95,-14.14)) ;
#139315=CARTESIAN_POINT('Origin',(-4.3,-3.95,-14.14)) ;
#139316=CARTESIAN_POINT('Origin',(-3.25,-3.9,-14.34)) ;
#139317=CARTESIAN_POINT('Origin',(-3.25,-3.85,-14.34)) ;
#139318=CARTESIAN_POINT('Origin',(-3.25,-3.85,-15.24)) ;
#139319=CARTESIAN_POINT('Origin',(-3.25,-3.85,-16.14)) ;
#139320=CARTESIAN_POINT('Origin',(-3.25,-3.85,-14.34)) ;
#139321=CARTESIAN_POINT('Origin',(-3.25,-3.9,-16.14)) ;
#139322=CARTESIAN_POINT('Origin',(-3.25,-3.85,-16.14)) ;
#139323=CARTESIAN_POINT('Origin',(-4.4,-3.95,-16.34)) ;
#139324=CARTESIAN_POINT('Origin',(-4.3,-3.95,-16.34)) ;
#139325=CARTESIAN_POINT('Origin',(-4.5,-3.95,-14.24)) ;
#139326=CARTESIAN_POINT('Origin',(-4.5,-3.95,-14.34)) ;
#139327=CARTESIAN_POINT('Origin',(-4.5,-3.95,-16.14)) ;
#139328=CARTESIAN_POINT('Origin',(-4.3,-3.95,-14.34)) ;
#139329=CARTESIAN_POINT('Origin',(-4.3,-3.95,-14.34)) ;
#139330=CARTESIAN_POINT('Origin',(-3.25,-3.85,-14.34)) ;
#139331=CARTESIAN_POINT('Origin',(-3.25,-3.85,-14.34)) ;
#139332=CARTESIAN_POINT('Origin',(-3.25,-3.85,-16.14)) ;
#139333=CARTESIAN_POINT('Origin',(-3.25,-3.85,-16.14)) ;
#139334=CARTESIAN_POINT('Origin',(-4.3,-3.95,-16.14)) ;
#139335=CARTESIAN_POINT('Origin',(-4.3,-3.95,-16.14)) ;
#139336=CARTESIAN_POINT('Origin',(-4.3,-3.9,-14.34)) ;
#139337=CARTESIAN_POINT('Origin',(-4.3,-3.85,-14.34)) ;
#139338=CARTESIAN_POINT('Origin',(-1.56125112837913E-16,-3.85,-14.34)) ;
#139339=CARTESIAN_POINT('Origin',(-4.3,-3.85,-14.34)) ;
#139340=CARTESIAN_POINT('Origin',(-1.56125112837913E-16,-3.85,-16.14)) ;
#139341=CARTESIAN_POINT('Origin',(-4.3,-3.85,-16.14)) ;
#139342=CARTESIAN_POINT('Origin',(-4.3,-3.9,-16.14)) ;
#139343=CARTESIAN_POINT('Origin',(-4.3,-3.85,-16.14)) ;
#139344=CARTESIAN_POINT('Origin',(-4.3,-3.85,-14.34)) ;
#139345=CARTESIAN_POINT('Origin',(-4.3,-3.85,-14.34)) ;
#139346=CARTESIAN_POINT('Origin',(-4.3,-3.85,-16.14)) ;
#139347=CARTESIAN_POINT('Origin',(-4.3,-3.85,-16.14)) ;
#139348=CARTESIAN_POINT('Origin',(-4.3,-3.85,-15.24)) ;
#139349=CARTESIAN_POINT('Origin',(-4.,10.85,-16.24)) ;
#139350=CARTESIAN_POINT('Origin',(-4.,10.85,-16.14)) ;
#139351=CARTESIAN_POINT('Origin',(-4.,10.85,-14.34)) ;
#139352=CARTESIAN_POINT('Origin',(-3.8,10.85,-14.34)) ;
#139353=CARTESIAN_POINT('Origin',(-3.8,10.85,-14.14)) ;
#139354=CARTESIAN_POINT('Origin',(-3.8,10.85,-14.34)) ;
#139355=CARTESIAN_POINT('Origin',(-3.8,10.85,-16.14)) ;
#139356=CARTESIAN_POINT('Origin',(-3.8,10.85,-16.14)) ;
#139357=CARTESIAN_POINT('Origin',(-3.8,10.85,-16.34)) ;
#139358=CARTESIAN_POINT('Origin',(-3.9,10.85,-14.14)) ;
#139359=CARTESIAN_POINT('Origin',(-2.75,10.85,-14.14)) ;
#139360=CARTESIAN_POINT('Origin',(-3.8,10.8,-14.34)) ;
#139361=CARTESIAN_POINT('Origin',(-3.8,10.75,-14.34)) ;
#139362=CARTESIAN_POINT('Origin',(-3.8,10.75,-15.24)) ;
#139363=CARTESIAN_POINT('Origin',(-3.8,10.75,-16.14)) ;
#139364=CARTESIAN_POINT('Origin',(-3.8,10.75,-14.34)) ;
#139365=CARTESIAN_POINT('Origin',(-3.8,10.8,-16.14)) ;
#139366=CARTESIAN_POINT('Origin',(-3.8,10.75,-16.14)) ;
#139367=CARTESIAN_POINT('Origin',(-3.9,10.85,-16.34)) ;
#139368=CARTESIAN_POINT('Origin',(-2.75,10.85,-16.34)) ;
#139369=CARTESIAN_POINT('Origin',(-2.55,10.85,-16.24)) ;
#139370=CARTESIAN_POINT('Origin',(-2.55,10.85,-14.34)) ;
#139371=CARTESIAN_POINT('Origin',(-2.55,10.85,-16.14)) ;
#139372=CARTESIAN_POINT('Origin',(-2.75,10.85,-14.34)) ;
#139373=CARTESIAN_POINT('Origin',(-2.75,10.85,-14.34)) ;
#139374=CARTESIAN_POINT('Origin',(-3.8,10.75,-14.34)) ;
#139375=CARTESIAN_POINT('Origin',(-3.8,10.75,-14.34)) ;
#139376=CARTESIAN_POINT('Origin',(-3.8,10.75,-16.14)) ;
#139377=CARTESIAN_POINT('Origin',(-3.8,10.75,-16.14)) ;
#139378=CARTESIAN_POINT('Origin',(-2.75,10.85,-16.14)) ;
#139379=CARTESIAN_POINT('Origin',(-2.75,10.85,-16.14)) ;
#139380=CARTESIAN_POINT('Origin',(-2.75,10.8,-14.34)) ;
#139381=CARTESIAN_POINT('Origin',(-2.75,10.75,-14.34)) ;
#139382=CARTESIAN_POINT('Origin',(1.56125112837912E-16,10.75,-14.34)) ;
#139383=CARTESIAN_POINT('Origin',(-2.75,10.75,-14.34)) ;
#139384=CARTESIAN_POINT('Origin',(-1.56125112837913E-16,10.75,-16.14)) ;
#139385=CARTESIAN_POINT('Origin',(-2.75,10.75,-16.14)) ;
#139386=CARTESIAN_POINT('Origin',(-2.75,10.8,-16.14)) ;
#139387=CARTESIAN_POINT('Origin',(-2.75,10.75,-16.14)) ;
#139388=CARTESIAN_POINT('Origin',(-2.75,10.75,-14.34)) ;
#139389=CARTESIAN_POINT('Origin',(-2.75,10.75,-14.34)) ;
#139390=CARTESIAN_POINT('Origin',(-2.75,10.75,-16.14)) ;
#139391=CARTESIAN_POINT('Origin',(-2.75,10.75,-16.14)) ;
#139392=CARTESIAN_POINT('Origin',(-2.75,10.75,-15.24)) ;
#139393=CARTESIAN_POINT('Origin',(4.6,0.,-15.24)) ;
#139394=CARTESIAN_POINT('Ctrl Pts',(4.5,-2.7,-13.7168453788272)) ;
#139395=CARTESIAN_POINT('Ctrl Pts',(4.5,-2.71827986285823,-13.7919647391751)) ;
#139396=CARTESIAN_POINT('Ctrl Pts',(4.50597963419107,-2.73556801027185,
-13.8667398604528)) ;
#139397=CARTESIAN_POINT('Ctrl Pts',(4.52394923367545,-2.75977758633329,
-13.9784368340216)) ;
#139398=CARTESIAN_POINT('Ctrl Pts',(4.53141024883993,-2.76757607569523,
-14.0156832823903)) ;
#139399=CARTESIAN_POINT('Ctrl Pts',(4.54734065524867,-2.77857284247615,
-14.070165689583)) ;
#139400=CARTESIAN_POINT('Ctrl Pts',(4.55339248498575,-2.78214991573955,
-14.0882382744149)) ;
#139401=CARTESIAN_POINT('Ctrl Pts',(4.56567492147096,-2.787183259287,-14.1141467218607)) ;
#139402=CARTESIAN_POINT('Ctrl Pts',(4.5702469143305,-2.78880341224556,-14.1225726050508)) ;
#139403=CARTESIAN_POINT('Ctrl Pts',(4.58215938980081,-2.79169669265294,
-14.1377434798851)) ;
#139404=CARTESIAN_POINT('Ctrl Pts',(4.59005470866978,-2.79310344827587,
-14.1452063540423)) ;
#139405=CARTESIAN_POINT('Ctrl Pts',(4.6,-2.79310344827586,-14.1452063540422)) ;
#139406=CARTESIAN_POINT('Origin',(4.6,-2.4,-13.2778583129651)) ;
#139407=CARTESIAN_POINT('Origin',(4.6,-2.4,-12.7)) ;
#139408=CARTESIAN_POINT('Origin',(4.6,-2.4,-13.2778583129651)) ;
#139409=CARTESIAN_POINT('Origin',(4.6,-2.4,-13.2778583129651)) ;
#139410=CARTESIAN_POINT('Origin',(4.6,-2.4,-13.2778583129651)) ;
#139411=CARTESIAN_POINT('Origin',(0.584645609909622,-2.4,-13.2778583129651)) ;
#139412=CARTESIAN_POINT('Origin',(12.7,-2.4,-13.2778583129651)) ;
#139413=CARTESIAN_POINT('Origin',(12.7,-2.2,-12.7)) ;
#139414=CARTESIAN_POINT('Origin',(12.7,-2.2,-13.2778583129651)) ;
#139415=CARTESIAN_POINT('Origin',(12.7,-2.4,-13.2778583129651)) ;
#139416=CARTESIAN_POINT('Origin',(12.7,-2.24516129032258,-13.4044480992255)) ;
#139417=CARTESIAN_POINT('Origin',(12.7,0.,-15.24)) ;
#139418=CARTESIAN_POINT('Origin',(12.7,-2.24516129032258,-17.0755519007745)) ;
#139419=CARTESIAN_POINT('Origin',(12.7,-2.4,-17.2021416870349)) ;
#139420=CARTESIAN_POINT('Origin',(12.7,-2.4,-17.2021416870349)) ;
#139421=CARTESIAN_POINT('Origin',(0.584645609909622,-2.4,-17.2021416870349)) ;
#139422=CARTESIAN_POINT('Origin',(4.6,-2.4,-17.2021416870349)) ;
#139423=CARTESIAN_POINT('Origin',(4.6,-2.4,-17.2021416870349)) ;
#139424=CARTESIAN_POINT('Origin',(4.6,-2.4,-17.2021416870349)) ;
#139425=CARTESIAN_POINT('Origin',(4.6,0.,-15.24)) ;
#139426=CARTESIAN_POINT('Ctrl Pts',(4.6,-2.79310344827586,-16.3347936459578)) ;
#139427=CARTESIAN_POINT('Ctrl Pts',(4.59007568892311,-2.79310344827586,
-16.3347936459578)) ;
#139428=CARTESIAN_POINT('Ctrl Pts',(4.58219207637239,-2.79170232102183,
-16.342226742276)) ;
#139429=CARTESIAN_POINT('Ctrl Pts',(4.57028631514659,-2.78881527838255,
-16.35736543899)) ;
#139430=CARTESIAN_POINT('Ctrl Pts',(4.56571532154372,-2.78719767797524,
-16.3657784885835)) ;
#139431=CARTESIAN_POINT('Ctrl Pts',(4.55343865632726,-2.78217307830036,
-16.3916436333089)) ;
#139432=CARTESIAN_POINT('Ctrl Pts',(4.54738888873344,-2.77860151743012,
-16.4096900859661)) ;
#139433=CARTESIAN_POINT('Ctrl Pts',(4.53146440752602,-2.76762263748299,
-16.4640903156831)) ;
#139434=CARTESIAN_POINT('Ctrl Pts',(4.52400917967609,-2.75984503873828,
-16.5012455063058)) ;
#139435=CARTESIAN_POINT('Ctrl Pts',(4.50599905604505,-2.7356206423885,-16.6130301354693)) ;
#139436=CARTESIAN_POINT('Ctrl Pts',(4.5,-2.71826422026483,-16.6880995425769)) ;
#139437=CARTESIAN_POINT('Ctrl Pts',(4.5,-2.7,-16.7631546211728)) ;
#139438=CARTESIAN_POINT('Origin',(-0.362523114814661,9.05,-15.4090473046963)) ;
#139439=CARTESIAN_POINT('Origin',(0.36252311481466,9.05,-15.0709526953037)) ;
#139440=CARTESIAN_POINT('Origin',(-1.31845674202095,9.85,-13.8322813422351)) ;
#139441=CARTESIAN_POINT('Origin',(-0.230887397576972,9.85,-13.3251394281462)) ;
#139442=CARTESIAN_POINT('Origin',(4.6,2.1,-13.8580460421716)) ;
#139443=CARTESIAN_POINT('Origin',(4.6,2.1,-13.8580460421716)) ;
#139444=CARTESIAN_POINT('Origin',(4.6,0.280857398566761,-13.5548556085994)) ;
#139445=CARTESIAN_POINT('Origin',(4.6,2.61712020253893,-13.9442327425948)) ;
#139446=CARTESIAN_POINT('Origin',(4.6,2.65,-13.7469539578284)) ;
#139447=CARTESIAN_POINT('Origin',(4.6,2.72431432344521,-13.932634816645)) ;
#139448=CARTESIAN_POINT('Ctrl Pts',(4.48762159086906,2.77250619842445,-13.8511756817496)) ;
#139449=CARTESIAN_POINT('Ctrl Pts',(4.51316716229104,2.72605970493114,-13.8142387941972)) ;
#139450=CARTESIAN_POINT('Ctrl Pts',(4.57527453405851,2.73535372386122,-13.799057153198)) ;
#139451=CARTESIAN_POINT('Ctrl Pts',(4.49363662433154,2.76156977394749,-13.8869995924717)) ;
#139452=CARTESIAN_POINT('Ctrl Pts',(4.5146945995807,2.70766535161857,-13.8362008473933)) ;
#139453=CARTESIAN_POINT('Ctrl Pts',(4.58732693581886,2.72440392220679,-13.816995041234)) ;
#139454=CARTESIAN_POINT('Ctrl Pts',(4.5,2.74488438438029,-13.9161692160662)) ;
#139455=CARTESIAN_POINT('Ctrl Pts',(4.50856472873622,2.69031482079682,-13.8384911137046)) ;
#139456=CARTESIAN_POINT('Ctrl Pts',(4.60003980620506,2.7077507326983,-13.8315523113747)) ;
#139457=CARTESIAN_POINT('Ctrl Pts',(4.5,2.72431432344521,-13.932634816645)) ;
#139458=CARTESIAN_POINT('Ctrl Pts',(4.5,2.68714136424468,-13.8397549158517)) ;
#139459=CARTESIAN_POINT('Ctrl Pts',(4.60004250625997,2.68715716507935,-13.8397943956238)) ;
#139460=CARTESIAN_POINT('Origin',(4.57524318173443,2.82069807340128,-13.8511756817495)) ;
#139461=CARTESIAN_POINT('Ctrl Pts',(4.47150553123747,2.80180812502279,-13.7469539578284)) ;
#139462=CARTESIAN_POINT('Ctrl Pts',(4.5,2.75,-13.7469539578284)) ;
#139463=CARTESIAN_POINT('Ctrl Pts',(4.55912712210514,2.75,-13.7469539578284)) ;
#139464=CARTESIAN_POINT('Ctrl Pts',(4.47150553186688,2.8018081238784,-13.7835744727347)) ;
#139465=CARTESIAN_POINT('Ctrl Pts',(4.50000000073523,2.74999999866316,-13.7712580842688)) ;
#139466=CARTESIAN_POINT('Ctrl Pts',(4.5591271227348,2.75,-13.7652720457593)) ;
#139467=CARTESIAN_POINT('Ctrl Pts',(4.4771244897161,2.79159183687982,-13.8199165373523)) ;
#139468=CARTESIAN_POINT('Ctrl Pts',(4.50480340096853,2.74126654369358,-13.795537950998)) ;
#139469=CARTESIAN_POINT('Ctrl Pts',(4.56473907811163,2.74489822224648,-13.7834248215822)) ;
#139470=CARTESIAN_POINT('Ctrl Pts',(4.48762159086676,2.77250619842407,-13.8511756817495)) ;
#139471=CARTESIAN_POINT('Ctrl Pts',(4.51315802400618,2.72607631998876,-13.8142520074343)) ;
#139472=CARTESIAN_POINT('Ctrl Pts',(4.57524318173443,2.73534903670064,-13.7990648197889)) ;
#139473=CARTESIAN_POINT('Origin',(4.55912712210513,2.85,-13.7469539578284)) ;
#139474=CARTESIAN_POINT('Origin',(4.55912712210514,2.85,-12.7)) ;
#139475=CARTESIAN_POINT('Ctrl Pts',(4.48762159086766,2.77250619842243,-16.6288243182478)) ;
#139476=CARTESIAN_POINT('Ctrl Pts',(4.51315802400691,2.72607631998744,-16.6657479925641)) ;
#139477=CARTESIAN_POINT('Ctrl Pts',(4.57524318173533,2.73534903669982,-16.6809351802097)) ;
#139478=CARTESIAN_POINT('Ctrl Pts',(4.47712448971643,2.79159183687922,-16.6600834626457)) ;
#139479=CARTESIAN_POINT('Ctrl Pts',(4.50480340096884,2.74126654369303,-16.6844620490007)) ;
#139480=CARTESIAN_POINT('Ctrl Pts',(4.56473907811196,2.74489822224618,-16.6965751784167)) ;
#139481=CARTESIAN_POINT('Ctrl Pts',(4.47150553186688,2.8018081238784,-16.6964255272642)) ;
#139482=CARTESIAN_POINT('Ctrl Pts',(4.50000000073523,2.74999999866316,-16.7087419157305)) ;
#139483=CARTESIAN_POINT('Ctrl Pts',(4.5591271227348,2.75,-16.7147279542401)) ;
#139484=CARTESIAN_POINT('Ctrl Pts',(4.47150553123747,2.80180812502279,-16.7330460421716)) ;
#139485=CARTESIAN_POINT('Ctrl Pts',(4.5,2.75,-16.7330460421716)) ;
#139486=CARTESIAN_POINT('Ctrl Pts',(4.55912712210513,2.75,-16.7330460421716)) ;
#139487=CARTESIAN_POINT('Origin',(4.57524318173533,2.82069807339964,-16.6288243182478)) ;
#139488=CARTESIAN_POINT('Ctrl Pts',(4.57527448145479,2.73535371598842,-16.6809428339419)) ;
#139489=CARTESIAN_POINT('Ctrl Pts',(4.51316714695683,2.7260597328105,-16.6657611836292)) ;
#139490=CARTESIAN_POINT('Ctrl Pts',(4.48762159086951,2.77250619842363,-16.6288243182477)) ;
#139491=CARTESIAN_POINT('Ctrl Pts',(4.5873268774263,2.72440390874888,-16.6630049433246)) ;
#139492=CARTESIAN_POINT('Ctrl Pts',(4.5146945862635,2.7076653857066,-16.6437991204817)) ;
#139493=CARTESIAN_POINT('Ctrl Pts',(4.49363662433185,2.76156977394669,-16.5930004075269)) ;
#139494=CARTESIAN_POINT('Ctrl Pts',(4.60003973844309,2.70775071978185,-16.648447683485)) ;
#139495=CARTESIAN_POINT('Ctrl Pts',(4.50856472285798,2.69031485824816,-16.6415088329841)) ;
#139496=CARTESIAN_POINT('Ctrl Pts',(4.5,2.74488438437978,-16.5638307839333)) ;
#139497=CARTESIAN_POINT('Ctrl Pts',(4.60004243494351,2.6871571650681,-16.6402056044043)) ;
#139498=CARTESIAN_POINT('Ctrl Pts',(4.5,2.68714139075511,-16.6402450179097)) ;
#139499=CARTESIAN_POINT('Ctrl Pts',(4.5,2.72431432344521,-16.547365183355)) ;
#139500=CARTESIAN_POINT('Origin',(4.6,0.280857398566761,-16.9251443914006)) ;
#139501=CARTESIAN_POINT('Origin',(4.6,2.1,-16.6219539578284)) ;
#139502=CARTESIAN_POINT('Origin',(4.6,2.1,-16.6219539578284)) ;
#139503=CARTESIAN_POINT('Origin',(4.6,0.,-15.24)) ;
#139504=CARTESIAN_POINT('',(4.5,-2.9,-15.2400000000038)) ;
#139505=CARTESIAN_POINT('',(4.57439618084313,-2.80937499999937,-16.2827958671254)) ;
#139506=CARTESIAN_POINT('Ctrl Pts',(4.5,-2.9,-15.2400000000038)) ;
#139507=CARTESIAN_POINT('Ctrl Pts',(4.5,-2.9000000234111,-15.4161762625703)) ;
#139508=CARTESIAN_POINT('Ctrl Pts',(4.49893459747296,-2.89187728142186,
-15.5922938225552)) ;
#139509=CARTESIAN_POINT('Ctrl Pts',(4.50498172725087,-2.86839426105774,
-15.8549432768872)) ;
#139510=CARTESIAN_POINT('Ctrl Pts',(4.50826226558342,-2.85869729223562,
-15.9422870271135)) ;
#139511=CARTESIAN_POINT('Ctrl Pts',(4.52028413974051,-2.84160518746962,
-16.0728409654328)) ;
#139512=CARTESIAN_POINT('Ctrl Pts',(4.52545003690602,-2.8354696349403,-16.116363113622)) ;
#139513=CARTESIAN_POINT('Ctrl Pts',(4.53741870680498,-2.82581179679252,
-16.1806394550107)) ;
#139514=CARTESIAN_POINT('Ctrl Pts',(4.54209540184575,-2.82251395224859,
-16.2019200182606)) ;
#139515=CARTESIAN_POINT('Ctrl Pts',(4.55451190949429,-2.81582803324483,
-16.2438742105328)) ;
#139516=CARTESIAN_POINT('Ctrl Pts',(4.56139306411848,-2.8124020390272,-16.2647435318249)) ;
#139517=CARTESIAN_POINT('Ctrl Pts',(4.57439618084313,-2.80937499999937,
-16.2827958671254)) ;
#139518=CARTESIAN_POINT('Ctrl Pts',(4.57439618084313,-2.80937499999939,
-16.2827958671254)) ;
#139519=CARTESIAN_POINT('Ctrl Pts',(4.5778881172051,-2.80856205104936,-16.2876438845913)) ;
#139520=CARTESIAN_POINT('Ctrl Pts',(4.58132110715662,-2.80743849592505,
-16.2926543114197)) ;
#139521=CARTESIAN_POINT('Ctrl Pts',(4.58591063786559,-2.80541025280315,
-16.3000683491598)) ;
#139522=CARTESIAN_POINT('Ctrl Pts',(4.58721694730497,-2.80476695238161,
-16.3022683250837)) ;
#139523=CARTESIAN_POINT('Ctrl Pts',(4.5887449802686,-2.80393035430392,-16.3049717146409)) ;
#139524=CARTESIAN_POINT('Ctrl Pts',(4.58900094431508,-2.80378708879839,
-16.305429423373)) ;
#139525=CARTESIAN_POINT('Ctrl Pts',(4.58924476828968,-2.80364801935069,
-16.30586949326)) ;
#139526=CARTESIAN_POINT('Ctrl Pts',(4.58924931741448,-2.80364542371033,
-16.3058777053493)) ;
#139527=CARTESIAN_POINT('Ctrl Pts',(4.59158188358133,-2.80231401319274,
-16.3100892401221)) ;
#139528=CARTESIAN_POINT('Ctrl Pts',(4.59377134212491,-2.80081309849101,
-16.3144383923964)) ;
#139529=CARTESIAN_POINT('Ctrl Pts',(4.59570408210449,-2.79909049146272,
-16.3191378632085)) ;
#139530=CARTESIAN_POINT('Ctrl Pts',(4.5957084873849,-2.79908656285629,-16.3191485795779)) ;
#139531=CARTESIAN_POINT('Ctrl Pts',(4.59603576097762,-2.79879453264352,
-16.3199450754362)) ;
#139532=CARTESIAN_POINT('Ctrl Pts',(4.59633794834607,-2.79851279959495,
-16.3207065253189)) ;
#139533=CARTESIAN_POINT('Ctrl Pts',(4.59727216584803,-2.79759800070515,
-16.32316063341)) ;
#139534=CARTESIAN_POINT('Ctrl Pts',(4.59785661125443,-2.79695684051616,
-16.3248529156094)) ;
#139535=CARTESIAN_POINT('Ctrl Pts',(4.59875882816121,-2.7958009226755,-16.3278683242216)) ;
#139536=CARTESIAN_POINT('Ctrl Pts',(4.59910960512327,-2.79529211440566,
-16.3291844992176)) ;
#139537=CARTESIAN_POINT('Ctrl Pts',(4.59950074890552,-2.79458032370895,
-16.3310150784121)) ;
#139538=CARTESIAN_POINT('Ctrl Pts',(4.59959271145697,-2.79439474074567,
-16.3314948405808)) ;
#139539=CARTESIAN_POINT('Ctrl Pts',(4.59970479219924,-2.79411978912795,
-16.3322025710462)) ;
#139540=CARTESIAN_POINT('Ctrl Pts',(4.59973686334512,-2.79403231884248,
-16.3324272684452)) ;
#139541=CARTESIAN_POINT('Ctrl Pts',(4.59980956306601,-2.7938042827674,-16.3330108264021)) ;
#139542=CARTESIAN_POINT('Ctrl Pts',(4.59984405921136,-2.79366555090847,
-16.3333689790042)) ;
#139543=CARTESIAN_POINT('Ctrl Pts',(4.59992170638736,-2.79338632637294,
-16.3340824135446)) ;
#139544=CARTESIAN_POINT('Ctrl Pts',(4.59995882625634,-2.79324305250058,
-16.3344374792565)) ;
#139545=CARTESIAN_POINT('Ctrl Pts',(4.59999999999999,-2.79310344827586,
-16.3347936459578)) ;
#139546=CARTESIAN_POINT('',(4.57439618084271,-2.80937499999947,-14.1972041328751)) ;
#139547=CARTESIAN_POINT('Ctrl Pts',(4.59999999999999,-2.79310344827586,
-14.1452063540422)) ;
#139548=CARTESIAN_POINT('Ctrl Pts',(4.59995895305209,-2.79324111387631,
-14.1455620070442)) ;
#139549=CARTESIAN_POINT('Ctrl Pts',(4.59992125133673,-2.79338175512528,
-14.1459166499952)) ;
#139550=CARTESIAN_POINT('Ctrl Pts',(4.59984242179761,-2.79365985893298,
-14.1466272182547)) ;
#139551=CARTESIAN_POINT('Ctrl Pts',(4.5998070294299,-2.79379858543765,-14.146981904003)) ;
#139552=CARTESIAN_POINT('Ctrl Pts',(4.59973261548695,-2.79401893257626,
-14.1475458212796)) ;
#139553=CARTESIAN_POINT('Ctrl Pts',(4.59970092564442,-2.7941005010842,-14.1477547044526)) ;
#139554=CARTESIAN_POINT('Ctrl Pts',(4.59958060815602,-2.79437456977472,
-14.1484570742577)) ;
#139555=CARTESIAN_POINT('Ctrl Pts',(4.59947821517875,-2.79456857658396,
-14.1489550953807)) ;
#139556=CARTESIAN_POINT('Ctrl Pts',(4.5990597198479,-2.79527981802028,-14.1507850643885)) ;
#139557=CARTESIAN_POINT('Ctrl Pts',(4.59869396429225,-2.79579226918928,
-14.1521114012001)) ;
#139558=CARTESIAN_POINT('Ctrl Pts',(4.59768320083749,-2.79706868650734,
-14.1554440738933)) ;
#139559=CARTESIAN_POINT('Ctrl Pts',(4.59698254015873,-2.79783590182173,
-14.1574731996627)) ;
#139560=CARTESIAN_POINT('Ctrl Pts',(4.59599705225881,-2.79876532988112,
-14.1599846842385)) ;
#139561=CARTESIAN_POINT('Ctrl Pts',(4.59580678362762,-2.7989396411024,-14.1604581050039)) ;
#139562=CARTESIAN_POINT('Ctrl Pts',(4.59367882781299,-2.80083904916685,
-14.1656449119971)) ;
#139563=CARTESIAN_POINT('Ctrl Pts',(4.59150707087691,-2.80233337893514,
-14.1699793277041)) ;
#139564=CARTESIAN_POINT('Ctrl Pts',(4.58628071719236,-2.80532570224271,
-14.1794514674292)) ;
#139565=CARTESIAN_POINT('Ctrl Pts',(4.58313959595708,-2.8067311076741,-14.1845102480658)) ;
#139566=CARTESIAN_POINT('Ctrl Pts',(4.57802611146331,-2.80844040952816,
-14.1920963574918)) ;
#139567=CARTESIAN_POINT('Ctrl Pts',(4.57624387811645,-2.80894486836997,
-14.1946389593417)) ;
#139568=CARTESIAN_POINT('Ctrl Pts',(4.57439618084271,-2.80937499999947,
-14.1972041328751)) ;
#139569=CARTESIAN_POINT('Ctrl Pts',(4.57439618084271,-2.80937499999947,
-14.1972041328751)) ;
#139570=CARTESIAN_POINT('Ctrl Pts',(4.56149777794589,-2.81237766235467,
-14.2151110931668)) ;
#139571=CARTESIAN_POINT('Ctrl Pts',(4.55451596106519,-2.81582788236477,
-14.2361262422968)) ;
#139572=CARTESIAN_POINT('Ctrl Pts',(4.54213610452188,-2.82249001163036,
-14.2779283596283)) ;
#139573=CARTESIAN_POINT('Ctrl Pts',(4.53742891479326,-2.82580422498964,
-14.299310967236)) ;
#139574=CARTESIAN_POINT('Ctrl Pts',(4.525451614243,-2.8354670333868,-14.3636179437949)) ;
#139575=CARTESIAN_POINT('Ctrl Pts',(4.52032009146395,-2.84156292603926,
-14.4068565734785)) ;
#139576=CARTESIAN_POINT('Ctrl Pts',(4.50830110904356,-2.85862448221642,
-14.5371164259574)) ;
#139577=CARTESIAN_POINT('Ctrl Pts',(4.50499166750953,-2.86836219567853,
-14.6247300385823)) ;
#139578=CARTESIAN_POINT('Ctrl Pts',(4.49892845988062,-2.8918880660271,-14.8877629968379)) ;
#139579=CARTESIAN_POINT('Ctrl Pts',(4.49999999999475,-2.89999999999869,
-15.0638300901178)) ;
#139580=CARTESIAN_POINT('Ctrl Pts',(4.5,-2.9,-15.2400000000038)) ;
#139581=CARTESIAN_POINT('Origin',(4.4,-2.7,-12.7)) ;
#139582=CARTESIAN_POINT('Origin',(4.4,-2.7,-13.7168453788272)) ;
#139583=CARTESIAN_POINT('Ctrl Pts',(4.40227435089074,-2.79999990867355,
-13.6494006928819)) ;
#139584=CARTESIAN_POINT('Ctrl Pts',(4.51828879250226,-2.80015667527379,
-13.6587855667925)) ;
#139585=CARTESIAN_POINT('Ctrl Pts',(4.50118227077259,-2.68533700727772,
-13.6579711074494)) ;
#139586=CARTESIAN_POINT('Ctrl Pts',(4.39419482113926,-2.79999992837382,
-13.7636876996691)) ;
#139587=CARTESIAN_POINT('Ctrl Pts',(4.48571792501723,-2.80010751836584,
-13.7426713667506)) ;
#139588=CARTESIAN_POINT('Ctrl Pts',(4.49717570077252,-2.71006921719248,
-13.7570318982145)) ;
#139589=CARTESIAN_POINT('Ctrl Pts',(4.40636790575269,-2.79999994706265,
-13.8749089073543)) ;
#139590=CARTESIAN_POINT('Ctrl Pts',(4.47481046024546,-2.80007242131914,
-13.8533224277991)) ;
#139591=CARTESIAN_POINT('Ctrl Pts',(4.503281318764,-2.73353293829095,-13.85702587481)) ;
#139592=CARTESIAN_POINT('Ctrl Pts',(4.4547973699423,-2.79999997092221,-14.0250736654711)) ;
#139593=CARTESIAN_POINT('Ctrl Pts',(4.49869786247046,-2.80003603117402,
-14.0062792434958)) ;
#139594=CARTESIAN_POINT('Ctrl Pts',(4.52748687875414,-2.76348976047509,
-13.9962891728587)) ;
#139595=CARTESIAN_POINT('Ctrl Pts',(4.47221929614096,-2.79999997745988,
-14.0673040602233)) ;
#139596=CARTESIAN_POINT('Ctrl Pts',(4.50880556767621,-2.80002725736477,
-14.0482748482858)) ;
#139597=CARTESIAN_POINT('Ctrl Pts',(4.53619137795527,-2.77169834185704,
-14.0359836823676)) ;
#139598=CARTESIAN_POINT('Ctrl Pts',(4.50882352800136,-2.79999998605361,
-14.1242843496091)) ;
#139599=CARTESIAN_POINT('Ctrl Pts',(4.53367802911268,-2.80001636071785,
-14.1053587024204)) ;
#139600=CARTESIAN_POINT('Ctrl Pts',(4.55447319025662,-2.78248861123826,
-14.0900956814255)) ;
#139601=CARTESIAN_POINT('Ctrl Pts',(4.52308919141484,-2.79999998878206,
-14.1426625616911)) ;
#139602=CARTESIAN_POINT('Ctrl Pts',(4.54363962638622,-2.80001303821803,
-14.1237261501717)) ;
#139603=CARTESIAN_POINT('Ctrl Pts',(4.56159739427507,-2.78591449131413,
-14.1076542708947)) ;
#139604=CARTESIAN_POINT('Ctrl Pts',(4.57467506176495,-2.79999999510246,
-14.1856965083993)) ;
#139605=CARTESIAN_POINT('Ctrl Pts',(4.5806240530329,-2.80000557393877,-14.1663341632778)) ;
#139606=CARTESIAN_POINT('Ctrl Pts',(4.58735613403293,-2.79385049254303,
-14.1489198149933)) ;
#139607=CARTESIAN_POINT('Ctrl Pts',(4.62437069655636,-2.79999999703807,
-14.1995313430601)) ;
#139608=CARTESIAN_POINT('Ctrl Pts',(4.61827372661888,-2.80000334969057,
-14.1809340454876)) ;
#139609=CARTESIAN_POINT('Ctrl Pts',(4.61212682540743,-2.79628090446622,
-14.1624028142182)) ;
#139610=CARTESIAN_POINT('Ctrl Pts',(4.67161368302037,-2.79999998860619,
-14.1407898267653)) ;
#139611=CARTESIAN_POINT('Ctrl Pts',(4.6540701010264,-2.80001325705921,-14.1204637395888)) ;
#139612=CARTESIAN_POINT('Ctrl Pts',(4.63587130780614,-2.78569367459188,
-14.1056281295941)) ;
#139613=CARTESIAN_POINT('Ctrl Pts',(4.54879236204369,-2.8,-14.1635655563675)) ;
#139614=CARTESIAN_POINT('Ctrl Pts',(4.55448837802385,-2.7999999999815,-14.1611788209137)) ;
#139615=CARTESIAN_POINT('Ctrl Pts',(4.56021842726587,-2.79959150783241,
-14.1588395427342)) ;
#139616=CARTESIAN_POINT('Ctrl Pts',(4.56730671984965,-2.79865167182178,
-14.1559788838636)) ;
#139617=CARTESIAN_POINT('Ctrl Pts',(4.5684777095826,-2.79848295770259,-14.1555073268348)) ;
#139618=CARTESIAN_POINT('Ctrl Pts',(4.57107523099021,-2.79808046368154,
-14.154462962897)) ;
#139619=CARTESIAN_POINT('Ctrl Pts',(4.5725009361248,-2.79784058543152,-14.153889643028)) ;
#139620=CARTESIAN_POINT('Ctrl Pts',(4.5764383594612,-2.79713266293194,-14.1523136864649)) ;
#139621=CARTESIAN_POINT('Ctrl Pts',(4.57879956048961,-2.79666132938901,
-14.1513758003969)) ;
#139622=CARTESIAN_POINT('Ctrl Pts',(4.58293855712952,-2.79579586318667,
-14.1497608159296)) ;
#139623=CARTESIAN_POINT('Ctrl Pts',(4.58471363403686,-2.79540911153441,
-14.1490746171912)) ;
#139624=CARTESIAN_POINT('Ctrl Pts',(4.58699082729421,-2.7949269768198,-14.148244529262)) ;
#139625=CARTESIAN_POINT('Ctrl Pts',(4.58739952300692,-2.79484234870239,
-14.1481019268464)) ;
#139626=CARTESIAN_POINT('Ctrl Pts',(4.58871515235475,-2.79457617288697,
-14.1476611291009)) ;
#139627=CARTESIAN_POINT('Ctrl Pts',(4.58961690596118,-2.79440247805564,
-14.1473849869996)) ;
#139628=CARTESIAN_POINT('Ctrl Pts',(4.5910537506584,-2.79414748185769,-14.146982981818)) ;
#139629=CARTESIAN_POINT('Ctrl Pts',(4.59155303909532,-2.79406229662444,
-14.1468492435071)) ;
#139630=CARTESIAN_POINT('Ctrl Pts',(4.59245965385665,-2.79391282221553,
-14.1466125941148)) ;
#139631=CARTESIAN_POINT('Ctrl Pts',(4.59286388425101,-2.79384761399903,
-14.1465084217845)) ;
#139632=CARTESIAN_POINT('Ctrl Pts',(4.59368973959976,-2.79370598615372,
-14.1462676726517)) ;
#139633=CARTESIAN_POINT('Ctrl Pts',(4.59407665941116,-2.79363973714593,
-14.1461515212332)) ;
#139634=CARTESIAN_POINT('Ctrl Pts',(4.59444371287726,-2.79357284110656,
-14.1460267927279)) ;
#139635=CARTESIAN_POINT('Ctrl Pts',(4.59448890259156,-2.79356452972317,
-14.1460111581995)) ;
#139636=CARTESIAN_POINT('Ctrl Pts',(4.5947084233491,-2.79352377141065,-14.1459338254522)) ;
#139637=CARTESIAN_POINT('Ctrl Pts',(4.59483598733268,-2.79349361011835,
-14.1458723314841)) ;
#139638=CARTESIAN_POINT('Ctrl Pts',(4.59514620525223,-2.79342971313629,
-14.1457459400492)) ;
#139639=CARTESIAN_POINT('Ctrl Pts',(4.59533334275102,-2.79339696908415,
-14.1456838378534)) ;
#139640=CARTESIAN_POINT('Ctrl Pts',(4.59563785533348,-2.79335634095568,
-14.1456129903403)) ;
#139641=CARTESIAN_POINT('Ctrl Pts',(4.59571710962763,-2.79334654412181,
-14.1455963912877)) ;
#139642=CARTESIAN_POINT('Ctrl Pts',(4.59594411915585,-2.79332043135007,
-14.1455533496182)) ;
#139643=CARTESIAN_POINT('Ctrl Pts',(4.59600288191152,-2.79330503361987,
-14.1455339512408)) ;
#139644=CARTESIAN_POINT('Ctrl Pts',(4.59613307952173,-2.79327450473786,
-14.1454992805194)) ;
#139645=CARTESIAN_POINT('Ctrl Pts',(4.59620389659311,-2.79325970788819,
-14.1454850060586)) ;
#139646=CARTESIAN_POINT('Ctrl Pts',(4.59651192984771,-2.79322709231927,
-14.1454502778629)) ;
#139647=CARTESIAN_POINT('Ctrl Pts',(4.59679543741296,-2.79320989448354,
-14.1454293441824)) ;
#139648=CARTESIAN_POINT('Ctrl Pts',(4.59784475938524,-2.793166495242,-14.1453578835066)) ;
#139649=CARTESIAN_POINT('Ctrl Pts',(4.5987491506478,-2.79313948637392,-14.1452992643108)) ;
#139650=CARTESIAN_POINT('Ctrl Pts',(4.59999999999999,-2.79310344827586,
-14.1452063540422)) ;
#139651=CARTESIAN_POINT('Ctrl Pts',(4.5011795914298,-2.68531903459914,-16.8220290201724)) ;
#139652=CARTESIAN_POINT('Ctrl Pts',(4.51828670358959,-2.8,-16.8212138251408)) ;
#139653=CARTESIAN_POINT('Ctrl Pts',(4.4024095222558,-2.8,-16.8305883721109)) ;
#139654=CARTESIAN_POINT('Ctrl Pts',(4.49717774927194,-2.71005310920082,
-16.7229655323624)) ;
#139655=CARTESIAN_POINT('Ctrl Pts',(4.4857462854107,-2.8,-16.7373148520403)) ;
#139656=CARTESIAN_POINT('Ctrl Pts',(4.39431668173578,-2.8,-16.7163402695083)) ;
#139657=CARTESIAN_POINT('Ctrl Pts',(4.5032869068519,-2.73351987602557,-16.6229733978621)) ;
#139658=CARTESIAN_POINT('Ctrl Pts',(4.47485145549547,-2.8,-16.6266766957416)) ;
#139659=CARTESIAN_POINT('Ctrl Pts',(4.40646789472124,-2.8,-16.6051226186384)) ;
#139660=CARTESIAN_POINT('Ctrl Pts',(4.52749311797092,-2.76348183928883,
-16.4837129921594)) ;
#139661=CARTESIAN_POINT('Ctrl Pts',(4.49873206155793,-2.8,-16.4737330953069)) ;
#139662=CARTESIAN_POINT('Ctrl Pts',(4.4548681704377,-2.8,-16.4549566433661)) ;
#139663=CARTESIAN_POINT('Ctrl Pts',(4.53619745972496,-2.77169205010104,
-16.4440190471853)) ;
#139664=CARTESIAN_POINT('Ctrl Pts',(4.50883664816671,-2.8,-16.4317394381723)) ;
#139665=CARTESIAN_POINT('Ctrl Pts',(4.47227975612143,-2.8,-16.4127273846038)) ;
#139666=CARTESIAN_POINT('Ctrl Pts',(4.55447795090011,-2.78248459830341,
-16.3899078127333)) ;
#139667=CARTESIAN_POINT('Ctrl Pts',(4.53370055749884,-2.8,-16.3746579183699)) ;
#139668=CARTESIAN_POINT('Ctrl Pts',(4.50886586566856,-2.8,-16.3557478882722)) ;
#139669=CARTESIAN_POINT('Ctrl Pts',(4.56160154376425,-2.78591123334062,
-16.3723494428157)) ;
#139670=CARTESIAN_POINT('Ctrl Pts',(4.54365878772218,-2.8,-16.3562910664543)) ;
#139671=CARTESIAN_POINT('Ctrl Pts',(4.52312452397685,-2.8,-16.3373699954867)) ;
#139672=CARTESIAN_POINT('Ctrl Pts',(4.58735772267362,-2.79384903998488,
-16.3310842943985)) ;
#139673=CARTESIAN_POINT('Ctrl Pts',(4.58063087367386,-2.8,-16.3136839633808)) ;
#139674=CARTESIAN_POINT('Ctrl Pts',(4.57468550767191,-2.8,-16.2943374866056)) ;
#139675=CARTESIAN_POINT('Ctrl Pts',(4.61212536563479,-2.79628002040276,
-16.3176015865955)) ;
#139676=CARTESIAN_POINT('Ctrl Pts',(4.61826745782994,-2.80000000000002,
-16.2990848793757)) ;
#139677=CARTESIAN_POINT('Ctrl Pts',(4.62435992349573,-2.8,-16.2805015173211)) ;
#139678=CARTESIAN_POINT('Ctrl Pts',(4.63586710715927,-2.78569036914665,
-16.3743752946751)) ;
#139679=CARTESIAN_POINT('Ctrl Pts',(4.6540510694572,-2.79999999999994,-16.3595525238841)) ;
#139680=CARTESIAN_POINT('Ctrl Pts',(4.67158355065736,-2.8,-16.3392450797819)) ;
#139681=CARTESIAN_POINT('Ctrl Pts',(4.59999999999999,-2.79310344827586,
-16.3347936459578)) ;
#139682=CARTESIAN_POINT('Ctrl Pts',(4.59840954578222,-2.79314968944988,
-16.3346756726912)) ;
#139683=CARTESIAN_POINT('Ctrl Pts',(4.59737383489099,-2.7931815960622,-16.3346133239717)) ;
#139684=CARTESIAN_POINT('Ctrl Pts',(4.59650507521656,-2.79322931786012,
-16.33455037726)) ;
#139685=CARTESIAN_POINT('Ctrl Pts',(4.59632758424309,-2.79324472590582,
-16.3345345791767)) ;
#139686=CARTESIAN_POINT('Ctrl Pts',(4.5961184721085,-2.79327477162036,-16.3345047565773)) ;
#139687=CARTESIAN_POINT('Ctrl Pts',(4.5960648950493,-2.79328892979786,-16.3344910265853)) ;
#139688=CARTESIAN_POINT('Ctrl Pts',(4.59594601677698,-2.79331605564258,
-16.334459114495)) ;
#139689=CARTESIAN_POINT('Ctrl Pts',(4.59588597444861,-2.7933285533825,-16.3344426561835)) ;
#139690=CARTESIAN_POINT('Ctrl Pts',(4.59549967474365,-2.79337285752324,
-16.3343702787606)) ;
#139691=CARTESIAN_POINT('Ctrl Pts',(4.59527331486238,-2.7934062238596,-16.3343100807083)) ;
#139692=CARTESIAN_POINT('Ctrl Pts',(4.5949320123953,-2.79346950514991,-16.3341870402937)) ;
#139693=CARTESIAN_POINT('Ctrl Pts',(4.59480393230128,-2.79349821606423,
-16.334128474279)) ;
#139694=CARTESIAN_POINT('Ctrl Pts',(4.59460326813595,-2.79353924388982,
-16.3340476351491)) ;
#139695=CARTESIAN_POINT('Ctrl Pts',(4.59455075953096,-2.79354963432651,
-16.3340274276715)) ;
#139696=CARTESIAN_POINT('Ctrl Pts',(4.59417008680875,-2.79361944405452,
-16.3338955937176)) ;
#139697=CARTESIAN_POINT('Ctrl Pts',(4.59377742096551,-2.79368602572532,
-16.3337773461555)) ;
#139698=CARTESIAN_POINT('Ctrl Pts',(4.59289939109635,-2.7938335466559,-16.3335254190241)) ;
#139699=CARTESIAN_POINT('Ctrl Pts',(4.59245006584786,-2.79390305456781,
-16.333416036199)) ;
#139700=CARTESIAN_POINT('Ctrl Pts',(4.59099552519247,-2.79413629528603,
-16.3330568524094)) ;
#139701=CARTESIAN_POINT('Ctrl Pts',(4.59002197881598,-2.79430302757313,
-16.332806370176)) ;
#139702=CARTESIAN_POINT('Ctrl Pts',(4.58861122644696,-2.79456793455697,
-16.3323921365669)) ;
#139703=CARTESIAN_POINT('Ctrl Pts',(4.58817904894409,-2.79465210327451,
-16.3322585234305)) ;
#139704=CARTESIAN_POINT('Ctrl Pts',(4.58736872283366,-2.79481449815582,
-16.3319941835896)) ;
#139705=CARTESIAN_POINT('Ctrl Pts',(4.58699491219416,-2.79489135860974,
-16.3318665823581)) ;
#139706=CARTESIAN_POINT('Ctrl Pts',(4.58468897497187,-2.79537899446708,
-16.3310351906196)) ;
#139707=CARTESIAN_POINT('Ctrl Pts',(4.58290717718701,-2.79577019617636,
-16.3303420642284)) ;
#139708=CARTESIAN_POINT('Ctrl Pts',(4.57867627871774,-2.79666451416567,
-16.3286707882875)) ;
#139709=CARTESIAN_POINT('Ctrl Pts',(4.5762632155413,-2.79715040843617,-16.3276877651429)) ;
#139710=CARTESIAN_POINT('Ctrl Pts',(4.57243386308705,-2.79784156172336,
-16.3261367865103)) ;
#139711=CARTESIAN_POINT('Ctrl Pts',(4.57107519984216,-2.79807176647234,
-16.325584021445)) ;
#139712=CARTESIAN_POINT('Ctrl Pts',(4.56513452430521,-2.79900074294384,
-16.3231693903582)) ;
#139713=CARTESIAN_POINT('Ctrl Pts',(4.56062162665837,-2.79951267011368,
-16.3213309293498)) ;
#139714=CARTESIAN_POINT('Ctrl Pts',(4.5536542059673,-2.79992470862864,-16.3184610302787)) ;
#139715=CARTESIAN_POINT('Ctrl Pts',(4.55124660967315,-2.79999983267432,
-16.3174632392509)) ;
#139716=CARTESIAN_POINT('Ctrl Pts',(4.54880051362942,-2.79999999972164,
-16.3164378607329)) ;
#139717=CARTESIAN_POINT('Ctrl Pts',(4.54879236166274,-2.8,-14.1635655565152)) ;
#139718=CARTESIAN_POINT('Ctrl Pts',(4.5622387183224,-2.79999999999679,-14.1812315262749)) ;
#139719=CARTESIAN_POINT('Ctrl Pts',(4.57442182196495,-2.80939476060286,
-14.1972378204668)) ;
#139720=CARTESIAN_POINT('Ctrl Pts',(4.555568425176,-2.79999999999889,-14.1607250640488)) ;
#139721=CARTESIAN_POINT('Ctrl Pts',(4.56783337210912,-2.80040661803736,
-14.1761863015518)) ;
#139722=CARTESIAN_POINT('Ctrl Pts',(4.57961823522365,-2.80818164104597,
-14.1900183413273)) ;
#139723=CARTESIAN_POINT('Ctrl Pts',(4.56238982831618,-2.7994260255176,-14.1579528515171)) ;
#139724=CARTESIAN_POINT('Ctrl Pts',(4.5735781038818,-2.80014618986471,-14.1709310721412)) ;
#139725=CARTESIAN_POINT('Ctrl Pts',(4.58462643299473,-2.80630261261111,
-14.1825232711649)) ;
#139726=CARTESIAN_POINT('Ctrl Pts',(4.57328757735258,-2.7977370397245,-14.1535699979501)) ;
#139727=CARTESIAN_POINT('Ctrl Pts',(4.58237922839515,-2.79856394574987,
-14.1622664089314)) ;
#139728=CARTESIAN_POINT('Ctrl Pts',(4.59151541127591,-2.80237286596199,
-14.1700830028806)) ;
#139729=CARTESIAN_POINT('Ctrl Pts',(4.57700059755674,-2.7970371466716,-14.152076076342)) ;
#139730=CARTESIAN_POINT('Ctrl Pts',(4.58532305318674,-2.79784352093717,
-14.1592625430044)) ;
#139731=CARTESIAN_POINT('Ctrl Pts',(4.59370961102545,-2.80088045369937,
-14.1657455141894)) ;
#139732=CARTESIAN_POINT('Ctrl Pts',(4.58319893207066,-2.79574016930783,
-14.1496546705211)) ;
#139733=CARTESIAN_POINT('Ctrl Pts',(4.5899041610924,-2.79637293360539,-14.1543303545622)) ;
#139734=CARTESIAN_POINT('Ctrl Pts',(4.59665800356694,-2.79825577077759,
-14.1585819448697)) ;
#139735=CARTESIAN_POINT('Ctrl Pts',(4.58534994317985,-2.79526732601294,
-14.1488188618872)) ;
#139736=CARTESIAN_POINT('Ctrl Pts',(4.59144552977843,-2.79581844972913,
-14.1526200366107)) ;
#139737=CARTESIAN_POINT('Ctrl Pts',(4.59758018705035,-2.79731769672696,
-14.1560885803939)) ;
#139738=CARTESIAN_POINT('Ctrl Pts',(4.58899927751307,-2.79450268149332,
-14.1475173012671)) ;
#139739=CARTESIAN_POINT('Ctrl Pts',(4.59386223202755,-2.79488630507105,
-14.1499495170303)) ;
#139740=CARTESIAN_POINT('Ctrl Pts',(4.59874684688641,-2.79582009356912,
-14.1521813652447)) ;
#139741=CARTESIAN_POINT('Ctrl Pts',(4.59026755692867,-2.79423885380164,
-14.14707439958)) ;
#139742=CARTESIAN_POINT('Ctrl Pts',(4.5946770606831,-2.79455862385202,-14.149040543336)) ;
#139743=CARTESIAN_POINT('Ctrl Pts',(4.59910266898802,-2.79530499526365,
-14.1508486399022)) ;
#139744=CARTESIAN_POINT('Ctrl Pts',(4.59257623319511,-2.79382131826659,
-14.14638413145)) ;
#139745=CARTESIAN_POINT('Ctrl Pts',(4.59605751036343,-2.79403163929513,
-14.1476227610336)) ;
#139746=CARTESIAN_POINT('Ctrl Pts',(4.59954701072604,-2.79449510806573,
-14.148765766817)) ;
#139747=CARTESIAN_POINT('Ctrl Pts',(4.593429769333,-2.79367543507711,-14.1461445374534)) ;
#139748=CARTESIAN_POINT('Ctrl Pts',(4.59655016100495,-2.79384713427256,
-14.1471348895303)) ;
#139749=CARTESIAN_POINT('Ctrl Pts',(4.59967640178298,-2.79421605292373,
-14.148050213937)) ;
#139750=CARTESIAN_POINT('Ctrl Pts',(4.59428414179641,-2.79346156087783,
-14.1457069361853)) ;
#139751=CARTESIAN_POINT('Ctrl Pts',(4.59704519451433,-2.79355469746529,
-14.146373635748)) ;
#139752=CARTESIAN_POINT('Ctrl Pts',(4.5998104157401,-2.79379877456676,-14.1469823712707)) ;
#139753=CARTESIAN_POINT('Ctrl Pts',(4.59432658472652,-2.7933916625364,-14.1455338181495)) ;
#139754=CARTESIAN_POINT('Ctrl Pts',(4.59708408719785,-2.79345234504014,
-14.1461090766463)) ;
#139755=CARTESIAN_POINT('Ctrl Pts',(4.59984563524625,-2.79366003518351,
-14.1466276543527)) ;
#139756=CARTESIAN_POINT('Ctrl Pts',(4.59537197237732,-2.79324260992761,
-14.1452872615939)) ;
#139757=CARTESIAN_POINT('Ctrl Pts',(4.59764722167536,-2.79326383513928,
-14.145620961855)) ;
#139758=CARTESIAN_POINT('Ctrl Pts',(4.59992475053754,-2.79338190759658,
-14.1459170306476)) ;
#139759=CARTESIAN_POINT('Ctrl Pts',(4.59364183392371,-2.79313407032025,
-14.1452844788451)) ;
#139760=CARTESIAN_POINT('Ctrl Pts',(4.59684754854894,-2.79327107597598,
-14.1456389310452)) ;
#139761=CARTESIAN_POINT('Ctrl Pts',(4.59996664298755,-2.79324102308607,
-14.1455617736815)) ;
#139762=CARTESIAN_POINT('Ctrl Pts',(4.59999999999999,-2.79310344827586,
-14.1452063540422)) ;
#139763=CARTESIAN_POINT('Ctrl Pts',(4.59999999999999,-2.79310344827586,
-14.1452063540422)) ;
#139764=CARTESIAN_POINT('Ctrl Pts',(4.59999999999999,-2.79310344827586,
-14.1452063540422)) ;
#139765=CARTESIAN_POINT('Origin',(4.54879236168542,-2.9,-14.1635655565161)) ;
#139766=CARTESIAN_POINT('Ctrl Pts',(4.39959973407451,-2.8,-15.3505922428027)) ;
#139767=CARTESIAN_POINT('Ctrl Pts',(4.49922290141874,-2.8,-15.3501052483316)) ;
#139768=CARTESIAN_POINT('Ctrl Pts',(4.49980764094185,-2.8996950427637,-15.3506080458952)) ;
#139769=CARTESIAN_POINT('Ctrl Pts',(4.40142712570759,-2.8,-15.1295338960075)) ;
#139770=CARTESIAN_POINT('Ctrl Pts',(4.50593622119642,-2.8,-15.126048013468)) ;
#139771=CARTESIAN_POINT('Ctrl Pts',(4.50067611734352,-2.90411960318532,
-15.1296502871252)) ;
#139772=CARTESIAN_POINT('Ctrl Pts',(4.39573539165433,-2.8,-14.9076225417887)) ;
#139773=CARTESIAN_POINT('Ctrl Pts',(4.49039105203438,-2.8,-14.926444866009)) ;
#139774=CARTESIAN_POINT('Ctrl Pts',(4.4979321089857,-2.89506044297337,-14.9065928350698)) ;
#139775=CARTESIAN_POINT('Ctrl Pts',(4.41164816536272,-2.8,-14.5944921486564)) ;
#139776=CARTESIAN_POINT('Ctrl Pts',(4.48203507549531,-2.8,-14.6030075383891)) ;
#139777=CARTESIAN_POINT('Ctrl Pts',(4.50604587949362,-2.86657833599726,
-14.601791633455)) ;
#139778=CARTESIAN_POINT('Ctrl Pts',(4.41940490599909,-2.8,-14.5021571319988)) ;
#139779=CARTESIAN_POINT('Ctrl Pts',(4.48133975791563,-2.8,-14.5133274637387)) ;
#139780=CARTESIAN_POINT('Ctrl Pts',(4.50997623336223,-2.85625883833129,
-14.5130646432391)) ;
#139781=CARTESIAN_POINT('Ctrl Pts',(4.44577434373642,-2.8,-14.3670206588259)) ;
#139782=CARTESIAN_POINT('Ctrl Pts',(4.49360122670476,-2.8,-14.3793305876678)) ;
#139783=CARTESIAN_POINT('Ctrl Pts',(4.52318558604181,-2.8389646555956,-14.3854850424376)) ;
#139784=CARTESIAN_POINT('Ctrl Pts',(4.45692583760033,-2.8,-14.3224768930528)) ;
#139785=CARTESIAN_POINT('Ctrl Pts',(4.49949391572662,-2.8,-14.3360543026461)) ;
#139786=CARTESIAN_POINT('Ctrl Pts',(4.5287634845838,-2.83289258157625,-14.3438029886043)) ;
#139787=CARTESIAN_POINT('Ctrl Pts',(4.50378503771657,-2.8,-14.2010759162583)) ;
#139788=CARTESIAN_POINT('Ctrl Pts',(4.52873519606809,-2.8,-14.2199253422749)) ;
#139789=CARTESIAN_POINT('Ctrl Pts',(4.55214466721901,-2.81552005845342,
-14.2312248698016)) ;
#139790=CARTESIAN_POINT('Ctrl Pts',(4.54714423790168,-2.8,-14.1222684950466)) ;
#139791=CARTESIAN_POINT('Ctrl Pts',(4.55761617337351,-2.80000000000013,
-14.1432065641883)) ;
#139792=CARTESIAN_POINT('Ctrl Pts',(4.57259584813406,-2.80338245043801,
-14.1612385951887)) ;
#139793=CARTESIAN_POINT('Ctrl Pts',(4.67762904165635,-2.8,-14.1314950447963)) ;
#139794=CARTESIAN_POINT('Ctrl Pts',(4.66093484724865,-2.79999999999969,
-14.1470670658377)) ;
#139795=CARTESIAN_POINT('Ctrl Pts',(4.64133868807401,-2.80368623369325,
-14.1646880063865)) ;
#139796=CARTESIAN_POINT('Origin',(4.4,-2.9,-15.2400000000038)) ;
#139797=CARTESIAN_POINT('Ctrl Pts',(4.72172783566991,-2.8000000024879,-16.3403629549132)) ;
#139798=CARTESIAN_POINT('Ctrl Pts',(4.69645430308101,-2.79999660525791,
-16.3270700473085)) ;
#139799=CARTESIAN_POINT('Ctrl Pts',(4.66463283185001,-2.80454824226955,
-16.3094903682925)) ;
#139800=CARTESIAN_POINT('Ctrl Pts',(4.55709227475149,-2.80000000030524,
-16.3759964363101)) ;
#139801=CARTESIAN_POINT('Ctrl Pts',(4.5639923747865,-2.79999958643654,-16.3539593792013)) ;
#139802=CARTESIAN_POINT('Ctrl Pts',(4.57729370999489,-2.80055804294511,
-16.335175905081)) ;
#139803=CARTESIAN_POINT('Ctrl Pts',(4.50667826286324,-2.80000000784871,
-16.2866146479982)) ;
#139804=CARTESIAN_POINT('Ctrl Pts',(4.5303738201498,-2.79998899178919,-16.2670846001166)) ;
#139805=CARTESIAN_POINT('Ctrl Pts',(4.55348183854634,-2.81434699509191,
-16.2559466041139)) ;
#139806=CARTESIAN_POINT('Ctrl Pts',(4.4569228015872,-2.80000001789831,-16.1576422182876)) ;
#139807=CARTESIAN_POINT('Ctrl Pts',(4.4993802926736,-2.79997354447563,-16.1440998880094)) ;
#139808=CARTESIAN_POINT('Ctrl Pts',(4.52864149761197,-2.83271033979001,
-16.13632906208)) ;
#139809=CARTESIAN_POINT('Ctrl Pts',(4.44554661086163,-2.80000002126189,
-16.1123774400141)) ;
#139810=CARTESIAN_POINT('Ctrl Pts',(4.49333665154847,-2.79996797963649,
-16.100096939874)) ;
#139811=CARTESIAN_POINT('Ctrl Pts',(4.52295544156353,-2.83885474437116,
-16.0939678582281)) ;
#139812=CARTESIAN_POINT('Ctrl Pts',(4.41903322104331,-2.8000000307772,-15.9758947975771)) ;
#139813=CARTESIAN_POINT('Ctrl Pts',(4.48100616080234,-2.7999509576918,-15.9647300040203)) ;
#139814=CARTESIAN_POINT('Ctrl Pts',(4.50969337368894,-2.85623179093868,
-15.9650696236088)) ;
#139815=CARTESIAN_POINT('Ctrl Pts',(4.41147189908668,-2.8000000363501,-15.8842415900433)) ;
#139816=CARTESIAN_POINT('Ctrl Pts',(4.48178828424042,-2.79993989905027,
-15.8757891492055)) ;
#139817=CARTESIAN_POINT('Ctrl Pts',(4.50589025525736,-2.86640526991131,
-15.8769681512009)) ;
#139818=CARTESIAN_POINT('Ctrl Pts',(4.39523119070916,-2.80000005228414,
-15.5631795198334)) ;
#139819=CARTESIAN_POINT('Ctrl Pts',(4.49033836345901,-2.799902616883,-15.5430741316609)) ;
#139820=CARTESIAN_POINT('Ctrl Pts',(4.49769757367179,-2.89547737952989,
-15.5643332157621)) ;
#139821=CARTESIAN_POINT('Ctrl Pts',(4.40178225889348,-2.80000005718968,
-15.3326239782844)) ;
#139822=CARTESIAN_POINT('Ctrl Pts',(4.50681341018172,-2.79988784121838,
-15.3370581988237)) ;
#139823=CARTESIAN_POINT('Ctrl Pts',(4.50092255053475,-2.90441958896084,
-15.3324406960384)) ;
#139824=CARTESIAN_POINT('Ctrl Pts',(4.39924589760303,-2.80000005405718,
-15.1030311688804)) ;
#139825=CARTESIAN_POINT('Ctrl Pts',(4.49795607191395,-2.79989746608213,
-15.1039229374963)) ;
#139826=CARTESIAN_POINT('Ctrl Pts',(4.49968270404899,-2.89870974459554,
-15.1030284945919)) ;
#139827=CARTESIAN_POINT('Origin',(4.54879236168626,-2.9,-16.3164344434846)) ;
#139828=CARTESIAN_POINT('Ctrl Pts',(4.57442492185553,-2.80939715119899,
-16.2827581068621)) ;
#139829=CARTESIAN_POINT('Ctrl Pts',(4.56210583156797,-2.7998961275033,-16.2989430617887)) ;
#139830=CARTESIAN_POINT('Ctrl Pts',(4.54850917782859,-2.80000109307748,
-16.316806493488)) ;
#139831=CARTESIAN_POINT('Ctrl Pts',(4.57959763980855,-2.80818914940071,
-16.2899453004955)) ;
#139832=CARTESIAN_POINT('Ctrl Pts',(4.56768008075466,-2.80031924975227,
-16.3039410457291)) ;
#139833=CARTESIAN_POINT('Ctrl Pts',(4.55527876038348,-2.79999229227378,
-16.3195899763868)) ;
#139834=CARTESIAN_POINT('Ctrl Pts',(4.58464248447265,-2.80630474344638,
-16.2974843126383)) ;
#139835=CARTESIAN_POINT('Ctrl Pts',(4.57346944634374,-2.80008318972136,
-16.3092012910521)) ;
#139836=CARTESIAN_POINT('Ctrl Pts',(4.56216307187797,-2.79941338753917,
-16.3223280915334)) ;
#139837=CARTESIAN_POINT('Ctrl Pts',(4.59159231899494,-2.80232720646228,
-16.3100563692959)) ;
#139838=CARTESIAN_POINT('Ctrl Pts',(4.58237910662986,-2.79850221241048,
-16.3179149362578)) ;
#139839=CARTESIAN_POINT('Ctrl Pts',(4.57321634584969,-2.79769868647539,
-16.3266644864947)) ;
#139840=CARTESIAN_POINT('Ctrl Pts',(4.59378564167737,-2.8008235544484,-16.3144145837655)) ;
#139841=CARTESIAN_POINT('Ctrl Pts',(4.58533966160573,-2.79778056279966,
-16.3209180694478)) ;
#139842=CARTESIAN_POINT('Ctrl Pts',(4.57696130093821,-2.79699227428058,
-16.3281320740362)) ;
#139843=CARTESIAN_POINT('Ctrl Pts',(4.59669734138576,-2.79821861236081,
-16.3215174469091)) ;
#139844=CARTESIAN_POINT('Ctrl Pts',(4.58989502505308,-2.79633072300511,
-16.325783702985)) ;
#139845=CARTESIAN_POINT('Ctrl Pts',(4.58314295739389,-2.79570785369251,
-16.3304789031814)) ;
#139846=CARTESIAN_POINT('Ctrl Pts',(4.59760632414569,-2.79728965034655,
-16.3239852466291)) ;
#139847=CARTESIAN_POINT('Ctrl Pts',(4.59142619397024,-2.79578507327359,
-16.3274678937229)) ;
#139848=CARTESIAN_POINT('Ctrl Pts',(4.58528630332435,-2.79524119148169,
-16.3312873783749)) ;
#139849=CARTESIAN_POINT('Ctrl Pts',(4.59875741430933,-2.79580683383092,
-16.327853004496)) ;
#139850=CARTESIAN_POINT('Ctrl Pts',(4.59383193680336,-2.79486773439435,
-16.3300980055339)) ;
#139851=CARTESIAN_POINT('Ctrl Pts',(4.58892874314203,-2.79448758877844,
-16.3325464730129)) ;
#139852=CARTESIAN_POINT('Ctrl Pts',(4.59910834609946,-2.79529718130591,
-16.3291714993015)) ;
#139853=CARTESIAN_POINT('Ctrl Pts',(4.59464343907619,-2.79454543406795,
-16.3309926958501)) ;
#139854=CARTESIAN_POINT('Ctrl Pts',(4.59019511689892,-2.79422790851556,
-16.3329746712091)) ;
#139855=CARTESIAN_POINT('Ctrl Pts',(4.59954688679868,-2.79449699552073,
-16.3312293846587)) ;
#139856=CARTESIAN_POINT('Ctrl Pts',(4.59601732089137,-2.79402779797775,
-16.3323863363518)) ;
#139857=CARTESIAN_POINT('Ctrl Pts',(4.59249627585273,-2.79381771894921,
-16.3336411141675)) ;
#139858=CARTESIAN_POINT('Ctrl Pts',(4.59967529310588,-2.79422450025963,
-16.3319354645612)) ;
#139859=CARTESIAN_POINT('Ctrl Pts',(4.59651100242294,-2.79384821317135,
-16.3328644108735)) ;
#139860=CARTESIAN_POINT('Ctrl Pts',(4.593352874124,-2.79367727499394,-16.3338714476574)) ;
#139861=CARTESIAN_POINT('Ctrl Pts',(4.59980981518572,-2.79380630943631,
-16.3330056452101)) ;
#139862=CARTESIAN_POINT('Ctrl Pts',(4.59701056623718,-2.79355888022806,
-16.3336249350365)) ;
#139863=CARTESIAN_POINT('Ctrl Pts',(4.59421559911326,-2.79346462438277,
-16.3343030289899)) ;
#139864=CARTESIAN_POINT('Ctrl Pts',(4.59984534134842,-2.79366726490194,
-16.3333646067489)) ;
#139865=CARTESIAN_POINT('Ctrl Pts',(4.59705039509825,-2.79345667046144,
-16.3338917393962)) ;
#139866=CARTESIAN_POINT('Ctrl Pts',(4.59425962044002,-2.79339574833516,
-16.3344765637043)) ;
#139867=CARTESIAN_POINT('Ctrl Pts',(4.59992484646001,-2.7933873519883,-16.33407980384)) ;
#139868=CARTESIAN_POINT('Ctrl Pts',(4.59761652863209,-2.79326682373741,
-16.334380589531)) ;
#139869=CARTESIAN_POINT('Ctrl Pts',(4.59531061070857,-2.79324678512396,
-16.3347204137335)) ;
#139870=CARTESIAN_POINT('Ctrl Pts',(4.59996721368508,-2.79324340897637,
-16.334436569794)) ;
#139871=CARTESIAN_POINT('Ctrl Pts',(4.59680854952869,-2.79327323421043,
-16.3343604778616)) ;
#139872=CARTESIAN_POINT('Ctrl Pts',(4.59356174266139,-2.79313094944461,
-16.3347234833207)) ;
#139873=CARTESIAN_POINT('Ctrl Pts',(4.59999999999999,-2.79310344827586,
-16.3347936459578)) ;
#139874=CARTESIAN_POINT('Ctrl Pts',(4.59999999999999,-2.79310344827586,
-16.3347936459578)) ;
#139875=CARTESIAN_POINT('Ctrl Pts',(4.59999999999999,-2.79310344827586,
-16.3347936459578)) ;
#139876=CARTESIAN_POINT('Origin',(8.6,4.09462794777298,-18.845)) ;
#139877=CARTESIAN_POINT('Origin',(8.6,4.09462794777298,-18.845)) ;
#139878=CARTESIAN_POINT('Origin',(8.6,4.09462794777298,-18.845)) ;
#139879=CARTESIAN_POINT('Origin',(8.6,4.09462794777298,-17.545)) ;
#139880=CARTESIAN_POINT('Origin',(8.6,4.09462794777298,-17.545)) ;
#139881=CARTESIAN_POINT('Origin',(8.6,4.09462794777298,-17.545)) ;
#139882=CARTESIAN_POINT('Origin',(8.6,3.95,-18.845)) ;
#139883=CARTESIAN_POINT('Origin',(8.6,3.95,-18.845)) ;
#139884=CARTESIAN_POINT('Origin',(8.6,4.09462794777298,-18.845)) ;
#139885=CARTESIAN_POINT('Origin',(7.25334304318326,5.40585602606554,-18.845)) ;
#139886=CARTESIAN_POINT('Origin',(7.25334304318326,5.40585602606554,-17.545)) ;
#139887=CARTESIAN_POINT('Origin',(7.25334304318326,5.40585602606554,-17.545)) ;
#139888=CARTESIAN_POINT('Origin',(8.6,5.40585602606554,-17.545)) ;
#139889=CARTESIAN_POINT('Origin',(8.6,3.95,-17.545)) ;
#139890=CARTESIAN_POINT('Origin',(8.6,3.95,-18.845)) ;
#139891=CARTESIAN_POINT('Origin',(8.6,3.95,-18.845)) ;
#139892=CARTESIAN_POINT('Origin',(7.25334304318326,5.40585602606554,-18.845)) ;
#139893=CARTESIAN_POINT('Origin',(7.25334304318326,5.40585602606554,-18.845)) ;
#139894=CARTESIAN_POINT('Origin',(7.25334304318326,5.40585602606554,-17.545)) ;
#139895=CARTESIAN_POINT('Origin',(7.25334304318326,5.40585602606554,-17.545)) ;
#139896=CARTESIAN_POINT('Origin',(8.6,3.95,-17.545)) ;
#139897=CARTESIAN_POINT('Origin',(8.6,3.95,-17.545)) ;
#139898=CARTESIAN_POINT('Origin',(7.36677829147199,4.5782099492339,-18.845)) ;
#139899=CARTESIAN_POINT('Origin',(7.36677829147199,4.5782099492339,-18.845)) ;
#139900=CARTESIAN_POINT('Origin',(7.25334304318326,5.40585602606554,-18.845)) ;
#139901=CARTESIAN_POINT('Ctrl Pts',(4.03523814377473,5.98727788898885,-18.845)) ;
#139902=CARTESIAN_POINT('Ctrl Pts',(4.03523814427722,5.98727788891385,-18.8994712801668)) ;
#139903=CARTESIAN_POINT('Ctrl Pts',(4.04195902792202,5.94024173112809,-18.945)) ;
#139904=CARTESIAN_POINT('Ctrl Pts',(4.05,5.88396692803319,-18.945)) ;
#139905=CARTESIAN_POINT('Origin',(4.05,6.08618232569815,-18.945)) ;
#139906=CARTESIAN_POINT('Origin',(4.05,6.08618232569815,-17.545)) ;
#139907=CARTESIAN_POINT('Origin',(4.05,6.08618232569815,-18.845)) ;
#139908=CARTESIAN_POINT('Origin',(7.25334304318326,5.40585602606554,-17.545)) ;
#139909=CARTESIAN_POINT('Ctrl Pts',(4.05,5.88396692803319,-17.445)) ;
#139910=CARTESIAN_POINT('Ctrl Pts',(4.04195902792202,5.94024173112809,-17.445)) ;
#139911=CARTESIAN_POINT('Ctrl Pts',(4.03523814427722,5.98727788891385,-17.4905287198332)) ;
#139912=CARTESIAN_POINT('Ctrl Pts',(4.03523814377473,5.98727788898885,-17.545)) ;
#139913=CARTESIAN_POINT('Origin',(6.94197060168454,4.79460933256464,-17.545)) ;
#139914=CARTESIAN_POINT('Origin',(7.36677829147199,4.5782099492339,-17.545)) ;
#139915=CARTESIAN_POINT('Origin',(7.27599715910381,4.4,-18.845)) ;
#139916=CARTESIAN_POINT('Origin',(7.27599715910381,4.6,-18.845)) ;
#139917=CARTESIAN_POINT('Ctrl Pts',(3.95,6.08618232569815,-18.845)) ;
#139918=CARTESIAN_POINT('Ctrl Pts',(3.95,6.,-18.845)) ;
#139919=CARTESIAN_POINT('Ctrl Pts',(4.03523814377473,5.98727788898885,-18.845)) ;
#139920=CARTESIAN_POINT('Ctrl Pts',(3.95,6.08618232225605,-18.9539425627718)) ;
#139921=CARTESIAN_POINT('Ctrl Pts',(3.95,5.99999999675454,-18.9083359403855)) ;
#139922=CARTESIAN_POINT('Ctrl Pts',(4.03523814427722,5.98727788891385,-18.8994712801668)) ;
#139923=CARTESIAN_POINT('Ctrl Pts',(3.95,5.9941162463882,-19.0449999967068)) ;
#139924=CARTESIAN_POINT('Ctrl Pts',(3.95,5.93865134487238,-18.9528138978372)) ;
#139925=CARTESIAN_POINT('Ctrl Pts',(4.04195902792202,5.94024173112809,-18.945)) ;
#139926=CARTESIAN_POINT('Ctrl Pts',(3.95,5.88396692803319,-19.045)) ;
#139927=CARTESIAN_POINT('Ctrl Pts',(3.95,5.8839669280332,-18.945)) ;
#139928=CARTESIAN_POINT('Ctrl Pts',(4.05,5.88396692803319,-18.945)) ;
#139929=CARTESIAN_POINT('Origin',(4.05,5.88396692803319,-19.045)) ;
#139930=CARTESIAN_POINT('Ctrl Pts',(3.95,5.88396692803319,-17.345)) ;
#139931=CARTESIAN_POINT('Ctrl Pts',(3.95,5.8839669280332,-17.445)) ;
#139932=CARTESIAN_POINT('Ctrl Pts',(4.05,5.88396692803319,-17.445)) ;
#139933=CARTESIAN_POINT('Ctrl Pts',(3.95,5.9941162463882,-17.3450000032932)) ;
#139934=CARTESIAN_POINT('Ctrl Pts',(3.95,5.93865134487238,-17.4371861021628)) ;
#139935=CARTESIAN_POINT('Ctrl Pts',(4.04195902792202,5.94024173112809,-17.445)) ;
#139936=CARTESIAN_POINT('Ctrl Pts',(3.95,6.08618232225605,-17.4360574372282)) ;
#139937=CARTESIAN_POINT('Ctrl Pts',(3.95,5.99999999675454,-17.4816640596145)) ;
#139938=CARTESIAN_POINT('Ctrl Pts',(4.03523814427722,5.98727788891385,-17.4905287198332)) ;
#139939=CARTESIAN_POINT('Ctrl Pts',(3.95,6.08618232569815,-17.545)) ;
#139940=CARTESIAN_POINT('Ctrl Pts',(3.95,6.,-17.545)) ;
#139941=CARTESIAN_POINT('Ctrl Pts',(4.03523814377473,5.98727788898885,-17.545)) ;
#139942=CARTESIAN_POINT('Origin',(4.05,5.88396692803319,-17.345)) ;
#139943=CARTESIAN_POINT('Origin',(7.27599715910381,4.4,-17.545)) ;
#139944=CARTESIAN_POINT('Origin',(7.27599715910381,4.6,-17.545)) ;
#139945=CARTESIAN_POINT('Origin',(3.95,4.6,-18.845)) ;
#139946=CARTESIAN_POINT('Origin',(4.05,4.6,-18.845)) ;
#139947=CARTESIAN_POINT('Origin',(4.05,3.75,-19.045)) ;
#139948=CARTESIAN_POINT('Origin',(4.05,4.6,-19.045)) ;
#139949=CARTESIAN_POINT('Origin',(4.05,5.40585602606554,-17.345)) ;
#139950=CARTESIAN_POINT('Origin',(4.05,4.6,-17.345)) ;
#139951=CARTESIAN_POINT('Origin',(7.25334304318326,4.6,-17.545)) ;
#139952=CARTESIAN_POINT('Origin',(4.05,4.6,-17.545)) ;
#139953=CARTESIAN_POINT('Origin',(4.05,4.6,-18.845)) ;
#139954=CARTESIAN_POINT('Origin',(4.05,4.4,-18.845)) ;
#139955=CARTESIAN_POINT('Origin',(4.05,4.6,-17.545)) ;
#139956=CARTESIAN_POINT('Origin',(4.05,4.4,-17.545)) ;
#139957=CARTESIAN_POINT('Origin',(4.05,4.4,-17.78)) ;
#139958=CARTESIAN_POINT('Origin',(4.6,2.65,-11.6530460421716)) ;
#139959=CARTESIAN_POINT('',(4.5,2.61712020253893,-11.4557672574052)) ;
#139960=CARTESIAN_POINT('',(4.5,2.72431432344521,-11.467365183355)) ;
#139961=CARTESIAN_POINT('Origin',(4.5,2.65,-11.6530460421716)) ;
#139962=CARTESIAN_POINT('',(4.6,2.63356010126946,-11.5544066497884)) ;
#139963=CARTESIAN_POINT('Origin',(4.6,2.61712020253893,-11.4557672574052)) ;
#139964=CARTESIAN_POINT('',(4.6,2.68715716172261,-11.5602056127633)) ;
#139965=CARTESIAN_POINT('Origin',(4.6,2.65,-11.6530460421716)) ;
#139966=CARTESIAN_POINT('Origin',(4.6,2.72431432344521,-11.467365183355)) ;
#139967=CARTESIAN_POINT('Origin',(-4.52198039027186,10.1,-7.62)) ;
#139968=CARTESIAN_POINT('',(-4.42392232270277,10.0803883864862,-12.7)) ;
#139969=CARTESIAN_POINT('',(-4.52198039027186,10.2,-12.7)) ;
#139970=CARTESIAN_POINT('Origin',(-4.52198039027186,10.1,-12.7)) ;
#139971=CARTESIAN_POINT('',(-4.42392232270277,10.0803883864862,-7.62)) ;
#139972=CARTESIAN_POINT('',(-4.42392232270277,10.0803883864862,-12.7)) ;
#139973=CARTESIAN_POINT('',(-4.52198039027186,10.2,-7.62)) ;
#139974=CARTESIAN_POINT('Origin',(-4.52198039027186,10.1,-7.62)) ;
#139975=CARTESIAN_POINT('',(-4.52198039027186,10.2,-7.62)) ;
#139976=CARTESIAN_POINT('Origin',(0.,10.85,-10.16)) ;
#139977=CARTESIAN_POINT('',(-2.44929359829471E-16,10.95,-8.16)) ;
#139978=CARTESIAN_POINT('Origin',(0.,10.95,-10.16)) ;
#139979=CARTESIAN_POINT('',(-2.32682891837997E-16,10.85,-8.26)) ;
#139980=CARTESIAN_POINT('Origin',(-2.44929359829471E-16,10.85,-8.16)) ;
#139981=CARTESIAN_POINT('',(2.32682891837997E-16,10.85,-12.06)) ;
#139982=CARTESIAN_POINT('Origin',(0.,10.85,-10.16)) ;
#139983=CARTESIAN_POINT('Origin',(0.,10.85,-10.16)) ;
#139984=CARTESIAN_POINT('Origin',(11.0914213562373,0.,-10.16)) ;
#139985=CARTESIAN_POINT('',(11.0207106781187,-1.80110112442984E-16,-8.68928932188135)) ;
#139986=CARTESIAN_POINT('Origin',(11.0207106781187,0.,-10.16)) ;
#139987=CARTESIAN_POINT('',(11.0914213562373,-1.83697019872103E-16,-8.66)) ;
#139988=CARTESIAN_POINT('Origin',(11.0914213562373,-1.71450551880629E-16,
-8.76)) ;
#139989=CARTESIAN_POINT('Origin',(11.0914213562373,0.,-10.16)) ;
#139990=CARTESIAN_POINT('Origin',(12.7,0.,-10.16)) ;
#139991=CARTESIAN_POINT('',(12.8,-1.95943487863577E-16,-11.76)) ;
#139992=CARTESIAN_POINT('Origin',(12.8,0.,-10.16)) ;
#139993=CARTESIAN_POINT('',(12.7,-1.83697019872103E-16,-11.66)) ;
#139994=CARTESIAN_POINT('Origin',(12.7,-1.95943487863577E-16,-11.76)) ;
#139995=CARTESIAN_POINT('',(12.7,1.83697019872103E-16,-8.66)) ;
#139996=CARTESIAN_POINT('Origin',(12.7,0.,-10.16)) ;
#139997=CARTESIAN_POINT('Origin',(12.7,0.,-10.16)) ;
#139998=CARTESIAN_POINT('Origin',(12.7,2.1,-8.77804604217164)) ;
#139999=CARTESIAN_POINT('',(12.7,2.,-8.77804604217164)) ;
#140000=CARTESIAN_POINT('',(12.7,2.11643989873054,-8.67940664978842)) ;
#140001=CARTESIAN_POINT('Origin',(12.7,2.1,-8.77804604217164)) ;
#140002=CARTESIAN_POINT('',(12.8,2.13287979746107,-8.58076725740521)) ;
#140003=CARTESIAN_POINT('Origin',(12.7,2.13287979746107,-8.58076725740521)) ;
#140004=CARTESIAN_POINT('',(12.8,1.9,-8.77804604217164)) ;
#140005=CARTESIAN_POINT('Origin',(12.8,2.1,-8.77804604217164)) ;
#140006=CARTESIAN_POINT('Origin',(12.7,1.9,-8.77804604217164)) ;
#140007=CARTESIAN_POINT('Origin',(12.7,2.65,-8.66695395782836)) ;
#140008=CARTESIAN_POINT('',(12.7,2.63356010126947,-8.76559335021158)) ;
#140009=CARTESIAN_POINT('',(12.7,2.75,-8.66695395782836)) ;
#140010=CARTESIAN_POINT('Origin',(12.7,2.65,-8.66695395782836)) ;
#140011=CARTESIAN_POINT('',(12.8,2.65,-8.66695395782836)) ;
#140012=CARTESIAN_POINT('Origin',(12.7,2.65,-8.66695395782836)) ;
#140013=CARTESIAN_POINT('Origin',(12.7,2.65,-8.66695395782836)) ;
#140014=CARTESIAN_POINT('Origin',(4.5,2.1,-8.77804604217164)) ;
#140015=CARTESIAN_POINT('',(4.6,2.,-8.77804604217164)) ;
#140016=CARTESIAN_POINT('',(12.8,2.,-8.77804604217164)) ;
#140017=CARTESIAN_POINT('',(4.6,2.11643989873054,-8.67940664978842)) ;
#140018=CARTESIAN_POINT('Origin',(4.6,2.1,-8.77804604217164)) ;
#140019=CARTESIAN_POINT('',(4.5,2.11643989873054,-8.67940664978842)) ;
#140020=CARTESIAN_POINT('Origin',(12.7,2.65,-11.6530460421716)) ;
#140021=CARTESIAN_POINT('',(12.8,2.65,-11.6530460421716)) ;
#140022=CARTESIAN_POINT('',(12.7,2.63356010126947,-11.5544066497884)) ;
#140023=CARTESIAN_POINT('Origin',(12.7,2.65,-11.6530460421716)) ;
#140024=CARTESIAN_POINT('',(12.7,2.75,-11.6530460421716)) ;
#140025=CARTESIAN_POINT('Origin',(12.7,2.65,-11.6530460421716)) ;
#140026=CARTESIAN_POINT('Origin',(12.7,2.65,-11.6530460421716)) ;
#140027=CARTESIAN_POINT('Origin',(11.05,0.,-10.16)) ;
#140028=CARTESIAN_POINT('',(10.3,-9.1848509936051E-17,-9.41000000000001)) ;
#140029=CARTESIAN_POINT('Origin',(10.3,0.,-10.16)) ;
#140030=CARTESIAN_POINT('',(11.05,-1.83697019872103E-16,-8.66)) ;
#140031=CARTESIAN_POINT('Origin',(11.05,0.,-10.16)) ;
#140032=CARTESIAN_POINT('',(11.05,-1.83697019872103E-16,-8.66)) ;
#140033=CARTESIAN_POINT('Origin',(0.,9.95,-10.16)) ;
#140034=CARTESIAN_POINT('',(0.218101234104781,9.95,-12.0474405558009)) ;
#140035=CARTESIAN_POINT('',(-2.32682891837997E-16,9.95,-12.06)) ;
#140036=CARTESIAN_POINT('Origin',(0.,9.95,-10.16)) ;
#140037=CARTESIAN_POINT('',(0.321518176280636,9.85,-12.0325987456797)) ;
#140038=CARTESIAN_POINT('Ctrl Pts',(0.218101234104783,9.95,-12.0474405558009)) ;
#140039=CARTESIAN_POINT('Ctrl Pts',(0.231193919344581,9.95,-12.0459276441493)) ;
#140040=CARTESIAN_POINT('Ctrl Pts',(0.245192892440024,9.94751445938575,
-12.0441565825739)) ;
#140041=CARTESIAN_POINT('Ctrl Pts',(0.270990685773162,9.93716996065971,
-12.0406215789467)) ;
#140042=CARTESIAN_POINT('Ctrl Pts',(0.282791986325044,9.92931613918426,
-12.0388607093668)) ;
#140043=CARTESIAN_POINT('Ctrl Pts',(0.300953024019397,9.91135900604096,
-12.0360350266619)) ;
#140044=CARTESIAN_POINT('Ctrl Pts',(0.308688523153916,9.90025653083842,
-12.034762561801)) ;
#140045=CARTESIAN_POINT('Ctrl Pts',(0.318969164829205,9.87583423571802,
-12.0330429866749)) ;
#140046=CARTESIAN_POINT('Ctrl Pts',(0.321518176280638,9.86251584266313,
-12.0325987456797)) ;
#140047=CARTESIAN_POINT('Ctrl Pts',(0.321518176280638,9.85,-12.0325987456797)) ;
#140048=CARTESIAN_POINT('',(0.321518176280636,9.05,-12.0325987456797)) ;
#140049=CARTESIAN_POINT('',(0.321518176280636,8.95,-12.0325987456797)) ;
#140050=CARTESIAN_POINT('',(0.422455466606969,8.95,-12.0124393050068)) ;
#140051=CARTESIAN_POINT('Ctrl Pts',(0.321518176280627,9.05,-12.0325987456797)) ;
#140052=CARTESIAN_POINT('Ctrl Pts',(0.321518176280627,9.03744936090869,
-12.0325987456797)) ;
#140053=CARTESIAN_POINT('Ctrl Pts',(0.324085473150902,9.02409774280079,
-12.0321645622427)) ;
#140054=CARTESIAN_POINT('Ctrl Pts',(0.334387313650431,8.99960748025859,
-12.0303498579077)) ;
#140055=CARTESIAN_POINT('Ctrl Pts',(0.34212249945656,8.98846937989492,-12.0289656420615)) ;
#140056=CARTESIAN_POINT('Ctrl Pts',(0.360004521225388,8.97064401154629,
-12.0256049780795)) ;
#140057=CARTESIAN_POINT('Ctrl Pts',(0.371447108749463,8.96285745107738,
-12.0233820840476)) ;
#140058=CARTESIAN_POINT('Ctrl Pts',(0.39637397952969,8.95253508546271,-12.0182373032789)) ;
#140059=CARTESIAN_POINT('Ctrl Pts',(0.409857901997321,8.95,-12.0153122250646)) ;
#140060=CARTESIAN_POINT('Ctrl Pts',(0.422455466606959,8.95,-12.0124393050068)) ;
#140061=CARTESIAN_POINT('',(1.14750169623629,8.95,-11.6743446956142)) ;
#140062=CARTESIAN_POINT('Origin',(0.,8.95,-10.16)) ;
#140063=CARTESIAN_POINT('',(1.22782596331729,9.05,-11.609980483939)) ;
#140064=CARTESIAN_POINT('Ctrl Pts',(1.14750169623629,8.95,-11.6743446956142)) ;
#140065=CARTESIAN_POINT('Ctrl Pts',(1.15780003912542,8.95,-11.6665410786649)) ;
#140066=CARTESIAN_POINT('Ctrl Pts',(1.16870807732935,8.95253508546271,-11.6580919988207)) ;
#140067=CARTESIAN_POINT('Ctrl Pts',(1.18867189173408,8.96285745107738,-11.6423039093078)) ;
#140068=CARTESIAN_POINT('Ctrl Pts',(1.19772988083811,8.97064401154629,-11.6349672274615)) ;
#140069=CARTESIAN_POINT('Ctrl Pts',(1.21179864083581,8.98846937989492,-11.6234289972217)) ;
#140070=CARTESIAN_POINT('Ctrl Pts',(1.21783109328768,8.99960748025859,-11.6183932579134)) ;
#140071=CARTESIAN_POINT('Ctrl Pts',(1.22584313288946,9.02409774280079,-11.6116680597067)) ;
#140072=CARTESIAN_POINT('Ctrl Pts',(1.22782596331729,9.03744936090869,-11.609980483939)) ;
#140073=CARTESIAN_POINT('Ctrl Pts',(1.22782596331729,9.05,-11.609980483939)) ;
#140074=CARTESIAN_POINT('',(1.22782596331729,9.85,-11.609980483939)) ;
#140075=CARTESIAN_POINT('',(1.22782596331729,8.95,-11.609980483939)) ;
#140076=CARTESIAN_POINT('',(1.30567057854876,9.95,-11.5402986417121)) ;
#140077=CARTESIAN_POINT('Ctrl Pts',(1.22782596331729,9.85,-11.609980483939)) ;
#140078=CARTESIAN_POINT('Ctrl Pts',(1.22782596331729,9.85579162428539,-11.609980483939)) ;
#140079=CARTESIAN_POINT('Ctrl Pts',(1.22822745887818,9.86162764920014,-11.6096405714653)) ;
#140080=CARTESIAN_POINT('Ctrl Pts',(1.22902753823171,9.86736607146313,-11.6089619546779)) ;
#140081=CARTESIAN_POINT('Ctrl Pts',(1.22973095933685,9.87241123018668,-11.6083653221458)) ;
#140082=CARTESIAN_POINT('Ctrl Pts',(1.2307416875192,9.87738020477702,-11.6075074302535)) ;
#140083=CARTESIAN_POINT('Ctrl Pts',(1.23203099150182,9.88218322835582,-11.6064092214793)) ;
#140084=CARTESIAN_POINT('Ctrl Pts',(1.23351897101725,9.88772637473068,-11.6051417840233)) ;
#140085=CARTESIAN_POINT('Ctrl Pts',(1.23540145579029,9.89313280655105,-11.6035343365783)) ;
#140086=CARTESIAN_POINT('Ctrl Pts',(1.23763252770621,9.89827011881555,-11.6016189827484)) ;
#140087=CARTESIAN_POINT('Ctrl Pts',(1.23953000874362,9.90263929783465,-11.5999900134865)) ;
#140088=CARTESIAN_POINT('Ctrl Pts',(1.24167862345461,9.90681364346946,-11.5981390311988)) ;
#140089=CARTESIAN_POINT('Ctrl Pts',(1.24403025306866,9.91072825704926,-11.5961019216791)) ;
#140090=CARTESIAN_POINT('Ctrl Pts',(1.24687926059922,9.91547082513966,-11.5936339563467)) ;
#140091=CARTESIAN_POINT('Ctrl Pts',(1.25006974298105,9.91990270163235,-11.5908551265321)) ;
#140092=CARTESIAN_POINT('Ctrl Pts',(1.25351940932648,9.92391762881322,-11.5878266146309)) ;
#140093=CARTESIAN_POINT('Ctrl Pts',(1.2563462050552,9.92720762206752,-11.5853449298389)) ;
#140094=CARTESIAN_POINT('Ctrl Pts',(1.25934609941472,9.93021806933732,-11.5826963101588)) ;
#140095=CARTESIAN_POINT('Ctrl Pts',(1.26246241000316,9.93291206679729,-11.5799255837293)) ;
#140096=CARTESIAN_POINT('Ctrl Pts',(1.26649145911189,9.93639511117203,-11.5763433371803)) ;
#140097=CARTESIAN_POINT('Ctrl Pts',(1.27077652588473,9.93940081548805,-11.5725022625241)) ;
#140098=CARTESIAN_POINT('Ctrl Pts',(1.27520851369615,9.94185862744775,-11.5684896739102)) ;
#140099=CARTESIAN_POINT('Ctrl Pts',(1.27864718185096,9.94376558208659,-11.5653764070711)) ;
#140100=CARTESIAN_POINT('Ctrl Pts',(1.28217366418729,9.94534362661778,-11.5621604997622)) ;
#140101=CARTESIAN_POINT('Ctrl Pts',(1.28573335778226,9.94658081625577,-11.5588887492202)) ;
#140102=CARTESIAN_POINT('Ctrl Pts',(1.29026904082681,9.94815721599754,-11.5547199568612)) ;
#140103=CARTESIAN_POINT('Ctrl Pts',(1.29492021413415,9.9491996901822,-11.5504036518226)) ;
#140104=CARTESIAN_POINT('Ctrl Pts',(1.29957290046263,9.9496832238817,-11.5460412243876)) ;
#140105=CARTESIAN_POINT('Ctrl Pts',(1.30160833994475,9.94989475836165,-11.5441327662599)) ;
#140106=CARTESIAN_POINT('Ctrl Pts',(1.30364403319562,9.95,-11.5422156186355)) ;
#140107=CARTESIAN_POINT('Ctrl Pts',(1.30567057854874,9.95,-11.5402986417121)) ;
#140108=CARTESIAN_POINT('',(-0.218101234104782,9.95,-8.27255944419911)) ;
#140109=CARTESIAN_POINT('Origin',(0.,9.95,-10.16)) ;
#140110=CARTESIAN_POINT('',(-0.321518176280637,9.85,-8.2874012543203)) ;
#140111=CARTESIAN_POINT('Ctrl Pts',(-0.218101234104781,9.95,-8.27255944419911)) ;
#140112=CARTESIAN_POINT('Ctrl Pts',(-0.231193919344579,9.95,-8.2740723558507)) ;
#140113=CARTESIAN_POINT('Ctrl Pts',(-0.245192892440022,9.94751445938575,
-8.27584341742608)) ;
#140114=CARTESIAN_POINT('Ctrl Pts',(-0.270990685773159,9.93716996065971,
-8.27937842105327)) ;
#140115=CARTESIAN_POINT('Ctrl Pts',(-0.282791986325042,9.92931613918426,
-8.28113929063325)) ;
#140116=CARTESIAN_POINT('Ctrl Pts',(-0.300953024019395,9.91135900604096,
-8.28396497333807)) ;
#140117=CARTESIAN_POINT('Ctrl Pts',(-0.308688523153914,9.90025653083842,
-8.28523743819905)) ;
#140118=CARTESIAN_POINT('Ctrl Pts',(-0.318969164829202,9.87583423571802,
-8.28695701332505)) ;
#140119=CARTESIAN_POINT('Ctrl Pts',(-0.321518176280635,9.86251584266313,
-8.2874012543203)) ;
#140120=CARTESIAN_POINT('Ctrl Pts',(-0.321518176280635,9.85,-8.2874012543203)) ;
#140121=CARTESIAN_POINT('',(-0.321518176280637,9.05,-8.2874012543203)) ;
#140122=CARTESIAN_POINT('',(-0.321518176280637,8.95,-8.2874012543203)) ;
#140123=CARTESIAN_POINT('',(-0.422455466606969,8.95,-8.30756069499325)) ;
#140124=CARTESIAN_POINT('Ctrl Pts',(-0.321518176280636,9.05,-8.2874012543203)) ;
#140125=CARTESIAN_POINT('Ctrl Pts',(-0.321518176280636,9.03744936090869,
-8.2874012543203)) ;
#140126=CARTESIAN_POINT('Ctrl Pts',(-0.324085473150912,9.02409774280079,
-8.28783543775733)) ;
#140127=CARTESIAN_POINT('Ctrl Pts',(-0.334387313650441,8.99960748025859,
-8.28965014209231)) ;
#140128=CARTESIAN_POINT('Ctrl Pts',(-0.342122499456568,8.98846937989492,
-8.29103435793852)) ;
#140129=CARTESIAN_POINT('Ctrl Pts',(-0.360004521225397,8.97064401154629,
-8.29439502192046)) ;
#140130=CARTESIAN_POINT('Ctrl Pts',(-0.371447108749471,8.96285745107738,
-8.29661791595238)) ;
#140131=CARTESIAN_POINT('Ctrl Pts',(-0.396373979529699,8.95253508546271,
-8.30176269672111)) ;
#140132=CARTESIAN_POINT('Ctrl Pts',(-0.409857901997331,8.95,-8.30468777493541)) ;
#140133=CARTESIAN_POINT('Ctrl Pts',(-0.422455466606968,8.95,-8.30756069499325)) ;
#140134=CARTESIAN_POINT('',(-1.14750169623629,8.95,-8.64565530438581)) ;
#140135=CARTESIAN_POINT('Origin',(0.,8.95,-10.16)) ;
#140136=CARTESIAN_POINT('',(-1.22782596331729,9.05,-8.710019516061)) ;
#140137=CARTESIAN_POINT('Ctrl Pts',(-1.1475016962363,8.95,-8.64565530438581)) ;
#140138=CARTESIAN_POINT('Ctrl Pts',(-1.15780003912543,8.95,-8.65345892133506)) ;
#140139=CARTESIAN_POINT('Ctrl Pts',(-1.16870807732935,8.95253508546271,
-8.66190800117932)) ;
#140140=CARTESIAN_POINT('Ctrl Pts',(-1.18867189173409,8.96285745107738,
-8.67769609069216)) ;
#140141=CARTESIAN_POINT('Ctrl Pts',(-1.19772988083812,8.97064401154629,
-8.68503277253852)) ;
#140142=CARTESIAN_POINT('Ctrl Pts',(-1.21179864083582,8.98846937989492,
-8.69657100277835)) ;
#140143=CARTESIAN_POINT('Ctrl Pts',(-1.21783109328768,8.99960748025859,
-8.70160674208656)) ;
#140144=CARTESIAN_POINT('Ctrl Pts',(-1.22584313288947,9.02409774280079,
-8.70833194029334)) ;
#140145=CARTESIAN_POINT('Ctrl Pts',(-1.22782596331729,9.03744936090869,
-8.71001951606101)) ;
#140146=CARTESIAN_POINT('Ctrl Pts',(-1.22782596331729,9.05,-8.71001951606101)) ;
#140147=CARTESIAN_POINT('',(-1.22782596331729,9.85,-8.710019516061)) ;
#140148=CARTESIAN_POINT('',(-1.22782596331729,8.95,-8.710019516061)) ;
#140149=CARTESIAN_POINT('',(-1.30567057854876,9.95,-8.77970135828795)) ;
#140150=CARTESIAN_POINT('Ctrl Pts',(-1.22782596331729,9.85,-8.710019516061)) ;
#140151=CARTESIAN_POINT('Ctrl Pts',(-1.22782596331729,9.8557916242854,-8.710019516061)) ;
#140152=CARTESIAN_POINT('Ctrl Pts',(-1.22822745887816,9.86162764920014,
-8.71035942853478)) ;
#140153=CARTESIAN_POINT('Ctrl Pts',(-1.22902753823169,9.86736607146313,
-8.71103804532216)) ;
#140154=CARTESIAN_POINT('Ctrl Pts',(-1.22973095933683,9.87241123018669,
-8.71163467785421)) ;
#140155=CARTESIAN_POINT('Ctrl Pts',(-1.23074168751919,9.87738020477703,
-8.71249256974653)) ;
#140156=CARTESIAN_POINT('Ctrl Pts',(-1.23203099150182,9.88218322835582,
-8.71359077852072)) ;
#140157=CARTESIAN_POINT('Ctrl Pts',(-1.23351897101725,9.88772637473068,
-8.71485821597665)) ;
#140158=CARTESIAN_POINT('Ctrl Pts',(-1.2354014557903,9.89313280655103,-8.71646566342165)) ;
#140159=CARTESIAN_POINT('Ctrl Pts',(-1.23763252770622,9.89827011881554,
-8.71838101725154)) ;
#140160=CARTESIAN_POINT('Ctrl Pts',(-1.23953000874363,9.90263929783464,
-8.72000998651346)) ;
#140161=CARTESIAN_POINT('Ctrl Pts',(-1.24167862345459,9.90681364346946,
-8.72186096880123)) ;
#140162=CARTESIAN_POINT('Ctrl Pts',(-1.24403025306866,9.91072825704926,
-8.72389807832091)) ;
#140163=CARTESIAN_POINT('Ctrl Pts',(-1.24687926059923,9.91547082513966,
-8.72636604365333)) ;
#140164=CARTESIAN_POINT('Ctrl Pts',(-1.25006974298105,9.91990270163234,
-8.72914487346783)) ;
#140165=CARTESIAN_POINT('Ctrl Pts',(-1.25351940932649,9.92391762881322,
-8.73217338536911)) ;
#140166=CARTESIAN_POINT('Ctrl Pts',(-1.25634620505522,9.92720762206752,
-8.7346550701611)) ;
#140167=CARTESIAN_POINT('Ctrl Pts',(-1.25934609941473,9.93021806933732,
-8.73730368984121)) ;
#140168=CARTESIAN_POINT('Ctrl Pts',(-1.26246241000317,9.93291206679729,
-8.74007441627068)) ;
#140169=CARTESIAN_POINT('Ctrl Pts',(-1.26649145911191,9.93639511117205,
-8.74365666281975)) ;
#140170=CARTESIAN_POINT('Ctrl Pts',(-1.27077652588473,9.93940081548806,
-8.74749773747593)) ;
#140171=CARTESIAN_POINT('Ctrl Pts',(-1.27520851369618,9.94185862744776,
-8.7515103260898)) ;
#140172=CARTESIAN_POINT('Ctrl Pts',(-1.27864718185098,9.9437655820866,-8.75462359292894)) ;
#140173=CARTESIAN_POINT('Ctrl Pts',(-1.2821736641873,9.94534362661778,-8.75783950023776)) ;
#140174=CARTESIAN_POINT('Ctrl Pts',(-1.28573335778226,9.94658081625577,
-8.76111125077976)) ;
#140175=CARTESIAN_POINT('Ctrl Pts',(-1.29026904082682,9.94815721599755,
-8.76528004313887)) ;
#140176=CARTESIAN_POINT('Ctrl Pts',(-1.29492021413418,9.94919969018221,
-8.7695963481774)) ;
#140177=CARTESIAN_POINT('Ctrl Pts',(-1.2995729004627,9.94968322388171,-8.77395877561253)) ;
#140178=CARTESIAN_POINT('Ctrl Pts',(-1.30160833994481,9.94989475836166,
-8.77586723374024)) ;
#140179=CARTESIAN_POINT('Ctrl Pts',(-1.30364403319567,9.95,-8.7777843813645)) ;
#140180=CARTESIAN_POINT('Ctrl Pts',(-1.30567057854876,9.95,-8.77970135828795)) ;
#140181=CARTESIAN_POINT('Origin',(0.,9.95,-10.16)) ;
#140182=CARTESIAN_POINT('',(-2.32682891837997E-16,9.95,-12.06)) ;
#140183=CARTESIAN_POINT('Origin',(4.5,-2.8,-7.62)) ;
#140184=CARTESIAN_POINT('',(4.5,-2.4,-12.1221416870349)) ;
#140185=CARTESIAN_POINT('',(4.5,-2.7,-11.6831546211728)) ;
#140186=CARTESIAN_POINT('Origin',(4.5,0.,-10.16)) ;
#140187=CARTESIAN_POINT('',(4.5,-2.7,-12.7)) ;
#140188=CARTESIAN_POINT('',(4.5,-2.7,-7.62)) ;
#140189=CARTESIAN_POINT('',(4.5,-2.4,-12.7)) ;
#140190=CARTESIAN_POINT('',(4.5,-2.8,-12.7)) ;
#140191=CARTESIAN_POINT('',(4.5,-2.4,-12.0861360284258)) ;
#140192=CARTESIAN_POINT('Origin',(4.5,-2.3,-7.62)) ;
#140193=CARTESIAN_POINT('',(4.6,-2.3,-7.62)) ;
#140194=CARTESIAN_POINT('',(12.7,-2.3,-7.62)) ;
#140195=CARTESIAN_POINT('',(4.5,-2.3,-7.62)) ;
#140196=CARTESIAN_POINT('',(4.6,-2.3,-8.19785831296514)) ;
#140197=CARTESIAN_POINT('',(4.6,-2.3,-8.23386397157418)) ;
#140198=CARTESIAN_POINT('',(12.7,-2.3,-8.19785831296514)) ;
#140199=CARTESIAN_POINT('',(4.5,-2.3,-8.19785831296514)) ;
#140200=CARTESIAN_POINT('',(12.7,-2.3,-7.62)) ;
#140201=CARTESIAN_POINT('Origin',(12.8,2.75,-7.62)) ;
#140202=CARTESIAN_POINT('',(12.7,2.75,-12.7)) ;
#140203=CARTESIAN_POINT('',(4.55912712210514,2.75,-12.7)) ;
#140204=CARTESIAN_POINT('',(12.8,2.75,-12.7)) ;
#140205=CARTESIAN_POINT('',(4.55912712210513,2.75,-11.6530460421716)) ;
#140206=CARTESIAN_POINT('',(4.55912712210514,2.75,-11.6530460421716)) ;
#140207=CARTESIAN_POINT('',(12.8,2.75,-11.6530460421716)) ;
#140208=CARTESIAN_POINT('',(12.7,2.75,-7.62)) ;
#140209=CARTESIAN_POINT('Origin',(0.,9.95,-10.16)) ;
#140210=CARTESIAN_POINT('',(0.230887397576971,9.95,-12.0748605718538)) ;
#140211=CARTESIAN_POINT('Origin',(12.8,-2.3,-7.62)) ;
#140212=CARTESIAN_POINT('',(12.8,-2.3359925337019,-7.83595520221138)) ;
#140213=CARTESIAN_POINT('',(12.8,2.65,-7.62)) ;
#140214=CARTESIAN_POINT('',(12.8,2.65,-7.62)) ;
#140215=CARTESIAN_POINT('',(12.8,-2.2,-7.62)) ;
#140216=CARTESIAN_POINT('',(12.8,-2.3,-7.62)) ;
#140217=CARTESIAN_POINT('',(12.8,-2.2,-8.19785831296514)) ;
#140218=CARTESIAN_POINT('',(12.8,-2.2,-7.62)) ;
#140219=CARTESIAN_POINT('',(12.8,-2.24516129032258,-8.32444809922546)) ;
#140220=CARTESIAN_POINT('Origin',(12.8,-2.4,-8.19785831296514)) ;
#140221=CARTESIAN_POINT('',(12.8,-2.24516129032258,-11.9955519007745)) ;
#140222=CARTESIAN_POINT('Origin',(12.8,0.,-10.16)) ;
#140223=CARTESIAN_POINT('',(12.8,-2.2,-12.1221416870349)) ;
#140224=CARTESIAN_POINT('Origin',(12.8,-2.4,-12.1221416870349)) ;
#140225=CARTESIAN_POINT('',(12.8,-2.2,-12.7)) ;
#140226=CARTESIAN_POINT('',(12.8,-2.2,-7.62)) ;
#140227=CARTESIAN_POINT('',(12.8,2.65,-12.7)) ;
#140228=CARTESIAN_POINT('',(12.8,-2.3,-12.7)) ;
#140229=CARTESIAN_POINT('',(12.8,2.65,-7.62)) ;
#140230=CARTESIAN_POINT('',(12.8,2.13287979746107,-11.7392327425948)) ;
#140231=CARTESIAN_POINT('',(12.8,-1.51220874991811,-12.3467475004913)) ;
#140232=CARTESIAN_POINT('',(12.8,1.9,-11.5419539578284)) ;
#140233=CARTESIAN_POINT('Origin',(12.8,2.1,-11.5419539578284)) ;
#140234=CARTESIAN_POINT('',(12.8,1.9,-7.62)) ;
#140235=CARTESIAN_POINT('Origin',(12.8,2.75,-7.62)) ;
#140236=CARTESIAN_POINT('',(4.55912712210513,2.75,-8.66695395782836)) ;
#140237=CARTESIAN_POINT('',(12.8,2.75,-8.66695395782836)) ;
#140238=CARTESIAN_POINT('',(4.55912712210514,2.75,-7.62)) ;
#140239=CARTESIAN_POINT('',(4.55912712210514,2.75,-7.62)) ;
#140240=CARTESIAN_POINT('',(12.7,2.75,-7.62)) ;
#140241=CARTESIAN_POINT('',(12.8,2.75,-7.62)) ;
#140242=CARTESIAN_POINT('',(12.7,2.75,-7.62)) ;
#140243=CARTESIAN_POINT('Origin',(4.5,2.75,-7.62)) ;
#140244=CARTESIAN_POINT('',(4.47150553123747,2.80180812502278,-7.62)) ;
#140245=CARTESIAN_POINT('',(3.96237840913234,3.72749380157757,-7.62)) ;
#140246=CARTESIAN_POINT('',(4.5,2.75,-7.62)) ;
#140247=CARTESIAN_POINT('',(4.47150553123747,2.80180812502279,-8.66695395782836)) ;
#140248=CARTESIAN_POINT('',(4.47150553123747,2.80180812502278,-8.66695395782836)) ;
#140249=CARTESIAN_POINT('',(4.48762159086767,2.77250619842243,-8.77117568174948)) ;
#140250=CARTESIAN_POINT('Origin',(4.56263299594785,2.6361218255494,-8.67660029409629)) ;
#140251=CARTESIAN_POINT('',(4.48762159086767,2.77250619842243,-11.5488243182478)) ;
#140252=CARTESIAN_POINT('',(4.48762159086767,2.77250619842243,-7.62)) ;
#140253=CARTESIAN_POINT('',(4.47150553123747,2.80180812502279,-11.6530460421716)) ;
#140254=CARTESIAN_POINT('Origin',(4.56263299596657,2.63612182551533,-11.6433997058941)) ;
#140255=CARTESIAN_POINT('',(4.47150553123747,2.80180812502278,-12.7)) ;
#140256=CARTESIAN_POINT('',(4.47150553123747,2.80180812502278,-12.7)) ;
#140257=CARTESIAN_POINT('',(3.96237840913234,3.72749380157757,-12.7)) ;
#140258=CARTESIAN_POINT('',(4.5,2.75,-12.7)) ;
#140259=CARTESIAN_POINT('',(3.96237840913234,3.72749380157757,-7.62)) ;
#140260=CARTESIAN_POINT('Origin',(3.95,3.75,-7.62)) ;
#140261=CARTESIAN_POINT('',(3.95,3.77568567655479,-12.7)) ;
#140262=CARTESIAN_POINT('',(3.95,6.92431432344521,-12.7)) ;
#140263=CARTESIAN_POINT('',(3.95,3.75,-12.7)) ;
#140264=CARTESIAN_POINT('',(3.95,6.92431432344521,-7.62)) ;
#140265=CARTESIAN_POINT('',(3.95,6.92431432344521,-7.62)) ;
#140266=CARTESIAN_POINT('',(3.95,3.77568567655479,-7.62)) ;
#140267=CARTESIAN_POINT('',(3.95,3.75,-7.62)) ;
#140268=CARTESIAN_POINT('',(3.95,3.77568567655479,-12.7)) ;
#140269=CARTESIAN_POINT('Origin',(3.95,6.95,-7.62)) ;
#140270=CARTESIAN_POINT('',(3.93762159086767,6.97250619842243,-12.7)) ;
#140271=CARTESIAN_POINT('',(3.42849446876253,7.89819187497721,-12.7)) ;
#140272=CARTESIAN_POINT('',(3.95,6.95,-12.7)) ;
#140273=CARTESIAN_POINT('',(3.42849446876253,7.89819187497721,-7.62)) ;
#140274=CARTESIAN_POINT('',(3.42849446876253,7.89819187497721,-7.62)) ;
#140275=CARTESIAN_POINT('',(3.93762159086767,6.97250619842243,-7.62)) ;
#140276=CARTESIAN_POINT('',(3.95,6.95,-7.62)) ;
#140277=CARTESIAN_POINT('',(3.93762159086767,6.97250619842243,-7.62)) ;
#140278=CARTESIAN_POINT('Origin',(3.4,7.95,-7.62)) ;
#140279=CARTESIAN_POINT('',(3.34087287789487,7.95,-12.7)) ;
#140280=CARTESIAN_POINT('',(3.,7.95,-12.7)) ;
#140281=CARTESIAN_POINT('',(3.4,7.95,-12.7)) ;
#140282=CARTESIAN_POINT('',(3.,7.95,-7.62)) ;
#140283=CARTESIAN_POINT('',(3.,7.95,-7.62)) ;
#140284=CARTESIAN_POINT('',(3.34087287789487,7.95,-7.62)) ;
#140285=CARTESIAN_POINT('',(3.4,7.95,-7.62)) ;
#140286=CARTESIAN_POINT('',(3.34087287789487,7.95,-7.62)) ;
#140287=CARTESIAN_POINT('Origin',(2.9,7.95,-7.62)) ;
#140288=CARTESIAN_POINT('',(2.9,8.05,-12.7)) ;
#140289=CARTESIAN_POINT('',(2.9,9.85,-12.7)) ;
#140290=CARTESIAN_POINT('',(2.9,7.95,-12.7)) ;
#140291=CARTESIAN_POINT('',(2.9,9.85,-7.62)) ;
#140292=CARTESIAN_POINT('',(2.9,9.85,-7.62)) ;
#140293=CARTESIAN_POINT('',(2.9,8.05,-7.62)) ;
#140294=CARTESIAN_POINT('',(2.9,7.95,-7.62)) ;
#140295=CARTESIAN_POINT('',(2.9,8.05,-12.7)) ;
#140296=CARTESIAN_POINT('Origin',(2.9,9.95,-7.62)) ;
#140297=CARTESIAN_POINT('',(3.,9.95,-12.7)) ;
#140298=CARTESIAN_POINT('',(3.3,9.95,-12.7)) ;
#140299=CARTESIAN_POINT('',(2.9,9.95,-12.7)) ;
#140300=CARTESIAN_POINT('',(3.3,9.95,-7.62)) ;
#140301=CARTESIAN_POINT('',(3.3,9.95,-7.62)) ;
#140302=CARTESIAN_POINT('',(3.,9.95,-7.62)) ;
#140303=CARTESIAN_POINT('',(2.9,9.95,-7.62)) ;
#140304=CARTESIAN_POINT('',(3.,9.95,-12.7)) ;
#140305=CARTESIAN_POINT('Origin',(3.4,9.95,-7.62)) ;
#140306=CARTESIAN_POINT('',(3.4,10.05,-12.7)) ;
#140307=CARTESIAN_POINT('',(3.4,10.85,-12.7)) ;
#140308=CARTESIAN_POINT('',(3.4,9.95,-12.7)) ;
#140309=CARTESIAN_POINT('',(3.4,10.85,-7.62)) ;
#140310=CARTESIAN_POINT('',(3.4,10.85,-7.62)) ;
#140311=CARTESIAN_POINT('',(3.4,10.05,-7.62)) ;
#140312=CARTESIAN_POINT('',(3.4,9.95,-7.62)) ;
#140313=CARTESIAN_POINT('',(3.4,10.05,-7.62)) ;
#140314=CARTESIAN_POINT('Origin',(3.4,10.95,-7.62)) ;
#140315=CARTESIAN_POINT('',(3.3,10.95,-12.7)) ;
#140316=CARTESIAN_POINT('',(-4.8,10.95,-12.7)) ;
#140317=CARTESIAN_POINT('',(3.4,10.95,-12.7)) ;
#140318=CARTESIAN_POINT('',(-4.8,10.95,-7.62)) ;
#140319=CARTESIAN_POINT('',(-4.8,10.95,-7.62)) ;
#140320=CARTESIAN_POINT('',(3.3,10.95,-7.62)) ;
#140321=CARTESIAN_POINT('',(3.4,10.95,-7.62)) ;
#140322=CARTESIAN_POINT('',(3.3,10.95,-7.62)) ;
#140323=CARTESIAN_POINT('',(-2.55,10.95,-11.06)) ;
#140324=CARTESIAN_POINT('',(-2.75,10.95,-11.26)) ;
#140325=CARTESIAN_POINT('Origin',(-2.75,10.95,-11.06)) ;
#140326=CARTESIAN_POINT('',(-2.55,10.95,-9.26)) ;
#140327=CARTESIAN_POINT('',(-2.55,10.95,-7.62)) ;
#140328=CARTESIAN_POINT('',(-2.75,10.95,-9.06)) ;
#140329=CARTESIAN_POINT('Origin',(-2.75,10.95,-9.26)) ;
#140330=CARTESIAN_POINT('',(-3.8,10.95,-9.06)) ;
#140331=CARTESIAN_POINT('',(3.4,10.95,-9.06)) ;
#140332=CARTESIAN_POINT('',(-4.,10.95,-9.26)) ;
#140333=CARTESIAN_POINT('Origin',(-3.8,10.95,-9.26)) ;
#140334=CARTESIAN_POINT('',(-4.,10.95,-11.06)) ;
#140335=CARTESIAN_POINT('',(-4.,10.95,-7.62)) ;
#140336=CARTESIAN_POINT('',(-3.8,10.95,-11.26)) ;
#140337=CARTESIAN_POINT('Origin',(-3.8,10.95,-11.06)) ;
#140338=CARTESIAN_POINT('',(3.4,10.95,-11.26)) ;
#140339=CARTESIAN_POINT('Origin',(-4.9,10.95,-7.62)) ;
#140340=CARTESIAN_POINT('',(-4.9,10.85,-12.7)) ;
#140341=CARTESIAN_POINT('',(-4.9,10.3,-12.7)) ;
#140342=CARTESIAN_POINT('',(-4.9,10.95,-12.7)) ;
#140343=CARTESIAN_POINT('',(-4.9,10.3,-7.62)) ;
#140344=CARTESIAN_POINT('',(-4.9,10.3,-7.62)) ;
#140345=CARTESIAN_POINT('',(-4.9,10.85,-7.62)) ;
#140346=CARTESIAN_POINT('',(-4.9,10.95,-7.62)) ;
#140347=CARTESIAN_POINT('',(-4.9,10.85,-7.62)) ;
#140348=CARTESIAN_POINT('Origin',(-4.9,10.2,-7.62)) ;
#140349=CARTESIAN_POINT('',(-4.8,10.2,-12.7)) ;
#140350=CARTESIAN_POINT('',(-4.9,10.2,-12.7)) ;
#140351=CARTESIAN_POINT('',(-4.8,10.2,-7.62)) ;
#140352=CARTESIAN_POINT('',(-4.9,10.2,-7.62)) ;
#140353=CARTESIAN_POINT('',(-4.8,10.2,-7.62)) ;
#140354=CARTESIAN_POINT('Origin',(-4.4,10.2,-7.62)) ;
#140355=CARTESIAN_POINT('',(-5.39805806756909,5.20970966215454,-12.7)) ;
#140356=CARTESIAN_POINT('',(-4.4,10.2,-12.7)) ;
#140357=CARTESIAN_POINT('',(-5.39805806756909,5.20970966215454,-7.62)) ;
#140358=CARTESIAN_POINT('',(-5.39805806756909,5.20970966215454,-7.62)) ;
#140359=CARTESIAN_POINT('',(-4.4,10.2,-7.62)) ;
#140360=CARTESIAN_POINT('Origin',(-5.4,5.2,-7.62)) ;
#140361=CARTESIAN_POINT('',(-5.4,5.19009804864072,-12.7)) ;
#140362=CARTESIAN_POINT('',(-5.4,-3.95,-12.7)) ;
#140363=CARTESIAN_POINT('',(-5.4,5.2,-12.7)) ;
#140364=CARTESIAN_POINT('',(-5.4,-3.95,-7.62)) ;
#140365=CARTESIAN_POINT('',(-5.4,-3.95,-7.62)) ;
#140366=CARTESIAN_POINT('',(-5.4,5.19009804864072,-7.62)) ;
#140367=CARTESIAN_POINT('',(-5.4,5.2,-7.62)) ;
#140368=CARTESIAN_POINT('',(-5.4,5.19009804864072,-7.62)) ;
#140369=CARTESIAN_POINT('',(-5.4,4.23801993223491,-12.06)) ;
#140370=CARTESIAN_POINT('',(-5.4,4.23801993223491,-8.26)) ;
#140371=CARTESIAN_POINT('',(-5.4,4.23801993223491,-8.16)) ;
#140372=CARTESIAN_POINT('',(-5.4,3.9369800677651,-8.06)) ;
#140373=CARTESIAN_POINT('Ctrl Pts',(-5.4,4.23801993223491,-8.26)) ;
#140374=CARTESIAN_POINT('Ctrl Pts',(-5.4,4.23801992976516,-8.20749312809024)) ;
#140375=CARTESIAN_POINT('Ctrl Pts',(-5.4,4.20557579169425,-8.15560257376828)) ;
#140376=CARTESIAN_POINT('Ctrl Pts',(-5.4,4.09411900298411,-8.0815547137571)) ;
#140377=CARTESIAN_POINT('Ctrl Pts',(-5.4,4.0160133758189,-8.06000000048129)) ;
#140378=CARTESIAN_POINT('Ctrl Pts',(-5.4,3.9369800677651,-8.06)) ;
#140379=CARTESIAN_POINT('',(-5.4,-1.88819660112502,-8.06)) ;
#140380=CARTESIAN_POINT('',(-5.4,-2.05,-8.06)) ;
#140381=CARTESIAN_POINT('',(-5.4,-2.11180339887499,-8.26)) ;
#140382=CARTESIAN_POINT('Ctrl Pts',(-5.4,-2.11180339887499,-8.26)) ;
#140383=CARTESIAN_POINT('Ctrl Pts',(-5.4,-2.11180339704051,-8.20749316010866)) ;
#140384=CARTESIAN_POINT('Ctrl Pts',(-5.4,-2.0877044485962,-8.15560253112148)) ;
#140385=CARTESIAN_POINT('Ctrl Pts',(-5.4,-2.00491651967066,-8.0815547564039)) ;
#140386=CARTESIAN_POINT('Ctrl Pts',(-5.4,-1.946901032774,-8.06000000117406)) ;
#140387=CARTESIAN_POINT('Ctrl Pts',(-5.4,-1.88819660112502,-8.06)) ;
#140388=CARTESIAN_POINT('',(-5.4,-2.11180339887499,-12.06)) ;
#140389=CARTESIAN_POINT('',(-5.4,-2.11180339887499,-12.16)) ;
#140390=CARTESIAN_POINT('',(-5.4,-1.88819660112501,-12.26)) ;
#140391=CARTESIAN_POINT('Ctrl Pts',(-5.4,-1.88819660112501,-12.26)) ;
#140392=CARTESIAN_POINT('Ctrl Pts',(-5.4,-1.946901032774,-12.2599999988259)) ;
#140393=CARTESIAN_POINT('Ctrl Pts',(-5.4,-2.00491651967066,-12.2384452435961)) ;
#140394=CARTESIAN_POINT('Ctrl Pts',(-5.4,-2.0877044485962,-12.1643974688785)) ;
#140395=CARTESIAN_POINT('Ctrl Pts',(-5.4,-2.11180339704051,-12.1125068398913)) ;
#140396=CARTESIAN_POINT('Ctrl Pts',(-5.4,-2.11180339887499,-12.06)) ;
#140397=CARTESIAN_POINT('',(-5.4,3.9369800677651,-12.26)) ;
#140398=CARTESIAN_POINT('',(-5.4,4.20000000000001,-12.26)) ;
#140399=CARTESIAN_POINT('Ctrl Pts',(-5.4,3.9369800677651,-12.26)) ;
#140400=CARTESIAN_POINT('Ctrl Pts',(-5.4,4.01601337581888,-12.2599999995187)) ;
#140401=CARTESIAN_POINT('Ctrl Pts',(-5.4,4.09411900298413,-12.2384452862428)) ;
#140402=CARTESIAN_POINT('Ctrl Pts',(-5.4,4.20557579169423,-12.1643974262318)) ;
#140403=CARTESIAN_POINT('Ctrl Pts',(-5.4,4.23801992976516,-12.1125068719097)) ;
#140404=CARTESIAN_POINT('Ctrl Pts',(-5.4,4.23801993223491,-12.06)) ;
#140405=CARTESIAN_POINT('Origin',(-5.4,-4.05,-7.62)) ;
#140406=CARTESIAN_POINT('',(-5.3,-4.05,-12.7)) ;
#140407=CARTESIAN_POINT('',(3.5,-4.05,-12.7)) ;
#140408=CARTESIAN_POINT('',(-5.4,-4.05,-12.7)) ;
#140409=CARTESIAN_POINT('',(3.5,-4.05,-7.62)) ;
#140410=CARTESIAN_POINT('',(3.5,-4.05,-7.62)) ;
#140411=CARTESIAN_POINT('',(-5.3,-4.05,-7.62)) ;
#140412=CARTESIAN_POINT('',(-5.4,-4.05,-7.62)) ;
#140413=CARTESIAN_POINT('',(-5.3,-4.05,-7.62)) ;
#140414=CARTESIAN_POINT('',(-4.5,-4.05,-11.06)) ;
#140415=CARTESIAN_POINT('',(-4.3,-4.05,-11.26)) ;
#140416=CARTESIAN_POINT('Origin',(-4.3,-4.05,-11.06)) ;
#140417=CARTESIAN_POINT('',(-4.5,-4.05,-9.26)) ;
#140418=CARTESIAN_POINT('',(-4.5,-4.05,-7.62)) ;
#140419=CARTESIAN_POINT('',(-4.3,-4.05,-9.06)) ;
#140420=CARTESIAN_POINT('Origin',(-4.3,-4.05,-9.26)) ;
#140421=CARTESIAN_POINT('',(-3.25,-4.05,-9.06)) ;
#140422=CARTESIAN_POINT('',(-5.4,-4.05,-9.06)) ;
#140423=CARTESIAN_POINT('',(-3.05,-4.05,-9.26)) ;
#140424=CARTESIAN_POINT('Origin',(-3.25,-4.05,-9.26)) ;
#140425=CARTESIAN_POINT('',(-3.05,-4.05,-11.06)) ;
#140426=CARTESIAN_POINT('',(-3.05,-4.05,-7.62)) ;
#140427=CARTESIAN_POINT('',(-3.25,-4.05,-11.26)) ;
#140428=CARTESIAN_POINT('Origin',(-3.25,-4.05,-11.06)) ;
#140429=CARTESIAN_POINT('',(-5.4,-4.05,-11.26)) ;
#140430=CARTESIAN_POINT('Origin',(3.6,-4.05,-7.62)) ;
#140431=CARTESIAN_POINT('',(3.6,-3.95,-12.7)) ;
#140432=CARTESIAN_POINT('',(3.6,-2.9,-12.7)) ;
#140433=CARTESIAN_POINT('',(3.6,-4.05,-12.7)) ;
#140434=CARTESIAN_POINT('',(3.6,-2.9,-7.62)) ;
#140435=CARTESIAN_POINT('',(3.6,-2.9,-7.62)) ;
#140436=CARTESIAN_POINT('',(3.6,-3.95,-7.62)) ;
#140437=CARTESIAN_POINT('',(3.6,-4.05,-7.62)) ;
#140438=CARTESIAN_POINT('',(3.6,-3.95,-7.62)) ;
#140439=CARTESIAN_POINT('Origin',(3.6,-2.8,-7.62)) ;
#140440=CARTESIAN_POINT('',(4.4,-2.8,-11.6831546211728)) ;
#140441=CARTESIAN_POINT('',(4.54880051362942,-2.79999999972164,-11.2364378607329)) ;
#140442=CARTESIAN_POINT('Ctrl Pts',(4.4,-2.8,-11.6831546211728)) ;
#140443=CARTESIAN_POINT('Ctrl Pts',(4.40001102013632,-2.8,-11.6464400198561)) ;
#140444=CARTESIAN_POINT('Ctrl Pts',(4.40220140384574,-2.79999999812164,
-11.6100681661137)) ;
#140445=CARTESIAN_POINT('Ctrl Pts',(4.4066417499344,-2.79999999722267,-11.5740727380185)) ;
#140446=CARTESIAN_POINT('Ctrl Pts',(4.41108209602305,-2.79999999632371,
-11.5380773099234)) ;
#140447=CARTESIAN_POINT('Ctrl Pts',(4.41777240449119,-2.79999999692353,
-11.5024583074757)) ;
#140448=CARTESIAN_POINT('Ctrl Pts',(4.42678327414413,-2.79999999844302,
-11.4672494087483)) ;
#140449=CARTESIAN_POINT('Ctrl Pts',(4.42864654534549,-2.79999999875722,
-11.4599688987024)) ;
#140450=CARTESIAN_POINT('Ctrl Pts',(4.43060908635821,-2.79999999907333,
-11.4527059171227)) ;
#140451=CARTESIAN_POINT('Ctrl Pts',(4.43267155768736,-2.79999999933982,
-11.4454607590652)) ;
#140452=CARTESIAN_POINT('Ctrl Pts',(4.43529000378769,-2.79999999967816,
-11.4362625435099)) ;
#140453=CARTESIAN_POINT('Ctrl Pts',(4.4380733085653,-2.79999999966609,-11.4270911025424)) ;
#140454=CARTESIAN_POINT('Ctrl Pts',(4.44102157277562,-2.79999999954234,
-11.4179480782015)) ;
#140455=CARTESIAN_POINT('Ctrl Pts',(4.4504649956914,-2.79999999914597,-11.388662559869)) ;
#140456=CARTESIAN_POINT('Ctrl Pts',(4.46157908226633,-2.79999999505379,
-11.3597202134932)) ;
#140457=CARTESIAN_POINT('Ctrl Pts',(4.47540732315415,-2.79999999166095,
-11.3322492625065)) ;
#140458=CARTESIAN_POINT('Ctrl Pts',(4.47702479055525,-2.79999999126409,
-11.3290360289464)) ;
#140459=CARTESIAN_POINT('Ctrl Pts',(4.47867903313992,-2.79999999107055,
-11.3258427221255)) ;
#140460=CARTESIAN_POINT('Ctrl Pts',(4.48037187481471,-2.79999999105954,
-11.322671097194)) ;
#140461=CARTESIAN_POINT('Ctrl Pts',(4.48545039983908,-2.79999999102651,
-11.3131562223995)) ;
#140462=CARTESIAN_POINT('Ctrl Pts',(4.49087631667453,-2.79999999265304,
-11.3038364846096)) ;
#140463=CARTESIAN_POINT('Ctrl Pts',(4.49669887079745,-2.79999999431461,
-11.2947592728789)) ;
#140464=CARTESIAN_POINT('Ctrl Pts',(4.5088870500619,-2.79999999779274,-11.2757582157036)) ;
#140465=CARTESIAN_POINT('Ctrl Pts',(4.52313265843748,-2.79999999982394,
-11.25737449918)) ;
#140466=CARTESIAN_POINT('Ctrl Pts',(4.54066913339539,-2.79999999997241,
-11.2427304219711)) ;
#140467=CARTESIAN_POINT('Ctrl Pts',(4.54329026609835,-2.79999999999461,
-11.240541608668)) ;
#140468=CARTESIAN_POINT('Ctrl Pts',(4.5460045281952,-2.8,-11.2384393445787)) ;
#140469=CARTESIAN_POINT('Ctrl Pts',(4.54880363749517,-2.8,-11.236450206041)) ;
#140470=CARTESIAN_POINT('',(4.4,-2.8,-10.1600000000039)) ;
#140471=CARTESIAN_POINT('Ctrl Pts',(4.54879236168152,-2.8,-11.23643444348)) ;
#140472=CARTESIAN_POINT('Ctrl Pts',(4.51096310105345,-2.8,-11.2076409078196)) ;
#140473=CARTESIAN_POINT('Ctrl Pts',(4.49022331291407,-2.8,-11.1638291192761)) ;
#140474=CARTESIAN_POINT('Ctrl Pts',(4.45698031182017,-2.8,-11.0776238713958)) ;
#140475=CARTESIAN_POINT('Ctrl Pts',(4.44561000227039,-2.8,-11.0323611449586)) ;
#140476=CARTESIAN_POINT('Ctrl Pts',(4.41911102299977,-2.8,-10.8958807916569)) ;
#140477=CARTESIAN_POINT('Ctrl Pts',(4.41155688769424,-2.8,-10.804231375192)) ;
#140478=CARTESIAN_POINT('Ctrl Pts',(4.39763503647248,-2.8,-10.528710456933)) ;
#140479=CARTESIAN_POINT('Ctrl Pts',(4.4,-2.8,-10.3442606621178)) ;
#140480=CARTESIAN_POINT('Ctrl Pts',(4.4,-2.8,-10.1600000000039)) ;
#140481=CARTESIAN_POINT('',(4.54879236179094,-2.79999999953044,-9.08356555650414)) ;
#140482=CARTESIAN_POINT('Ctrl Pts',(4.4,-2.8,-10.1600000000039)) ;
#140483=CARTESIAN_POINT('Ctrl Pts',(4.4,-2.8,-9.9754847183429)) ;
#140484=CARTESIAN_POINT('Ctrl Pts',(4.39760751905643,-2.8,-9.79078367328513)) ;
#140485=CARTESIAN_POINT('Ctrl Pts',(4.40696794948104,-2.8,-9.60658932370333)) ;
#140486=CARTESIAN_POINT('Ctrl Pts',(4.41164816469334,-2.8,-9.51449214891243)) ;
#140487=CARTESIAN_POINT('Ctrl Pts',(4.41940496802384,-2.80000000000001,
-9.42215714350079)) ;
#140488=CARTESIAN_POINT('Ctrl Pts',(4.43698455094238,-2.8,-9.3320661537484)) ;
#140489=CARTESIAN_POINT('Ctrl Pts',(4.44577434240166,-2.8,-9.2870206588722)) ;
#140490=CARTESIAN_POINT('Ctrl Pts',(4.456925956929,-2.80000000000001,-9.24247691748965)) ;
#140491=CARTESIAN_POINT('Ctrl Pts',(4.47366127850409,-2.8,-9.19911940609041)) ;
#140492=CARTESIAN_POINT('Ctrl Pts',(4.47575319370098,-2.8,-9.19369971716552)) ;
#140493=CARTESIAN_POINT('Ctrl Pts',(4.47791173590511,-2.79999999997843,
-9.18827415478058)) ;
#140494=CARTESIAN_POINT('Ctrl Pts',(4.48016062485992,-2.80000000010461,
-9.18287328752205)) ;
#140495=CARTESIAN_POINT('Ctrl Pts',(4.48803173620173,-2.80000000054624,
-9.1639702521172)) ;
#140496=CARTESIAN_POINT('Ctrl Pts',(4.49700942865457,-2.80000000534986,
-9.14536966581437)) ;
#140497=CARTESIAN_POINT('Ctrl Pts',(4.50810946414921,-2.80000000469598,
-9.12838166513933)) ;
#140498=CARTESIAN_POINT('Ctrl Pts',(4.51435323411495,-2.80000000432818,
-9.11882591475961)) ;
#140499=CARTESIAN_POINT('Ctrl Pts',(4.52126852668377,-2.80000000204489,
-9.10978039655139)) ;
#140500=CARTESIAN_POINT('Ctrl Pts',(4.5290361256546,-2.80000000089509,-9.10147828666764)) ;
#140501=CARTESIAN_POINT('Ctrl Pts',(4.5320568585877,-2.80000000044794,-9.09824968837951)) ;
#140502=CARTESIAN_POINT('Ctrl Pts',(4.53520648971123,-2.80000000018876,
-9.09513351912811)) ;
#140503=CARTESIAN_POINT('Ctrl Pts',(4.53849565154303,-2.80000000008376,
-9.09214349280593)) ;
#140504=CARTESIAN_POINT('Ctrl Pts',(4.54178481337482,-2.79999999997876,
-9.08915346648376)) ;
#140505=CARTESIAN_POINT('Ctrl Pts',(4.54521363891047,-2.8,-9.08628975782186)) ;
#140506=CARTESIAN_POINT('Ctrl Pts',(4.54879236168087,-2.8,-9.08356555651953)) ;
#140507=CARTESIAN_POINT('',(4.4,-2.8,-8.63684537882721)) ;
#140508=CARTESIAN_POINT('Ctrl Pts',(4.54879236168109,-2.79999999812176,
-9.08356555651923)) ;
#140509=CARTESIAN_POINT('Ctrl Pts',(4.54599316991904,-2.79999999835896,
-9.08157561433548)) ;
#140510=CARTESIAN_POINT('Ctrl Pts',(4.54327885465675,-2.7999999985882,-9.07947265683989)) ;
#140511=CARTESIAN_POINT('Ctrl Pts',(4.52311604063301,-2.80000000023132,
-9.06263105969308)) ;
#140512=CARTESIAN_POINT('Ctrl Pts',(4.50886780632329,-2.80000000100534,
-9.04424219964313)) ;
#140513=CARTESIAN_POINT('Ctrl Pts',(4.48892103801305,-2.79999999510253,
-9.01312902183043)) ;
#140514=CARTESIAN_POINT('Ctrl Pts',(4.4818652331329,-2.79999999099551,-9.00058320502371)) ;
#140515=CARTESIAN_POINT('Ctrl Pts',(4.46162186753408,-2.79999997126272,
-8.96025671394186)) ;
#140516=CARTESIAN_POINT('Ctrl Pts',(4.45052849087262,-2.7999999685384,-8.93131896170922)) ;
#140517=CARTESIAN_POINT('Ctrl Pts',(4.43813540717735,-2.79999997674815,
-8.8929060591291)) ;
#140518=CARTESIAN_POINT('Ctrl Pts',(4.43535270120344,-2.79999997903695,
-8.88375026405077)) ;
#140519=CARTESIAN_POINT('Ctrl Pts',(4.41677772587857,-2.79999999273252,
-8.81866880149579)) ;
#140520=CARTESIAN_POINT('Ctrl Pts',(4.40678488791117,-2.79999999887621,
-8.76171951851187)) ;
#140521=CARTESIAN_POINT('Ctrl Pts',(4.40081887576568,-2.80000000006435,
-8.68161989678019)) ;
#140522=CARTESIAN_POINT('Ctrl Pts',(4.4,-2.8,-8.65930189818788)) ;
#140523=CARTESIAN_POINT('Ctrl Pts',(4.4,-2.8,-8.63684537882721)) ;
#140524=CARTESIAN_POINT('',(4.4,-2.8,-7.62)) ;
#140525=CARTESIAN_POINT('',(4.4,-2.8,-7.62)) ;
#140526=CARTESIAN_POINT('',(3.7,-2.8,-7.62)) ;
#140527=CARTESIAN_POINT('',(3.6,-2.8,-7.62)) ;
#140528=CARTESIAN_POINT('',(3.7,-2.8,-12.7)) ;
#140529=CARTESIAN_POINT('',(3.7,-2.8,-12.7)) ;
#140530=CARTESIAN_POINT('',(4.4,-2.8,-12.7)) ;
#140531=CARTESIAN_POINT('',(3.6,-2.8,-12.7)) ;
#140532=CARTESIAN_POINT('',(4.4,-2.8,-7.62)) ;
#140533=CARTESIAN_POINT('Origin',(4.5,-2.8,-7.62)) ;
#140534=CARTESIAN_POINT('',(4.5,-2.7,-7.62)) ;
#140535=CARTESIAN_POINT('',(4.5,-2.4,-7.62)) ;
#140536=CARTESIAN_POINT('',(4.5,-2.8,-7.62)) ;
#140537=CARTESIAN_POINT('',(4.5,-2.7,-8.63684537882721)) ;
#140538=CARTESIAN_POINT('',(4.5,-2.7,-7.62)) ;
#140539=CARTESIAN_POINT('',(4.5,-2.4,-8.19785831296514)) ;
#140540=CARTESIAN_POINT('Origin',(4.5,0.,-10.16)) ;
#140541=CARTESIAN_POINT('',(4.5,-2.4,-7.62)) ;
#140542=CARTESIAN_POINT('Origin',(4.5,-2.3,-7.62)) ;
#140543=CARTESIAN_POINT('',(12.7,-2.3,-12.1221416870349)) ;
#140544=CARTESIAN_POINT('',(4.6,-2.3,-12.1221416870349)) ;
#140545=CARTESIAN_POINT('',(4.5,-2.3,-12.1221416870349)) ;
#140546=CARTESIAN_POINT('',(4.6,-2.3,-12.7)) ;
#140547=CARTESIAN_POINT('',(4.6,-2.3,-12.7)) ;
#140548=CARTESIAN_POINT('',(12.7,-2.3,-12.7)) ;
#140549=CARTESIAN_POINT('',(4.5,-2.3,-12.7)) ;
#140550=CARTESIAN_POINT('',(12.7,-2.3,-7.62)) ;
#140551=CARTESIAN_POINT('Origin',(0.,0.,-7.62)) ;
#140552=CARTESIAN_POINT('Origin',(4.4,-2.7,-7.62)) ;
#140553=CARTESIAN_POINT('Origin',(4.6,-2.4,-7.62)) ;
#140554=CARTESIAN_POINT('Origin',(12.7,-2.2,-7.62)) ;
#140555=CARTESIAN_POINT('Origin',(12.7,2.65,-7.62)) ;
#140556=CARTESIAN_POINT('Origin',(4.55912712210514,2.85,-7.62)) ;
#140557=CARTESIAN_POINT('Origin',(4.05,3.77568567655479,-7.62)) ;
#140558=CARTESIAN_POINT('Origin',(3.85,6.92431432344521,-7.62)) ;
#140559=CARTESIAN_POINT('Origin',(3.34087287789487,7.85,-7.62)) ;
#140560=CARTESIAN_POINT('Origin',(3.,8.05,-7.62)) ;
#140561=CARTESIAN_POINT('Origin',(3.,9.85,-7.62)) ;
#140562=CARTESIAN_POINT('Origin',(3.3,10.05,-7.62)) ;
#140563=CARTESIAN_POINT('Origin',(3.3,10.85,-7.62)) ;
#140564=CARTESIAN_POINT('Origin',(-4.8,10.85,-7.62)) ;
#140565=CARTESIAN_POINT('Origin',(-4.8,10.3,-7.62)) ;
#140566=CARTESIAN_POINT('Origin',(-5.3,5.19009804864072,-7.62)) ;
#140567=CARTESIAN_POINT('Origin',(-5.3,-3.95,-7.62)) ;
#140568=CARTESIAN_POINT('Origin',(3.5,-3.95,-7.62)) ;
#140569=CARTESIAN_POINT('Origin',(3.7,-2.9,-7.62)) ;
#140570=CARTESIAN_POINT('Origin',(0.,0.,-12.7)) ;
#140571=CARTESIAN_POINT('Origin',(4.4,-2.7,-12.7)) ;
#140572=CARTESIAN_POINT('Origin',(3.7,-2.9,-12.7)) ;
#140573=CARTESIAN_POINT('Origin',(3.5,-3.95,-12.7)) ;
#140574=CARTESIAN_POINT('Origin',(-5.3,-3.95,-12.7)) ;
#140575=CARTESIAN_POINT('Origin',(-5.3,5.19009804864072,-12.7)) ;
#140576=CARTESIAN_POINT('Origin',(-4.8,10.3,-12.7)) ;
#140577=CARTESIAN_POINT('Origin',(-4.8,10.85,-12.7)) ;
#140578=CARTESIAN_POINT('Origin',(3.3,10.85,-12.7)) ;
#140579=CARTESIAN_POINT('Origin',(3.3,10.05,-12.7)) ;
#140580=CARTESIAN_POINT('Origin',(3.,9.85,-12.7)) ;
#140581=CARTESIAN_POINT('Origin',(3.,8.05,-12.7)) ;
#140582=CARTESIAN_POINT('Origin',(3.34087287789487,7.85,-12.7)) ;
#140583=CARTESIAN_POINT('Origin',(3.85,6.92431432344521,-12.7)) ;
#140584=CARTESIAN_POINT('Origin',(4.05,3.77568567655479,-12.7)) ;
#140585=CARTESIAN_POINT('Origin',(4.55912712210514,2.85,-12.7)) ;
#140586=CARTESIAN_POINT('Origin',(12.7,2.65,-12.7)) ;
#140587=CARTESIAN_POINT('Origin',(12.7,-2.2,-12.7)) ;
#140588=CARTESIAN_POINT('Origin',(4.6,-2.4,-12.7)) ;
#140589=CARTESIAN_POINT('Origin',(-4.65,1.95,-12.16)) ;
#140590=CARTESIAN_POINT('',(-4.66204490261456,3.21928058320648,-12.16)) ;
#140591=CARTESIAN_POINT('',(-5.3,3.9369800677651,-12.16)) ;
#140592=CARTESIAN_POINT('',(-5.47474093186837,4.13356361611701,-12.16)) ;
#140593=CARTESIAN_POINT('',(-5.3,-1.88819660112501,-12.16)) ;
#140594=CARTESIAN_POINT('',(-5.3,-2.05,-12.16)) ;
#140595=CARTESIAN_POINT('',(-4.66204490261456,-1.5692190524323,-12.16)) ;
#140596=CARTESIAN_POINT('',(-4.69472135955,-1.58555728090001,-12.16)) ;
#140597=CARTESIAN_POINT('',(-4.66204490261456,3.35625,-12.16)) ;
#140598=CARTESIAN_POINT('Origin',(-5.4,1.95,-8.16)) ;
#140599=CARTESIAN_POINT('',(-4.66204490261456,-1.5692190524323,-8.16)) ;
#140600=CARTESIAN_POINT('',(-5.3,-1.88819660112502,-8.16)) ;
#140601=CARTESIAN_POINT('',(-5.44472135955,-1.96055728090001,-8.16)) ;
#140602=CARTESIAN_POINT('',(-5.3,3.9369800677651,-8.16)) ;
#140603=CARTESIAN_POINT('',(-5.3,4.20000000000001,-8.16)) ;
#140604=CARTESIAN_POINT('',(-4.66204490261456,3.21928058320648,-8.16)) ;
#140605=CARTESIAN_POINT('',(-4.72474093186837,3.28981361611701,-8.16)) ;
#140606=CARTESIAN_POINT('',(-4.66204490261456,-1.67500000000001,-8.16)) ;
#140607=CARTESIAN_POINT('Origin',(-4.65,1.95,-8.16)) ;
#140608=CARTESIAN_POINT('',(-3.33134808452128,1.85,-8.4823371348948)) ;
#140609=CARTESIAN_POINT('',(-3.48082994825801,1.91712723223402,-8.44579712375915)) ;
#140610=CARTESIAN_POINT('Origin',(-3.34328863644876,2.02341244982311,-8.47941833331253)) ;
#140611=CARTESIAN_POINT('',(-2.4,1.85,-8.71)) ;
#140612=CARTESIAN_POINT('',(-4.65,1.85,-8.16)) ;
#140613=CARTESIAN_POINT('',(-2.4,-0.95,-8.71)) ;
#140614=CARTESIAN_POINT('',(-2.4,1.95,-8.71)) ;
#140615=CARTESIAN_POINT('',(-3.3526478932023,-0.95,-8.47713051499499)) ;
#140616=CARTESIAN_POINT('',(-3.39999999999998,-0.95,-8.46555555555556)) ;
#140617=CARTESIAN_POINT('',(-3.44209061230229,-0.971114561800017,-8.455266739215)) ;
#140618=CARTESIAN_POINT('Origin',(-3.36201220558124,-1.11033257691482,-8.47484146085793)) ;
#140619=CARTESIAN_POINT('',(-4.63829959356686,-1.5692190524323,-8.16286009935032)) ;
#140620=CARTESIAN_POINT('',(-4.68814869588294,-1.59414360359034,-8.15067476322861)) ;
#140621=CARTESIAN_POINT('',(-4.63829959356686,3.21928058320648,-8.16286009935032)) ;
#140622=CARTESIAN_POINT('',(-4.63829959356686,3.35625,-8.16286009935032)) ;
#140623=CARTESIAN_POINT('',(-3.45989661114215,1.89357722797868,-8.45091416172081)) ;
#140624=CARTESIAN_POINT('Origin',(-2.4,1.95,-8.71)) ;
#140625=CARTESIAN_POINT('',(-2.4,1.85,-11.61)) ;
#140626=CARTESIAN_POINT('',(-2.4,-0.95,-11.61)) ;
#140627=CARTESIAN_POINT('',(-2.4,1.95,-11.61)) ;
#140628=CARTESIAN_POINT('',(-2.4,-1.05,-11.507055690472)) ;
#140629=CARTESIAN_POINT('Origin',(-2.4,-0.949999999999936,-11.5070556904719)) ;
#140630=CARTESIAN_POINT('',(-2.4,-1.05,-8.81294430952801)) ;
#140631=CARTESIAN_POINT('',(-2.4,-1.05,-8.71)) ;
#140632=CARTESIAN_POINT('Origin',(-2.4,-0.9499999999999,-8.8129443095281)) ;
#140633=CARTESIAN_POINT('',(-2.4,1.95,-8.81294430952801)) ;
#140634=CARTESIAN_POINT('Origin',(-2.4,1.84999999999991,-8.81294430952809)) ;
#140635=CARTESIAN_POINT('',(-2.4,1.95,-11.507055690472)) ;
#140636=CARTESIAN_POINT('',(-2.4,1.95,-8.71)) ;
#140637=CARTESIAN_POINT('Origin',(-2.4,1.85000000000013,-11.5070556904721)) ;
#140638=CARTESIAN_POINT('Origin',(-2.4,1.95,-11.61)) ;
#140639=CARTESIAN_POINT('',(-3.3526478932023,-0.95,-11.842869485005)) ;
#140640=CARTESIAN_POINT('',(-3.44209061230229,-0.971114561800017,-11.864733260785)) ;
#140641=CARTESIAN_POINT('Origin',(-3.36201220558131,-1.11033257691521,-11.8451585391422)) ;
#140642=CARTESIAN_POINT('',(-2.4,-0.95,-11.61)) ;
#140643=CARTESIAN_POINT('',(-3.33134808452128,1.85,-11.8376628651052)) ;
#140644=CARTESIAN_POINT('',(-2.4,1.85,-11.61)) ;
#140645=CARTESIAN_POINT('',(-3.48082994825801,1.91712723223402,-11.8742028762408)) ;
#140646=CARTESIAN_POINT('Origin',(-3.34328863644893,2.02341244982219,-11.8405816666875)) ;
#140647=CARTESIAN_POINT('',(-4.63829959356686,3.21928058320648,-12.1571399006497)) ;
#140648=CARTESIAN_POINT('',(-4.70989661114216,3.29982722797869,-12.1746413938348)) ;
#140649=CARTESIAN_POINT('',(-4.63829959356686,-1.5692190524323,-12.1571399006497)) ;
#140650=CARTESIAN_POINT('',(-4.63829959356686,-1.67500000000001,-12.1571399006497)) ;
#140651=CARTESIAN_POINT('',(-3.43814869588292,-0.969143603590331,-11.8637696812158)) ;
#140652=CARTESIAN_POINT('Origin',(0.,1.95,-10.16)) ;
#140653=CARTESIAN_POINT('',(-3.35509339356897,1.95,-8.57947703554448)) ;
#140654=CARTESIAN_POINT('',(0.175392621986784,1.95,-9.44248472823589)) ;
#140655=CARTESIAN_POINT('',(-3.35509339356897,1.95,-11.7405229644555)) ;
#140656=CARTESIAN_POINT('',(-3.35509339356897,1.95,-11.8544444444444)) ;
#140657=CARTESIAN_POINT('',(0.175392621986784,1.95,-10.8775152717641)) ;
#140658=CARTESIAN_POINT('Origin',(0.,-1.05,-10.16)) ;
#140659=CARTESIAN_POINT('',(-3.37639320225,-1.05,-11.7457295843553)) ;
#140660=CARTESIAN_POINT('',(-3.42374530904768,-1.05,-11.7573045437948)) ;
#140661=CARTESIAN_POINT('',(-3.37639320225,-1.05,-8.57427041564467)) ;
#140662=CARTESIAN_POINT('',(-3.37639320225,-1.05,-10.16)) ;
#140663=CARTESIAN_POINT('',(-2.4237453090477,-1.05,-8.80713990064968)) ;
#140664=CARTESIAN_POINT('Origin',(-3.39999999999998,-1.05,-10.16)) ;
#140665=CARTESIAN_POINT('',(-3.4211145618,-1.06055728090001,-8.55240663986467)) ;
#140666=CARTESIAN_POINT('',(-3.4211145618,-1.06055728090001,-11.7675933601353)) ;
#140667=CARTESIAN_POINT('',(-3.4211145618,-1.06055728090001,-10.16)) ;
#140668=CARTESIAN_POINT('',(-4.61732354306457,-1.65866177153229,-12.06)) ;
#140669=CARTESIAN_POINT('',(-4.66717264538064,-1.68358632269033,-12.0721853361217)) ;
#140670=CARTESIAN_POINT('',(-5.34472135954999,-2.022360679775,-12.06)) ;
#140671=CARTESIAN_POINT('',(-5.4,-2.05,-12.06)) ;
#140672=CARTESIAN_POINT('',(-5.34472135954999,-2.022360679775,-8.26)) ;
#140673=CARTESIAN_POINT('',(-5.34472135954999,-2.022360679775,-8.16)) ;
#140674=CARTESIAN_POINT('',(-4.61732354306457,-1.65866177153229,-8.26)) ;
#140675=CARTESIAN_POINT('',(-4.65,-1.67500000000001,-8.26)) ;
#140676=CARTESIAN_POINT('',(-3.41717264538063,-1.05858632269032,-8.55337021943385)) ;
#140677=CARTESIAN_POINT('Origin',(-5.4,4.20000000000001,-7.62)) ;
#140678=CARTESIAN_POINT('',(-5.37474093186837,4.17158354835192,-8.26)) ;
#140679=CARTESIAN_POINT('',(-5.37474093186837,4.17158354835192,-12.06)) ;
#140680=CARTESIAN_POINT('',(-5.37474093186837,4.17158354835192,-12.16)) ;
#140681=CARTESIAN_POINT('',(-4.58730397074619,3.28571696708947,-12.06)) ;
#140682=CARTESIAN_POINT('',(-4.65,3.35625,-12.06)) ;
#140683=CARTESIAN_POINT('',(-3.42983432543734,1.98356361611701,-11.7770629755912)) ;
#140684=CARTESIAN_POINT('',(-3.40890098832149,1.96001361186167,-11.7719459376295)) ;
#140685=CARTESIAN_POINT('',(-3.42983432543734,1.98356361611701,-8.54293702440883)) ;
#140686=CARTESIAN_POINT('',(-3.42983432543734,1.98356361611701,-8.46555555555556)) ;
#140687=CARTESIAN_POINT('',(-4.58730397074619,3.28571696708947,-8.26)) ;
#140688=CARTESIAN_POINT('',(-4.65890098832149,3.36626361186168,-8.24249850681493)) ;
#140689=CARTESIAN_POINT('',(-5.4,4.20000000000001,-8.26)) ;
#140690=CARTESIAN_POINT('Origin',(-3.15,-3.9,-9.16)) ;
#140691=CARTESIAN_POINT('',(-3.15,-3.95,-9.26)) ;
#140692=CARTESIAN_POINT('',(-3.15,-3.85,-9.26)) ;
#140693=CARTESIAN_POINT('',(-3.15,-3.75,-9.26)) ;
#140694=CARTESIAN_POINT('',(-3.15,-3.85,-11.06)) ;
#140695=CARTESIAN_POINT('',(-3.15,-3.85,-9.16)) ;
#140696=CARTESIAN_POINT('',(-3.15,-3.95,-11.06)) ;
#140697=CARTESIAN_POINT('',(-3.15,-4.05,-11.06)) ;
#140698=CARTESIAN_POINT('',(-3.15,-3.95,-9.16)) ;
#140699=CARTESIAN_POINT('Origin',(-4.4,-3.9,-11.16)) ;
#140700=CARTESIAN_POINT('',(-3.25,-3.85,-11.16)) ;
#140701=CARTESIAN_POINT('',(-4.3,-3.85,-11.16)) ;
#140702=CARTESIAN_POINT('',(-4.4,-3.85,-11.16)) ;
#140703=CARTESIAN_POINT('',(-4.3,-3.95,-11.16)) ;
#140704=CARTESIAN_POINT('',(-4.3,-4.05,-11.16)) ;
#140705=CARTESIAN_POINT('',(-3.25,-3.95,-11.16)) ;
#140706=CARTESIAN_POINT('',(-4.4,-3.95,-11.16)) ;
#140707=CARTESIAN_POINT('',(-3.25,-3.75,-11.16)) ;
#140708=CARTESIAN_POINT('Origin',(-4.4,-3.9,-9.16)) ;
#140709=CARTESIAN_POINT('',(-4.4,-3.85,-11.06)) ;
#140710=CARTESIAN_POINT('',(-4.4,-3.85,-9.26)) ;
#140711=CARTESIAN_POINT('',(-4.4,-3.85,-9.16)) ;
#140712=CARTESIAN_POINT('',(-4.4,-3.95,-9.26)) ;
#140713=CARTESIAN_POINT('',(-4.4,-4.05,-9.26)) ;
#140714=CARTESIAN_POINT('',(-4.4,-3.95,-11.06)) ;
#140715=CARTESIAN_POINT('',(-4.4,-3.95,-9.16)) ;
#140716=CARTESIAN_POINT('',(-4.4,-3.75,-11.06)) ;
#140717=CARTESIAN_POINT('Origin',(-4.4,-3.9,-9.16)) ;
#140718=CARTESIAN_POINT('',(-4.3,-3.95,-9.16)) ;
#140719=CARTESIAN_POINT('',(-4.3,-3.85,-9.16)) ;
#140720=CARTESIAN_POINT('',(-4.3,-3.75,-9.16)) ;
#140721=CARTESIAN_POINT('',(-3.25,-3.85,-9.16)) ;
#140722=CARTESIAN_POINT('',(-4.4,-3.85,-9.16)) ;
#140723=CARTESIAN_POINT('',(-3.25,-3.95,-9.16)) ;
#140724=CARTESIAN_POINT('',(-3.25,-4.05,-9.16)) ;
#140725=CARTESIAN_POINT('',(-4.4,-3.95,-9.16)) ;
#140726=CARTESIAN_POINT('Origin',(0.,-3.75,-10.16)) ;
#140727=CARTESIAN_POINT('',(-3.25,-3.75,-9.26)) ;
#140728=CARTESIAN_POINT('',(-4.3,-3.75,-9.26)) ;
#140729=CARTESIAN_POINT('',(-1.56125112837913E-16,-3.75,-9.26)) ;
#140730=CARTESIAN_POINT('',(-4.3,-3.75,-11.06)) ;
#140731=CARTESIAN_POINT('',(-4.3,-3.75,-10.16)) ;
#140732=CARTESIAN_POINT('',(-3.25,-3.75,-11.06)) ;
#140733=CARTESIAN_POINT('',(-1.56125112837913E-16,-3.75,-11.06)) ;
#140734=CARTESIAN_POINT('',(-3.25,-3.75,-10.16)) ;
#140735=CARTESIAN_POINT('',(-4.15,-3.75,-11.01)) ;
#140736=CARTESIAN_POINT('',(-3.4,-3.75,-11.01)) ;
#140737=CARTESIAN_POINT('',(-4.15,-3.75,-11.01)) ;
#140738=CARTESIAN_POINT('',(-4.25,-3.75,-10.91)) ;
#140739=CARTESIAN_POINT('Origin',(-4.15,-3.75,-10.91)) ;
#140740=CARTESIAN_POINT('',(-4.25,-3.75,-9.41)) ;
#140741=CARTESIAN_POINT('',(-4.25,-3.75,-9.41)) ;
#140742=CARTESIAN_POINT('',(-4.15,-3.75,-9.31)) ;
#140743=CARTESIAN_POINT('Origin',(-4.15,-3.75,-9.41)) ;
#140744=CARTESIAN_POINT('',(-3.4,-3.75,-9.31)) ;
#140745=CARTESIAN_POINT('',(-3.4,-3.75,-9.31)) ;
#140746=CARTESIAN_POINT('',(-3.3,-3.75,-9.41)) ;
#140747=CARTESIAN_POINT('Origin',(-3.4,-3.75,-9.41)) ;
#140748=CARTESIAN_POINT('',(-3.3,-3.75,-10.91)) ;
#140749=CARTESIAN_POINT('',(-3.3,-3.75,-10.91)) ;
#140750=CARTESIAN_POINT('Origin',(-3.4,-3.75,-10.91)) ;
#140751=CARTESIAN_POINT('Origin',(-3.4,-3.75,-10.91)) ;
#140752=CARTESIAN_POINT('',(-3.4,-3.9,-11.01)) ;
#140753=CARTESIAN_POINT('',(-3.3,-3.9,-10.91)) ;
#140754=CARTESIAN_POINT('Origin',(-3.4,-3.9,-10.91)) ;
#140755=CARTESIAN_POINT('',(-3.4,-3.75,-11.01)) ;
#140756=CARTESIAN_POINT('',(-3.3,-3.75,-10.91)) ;
#140757=CARTESIAN_POINT('Origin',(-4.15,-3.75,-11.01)) ;
#140758=CARTESIAN_POINT('',(-4.15,-3.9,-11.01)) ;
#140759=CARTESIAN_POINT('',(-4.15,-3.9,-11.01)) ;
#140760=CARTESIAN_POINT('',(-4.15,-3.75,-11.01)) ;
#140761=CARTESIAN_POINT('Origin',(-4.15,-3.75,-10.91)) ;
#140762=CARTESIAN_POINT('',(-4.25,-3.9,-10.91)) ;
#140763=CARTESIAN_POINT('Origin',(-4.15,-3.9,-10.91)) ;
#140764=CARTESIAN_POINT('',(-4.25,-3.75,-10.91)) ;
#140765=CARTESIAN_POINT('Origin',(-4.25,-3.75,-9.41)) ;
#140766=CARTESIAN_POINT('',(-4.25,-3.9,-9.41)) ;
#140767=CARTESIAN_POINT('',(-4.25,-3.9,-9.41)) ;
#140768=CARTESIAN_POINT('',(-4.25,-3.75,-9.41)) ;
#140769=CARTESIAN_POINT('Origin',(-4.15,-3.75,-9.41)) ;
#140770=CARTESIAN_POINT('',(-4.15,-3.9,-9.31)) ;
#140771=CARTESIAN_POINT('Origin',(-4.15,-3.9,-9.41)) ;
#140772=CARTESIAN_POINT('',(-4.15,-3.75,-9.31)) ;
#140773=CARTESIAN_POINT('Origin',(-3.4,-3.75,-9.31)) ;
#140774=CARTESIAN_POINT('',(-3.4,-3.9,-9.31)) ;
#140775=CARTESIAN_POINT('',(-3.4,-3.9,-9.31)) ;
#140776=CARTESIAN_POINT('',(-3.4,-3.75,-9.31)) ;
#140777=CARTESIAN_POINT('Origin',(-3.4,-3.75,-9.41)) ;
#140778=CARTESIAN_POINT('',(-3.3,-3.9,-9.41)) ;
#140779=CARTESIAN_POINT('Origin',(-3.4,-3.9,-9.41)) ;
#140780=CARTESIAN_POINT('',(-3.3,-3.75,-9.41)) ;
#140781=CARTESIAN_POINT('Origin',(-3.3,-3.75,-10.91)) ;
#140782=CARTESIAN_POINT('',(-3.3,-3.9,-10.91)) ;
#140783=CARTESIAN_POINT('Origin',(0.,-3.9,-10.16)) ;
#140784=CARTESIAN_POINT('Origin',(0.,9.95,-10.16)) ;
#140785=CARTESIAN_POINT('',(-0.230887397576972,9.95,-8.24513942814623)) ;
#140786=CARTESIAN_POINT('Origin',(-0.321518176280637,8.95,-8.2874012543203)) ;
#140787=CARTESIAN_POINT('',(-0.321518176280637,9.05,-8.2874012543203)) ;
#140788=CARTESIAN_POINT('',(1.22782596331729,9.85,-11.609980483939)) ;
#140789=CARTESIAN_POINT('Origin',(-1.22782596331729,8.95,-8.710019516061)) ;
#140790=CARTESIAN_POINT('',(-1.22782596331729,9.05,-8.710019516061)) ;
#140791=CARTESIAN_POINT('',(-1.22782596331729,9.85,-8.710019516061)) ;
#140792=CARTESIAN_POINT('Origin',(0.,8.95,-10.16)) ;
#140793=CARTESIAN_POINT('',(-0.362523114814661,8.95,-10.3290473046963)) ;
#140794=CARTESIAN_POINT('',(0.36252311481466,8.95,-9.99095269530372)) ;
#140795=CARTESIAN_POINT('Origin',(-2.65,10.8,-11.16)) ;
#140796=CARTESIAN_POINT('',(-2.65,10.75,-11.06)) ;
#140797=CARTESIAN_POINT('',(-2.65,10.75,-9.26)) ;
#140798=CARTESIAN_POINT('',(-2.65,10.75,-11.16)) ;
#140799=CARTESIAN_POINT('',(-2.65,10.85,-9.26)) ;
#140800=CARTESIAN_POINT('',(-2.65,10.95,-9.26)) ;
#140801=CARTESIAN_POINT('',(-2.65,10.85,-11.06)) ;
#140802=CARTESIAN_POINT('',(-2.65,10.85,-11.16)) ;
#140803=CARTESIAN_POINT('',(-2.65,10.65,-11.06)) ;
#140804=CARTESIAN_POINT('Origin',(-3.9,10.8,-9.16)) ;
#140805=CARTESIAN_POINT('',(-2.75,10.85,-9.16)) ;
#140806=CARTESIAN_POINT('',(-2.75,10.75,-9.16)) ;
#140807=CARTESIAN_POINT('',(-2.75,10.65,-9.16)) ;
#140808=CARTESIAN_POINT('',(-3.8,10.75,-9.16)) ;
#140809=CARTESIAN_POINT('',(-3.9,10.75,-9.16)) ;
#140810=CARTESIAN_POINT('',(-3.8,10.85,-9.16)) ;
#140811=CARTESIAN_POINT('',(-3.8,10.95,-9.16)) ;
#140812=CARTESIAN_POINT('',(-3.9,10.85,-9.16)) ;
#140813=CARTESIAN_POINT('Origin',(-3.9,10.8,-11.16)) ;
#140814=CARTESIAN_POINT('',(-3.9,10.85,-9.26)) ;
#140815=CARTESIAN_POINT('',(-3.9,10.75,-9.26)) ;
#140816=CARTESIAN_POINT('',(-3.9,10.65,-9.26)) ;
#140817=CARTESIAN_POINT('',(-3.9,10.75,-11.06)) ;
#140818=CARTESIAN_POINT('',(-3.9,10.75,-11.16)) ;
#140819=CARTESIAN_POINT('',(-3.9,10.85,-11.06)) ;
#140820=CARTESIAN_POINT('',(-3.9,10.95,-11.06)) ;
#140821=CARTESIAN_POINT('',(-3.9,10.85,-11.16)) ;
#140822=CARTESIAN_POINT('Origin',(-3.9,10.8,-11.16)) ;
#140823=CARTESIAN_POINT('',(-3.8,10.75,-11.16)) ;
#140824=CARTESIAN_POINT('',(-2.75,10.75,-11.16)) ;
#140825=CARTESIAN_POINT('',(-3.9,10.75,-11.16)) ;
#140826=CARTESIAN_POINT('',(-2.75,10.85,-11.16)) ;
#140827=CARTESIAN_POINT('',(-2.75,10.95,-11.16)) ;
#140828=CARTESIAN_POINT('',(-3.8,10.85,-11.16)) ;
#140829=CARTESIAN_POINT('',(-3.9,10.85,-11.16)) ;
#140830=CARTESIAN_POINT('',(-3.8,10.65,-11.16)) ;
#140831=CARTESIAN_POINT('Origin',(0.,10.65,-10.16)) ;
#140832=CARTESIAN_POINT('',(-3.8,10.65,-9.26)) ;
#140833=CARTESIAN_POINT('',(-2.75,10.65,-9.26)) ;
#140834=CARTESIAN_POINT('',(1.56125112837912E-16,10.65,-9.26)) ;
#140835=CARTESIAN_POINT('',(-2.75,10.65,-11.06)) ;
#140836=CARTESIAN_POINT('',(-2.75,10.65,-10.16)) ;
#140837=CARTESIAN_POINT('',(-3.8,10.65,-11.06)) ;
#140838=CARTESIAN_POINT('',(-1.56125112837913E-16,10.65,-11.06)) ;
#140839=CARTESIAN_POINT('',(-3.8,10.65,-10.16)) ;
#140840=CARTESIAN_POINT('',(-3.65,10.65,-9.31)) ;
#140841=CARTESIAN_POINT('',(-2.9,10.65,-9.31)) ;
#140842=CARTESIAN_POINT('',(-3.65,10.65,-9.31)) ;
#140843=CARTESIAN_POINT('',(-3.75,10.65,-9.41)) ;
#140844=CARTESIAN_POINT('Origin',(-3.65,10.65,-9.41)) ;
#140845=CARTESIAN_POINT('',(-3.75,10.65,-10.91)) ;
#140846=CARTESIAN_POINT('',(-3.75,10.65,-10.91)) ;
#140847=CARTESIAN_POINT('',(-3.65,10.65,-11.01)) ;
#140848=CARTESIAN_POINT('Origin',(-3.65,10.65,-10.91)) ;
#140849=CARTESIAN_POINT('',(-2.9,10.65,-11.01)) ;
#140850=CARTESIAN_POINT('',(-2.9,10.65,-11.01)) ;
#140851=CARTESIAN_POINT('',(-2.8,10.65,-10.91)) ;
#140852=CARTESIAN_POINT('Origin',(-2.9,10.65,-10.91)) ;
#140853=CARTESIAN_POINT('',(-2.8,10.65,-9.41)) ;
#140854=CARTESIAN_POINT('',(-2.8,10.65,-9.41)) ;
#140855=CARTESIAN_POINT('Origin',(-2.9,10.65,-9.41)) ;
#140856=CARTESIAN_POINT('Origin',(-2.9,10.65,-9.41)) ;
#140857=CARTESIAN_POINT('',(-2.8,10.7,-9.41)) ;
#140858=CARTESIAN_POINT('',(-2.8,10.65,-9.41)) ;
#140859=CARTESIAN_POINT('',(-2.9,10.7,-9.31)) ;
#140860=CARTESIAN_POINT('Origin',(-2.9,10.7,-9.41)) ;
#140861=CARTESIAN_POINT('',(-2.9,10.65,-9.31)) ;
#140862=CARTESIAN_POINT('Origin',(-3.65,10.65,-9.31)) ;
#140863=CARTESIAN_POINT('',(-3.65,10.7,-9.31)) ;
#140864=CARTESIAN_POINT('',(-3.65,10.7,-9.31)) ;
#140865=CARTESIAN_POINT('',(-3.65,10.65,-9.31)) ;
#140866=CARTESIAN_POINT('Origin',(-3.65,10.65,-9.41)) ;
#140867=CARTESIAN_POINT('',(-3.75,10.7,-9.41)) ;
#140868=CARTESIAN_POINT('Origin',(-3.65,10.7,-9.41)) ;
#140869=CARTESIAN_POINT('',(-3.75,10.65,-9.41)) ;
#140870=CARTESIAN_POINT('Origin',(-3.75,10.65,-10.91)) ;
#140871=CARTESIAN_POINT('',(-3.75,10.7,-10.91)) ;
#140872=CARTESIAN_POINT('',(-3.75,10.7,-10.91)) ;
#140873=CARTESIAN_POINT('',(-3.75,10.65,-10.91)) ;
#140874=CARTESIAN_POINT('Origin',(-3.65,10.65,-10.91)) ;
#140875=CARTESIAN_POINT('',(-3.65,10.7,-11.01)) ;
#140876=CARTESIAN_POINT('Origin',(-3.65,10.7,-10.91)) ;
#140877=CARTESIAN_POINT('',(-3.65,10.65,-11.01)) ;
#140878=CARTESIAN_POINT('Origin',(-2.9,10.65,-11.01)) ;
#140879=CARTESIAN_POINT('',(-2.9,10.7,-11.01)) ;
#140880=CARTESIAN_POINT('',(-2.9,10.7,-11.01)) ;
#140881=CARTESIAN_POINT('',(-2.9,10.65,-11.01)) ;
#140882=CARTESIAN_POINT('Origin',(-2.9,10.65,-10.91)) ;
#140883=CARTESIAN_POINT('',(-2.8,10.7,-10.91)) ;
#140884=CARTESIAN_POINT('Origin',(-2.9,10.7,-10.91)) ;
#140885=CARTESIAN_POINT('',(-2.8,10.65,-10.91)) ;
#140886=CARTESIAN_POINT('Origin',(-2.8,10.65,-9.41)) ;
#140887=CARTESIAN_POINT('',(-2.8,10.7,-9.41)) ;
#140888=CARTESIAN_POINT('Origin',(0.,10.8,-10.16)) ;
#140889=CARTESIAN_POINT('',(-3.65,10.8,-9.41)) ;
#140890=CARTESIAN_POINT('',(-2.9,10.8,-9.41)) ;
#140891=CARTESIAN_POINT('',(0.,10.8,-9.41)) ;
#140892=CARTESIAN_POINT('',(-2.9,10.8,-10.91)) ;
#140893=CARTESIAN_POINT('',(-2.9,10.8,-10.16)) ;
#140894=CARTESIAN_POINT('',(-3.65,10.8,-10.91)) ;
#140895=CARTESIAN_POINT('',(0.,10.8,-10.91)) ;
#140896=CARTESIAN_POINT('',(-3.65,10.8,-10.16)) ;
#140897=CARTESIAN_POINT('Origin',(4.5,2.75,-11.535)) ;
#140898=CARTESIAN_POINT('',(4.5,2.63356010126946,-11.5544066497884)) ;
#140899=CARTESIAN_POINT('',(4.6,2.11643989873054,-11.6405933502116)) ;
#140900=CARTESIAN_POINT('',(4.6,2.11643989873054,-11.6405933502116)) ;
#140901=CARTESIAN_POINT('',(12.7,2.11643989873054,-11.6405933502116)) ;
#140902=CARTESIAN_POINT('',(12.8,2.11643989873054,-11.6405933502116)) ;
#140903=CARTESIAN_POINT('',(12.7,2.75,-11.535)) ;
#140904=CARTESIAN_POINT('Origin',(4.5,2.,-11.66)) ;
#140905=CARTESIAN_POINT('',(4.6,2.,-11.5419539578284)) ;
#140906=CARTESIAN_POINT('',(4.6,2.,-8.66)) ;
#140907=CARTESIAN_POINT('',(12.7,2.,-11.5419539578284)) ;
#140908=CARTESIAN_POINT('',(12.7,2.,-11.66)) ;
#140909=CARTESIAN_POINT('',(4.5,2.,-11.5419539578284)) ;
#140910=CARTESIAN_POINT('Origin',(4.5,2.,-8.66)) ;
#140911=CARTESIAN_POINT('',(4.6,2.63356010126946,-8.76559335021158)) ;
#140912=CARTESIAN_POINT('',(4.6,2.63356010126947,-8.76559335021158)) ;
#140913=CARTESIAN_POINT('',(4.5,2.63356010126946,-8.76559335021158)) ;
#140914=CARTESIAN_POINT('',(12.7,2.,-8.66)) ;
#140915=CARTESIAN_POINT('Origin',(4.5,0.,-10.16)) ;
#140916=CARTESIAN_POINT('',(4.5,2.72431432344521,-8.85263481664499)) ;
#140917=CARTESIAN_POINT('',(4.5,2.72431432344521,-10.16)) ;
#140918=CARTESIAN_POINT('',(4.5,2.61712020253893,-8.86423274259479)) ;
#140919=CARTESIAN_POINT('Origin',(4.5,2.65,-8.66695395782836)) ;
#140920=CARTESIAN_POINT('',(4.5,2.1,-8.77804604217164)) ;
#140921=CARTESIAN_POINT('',(4.5,2.1,-8.77804604217164)) ;
#140922=CARTESIAN_POINT('',(4.5,2.1,-11.5419539578284)) ;
#140923=CARTESIAN_POINT('',(4.5,2.1,-11.66)) ;
#140924=CARTESIAN_POINT('',(4.5,2.61712020253893,-11.4557672574052)) ;
#140925=CARTESIAN_POINT('Origin',(10.3,0.,-10.16)) ;
#140926=CARTESIAN_POINT('Origin',(0.584645609909621,0.,-10.16)) ;
#140927=CARTESIAN_POINT('',(4.6,-2.32258064516129,-8.2611532060953)) ;
#140928=CARTESIAN_POINT('',(4.6,-2.79310344827574,-9.06520635404194)) ;
#140929=CARTESIAN_POINT('Origin',(4.6,0.,-10.16)) ;
#140930=CARTESIAN_POINT('',(4.6,-2.79310344827574,-11.2547936459581)) ;
#140931=CARTESIAN_POINT('Origin',(4.6,0.,-10.16)) ;
#140932=CARTESIAN_POINT('',(4.6,-2.32258064516129,-12.0588467939047)) ;
#140933=CARTESIAN_POINT('Origin',(4.6,0.,-10.16)) ;
#140934=CARTESIAN_POINT('',(12.7,-2.32258064516129,-12.0588467939047)) ;
#140935=CARTESIAN_POINT('',(0.584645609909621,-2.32258064516129,-12.0588467939047)) ;
#140936=CARTESIAN_POINT('',(12.7,-2.32258064516129,-8.2611532060953)) ;
#140937=CARTESIAN_POINT('Origin',(12.7,0.,-10.16)) ;
#140938=CARTESIAN_POINT('',(0.584645609909621,-2.32258064516129,-8.2611532060953)) ;
#140939=CARTESIAN_POINT('Ctrl Pts',(-5.37474093186837,4.17158354835192,
-8.26)) ;
#140940=CARTESIAN_POINT('Ctrl Pts',(-5.4,4.2,-8.26)) ;
#140941=CARTESIAN_POINT('Ctrl Pts',(-5.4,4.23801993223491,-8.26)) ;
#140942=CARTESIAN_POINT('Ctrl Pts',(-5.37474093064202,4.17158354697228,
-8.23374656406105)) ;
#140943=CARTESIAN_POINT('Ctrl Pts',(-5.4,4.19999999724801,-8.22248141279891)) ;
#140944=CARTESIAN_POINT('Ctrl Pts',(-5.4,4.23801992976516,-8.20749312809024)) ;
#140945=CARTESIAN_POINT('Ctrl Pts',(-5.36668583490655,4.14629949399955,
-8.20780128688413)) ;
#140946=CARTESIAN_POINT('Ctrl Pts',(-5.4,4.16739198385624,-8.18466783506585)) ;
#140947=CARTESIAN_POINT('Ctrl Pts',(-5.4,4.20557579169425,-8.15560257376828)) ;
#140948=CARTESIAN_POINT('Ctrl Pts',(-5.3390138046061,4.05944006555646,-8.17077735687856)) ;
#140949=CARTESIAN_POINT('Ctrl Pts',(-5.4,4.06625640449639,-8.14313263661412)) ;
#140950=CARTESIAN_POINT('Ctrl Pts',(-5.4,4.09411900298411,-8.0815547137571)) ;
#140951=CARTESIAN_POINT('Ctrl Pts',(-5.31962206268973,3.99857154231912,
-8.16)) ;
#140952=CARTESIAN_POINT('Ctrl Pts',(-5.4,3.99346933127518,-8.14200350742663)) ;
#140953=CARTESIAN_POINT('Ctrl Pts',(-5.4,4.0160133758189,-8.06000000048129)) ;
#140954=CARTESIAN_POINT('Ctrl Pts',(-5.3,3.9369800677651,-8.16)) ;
#140955=CARTESIAN_POINT('Ctrl Pts',(-5.4,3.9369800677651,-8.16)) ;
#140956=CARTESIAN_POINT('Ctrl Pts',(-5.4,3.9369800677651,-8.06)) ;
#140957=CARTESIAN_POINT('Origin',(-5.3,4.23801993223491,-8.26)) ;
#140958=CARTESIAN_POINT('Ctrl Pts',(-5.3,3.9369800677651,-8.16)) ;
#140959=CARTESIAN_POINT('Ctrl Pts',(-5.31962206268973,3.99857154231912,
-8.16)) ;
#140960=CARTESIAN_POINT('Ctrl Pts',(-5.3390138046061,4.05944006555646,-8.17077735687856)) ;
#140961=CARTESIAN_POINT('Ctrl Pts',(-5.36668583490655,4.14629949399955,
-8.20780128688413)) ;
#140962=CARTESIAN_POINT('Ctrl Pts',(-5.37474093064202,4.17158354697228,
-8.23374656406105)) ;
#140963=CARTESIAN_POINT('Ctrl Pts',(-5.37474093186837,4.17158354835192,
-8.26)) ;
#140964=CARTESIAN_POINT('Origin',(-5.3,3.9369800677651,-8.06)) ;
#140965=CARTESIAN_POINT('Origin',(-4.6737453090477,1.85,-8.25713990064968)) ;
#140966=CARTESIAN_POINT('Origin',(-3.35509339356897,1.85,-8.57947703554448)) ;
#140967=CARTESIAN_POINT('Ctrl Pts',(-3.35509339356897,1.95,-8.57947703554448)) ;
#140968=CARTESIAN_POINT('Ctrl Pts',(-3.33134808452128,1.95,-8.4823371348948)) ;
#140969=CARTESIAN_POINT('Ctrl Pts',(-3.33134808452128,1.85,-8.4823371348948)) ;
#140970=CARTESIAN_POINT('Ctrl Pts',(-3.38343213690417,1.95,-8.56562253880276)) ;
#140971=CARTESIAN_POINT('Ctrl Pts',(-3.36046743872483,1.94345445676969,
-8.47521907053384)) ;
#140972=CARTESIAN_POINT('Ctrl Pts',(-3.38803897426454,1.85000000162387,
-8.46847936184645)) ;
#140973=CARTESIAN_POINT('Ctrl Pts',(-3.41101314049054,1.96238978305186,
-8.55213849291617)) ;
#140974=CARTESIAN_POINT('Ctrl Pts',(-3.39538881861723,1.95068928167334,
-8.46668273322692)) ;
#140975=CARTESIAN_POINT('Ctrl Pts',(-3.44316973238525,1.87475949194143,
-8.45500295430583)) ;
#140976=CARTESIAN_POINT('Ctrl Pts',(-3.42983432543734,1.98356361611701,
-8.54293702440883)) ;
#140977=CARTESIAN_POINT('Ctrl Pts',(-3.42093333711585,1.97355000425533,
-8.4604385175939)) ;
#140978=CARTESIAN_POINT('Ctrl Pts',(-3.48082994825801,1.91712723223402,
-8.44579712375915)) ;
#140979=CARTESIAN_POINT('Origin',(-3.50457525730571,1.91712723223402,-8.54293702440883)) ;
#140980=CARTESIAN_POINT('Origin',(-3.36128627567764,2.03621361435732,-8.57644940433519)) ;
#140981=CARTESIAN_POINT('Origin',(-4.05330900605469,2.53445269957662,-8.40880210804797)) ;
#140982=CARTESIAN_POINT('Origin',(-4.66204490261456,3.21928058320648,-8.26)) ;
#140983=CARTESIAN_POINT('Origin',(-4.35749955255802,2.87666706439287,-8.26)) ;
#140984=CARTESIAN_POINT('Origin',(-4.66204490261456,3.21928058320648,-8.26)) ;
#140985=CARTESIAN_POINT('Origin',(-5.3,5.2,-8.06)) ;
#140986=CARTESIAN_POINT('Origin',(-5.3,-1.88819660112502,-8.06)) ;
#140987=CARTESIAN_POINT('Origin',(-5.3,4.23801993223491,-7.62)) ;
#140988=CARTESIAN_POINT('Origin',(-5.3,4.23801993223491,-12.06)) ;
#140989=CARTESIAN_POINT('Origin',(-3.35509339356897,2.05,-10.16)) ;
#140990=CARTESIAN_POINT('Origin',(-3.36128627567776,2.03621361435703,-11.7435505956648)) ;
#140991=CARTESIAN_POINT('Origin',(-2.4237453090477,1.85,-11.5128600993503)) ;
#140992=CARTESIAN_POINT('Origin',(-3.35509339356897,1.85,-11.7405229644555)) ;
#140993=CARTESIAN_POINT('Origin',(-4.66204490261456,3.21928058320648,-8.26)) ;
#140994=CARTESIAN_POINT('Origin',(-4.66204490261456,3.21928058320648,-8.26)) ;
#140995=CARTESIAN_POINT('Ctrl Pts',(-5.29976814257748,-1.88802911972919,
-8.15999982737782)) ;
#140996=CARTESIAN_POINT('Ctrl Pts',(-5.4,-1.88802831720456,-8.16023259354297)) ;
#140997=CARTESIAN_POINT('Ctrl Pts',(-5.4,-1.88791746283072,-8.06000016246237)) ;
#140998=CARTESIAN_POINT('Ctrl Pts',(-5.31153957531165,-1.92331224822998,
-8.15998646768893)) ;
#140999=CARTESIAN_POINT('Ctrl Pts',(-5.4,-1.92148676945297,-8.14897789253814)) ;
#141000=CARTESIAN_POINT('Ctrl Pts',(-5.4,-1.94671708614658,-8.05993171302843)) ;
#141001=CARTESIAN_POINT('Ctrl Pts',(-5.32318090226696,-1.95817527052249,
-8.17078449726811)) ;
#141002=CARTESIAN_POINT('Ctrl Pts',(-5.4,-1.96527310172483,-8.15216338375281)) ;
#141003=CARTESIAN_POINT('Ctrl Pts',(-5.4,-2.00485091174287,-8.08149607488934)) ;
#141004=CARTESIAN_POINT('Ctrl Pts',(-5.33978950165955,-2.00789652656156,
-8.20786496501965)) ;
#141005=CARTESIAN_POINT('Ctrl Pts',(-5.4,-2.02908601268744,-8.1913665145317)) ;
#141006=CARTESIAN_POINT('Ctrl Pts',(-5.4,-2.08777005652399,-8.15566121263604)) ;
#141007=CARTESIAN_POINT('Ctrl Pts',(-5.34461954754097,-2.02234798681676,
-8.2338461447183)) ;
#141008=CARTESIAN_POINT('Ctrl Pts',(-5.4,-2.04997459329993,-8.22567566483998)) ;
#141009=CARTESIAN_POINT('Ctrl Pts',(-5.4,-2.1118797455067,-8.20765768697394)) ;
#141010=CARTESIAN_POINT('Ctrl Pts',(-5.34460423617423,-2.02230212313483,
-8.26012475187013)) ;
#141011=CARTESIAN_POINT('Ctrl Pts',(-5.4,-2.04990938338631,-8.26016375427653)) ;
#141012=CARTESIAN_POINT('Ctrl Pts',(-5.4,-2.11180321723903,-8.26024966888043)) ;
#141013=CARTESIAN_POINT('Origin',(-5.29999999999998,-1.88819660112496,-8.26000000000004)) ;
#141014=CARTESIAN_POINT('Origin',(-5.3,-2.11180339887499,-8.26)) ;
#141015=CARTESIAN_POINT('Ctrl Pts',(-5.3,3.9369800677651,-12.16)) ;
#141016=CARTESIAN_POINT('Ctrl Pts',(-5.4,3.9369800677651,-12.16)) ;
#141017=CARTESIAN_POINT('Ctrl Pts',(-5.4,3.9369800677651,-12.26)) ;
#141018=CARTESIAN_POINT('Ctrl Pts',(-5.31962206268973,3.9985715423191,-12.16)) ;
#141019=CARTESIAN_POINT('Ctrl Pts',(-5.40000000000019,3.99346933127519,
-12.1779964925734)) ;
#141020=CARTESIAN_POINT('Ctrl Pts',(-5.4,4.01601337581888,-12.2599999995187)) ;
#141021=CARTESIAN_POINT('Ctrl Pts',(-5.33901380460608,4.05944006555649,
-12.1492226431214)) ;
#141022=CARTESIAN_POINT('Ctrl Pts',(-5.39999999999997,4.06625640449642,
-12.1768673633858)) ;
#141023=CARTESIAN_POINT('Ctrl Pts',(-5.4,4.09411900298413,-12.2384452862428)) ;
#141024=CARTESIAN_POINT('Ctrl Pts',(-5.36668583490657,4.14629949399951,
-12.1121987131159)) ;
#141025=CARTESIAN_POINT('Ctrl Pts',(-5.40000000000003,4.16739198385622,
-12.1353321649343)) ;
#141026=CARTESIAN_POINT('Ctrl Pts',(-5.4,4.20557579169423,-12.1643974262318)) ;
#141027=CARTESIAN_POINT('Ctrl Pts',(-5.37474093064202,4.17158354697228,
-12.0862534359389)) ;
#141028=CARTESIAN_POINT('Ctrl Pts',(-5.4,4.19999999724801,-12.097518587201)) ;
#141029=CARTESIAN_POINT('Ctrl Pts',(-5.4,4.23801992976516,-12.1125068719097)) ;
#141030=CARTESIAN_POINT('Ctrl Pts',(-5.37474093186837,4.17158354835192,
-12.06)) ;
#141031=CARTESIAN_POINT('Ctrl Pts',(-5.4,4.2,-12.06)) ;
#141032=CARTESIAN_POINT('Ctrl Pts',(-5.4,4.23801993223491,-12.06)) ;
#141033=CARTESIAN_POINT('Origin',(-5.3,3.9369800677651,-12.26)) ;
#141034=CARTESIAN_POINT('Ctrl Pts',(-5.37474093186837,4.17158354835192,
-12.06)) ;
#141035=CARTESIAN_POINT('Ctrl Pts',(-5.37474093064202,4.17158354697228,
-12.0862534359389)) ;
#141036=CARTESIAN_POINT('Ctrl Pts',(-5.36668583490657,4.14629949399951,
-12.1121987131159)) ;
#141037=CARTESIAN_POINT('Ctrl Pts',(-5.33901380460608,4.05944006555649,
-12.1492226431214)) ;
#141038=CARTESIAN_POINT('Ctrl Pts',(-5.31962206268973,3.9985715423191,-12.16)) ;
#141039=CARTESIAN_POINT('Ctrl Pts',(-5.3,3.9369800677651,-12.16)) ;
#141040=CARTESIAN_POINT('Ctrl Pts',(-3.42983432543734,1.98356361611701,
-11.7770629755912)) ;
#141041=CARTESIAN_POINT('Ctrl Pts',(-3.42093333711585,1.97355000425533,
-11.8595614824061)) ;
#141042=CARTESIAN_POINT('Ctrl Pts',(-3.48082994825801,1.91712723223402,
-11.8742028762408)) ;
#141043=CARTESIAN_POINT('Ctrl Pts',(-3.41101314049054,1.96238978305186,
-11.7678615070838)) ;
#141044=CARTESIAN_POINT('Ctrl Pts',(-3.39538881861728,1.95068928167332,
-11.8533172667731)) ;
#141045=CARTESIAN_POINT('Ctrl Pts',(-3.44316973238528,1.87475949194142,
-11.8649970456942)) ;
#141046=CARTESIAN_POINT('Ctrl Pts',(-3.38343213690417,1.95,-11.7543774611972)) ;
#141047=CARTESIAN_POINT('Ctrl Pts',(-3.36046743872479,1.94345445676969,
-11.8447809294662)) ;
#141048=CARTESIAN_POINT('Ctrl Pts',(-3.38803897426452,1.85000000162387,
-11.8515206381536)) ;
#141049=CARTESIAN_POINT('Ctrl Pts',(-3.35509339356897,1.95,-11.7405229644555)) ;
#141050=CARTESIAN_POINT('Ctrl Pts',(-3.33134808452128,1.95,-11.8376628651052)) ;
#141051=CARTESIAN_POINT('Ctrl Pts',(-3.33134808452128,1.85,-11.8376628651052)) ;
#141052=CARTESIAN_POINT('Origin',(-3.50457525730571,1.91712723223402,-11.7770629755912)) ;
#141053=CARTESIAN_POINT('Origin',(-4.66204490261456,1.95,-8.26)) ;
#141054=CARTESIAN_POINT('Origin',(-4.66204490261456,-1.5692190524323,-8.26)) ;
#141055=CARTESIAN_POINT('Origin',(-3.84472135955,-1.16055728090002,-8.26)) ;
#141056=CARTESIAN_POINT('Origin',(-4.66204490261456,-1.5692190524323,-8.26)) ;
#141057=CARTESIAN_POINT('Origin',(-5.3,-2.11180339887499,-7.62)) ;
#141058=CARTESIAN_POINT('Origin',(-5.3,-2.11180339887499,-12.06)) ;
#141059=CARTESIAN_POINT('Origin',(-5.3,1.95,-12.26)) ;
#141060=CARTESIAN_POINT('Origin',(-5.3,-1.88819660112501,-12.26)) ;
#141061=CARTESIAN_POINT('Origin',(-4.0264650697994,2.50425327128942,-12.06)) ;
#141062=CARTESIAN_POINT('Origin',(-4.66204490261456,3.21928058320648,-12.06)) ;
#141063=CARTESIAN_POINT('Origin',(-3.02790825149799,1.38087685070033,-11.6605443741715)) ;
#141064=CARTESIAN_POINT('Origin',(-4.66204490261456,3.21928058320648,-12.06)) ;
#141065=CARTESIAN_POINT('Origin',(-4.66204490261456,-1.5692190524323,-8.26)) ;
#141066=CARTESIAN_POINT('Origin',(-4.66204490261456,-1.5692190524323,-8.26)) ;
#141067=CARTESIAN_POINT('Ctrl Pts',(-5.34460423617423,-2.02230212313483,
-12.0598752481299)) ;
#141068=CARTESIAN_POINT('Ctrl Pts',(-5.4,-2.04990938338631,-12.0598362457235)) ;
#141069=CARTESIAN_POINT('Ctrl Pts',(-5.4,-2.11180321723903,-12.0597503311196)) ;
#141070=CARTESIAN_POINT('Ctrl Pts',(-5.34461954754098,-2.02234798681676,
-12.0861538552817)) ;
#141071=CARTESIAN_POINT('Ctrl Pts',(-5.4,-2.04997459329993,-12.09432433516)) ;
#141072=CARTESIAN_POINT('Ctrl Pts',(-5.4,-2.1118797455067,-12.1123423130261)) ;
#141073=CARTESIAN_POINT('Ctrl Pts',(-5.33978950165958,-2.00789652656157,
-12.1121350349804)) ;
#141074=CARTESIAN_POINT('Ctrl Pts',(-5.4,-2.02908601268744,-12.1286334854683)) ;
#141075=CARTESIAN_POINT('Ctrl Pts',(-5.4,-2.08777005652399,-12.164338787364)) ;
#141076=CARTESIAN_POINT('Ctrl Pts',(-5.32318090226695,-1.95817527052248,
-12.1492155027319)) ;
#141077=CARTESIAN_POINT('Ctrl Pts',(-5.4,-1.96527310172483,-12.1678366162472)) ;
#141078=CARTESIAN_POINT('Ctrl Pts',(-5.4,-2.00485091174288,-12.2385039251107)) ;
#141079=CARTESIAN_POINT('Ctrl Pts',(-5.31153957531166,-1.92331224822999,
-12.1600135323111)) ;
#141080=CARTESIAN_POINT('Ctrl Pts',(-5.40000000000019,-1.92148676945297,
-12.1710221074619)) ;
#141081=CARTESIAN_POINT('Ctrl Pts',(-5.4,-1.94671708614658,-12.2600682869716)) ;
#141082=CARTESIAN_POINT('Ctrl Pts',(-5.29976814257748,-1.88802911972919,
-12.1600001726222)) ;
#141083=CARTESIAN_POINT('Ctrl Pts',(-5.4,-1.88802831720457,-12.159767406457)) ;
#141084=CARTESIAN_POINT('Ctrl Pts',(-5.4,-1.88791746283074,-12.2599998375376)) ;
#141085=CARTESIAN_POINT('Origin',(-5.30000000000005,-1.88819660112517,-12.0600000000001)) ;
#141086=CARTESIAN_POINT('Origin',(-4.66204490261456,3.21928058320648,-12.06)) ;
#141087=CARTESIAN_POINT('Origin',(-4.66204490261456,3.21928058320648,-12.06)) ;
#141088=CARTESIAN_POINT('Origin',(0.175392621986784,-0.95,-9.44248472823589)) ;
#141089=CARTESIAN_POINT('Origin',(-3.37639320225,-0.95,-8.57427041564467)) ;
#141090=CARTESIAN_POINT('Origin',(-3.32804538583365,-0.902219294041845,
-8.58608877076867)) ;
#141091=CARTESIAN_POINT('Origin',(-3.46583592134999,-0.971114561800017,
-8.55240663986467)) ;
#141092=CARTESIAN_POINT('Origin',(-3.24472135955,-0.860557280900019,-12.06)) ;
#141093=CARTESIAN_POINT('Origin',(-4.66204490261456,-1.5692190524323,-12.06)) ;
#141094=CARTESIAN_POINT('Origin',(-4.66204490261456,1.95,-12.06)) ;
#141095=CARTESIAN_POINT('Origin',(-4.66204490261456,-1.5692190524323,-12.06)) ;
#141096=CARTESIAN_POINT('Ctrl Pts',(-3.4211145618,-1.06055728090001,-8.55240663986467)) ;
#141097=CARTESIAN_POINT('Ctrl Pts',(-3.40394191641935,-1.05197095820969,
-8.46459197598638)) ;
#141098=CARTESIAN_POINT('Ctrl Pts',(-3.44209061230229,-0.971114561800017,
-8.455266739215)) ;
#141099=CARTESIAN_POINT('Ctrl Pts',(-3.40727897628737,-1.05363948814369,
-8.55917070399163)) ;
#141100=CARTESIAN_POINT('Ctrl Pts',(-3.38665319245547,-1.04670310838587,
-8.46881810851093)) ;
#141101=CARTESIAN_POINT('Ctrl Pts',(-3.4144159452097,-0.957277229261619,
-8.46203165783763)) ;
#141102=CARTESIAN_POINT('Ctrl Pts',(-3.39186274464429,-1.05,-8.56670752825188)) ;
#141103=CARTESIAN_POINT('Ctrl Pts',(-3.36870744055524,-1.04639008266724,
-8.47320484786421)) ;
#141104=CARTESIAN_POINT('Ctrl Pts',(-3.38358960366098,-0.950000000886305,
-8.46956698577176)) ;
#141105=CARTESIAN_POINT('Ctrl Pts',(-3.37639320225,-1.05,-8.57427041564467)) ;
#141106=CARTESIAN_POINT('Ctrl Pts',(-3.3526478932023,-1.05,-8.47713051499499)) ;
#141107=CARTESIAN_POINT('Ctrl Pts',(-3.3526478932023,-0.95,-8.47713051499499)) ;
#141108=CARTESIAN_POINT('Origin',(-3.37639320224955,-1.15000000000196,-8.57427041564492)) ;
#141109=CARTESIAN_POINT('Origin',(-4.66204490261456,-1.5692190524323,-12.06)) ;
#141110=CARTESIAN_POINT('Origin',(-4.66204490261456,-1.5692190524323,-12.06)) ;
#141111=CARTESIAN_POINT('Origin',(-3.37639320225,-1.15,-10.16)) ;
#141112=CARTESIAN_POINT('Origin',(-3.37639320224944,-1.15000000000305,-11.745729584355)) ;
#141113=CARTESIAN_POINT('Origin',(-1.50751564693271,0.00804557540861825,
-11.2888928486111)) ;
#141114=CARTESIAN_POINT('Origin',(-3.46583592134999,-0.971114561800017,
-11.7675933601353)) ;
#141115=CARTESIAN_POINT('Ctrl Pts',(-3.37639320225,-1.05,-11.7457295843553)) ;
#141116=CARTESIAN_POINT('Ctrl Pts',(-3.3526478932023,-1.05,-11.842869485005)) ;
#141117=CARTESIAN_POINT('Ctrl Pts',(-3.3526478932023,-0.95,-11.842869485005)) ;
#141118=CARTESIAN_POINT('Ctrl Pts',(-3.3918627446443,-1.05,-11.7532924717481)) ;
#141119=CARTESIAN_POINT('Ctrl Pts',(-3.36870744055522,-1.04639008266722,
-11.8467951521358)) ;
#141120=CARTESIAN_POINT('Ctrl Pts',(-3.38358960366098,-0.950000000886305,
-11.8504330142282)) ;
#141121=CARTESIAN_POINT('Ctrl Pts',(-3.40727897628736,-1.05363948814369,
-11.7608292960084)) ;
#141122=CARTESIAN_POINT('Ctrl Pts',(-3.38665319245549,-1.04670310838587,
-11.8511818914891)) ;
#141123=CARTESIAN_POINT('Ctrl Pts',(-3.41441594520969,-0.957277229261623,
-11.8579683421624)) ;
#141124=CARTESIAN_POINT('Ctrl Pts',(-3.4211145618,-1.06055728090001,-11.7675933601353)) ;
#141125=CARTESIAN_POINT('Ctrl Pts',(-3.40394191641935,-1.05197095820969,
-11.8554080240136)) ;
#141126=CARTESIAN_POINT('Ctrl Pts',(-3.44209061230229,-0.971114561800017,
-11.864733260785)) ;
#141127=CARTESIAN_POINT('Origin',(-3.37639320225,-0.95,-11.7457295843553)) ;
#141128=CARTESIAN_POINT('Origin',(0.175392621986784,-0.95,-10.8775152717641)) ;
#141129=CARTESIAN_POINT('Origin',(12.7,2.65,-7.62)) ;
#141130=CARTESIAN_POINT('Origin',(12.8,2.65,-11.6530460421716)) ;
#141131=CARTESIAN_POINT('',(4.57524318173533,2.73534903669982,-11.6009351802097)) ;
#141132=CARTESIAN_POINT('Origin',(4.65232986199875,2.66527023615951,-11.6487542111836)) ;
#141133=CARTESIAN_POINT('Ctrl Pts',(4.57524318173533,2.73534903669982,-11.6009351802097)) ;
#141134=CARTESIAN_POINT('Ctrl Pts',(4.5761458558036,2.73452842391049,-11.5995911511832)) ;
#141135=CARTESIAN_POINT('Ctrl Pts',(4.57705238626145,2.73367683201793,-11.5982681293393)) ;
#141136=CARTESIAN_POINT('Ctrl Pts',(4.5779495181309,2.73280244902548,-11.5969768488888)) ;
#141137=CARTESIAN_POINT('Ctrl Pts',(4.58144263576927,2.72939790755547,-11.5919490545686)) ;
#141138=CARTESIAN_POINT('Ctrl Pts',(4.58496694799967,2.72549786515199,-11.5871699445181)) ;
#141139=CARTESIAN_POINT('Ctrl Pts',(4.58815670056882,2.72107165565079,-11.582698193853)) ;
#141140=CARTESIAN_POINT('Ctrl Pts',(4.5906912384746,2.71755464437279,-11.5791449961299)) ;
#141141=CARTESIAN_POINT('Ctrl Pts',(4.59301454561848,2.7137045982392,-11.5757863127243)) ;
#141142=CARTESIAN_POINT('Ctrl Pts',(4.5949431309995,2.70950205848694,-11.5726749961674)) ;
#141143=CARTESIAN_POINT('Ctrl Pts',(4.59651854606295,2.70606910472943,-11.5701334364214)) ;
#141144=CARTESIAN_POINT('Ctrl Pts',(4.59783685868322,2.70233705077422,-11.5677160861571)) ;
#141145=CARTESIAN_POINT('Ctrl Pts',(4.59873118971425,2.69838744819993,-11.5655323012123)) ;
#141146=CARTESIAN_POINT('Ctrl Pts',(4.59916508318199,2.69647125978905,-11.5644728165364)) ;
#141147=CARTESIAN_POINT('Ctrl Pts',(4.59949917984823,2.69450444432188,-11.563467798882)) ;
#141148=CARTESIAN_POINT('Ctrl Pts',(4.5997144226265,2.692499226592,-11.5625263440994)) ;
#141149=CARTESIAN_POINT('Ctrl Pts',(4.59990113259977,2.69075982259552,-11.5617096895352)) ;
#141150=CARTESIAN_POINT('Ctrl Pts',(4.6,2.68896788689974,-11.5609303122145)) ;
#141151=CARTESIAN_POINT('Ctrl Pts',(4.6,2.68715716172261,-11.5602056127633)) ;
#141152=CARTESIAN_POINT('Origin',(4.5,2.1,-11.5419539578284)) ;
#141153=CARTESIAN_POINT('Origin',(4.6,2.1,-11.5419539578284)) ;
#141154=CARTESIAN_POINT('Origin',(12.7,2.1,-11.5419539578284)) ;
#141155=CARTESIAN_POINT('Origin',(12.7,2.76643989873054,-11.6336393923832)) ;
#141156=CARTESIAN_POINT('Origin',(12.7,2.13287979746107,-11.7392327425948)) ;
#141157=CARTESIAN_POINT('Origin',(4.4,2.72431432344521,-10.16)) ;
#141158=CARTESIAN_POINT('Ctrl Pts',(4.48762159086959,2.77250619842348,-8.77117568174948)) ;
#141159=CARTESIAN_POINT('Ctrl Pts',(4.48806820038223,2.77169418112776,-8.77383556708983)) ;
#141160=CARTESIAN_POINT('Ctrl Pts',(4.48852084821546,2.77084293101113,-8.77648271501847)) ;
#141161=CARTESIAN_POINT('Ctrl Pts',(4.49012932137854,2.76769877392855,-8.78576300952073)) ;
#141162=CARTESIAN_POINT('Ctrl Pts',(4.49131046584974,2.76517764467229,-8.79234413170344)) ;
#141163=CARTESIAN_POINT('Ctrl Pts',(4.49351977821776,2.75978760391033,-8.80463528016206)) ;
#141164=CARTESIAN_POINT('Ctrl Pts',(4.49455195297827,2.75697653750126,-8.8103677406013)) ;
#141165=CARTESIAN_POINT('Ctrl Pts',(4.49620670090465,2.75163165728875,-8.81994332160325)) ;
#141166=CARTESIAN_POINT('Ctrl Pts',(4.49686252944492,2.74924176842724,-8.82386402620333)) ;
#141167=CARTESIAN_POINT('Ctrl Pts',(4.49822764032849,2.74331716058958,-8.83264463163462)) ;
#141168=CARTESIAN_POINT('Ctrl Pts',(4.49890203357902,2.73961076902722,-8.8374865001603)) ;
#141169=CARTESIAN_POINT('Ctrl Pts',(4.49975897856021,2.73206576252699,-8.84582777843958)) ;
#141170=CARTESIAN_POINT('Ctrl Pts',(4.5,2.72833175948626,-8.84941900229172)) ;
#141171=CARTESIAN_POINT('Ctrl Pts',(4.5,2.72431432344521,-8.85263481664499)) ;
#141172=CARTESIAN_POINT('Ctrl Pts',(4.5,2.72431432344521,-11.467365183355)) ;
#141173=CARTESIAN_POINT('Ctrl Pts',(4.5,2.72904669151454,-11.4711532753139)) ;
#141174=CARTESIAN_POINT('Ctrl Pts',(4.4996664568447,2.73338556955604,-11.4754614101765)) ;
#141175=CARTESIAN_POINT('Ctrl Pts',(4.49869539480385,2.74072289096416,-11.483980241438)) ;
#141176=CARTESIAN_POINT('Ctrl Pts',(4.49811062025683,2.74382502998103,-11.4881080596589)) ;
#141177=CARTESIAN_POINT('Ctrl Pts',(4.49664125196624,2.7502021169969,-11.4975592649406)) ;
#141178=CARTESIAN_POINT('Ctrl Pts',(4.49570721389709,2.75339870015146,-11.5030103903194)) ;
#141179=CARTESIAN_POINT('Ctrl Pts',(4.49363760641474,2.75952863263957,-11.5147517051871)) ;
#141180=CARTESIAN_POINT('Ctrl Pts',(4.49249077386338,2.76240287369082,-11.521071225831)) ;
#141181=CARTESIAN_POINT('Ctrl Pts',(4.49055019898869,2.76677757270145,-11.531914125621)) ;
#141182=CARTESIAN_POINT('Ctrl Pts',(4.48975662823142,2.76842729450637,-11.5363872919227)) ;
#141183=CARTESIAN_POINT('Ctrl Pts',(4.4885208482156,2.77084293101086,-11.5435172849807)) ;
#141184=CARTESIAN_POINT('Ctrl Pts',(4.48806820038252,2.77169418112725,-11.5461644329085)) ;
#141185=CARTESIAN_POINT('Ctrl Pts',(4.48762159086959,2.77250619842348,-11.5488243182478)) ;
#141186=CARTESIAN_POINT('Origin',(4.6,2.1,-10.16)) ;
#141187=CARTESIAN_POINT('Origin',(4.6,2.1,-8.77804604217164)) ;
#141188=CARTESIAN_POINT('Origin',(4.6,2.1,-11.5419539578284)) ;
#141189=CARTESIAN_POINT('Origin',(12.7,2.1,-11.5419539578284)) ;
#141190=CARTESIAN_POINT('Origin',(12.7,1.9,-11.5419539578284)) ;
#141191=CARTESIAN_POINT('Origin',(12.7,2.65,-7.62)) ;
#141192=CARTESIAN_POINT('Origin',(4.5,2.65,-8.66695395782836)) ;
#141193=CARTESIAN_POINT('',(4.6,2.68715716172261,-8.75979438723668)) ;
#141194=CARTESIAN_POINT('',(4.57524318173443,2.73534903670064,-8.71906481978892)) ;
#141195=CARTESIAN_POINT('Ctrl Pts',(4.6,2.68715716172261,-8.75979438723667)) ;
#141196=CARTESIAN_POINT('Ctrl Pts',(4.6,2.6910603667141,-8.75823222277848)) ;
#141197=CARTESIAN_POINT('Ctrl Pts',(4.59952510519174,2.69488861888984,-8.75640970947472)) ;
#141198=CARTESIAN_POINT('Ctrl Pts',(4.59869497748256,2.69852743640765,-8.75439015122504)) ;
#141199=CARTESIAN_POINT('Ctrl Pts',(4.59815316003465,2.70090246232124,-8.75307200236116)) ;
#141200=CARTESIAN_POINT('Ctrl Pts',(4.59746001108779,2.70319720658045,-8.75167096804522)) ;
#141201=CARTESIAN_POINT('Ctrl Pts',(4.59664880273703,2.70538659711789,-8.7502145418985)) ;
#141202=CARTESIAN_POINT('Ctrl Pts',(4.59612777291939,2.70679281754376,-8.74927909609234)) ;
#141203=CARTESIAN_POINT('Ctrl Pts',(4.59555051815356,2.70817855133085,-8.74830492990722)) ;
#141204=CARTESIAN_POINT('Ctrl Pts',(4.59494172533681,2.70950512149367,-8.74732273606981)) ;
#141205=CARTESIAN_POINT('Ctrl Pts',(4.59250947890864,2.7148050288701,-8.74339867949909)) ;
#141206=CARTESIAN_POINT('Ctrl Pts',(4.58944857812998,2.71954517005242,-8.73908233758092)) ;
#141207=CARTESIAN_POINT('Ctrl Pts',(4.58612768646824,2.72376361218905,-8.73447380318381)) ;
#141208=CARTESIAN_POINT('Ctrl Pts',(4.58350334758182,2.72709724148711,-8.73083190297759)) ;
#141209=CARTESIAN_POINT('Ctrl Pts',(4.58071664514666,2.73010548898771,-8.72700599593156)) ;
#141210=CARTESIAN_POINT('Ctrl Pts',(4.5779495181309,2.73280244902547,-8.72302315111116)) ;
#141211=CARTESIAN_POINT('Ctrl Pts',(4.57705238626115,2.73367683201821,-8.72173187066024)) ;
#141212=CARTESIAN_POINT('Ctrl Pts',(4.576145855803,2.73452842391106,-8.72040884881589)) ;
#141213=CARTESIAN_POINT('Ctrl Pts',(4.57524318173443,2.73534903670064,-8.71906481978892)) ;
#141214=CARTESIAN_POINT('Origin',(4.65232986200533,2.66527023615349,-8.67124578881467)) ;
#141215=CARTESIAN_POINT('Origin',(4.6,2.65,-8.66695395782836)) ;
#141216=CARTESIAN_POINT('Origin',(12.7,1.9,-11.66)) ;
#141217=CARTESIAN_POINT('Origin',(12.7,2.01643989873054,-8.56136060761679)) ;
#141218=CARTESIAN_POINT('Origin',(-3.65,10.7,-9.41)) ;
#141219=CARTESIAN_POINT('Origin',(-3.65,10.7,-9.41)) ;
#141220=CARTESIAN_POINT('Origin',(-3.65,10.7,-9.41)) ;
#141221=CARTESIAN_POINT('Origin',(0.,10.7,-9.41)) ;
#141222=CARTESIAN_POINT('Origin',(-2.9,10.7,-9.41)) ;
#141223=CARTESIAN_POINT('Origin',(-3.65,10.7,-10.16)) ;
#141224=CARTESIAN_POINT('Origin',(-3.65,10.7,-10.91)) ;
#141225=CARTESIAN_POINT('Origin',(-2.9,10.7,-9.41)) ;
#141226=CARTESIAN_POINT('Origin',(-2.9,10.7,-9.41)) ;
#141227=CARTESIAN_POINT('Origin',(-3.65,10.7,-10.91)) ;
#141228=CARTESIAN_POINT('Origin',(-3.65,10.7,-10.91)) ;
#141229=CARTESIAN_POINT('Origin',(-2.9,10.7,-10.16)) ;
#141230=CARTESIAN_POINT('Origin',(-2.9,10.7,-10.91)) ;
#141231=CARTESIAN_POINT('Origin',(0.,10.7,-10.91)) ;
#141232=CARTESIAN_POINT('Origin',(-2.9,10.7,-10.91)) ;
#141233=CARTESIAN_POINT('Origin',(-2.9,10.7,-10.91)) ;
#141234=CARTESIAN_POINT('Origin',(-3.05,-3.95,-9.16)) ;
#141235=CARTESIAN_POINT('Origin',(-3.05,-3.95,-11.06)) ;
#141236=CARTESIAN_POINT('Origin',(-3.05,-3.95,-9.26)) ;
#141237=CARTESIAN_POINT('Origin',(-3.25,-3.95,-9.26)) ;
#141238=CARTESIAN_POINT('Origin',(-3.25,-3.95,-9.06)) ;
#141239=CARTESIAN_POINT('Origin',(-3.25,-3.95,-9.26)) ;
#141240=CARTESIAN_POINT('Origin',(-3.25,-3.95,-11.06)) ;
#141241=CARTESIAN_POINT('Origin',(-3.25,-3.95,-11.06)) ;
#141242=CARTESIAN_POINT('Origin',(-3.25,-3.95,-11.26)) ;
#141243=CARTESIAN_POINT('Origin',(-4.4,-3.95,-9.06)) ;
#141244=CARTESIAN_POINT('Origin',(-4.3,-3.95,-9.06)) ;
#141245=CARTESIAN_POINT('Origin',(-3.25,-3.9,-9.26)) ;
#141246=CARTESIAN_POINT('Origin',(-3.25,-3.85,-9.26)) ;
#141247=CARTESIAN_POINT('Origin',(-3.25,-3.85,-10.16)) ;
#141248=CARTESIAN_POINT('Origin',(-3.25,-3.85,-11.06)) ;
#141249=CARTESIAN_POINT('Origin',(-3.25,-3.85,-9.26)) ;
#141250=CARTESIAN_POINT('Origin',(-3.25,-3.9,-11.06)) ;
#141251=CARTESIAN_POINT('Origin',(-3.25,-3.85,-11.06)) ;
#141252=CARTESIAN_POINT('Origin',(-4.4,-3.95,-11.26)) ;
#141253=CARTESIAN_POINT('Origin',(-4.3,-3.95,-11.26)) ;
#141254=CARTESIAN_POINT('Origin',(-4.5,-3.95,-9.16)) ;
#141255=CARTESIAN_POINT('Origin',(-4.5,-3.95,-9.26)) ;
#141256=CARTESIAN_POINT('Origin',(-4.5,-3.95,-11.06)) ;
#141257=CARTESIAN_POINT('Origin',(-4.3,-3.95,-9.26)) ;
#141258=CARTESIAN_POINT('Origin',(-4.3,-3.95,-9.26)) ;
#141259=CARTESIAN_POINT('Origin',(-3.25,-3.85,-9.26)) ;
#141260=CARTESIAN_POINT('Origin',(-3.25,-3.85,-9.26)) ;
#141261=CARTESIAN_POINT('Origin',(-3.25,-3.85,-11.06)) ;
#141262=CARTESIAN_POINT('Origin',(-3.25,-3.85,-11.06)) ;
#141263=CARTESIAN_POINT('Origin',(-4.3,-3.95,-11.06)) ;
#141264=CARTESIAN_POINT('Origin',(-4.3,-3.95,-11.06)) ;
#141265=CARTESIAN_POINT('Origin',(-4.3,-3.9,-9.26)) ;
#141266=CARTESIAN_POINT('Origin',(-4.3,-3.85,-9.26)) ;
#141267=CARTESIAN_POINT('Origin',(-1.56125112837913E-16,-3.85,-9.26)) ;
#141268=CARTESIAN_POINT('Origin',(-4.3,-3.85,-9.26)) ;
#141269=CARTESIAN_POINT('Origin',(-1.56125112837913E-16,-3.85,-11.06)) ;
#141270=CARTESIAN_POINT('Origin',(-4.3,-3.85,-11.06)) ;
#141271=CARTESIAN_POINT('Origin',(-4.3,-3.9,-11.06)) ;
#141272=CARTESIAN_POINT('Origin',(-4.3,-3.85,-11.06)) ;
#141273=CARTESIAN_POINT('Origin',(-4.3,-3.85,-9.26)) ;
#141274=CARTESIAN_POINT('Origin',(-4.3,-3.85,-9.26)) ;
#141275=CARTESIAN_POINT('Origin',(-4.3,-3.85,-11.06)) ;
#141276=CARTESIAN_POINT('Origin',(-4.3,-3.85,-11.06)) ;
#141277=CARTESIAN_POINT('Origin',(-4.3,-3.85,-10.16)) ;
#141278=CARTESIAN_POINT('Origin',(-4.,10.85,-11.16)) ;
#141279=CARTESIAN_POINT('Origin',(-4.,10.85,-11.06)) ;
#141280=CARTESIAN_POINT('Origin',(-4.,10.85,-9.26)) ;
#141281=CARTESIAN_POINT('Origin',(-3.8,10.85,-9.26)) ;
#141282=CARTESIAN_POINT('Origin',(-3.8,10.85,-9.06)) ;
#141283=CARTESIAN_POINT('Origin',(-3.8,10.85,-9.26)) ;
#141284=CARTESIAN_POINT('Origin',(-3.8,10.85,-11.06)) ;
#141285=CARTESIAN_POINT('Origin',(-3.8,10.85,-11.06)) ;
#141286=CARTESIAN_POINT('Origin',(-3.8,10.85,-11.26)) ;
#141287=CARTESIAN_POINT('Origin',(-3.9,10.85,-9.06)) ;
#141288=CARTESIAN_POINT('Origin',(-2.75,10.85,-9.06)) ;
#141289=CARTESIAN_POINT('Origin',(-3.8,10.8,-9.26)) ;
#141290=CARTESIAN_POINT('Origin',(-3.8,10.75,-9.26)) ;
#141291=CARTESIAN_POINT('Origin',(-3.8,10.75,-10.16)) ;
#141292=CARTESIAN_POINT('Origin',(-3.8,10.75,-11.06)) ;
#141293=CARTESIAN_POINT('Origin',(-3.8,10.75,-9.26)) ;
#141294=CARTESIAN_POINT('Origin',(-3.8,10.8,-11.06)) ;
#141295=CARTESIAN_POINT('Origin',(-3.8,10.75,-11.06)) ;
#141296=CARTESIAN_POINT('Origin',(-3.9,10.85,-11.26)) ;
#141297=CARTESIAN_POINT('Origin',(-2.75,10.85,-11.26)) ;
#141298=CARTESIAN_POINT('Origin',(-2.55,10.85,-11.16)) ;
#141299=CARTESIAN_POINT('Origin',(-2.55,10.85,-9.26)) ;
#141300=CARTESIAN_POINT('Origin',(-2.55,10.85,-11.06)) ;
#141301=CARTESIAN_POINT('Origin',(-2.75,10.85,-9.26)) ;
#141302=CARTESIAN_POINT('Origin',(-2.75,10.85,-9.26)) ;
#141303=CARTESIAN_POINT('Origin',(-3.8,10.75,-9.26)) ;
#141304=CARTESIAN_POINT('Origin',(-3.8,10.75,-9.26)) ;
#141305=CARTESIAN_POINT('Origin',(-3.8,10.75,-11.06)) ;
#141306=CARTESIAN_POINT('Origin',(-3.8,10.75,-11.06)) ;
#141307=CARTESIAN_POINT('Origin',(-2.75,10.85,-11.06)) ;
#141308=CARTESIAN_POINT('Origin',(-2.75,10.85,-11.06)) ;
#141309=CARTESIAN_POINT('Origin',(-2.75,10.8,-9.26)) ;
#141310=CARTESIAN_POINT('Origin',(-2.75,10.75,-9.26)) ;
#141311=CARTESIAN_POINT('Origin',(1.56125112837912E-16,10.75,-9.26)) ;
#141312=CARTESIAN_POINT('Origin',(-2.75,10.75,-9.26)) ;
#141313=CARTESIAN_POINT('Origin',(-1.56125112837913E-16,10.75,-11.06)) ;
#141314=CARTESIAN_POINT('Origin',(-2.75,10.75,-11.06)) ;
#141315=CARTESIAN_POINT('Origin',(-2.75,10.8,-11.06)) ;
#141316=CARTESIAN_POINT('Origin',(-2.75,10.75,-11.06)) ;
#141317=CARTESIAN_POINT('Origin',(-2.75,10.75,-9.26)) ;
#141318=CARTESIAN_POINT('Origin',(-2.75,10.75,-9.26)) ;
#141319=CARTESIAN_POINT('Origin',(-2.75,10.75,-11.06)) ;
#141320=CARTESIAN_POINT('Origin',(-2.75,10.75,-11.06)) ;
#141321=CARTESIAN_POINT('Origin',(-2.75,10.75,-10.16)) ;
#141322=CARTESIAN_POINT('Origin',(4.6,0.,-10.16)) ;
#141323=CARTESIAN_POINT('Ctrl Pts',(4.5,-2.7,-8.63684537882721)) ;
#141324=CARTESIAN_POINT('Ctrl Pts',(4.5,-2.71827986285823,-8.71196473917507)) ;
#141325=CARTESIAN_POINT('Ctrl Pts',(4.50597963419107,-2.73556801027185,
-8.78673986045281)) ;
#141326=CARTESIAN_POINT('Ctrl Pts',(4.52394923367545,-2.75977758633329,
-8.89843683402156)) ;
#141327=CARTESIAN_POINT('Ctrl Pts',(4.53141024883993,-2.76757607569523,
-8.93568328239029)) ;
#141328=CARTESIAN_POINT('Ctrl Pts',(4.54734065524867,-2.77857284247615,
-8.99016568958296)) ;
#141329=CARTESIAN_POINT('Ctrl Pts',(4.55339248498575,-2.78214991573955,
-9.00823827441494)) ;
#141330=CARTESIAN_POINT('Ctrl Pts',(4.56567492147096,-2.787183259287,-9.03414672186072)) ;
#141331=CARTESIAN_POINT('Ctrl Pts',(4.5702469143305,-2.78880341224557,-9.04257260505081)) ;
#141332=CARTESIAN_POINT('Ctrl Pts',(4.58215938980081,-2.79169669265294,
-9.0577434798851)) ;
#141333=CARTESIAN_POINT('Ctrl Pts',(4.59005470866978,-2.79310344827587,
-9.06520635404226)) ;
#141334=CARTESIAN_POINT('Ctrl Pts',(4.6,-2.79310344827586,-9.06520635404224)) ;
#141335=CARTESIAN_POINT('Origin',(4.6,-2.4,-8.19785831296514)) ;
#141336=CARTESIAN_POINT('Origin',(4.6,-2.4,-7.62)) ;
#141337=CARTESIAN_POINT('Origin',(4.6,-2.4,-8.19785831296514)) ;
#141338=CARTESIAN_POINT('Origin',(4.6,-2.4,-8.19785831296514)) ;
#141339=CARTESIAN_POINT('Origin',(4.6,-2.4,-8.19785831296514)) ;
#141340=CARTESIAN_POINT('Origin',(0.584645609909622,-2.4,-8.19785831296514)) ;
#141341=CARTESIAN_POINT('Origin',(12.7,-2.4,-8.19785831296514)) ;
#141342=CARTESIAN_POINT('Origin',(12.7,-2.2,-7.62)) ;
#141343=CARTESIAN_POINT('Origin',(12.7,-2.2,-8.19785831296514)) ;
#141344=CARTESIAN_POINT('Origin',(12.7,-2.4,-8.19785831296514)) ;
#141345=CARTESIAN_POINT('Origin',(12.7,-2.24516129032258,-8.32444809922546)) ;
#141346=CARTESIAN_POINT('Origin',(12.7,0.,-10.16)) ;
#141347=CARTESIAN_POINT('Origin',(12.7,-2.24516129032258,-11.9955519007745)) ;
#141348=CARTESIAN_POINT('Origin',(12.7,-2.2,-7.62)) ;
#141349=CARTESIAN_POINT('Origin',(12.7,-2.2,-12.1221416870349)) ;
#141350=CARTESIAN_POINT('Origin',(12.7,-2.4,-12.1221416870349)) ;
#141351=CARTESIAN_POINT('Origin',(12.7,-2.4,-12.1221416870349)) ;
#141352=CARTESIAN_POINT('Origin',(0.584645609909622,-2.4,-12.1221416870349)) ;
#141353=CARTESIAN_POINT('Origin',(4.6,-2.4,-12.1221416870349)) ;
#141354=CARTESIAN_POINT('Origin',(4.6,-2.4,-7.62)) ;
#141355=CARTESIAN_POINT('Origin',(4.6,-2.4,-12.1221416870349)) ;
#141356=CARTESIAN_POINT('Origin',(4.6,-2.4,-12.1221416870349)) ;
#141357=CARTESIAN_POINT('Origin',(4.6,-2.4,-12.1221416870349)) ;
#141358=CARTESIAN_POINT('Origin',(4.6,0.,-10.16)) ;
#141359=CARTESIAN_POINT('Ctrl Pts',(4.6,-2.79310344827586,-11.2547936459578)) ;
#141360=CARTESIAN_POINT('Ctrl Pts',(4.59007568892311,-2.79310344827586,
-11.2547936459578)) ;
#141361=CARTESIAN_POINT('Ctrl Pts',(4.58219207637239,-2.79170232102182,
-11.262226742276)) ;
#141362=CARTESIAN_POINT('Ctrl Pts',(4.57028631514659,-2.78881527838255,
-11.27736543899)) ;
#141363=CARTESIAN_POINT('Ctrl Pts',(4.56571532154372,-2.78719767797524,
-11.2857784885835)) ;
#141364=CARTESIAN_POINT('Ctrl Pts',(4.55343865632726,-2.78217307830036,
-11.3116436333089)) ;
#141365=CARTESIAN_POINT('Ctrl Pts',(4.54738888873343,-2.77860151743012,
-11.3296900859661)) ;
#141366=CARTESIAN_POINT('Ctrl Pts',(4.53146440752601,-2.76762263748299,
-11.3840903156831)) ;
#141367=CARTESIAN_POINT('Ctrl Pts',(4.52400917967609,-2.75984503873828,
-11.4212455063058)) ;
#141368=CARTESIAN_POINT('Ctrl Pts',(4.50599905604505,-2.7356206423885,-11.5330301354693)) ;
#141369=CARTESIAN_POINT('Ctrl Pts',(4.5,-2.71826422026483,-11.6080995425769)) ;
#141370=CARTESIAN_POINT('Ctrl Pts',(4.5,-2.7,-11.6831546211728)) ;
#141371=CARTESIAN_POINT('Origin',(3.7,-2.9,-7.62)) ;
#141372=CARTESIAN_POINT('Origin',(3.5,-3.95,-7.62)) ;
#141373=CARTESIAN_POINT('Origin',(-5.3,-3.95,-7.62)) ;
#141374=CARTESIAN_POINT('Origin',(-5.3,5.19009804864072,-7.62)) ;
#141375=CARTESIAN_POINT('Origin',(-4.8,10.3,-7.62)) ;
#141376=CARTESIAN_POINT('Origin',(-4.8,10.85,-7.62)) ;
#141377=CARTESIAN_POINT('Origin',(-0.362523114814661,9.05,-10.3290473046963)) ;
#141378=CARTESIAN_POINT('Origin',(0.36252311481466,9.05,-9.99095269530372)) ;
#141379=CARTESIAN_POINT('Origin',(-1.31845674202095,9.85,-8.75228134223507)) ;
#141380=CARTESIAN_POINT('Origin',(-0.230887397576972,9.85,-8.24513942814623)) ;
#141381=CARTESIAN_POINT('Origin',(3.3,10.85,-7.62)) ;
#141382=CARTESIAN_POINT('Origin',(3.3,10.05,-7.62)) ;
#141383=CARTESIAN_POINT('Origin',(3.,9.85,-7.62)) ;
#141384=CARTESIAN_POINT('Origin',(3.,8.05,-7.62)) ;
#141385=CARTESIAN_POINT('Origin',(3.34087287789487,7.85,-7.62)) ;
#141386=CARTESIAN_POINT('Origin',(3.85,6.92431432344521,-7.62)) ;
#141387=CARTESIAN_POINT('Origin',(4.05,3.77568567655479,-7.62)) ;
#141388=CARTESIAN_POINT('Origin',(4.6,2.1,-8.77804604217164)) ;
#141389=CARTESIAN_POINT('Origin',(4.6,2.1,-8.77804604217164)) ;
#141390=CARTESIAN_POINT('Origin',(4.6,0.280857398566761,-8.47485560859943)) ;
#141391=CARTESIAN_POINT('Origin',(4.6,2.61712020253893,-8.86423274259479)) ;
#141392=CARTESIAN_POINT('Origin',(4.6,2.65,-8.66695395782836)) ;
#141393=CARTESIAN_POINT('Origin',(4.6,2.72431432344521,-8.85263481664499)) ;
#141394=CARTESIAN_POINT('Ctrl Pts',(4.48762159086906,2.77250619842445,-8.77117568174961)) ;
#141395=CARTESIAN_POINT('Ctrl Pts',(4.51316716229104,2.72605970493114,-8.73423879419717)) ;
#141396=CARTESIAN_POINT('Ctrl Pts',(4.5752745340585,2.73535372386122,-8.71905715319801)) ;
#141397=CARTESIAN_POINT('Ctrl Pts',(4.49363662433154,2.76156977394749,-8.80699959247167)) ;
#141398=CARTESIAN_POINT('Ctrl Pts',(4.5146945995807,2.70766535161862,-8.75620084739328)) ;
#141399=CARTESIAN_POINT('Ctrl Pts',(4.58732693581886,2.72440392220679,-8.73699504123404)) ;
#141400=CARTESIAN_POINT('Ctrl Pts',(4.5,2.7448843843803,-8.8361692160662)) ;
#141401=CARTESIAN_POINT('Ctrl Pts',(4.50856472873623,2.69031482079683,-8.75849111370477)) ;
#141402=CARTESIAN_POINT('Ctrl Pts',(4.60003980620505,2.7077507326983,-8.75155231137473)) ;
#141403=CARTESIAN_POINT('Ctrl Pts',(4.5,2.72431432344521,-8.85263481664499)) ;
#141404=CARTESIAN_POINT('Ctrl Pts',(4.5,2.68714136424468,-8.75975491585172)) ;
#141405=CARTESIAN_POINT('Ctrl Pts',(4.60004250625996,2.68715716507935,-8.7597943956238)) ;
#141406=CARTESIAN_POINT('Origin',(4.57524318173443,2.82069807340128,-8.77117568174948)) ;
#141407=CARTESIAN_POINT('Ctrl Pts',(4.47150553123747,2.80180812502279,-8.66695395782836)) ;
#141408=CARTESIAN_POINT('Ctrl Pts',(4.5,2.75,-8.66695395782836)) ;
#141409=CARTESIAN_POINT('Ctrl Pts',(4.55912712210514,2.75,-8.66695395782836)) ;
#141410=CARTESIAN_POINT('Ctrl Pts',(4.47150553186688,2.8018081238784,-8.7035744727347)) ;
#141411=CARTESIAN_POINT('Ctrl Pts',(4.50000000073523,2.74999999866316,-8.69125808426882)) ;
#141412=CARTESIAN_POINT('Ctrl Pts',(4.5591271227348,2.75,-8.68527204575931)) ;
#141413=CARTESIAN_POINT('Ctrl Pts',(4.4771244897161,2.79159183687982,-8.73991653735229)) ;
#141414=CARTESIAN_POINT('Ctrl Pts',(4.50480340096853,2.74126654369358,-8.71553795099799)) ;
#141415=CARTESIAN_POINT('Ctrl Pts',(4.56473907811163,2.74489822224647,-8.70342482158223)) ;
#141416=CARTESIAN_POINT('Ctrl Pts',(4.48762159086676,2.77250619842407,-8.77117568174948)) ;
#141417=CARTESIAN_POINT('Ctrl Pts',(4.51315802400618,2.72607631998876,-8.7342520074343)) ;
#141418=CARTESIAN_POINT('Ctrl Pts',(4.57524318173443,2.73534903670064,-8.71906481978892)) ;
#141419=CARTESIAN_POINT('Origin',(4.55912712210513,2.85,-8.66695395782836)) ;
#141420=CARTESIAN_POINT('Origin',(4.55912712210514,2.85,-7.62)) ;
#141421=CARTESIAN_POINT('Origin',(4.55912712210514,2.85,-7.62)) ;
#141422=CARTESIAN_POINT('Origin',(4.55912712210514,2.85,-11.6530460421716)) ;
#141423=CARTESIAN_POINT('Ctrl Pts',(4.48762159086767,2.77250619842243,-11.5488243182478)) ;
#141424=CARTESIAN_POINT('Ctrl Pts',(4.51315802400691,2.72607631998743,-11.5857479925641)) ;
#141425=CARTESIAN_POINT('Ctrl Pts',(4.57524318173533,2.73534903669982,-11.6009351802097)) ;
#141426=CARTESIAN_POINT('Ctrl Pts',(4.47712448971642,2.79159183687924,-11.5800834626456)) ;
#141427=CARTESIAN_POINT('Ctrl Pts',(4.50480340096883,2.7412665436931,-11.6044620490005)) ;
#141428=CARTESIAN_POINT('Ctrl Pts',(4.56473907811193,2.74489822224616,-11.6165751784167)) ;
#141429=CARTESIAN_POINT('Ctrl Pts',(4.47150553186688,2.8018081238784,-11.6164255272643)) ;
#141430=CARTESIAN_POINT('Ctrl Pts',(4.50000000073523,2.74999999866316,-11.6287419157305)) ;
#141431=CARTESIAN_POINT('Ctrl Pts',(4.5591271227348,2.75,-11.6347279542402)) ;
#141432=CARTESIAN_POINT('Ctrl Pts',(4.47150553123747,2.80180812502279,-11.6530460421716)) ;
#141433=CARTESIAN_POINT('Ctrl Pts',(4.5,2.75,-11.6530460421716)) ;
#141434=CARTESIAN_POINT('Ctrl Pts',(4.55912712210513,2.75,-11.6530460421716)) ;
#141435=CARTESIAN_POINT('Origin',(4.57524318173533,2.82069807339964,-11.5488243182478)) ;
#141436=CARTESIAN_POINT('Ctrl Pts',(4.57527448145475,2.73535371598842,-11.6009428339419)) ;
#141437=CARTESIAN_POINT('Ctrl Pts',(4.51316714695681,2.72605973281053,-11.5857611836291)) ;
#141438=CARTESIAN_POINT('Ctrl Pts',(4.48762159086951,2.77250619842363,-11.5488243182477)) ;
#141439=CARTESIAN_POINT('Ctrl Pts',(4.58732687742636,2.72440390874893,-11.5830049433246)) ;
#141440=CARTESIAN_POINT('Ctrl Pts',(4.51469458626359,2.70766538570633,-11.5637991204816)) ;
#141441=CARTESIAN_POINT('Ctrl Pts',(4.49363662433188,2.76156977394663,-11.5130004075268)) ;
#141442=CARTESIAN_POINT('Ctrl Pts',(4.60003973844303,2.70775071978178,-11.568447683485)) ;
#141443=CARTESIAN_POINT('Ctrl Pts',(4.50856472285792,2.69031485824814,-11.5615088329844)) ;
#141444=CARTESIAN_POINT('Ctrl Pts',(4.5,2.74488438437974,-11.4838307839335)) ;
#141445=CARTESIAN_POINT('Ctrl Pts',(4.60004243494346,2.6871571650681,-11.5602056044043)) ;
#141446=CARTESIAN_POINT('Ctrl Pts',(4.5,2.68714139075513,-11.5602450179096)) ;
#141447=CARTESIAN_POINT('Ctrl Pts',(4.5,2.72431432344521,-11.467365183355)) ;
#141448=CARTESIAN_POINT('Origin',(4.6,0.280857398566761,-11.8451443914006)) ;
#141449=CARTESIAN_POINT('Origin',(4.6,2.1,-11.5419539578284)) ;
#141450=CARTESIAN_POINT('Origin',(4.6,2.1,-11.5419539578284)) ;
#141451=CARTESIAN_POINT('Origin',(4.6,0.,-10.16)) ;
#141452=CARTESIAN_POINT('',(4.5,-2.9,-10.1600000000039)) ;
#141453=CARTESIAN_POINT('',(4.57439618084313,-2.80937499999937,-11.2027958671254)) ;
#141454=CARTESIAN_POINT('Ctrl Pts',(4.5,-2.9,-10.1600000000039)) ;
#141455=CARTESIAN_POINT('Ctrl Pts',(4.5,-2.9000000234111,-10.3361762625703)) ;
#141456=CARTESIAN_POINT('Ctrl Pts',(4.49893459747296,-2.89187728142186,
-10.5122938225552)) ;
#141457=CARTESIAN_POINT('Ctrl Pts',(4.50498172725087,-2.86839426105774,
-10.7749432768872)) ;
#141458=CARTESIAN_POINT('Ctrl Pts',(4.50826226558342,-2.85869729223562,
-10.8622870271135)) ;
#141459=CARTESIAN_POINT('Ctrl Pts',(4.52028413974051,-2.84160518746962,
-10.9928409654328)) ;
#141460=CARTESIAN_POINT('Ctrl Pts',(4.52545003690602,-2.8354696349403,-11.036363113622)) ;
#141461=CARTESIAN_POINT('Ctrl Pts',(4.53741870680498,-2.82581179679252,
-11.1006394550108)) ;
#141462=CARTESIAN_POINT('Ctrl Pts',(4.54209540184575,-2.82251395224859,
-11.1219200182606)) ;
#141463=CARTESIAN_POINT('Ctrl Pts',(4.55451190949429,-2.81582803324483,
-11.1638742105328)) ;
#141464=CARTESIAN_POINT('Ctrl Pts',(4.56139306411848,-2.8124020390272,-11.1847435318249)) ;
#141465=CARTESIAN_POINT('Ctrl Pts',(4.57439618084313,-2.80937499999937,
-11.2027958671254)) ;
#141466=CARTESIAN_POINT('Ctrl Pts',(4.57439618084312,-2.80937499999939,
-11.2027958671254)) ;
#141467=CARTESIAN_POINT('Ctrl Pts',(4.57788811720513,-2.80856205104937,
-11.2076438845913)) ;
#141468=CARTESIAN_POINT('Ctrl Pts',(4.58132110715668,-2.80743849592502,
-11.2126543114198)) ;
#141469=CARTESIAN_POINT('Ctrl Pts',(4.58591063786564,-2.80541025280312,
-11.2200683491599)) ;
#141470=CARTESIAN_POINT('Ctrl Pts',(4.58721694730502,-2.80476695238159,
-11.2222683250838)) ;
#141471=CARTESIAN_POINT('Ctrl Pts',(4.5887449802686,-2.80393035430396,-11.2249717146408)) ;
#141472=CARTESIAN_POINT('Ctrl Pts',(4.58900094431508,-2.80378708879839,
-11.225429423373)) ;
#141473=CARTESIAN_POINT('Ctrl Pts',(4.58924476828968,-2.80364801935069,
-11.22586949326)) ;
#141474=CARTESIAN_POINT('Ctrl Pts',(4.58924931741448,-2.80364542371033,
-11.2258777053493)) ;
#141475=CARTESIAN_POINT('Ctrl Pts',(4.59158188358133,-2.80231401319274,
-11.2300892401221)) ;
#141476=CARTESIAN_POINT('Ctrl Pts',(4.59377134212491,-2.800813098491,-11.2344383923963)) ;
#141477=CARTESIAN_POINT('Ctrl Pts',(4.59570408210449,-2.79909049146272,
-11.2391378632085)) ;
#141478=CARTESIAN_POINT('Ctrl Pts',(4.5957084873849,-2.79908656285628,-11.2391485795778)) ;
#141479=CARTESIAN_POINT('Ctrl Pts',(4.59603576097762,-2.79879453264352,
-11.2399450754361)) ;
#141480=CARTESIAN_POINT('Ctrl Pts',(4.59633794834607,-2.79851279959495,
-11.2407065253189)) ;
#141481=CARTESIAN_POINT('Ctrl Pts',(4.59727216584803,-2.79759800070515,
-11.24316063341)) ;
#141482=CARTESIAN_POINT('Ctrl Pts',(4.59785661125443,-2.79695684051616,
-11.2448529156094)) ;
#141483=CARTESIAN_POINT('Ctrl Pts',(4.59875882816121,-2.79580092267551,
-11.2478683242216)) ;
#141484=CARTESIAN_POINT('Ctrl Pts',(4.59910960512328,-2.79529211440566,
-11.2491844992175)) ;
#141485=CARTESIAN_POINT('Ctrl Pts',(4.59950074890552,-2.79458032370894,
-11.2510150784121)) ;
#141486=CARTESIAN_POINT('Ctrl Pts',(4.59959271145697,-2.79439474074567,
-11.2514948405808)) ;
#141487=CARTESIAN_POINT('Ctrl Pts',(4.59970479219924,-2.79411978912794,
-11.2522025710462)) ;
#141488=CARTESIAN_POINT('Ctrl Pts',(4.59973686334512,-2.79403231884248,
-11.2524272684452)) ;
#141489=CARTESIAN_POINT('Ctrl Pts',(4.59980956306602,-2.7938042827674,-11.2530108264021)) ;
#141490=CARTESIAN_POINT('Ctrl Pts',(4.59984405921136,-2.79366555090847,
-11.2533689790042)) ;
#141491=CARTESIAN_POINT('Ctrl Pts',(4.59992170638737,-2.79338632637294,
-11.2540824135446)) ;
#141492=CARTESIAN_POINT('Ctrl Pts',(4.59995882625635,-2.79324305250058,
-11.2544374792565)) ;
#141493=CARTESIAN_POINT('Ctrl Pts',(4.59999999999999,-2.79310344827586,
-11.2547936459578)) ;
#141494=CARTESIAN_POINT('',(4.57439618084271,-2.80937499999947,-9.11720413287514)) ;
#141495=CARTESIAN_POINT('Ctrl Pts',(4.59999999999999,-2.79310344827586,
-9.06520635404223)) ;
#141496=CARTESIAN_POINT('Ctrl Pts',(4.59995895305209,-2.79324111387631,
-9.06556200704419)) ;
#141497=CARTESIAN_POINT('Ctrl Pts',(4.59992125133673,-2.79338175512528,
-9.06591664999517)) ;
#141498=CARTESIAN_POINT('Ctrl Pts',(4.59984242179761,-2.79365985893298,
-9.06662721825472)) ;
#141499=CARTESIAN_POINT('Ctrl Pts',(4.5998070294299,-2.79379858543765,-9.06698190400296)) ;
#141500=CARTESIAN_POINT('Ctrl Pts',(4.59973261548694,-2.79401893257626,
-9.06754582127962)) ;
#141501=CARTESIAN_POINT('Ctrl Pts',(4.59970092564442,-2.79410050108421,
-9.06775470445263)) ;
#141502=CARTESIAN_POINT('Ctrl Pts',(4.59958060815602,-2.79437456977472,
-9.06845707425772)) ;
#141503=CARTESIAN_POINT('Ctrl Pts',(4.59947821517875,-2.79456857658396,
-9.06895509538074)) ;
#141504=CARTESIAN_POINT('Ctrl Pts',(4.59905971984789,-2.79527981802027,
-9.07078506438848)) ;
#141505=CARTESIAN_POINT('Ctrl Pts',(4.59869396429224,-2.79579226918927,
-9.07211140120008)) ;
#141506=CARTESIAN_POINT('Ctrl Pts',(4.59768320083748,-2.79706868650734,
-9.07544407389332)) ;
#141507=CARTESIAN_POINT('Ctrl Pts',(4.59698254015872,-2.79783590182172,
-9.07747319966266)) ;
#141508=CARTESIAN_POINT('Ctrl Pts',(4.5959970522588,-2.79876532988112,-9.07998468423845)) ;
#141509=CARTESIAN_POINT('Ctrl Pts',(4.59580678362761,-2.79893964110239,
-9.08045810500392)) ;
#141510=CARTESIAN_POINT('Ctrl Pts',(4.59367882781298,-2.80083904916685,
-9.0856449119971)) ;
#141511=CARTESIAN_POINT('Ctrl Pts',(4.5915070708769,-2.80233337893514,-9.08997932770411)) ;
#141512=CARTESIAN_POINT('Ctrl Pts',(4.58628071719239,-2.80532570224269,
-9.09945146742918)) ;
#141513=CARTESIAN_POINT('Ctrl Pts',(4.58313959595716,-2.80673110767406,
-9.10451024806567)) ;
#141514=CARTESIAN_POINT('Ctrl Pts',(4.5780261114634,-2.80844040952813,-9.11209635749167)) ;
#141515=CARTESIAN_POINT('Ctrl Pts',(4.57624387811649,-2.80894486836995,
-9.11463895934166)) ;
#141516=CARTESIAN_POINT('Ctrl Pts',(4.57439618084271,-2.80937499999947,
-9.11720413287514)) ;
#141517=CARTESIAN_POINT('Ctrl Pts',(4.57439618084271,-2.80937499999947,
-9.11720413287514)) ;
#141518=CARTESIAN_POINT('Ctrl Pts',(4.56149777794589,-2.81237766235468,
-9.1351110931668)) ;
#141519=CARTESIAN_POINT('Ctrl Pts',(4.55451596106519,-2.81582788236477,
-9.15612624229681)) ;
#141520=CARTESIAN_POINT('Ctrl Pts',(4.54213610452188,-2.82249001163036,
-9.19792835962828)) ;
#141521=CARTESIAN_POINT('Ctrl Pts',(4.53742891479326,-2.82580422498964,
-9.219310967236)) ;
#141522=CARTESIAN_POINT('Ctrl Pts',(4.525451614243,-2.8354670333868,-9.28361794379489)) ;
#141523=CARTESIAN_POINT('Ctrl Pts',(4.52032009146395,-2.84156292603926,
-9.32685657347848)) ;
#141524=CARTESIAN_POINT('Ctrl Pts',(4.50830110904356,-2.85862448221642,
-9.45711642595738)) ;
#141525=CARTESIAN_POINT('Ctrl Pts',(4.50499166750953,-2.86836219567853,
-9.5447300385823)) ;
#141526=CARTESIAN_POINT('Ctrl Pts',(4.49892845988062,-2.8918880660271,-9.80776299683786)) ;
#141527=CARTESIAN_POINT('Ctrl Pts',(4.49999999999474,-2.89999999999869,
-9.98383009011777)) ;
#141528=CARTESIAN_POINT('Ctrl Pts',(4.5,-2.9,-10.1600000000039)) ;
#141529=CARTESIAN_POINT('Origin',(4.4,-2.7,-7.62)) ;
#141530=CARTESIAN_POINT('Origin',(4.4,-2.7,-8.63684537882721)) ;
#141531=CARTESIAN_POINT('Ctrl Pts',(4.40227435089074,-2.79999990867355,
-8.56940069288188)) ;
#141532=CARTESIAN_POINT('Ctrl Pts',(4.51828879250235,-2.80015667527379,
-8.57878556679247)) ;
#141533=CARTESIAN_POINT('Ctrl Pts',(4.50118227077259,-2.68533700727769,
-8.57797110744942)) ;
#141534=CARTESIAN_POINT('Ctrl Pts',(4.39419482113926,-2.79999992837382,
-8.68368769966915)) ;
#141535=CARTESIAN_POINT('Ctrl Pts',(4.4857179250172,-2.80010751836584,-8.66267136675065)) ;
#141536=CARTESIAN_POINT('Ctrl Pts',(4.49717570077253,-2.71006921719245,
-8.67703189821457)) ;
#141537=CARTESIAN_POINT('Ctrl Pts',(4.40636790575269,-2.79999994706265,
-8.79490890735427)) ;
#141538=CARTESIAN_POINT('Ctrl Pts',(4.47481046024548,-2.80007242131914,
-8.77332242779906)) ;
#141539=CARTESIAN_POINT('Ctrl Pts',(4.50328131876401,-2.73353293829092,
-8.77702587481)) ;
#141540=CARTESIAN_POINT('Ctrl Pts',(4.4547973699423,-2.79999997092221,-8.94507366547111)) ;
#141541=CARTESIAN_POINT('Ctrl Pts',(4.49869786247047,-2.80003603117402,
-8.92627924349578)) ;
#141542=CARTESIAN_POINT('Ctrl Pts',(4.52748687875415,-2.76348976047508,
-8.91628917285872)) ;
#141543=CARTESIAN_POINT('Ctrl Pts',(4.47221929614096,-2.79999997745988,
-8.98730406022326)) ;
#141544=CARTESIAN_POINT('Ctrl Pts',(4.5088055676762,-2.80002725736479,-8.9682748482859)) ;
#141545=CARTESIAN_POINT('Ctrl Pts',(4.53619137795529,-2.77169834185702,
-8.95598368236755)) ;
#141546=CARTESIAN_POINT('Ctrl Pts',(4.50882352800136,-2.79999998605361,
-9.04428434960906)) ;
#141547=CARTESIAN_POINT('Ctrl Pts',(4.5336780291127,-2.80001636071784,-9.02535870242034)) ;
#141548=CARTESIAN_POINT('Ctrl Pts',(4.55447319025663,-2.78248861123826,
-9.01009568142552)) ;
#141549=CARTESIAN_POINT('Ctrl Pts',(4.52308919141484,-2.79999998878206,
-9.06266256169107)) ;
#141550=CARTESIAN_POINT('Ctrl Pts',(4.54363962638622,-2.80001303821803,
-9.04372615017166)) ;
#141551=CARTESIAN_POINT('Ctrl Pts',(4.56159739427507,-2.78591449131413,
-9.0276542708947)) ;
#141552=CARTESIAN_POINT('Ctrl Pts',(4.57467506176493,-2.79999999510246,
-9.10569650839936)) ;
#141553=CARTESIAN_POINT('Ctrl Pts',(4.5806240530329,-2.80000557393877,-9.08633416327778)) ;
#141554=CARTESIAN_POINT('Ctrl Pts',(4.58735613403293,-2.79385049254303,
-9.06891981499325)) ;
#141555=CARTESIAN_POINT('Ctrl Pts',(4.62437069655637,-2.79999999703807,
-9.11953134306007)) ;
#141556=CARTESIAN_POINT('Ctrl Pts',(4.61827372661886,-2.80000334969057,
-9.10093404548759)) ;
#141557=CARTESIAN_POINT('Ctrl Pts',(4.61212682540743,-2.79628090446621,
-9.08240281421819)) ;
#141558=CARTESIAN_POINT('Ctrl Pts',(4.67161368302031,-2.79999998860619,
-9.06078982676527)) ;
#141559=CARTESIAN_POINT('Ctrl Pts',(4.65407010102641,-2.80001325705921,
-9.04046373958886)) ;
#141560=CARTESIAN_POINT('Ctrl Pts',(4.63587130780614,-2.78569367459188,
-9.02562812959412)) ;
#141561=CARTESIAN_POINT('Ctrl Pts',(4.54879236204369,-2.8,-9.0835655563675)) ;
#141562=CARTESIAN_POINT('Ctrl Pts',(4.55448837802391,-2.7999999999815,-9.08117882091364)) ;
#141563=CARTESIAN_POINT('Ctrl Pts',(4.56021842726602,-2.7995915078324,-9.07883954273416)) ;
#141564=CARTESIAN_POINT('Ctrl Pts',(4.5673067198498,-2.79865167182176,-9.07597888386358)) ;
#141565=CARTESIAN_POINT('Ctrl Pts',(4.56847770958267,-2.79848295770258,
-9.07550732683475)) ;
#141566=CARTESIAN_POINT('Ctrl Pts',(4.5710752309902,-2.79808046368153,-9.07446296289698)) ;
#141567=CARTESIAN_POINT('Ctrl Pts',(4.57250093612479,-2.79784058543152,
-9.07388964302801)) ;
#141568=CARTESIAN_POINT('Ctrl Pts',(4.5764383594612,-2.79713266293194,-9.07231368646489)) ;
#141569=CARTESIAN_POINT('Ctrl Pts',(4.57879956048961,-2.79666132938902,
-9.07137580039694)) ;
#141570=CARTESIAN_POINT('Ctrl Pts',(4.58293855712952,-2.79579586318667,
-9.06976081592962)) ;
#141571=CARTESIAN_POINT('Ctrl Pts',(4.58471363403686,-2.79540911153441,
-9.06907461719118)) ;
#141572=CARTESIAN_POINT('Ctrl Pts',(4.58699082729421,-2.7949269768198,-9.06824452926202)) ;
#141573=CARTESIAN_POINT('Ctrl Pts',(4.58739952300691,-2.79484234870239,
-9.0681019268464)) ;
#141574=CARTESIAN_POINT('Ctrl Pts',(4.58871515235473,-2.79457617288697,
-9.06766112910089)) ;
#141575=CARTESIAN_POINT('Ctrl Pts',(4.58961690596117,-2.79440247805564,
-9.06738498699956)) ;
#141576=CARTESIAN_POINT('Ctrl Pts',(4.59105375065842,-2.79414748185769,
-9.06698298181798)) ;
#141577=CARTESIAN_POINT('Ctrl Pts',(4.59155303909535,-2.79406229662444,
-9.06684924350716)) ;
#141578=CARTESIAN_POINT('Ctrl Pts',(4.59245965385672,-2.79391282221553,
-9.06661259411486)) ;
#141579=CARTESIAN_POINT('Ctrl Pts',(4.59286388425107,-2.79384761399903,
-9.06650842178453)) ;
#141580=CARTESIAN_POINT('Ctrl Pts',(4.59368973959986,-2.7937059861537,-9.06626767265164)) ;
#141581=CARTESIAN_POINT('Ctrl Pts',(4.59407665941131,-2.7936397371459,-9.06615152123315)) ;
#141582=CARTESIAN_POINT('Ctrl Pts',(4.59444371287738,-2.79357284110654,
-9.06602679272787)) ;
#141583=CARTESIAN_POINT('Ctrl Pts',(4.59448890259162,-2.79356452972316,
-9.0660111581995)) ;
#141584=CARTESIAN_POINT('Ctrl Pts',(4.59470842334911,-2.79352377141065,
-9.06593382545217)) ;
#141585=CARTESIAN_POINT('Ctrl Pts',(4.5948359873327,-2.79349361011836,-9.0658723314841)) ;
#141586=CARTESIAN_POINT('Ctrl Pts',(4.59514620525224,-2.7934297131363,-9.0657459400492)) ;
#141587=CARTESIAN_POINT('Ctrl Pts',(4.59533334275102,-2.79339696908416,
-9.06568383785339)) ;
#141588=CARTESIAN_POINT('Ctrl Pts',(4.59563785533348,-2.79335634095568,
-9.06561299034027)) ;
#141589=CARTESIAN_POINT('Ctrl Pts',(4.59571710962763,-2.79334654412181,
-9.06559639128765)) ;
#141590=CARTESIAN_POINT('Ctrl Pts',(4.59594411915586,-2.79332043135007,
-9.0655533496182)) ;
#141591=CARTESIAN_POINT('Ctrl Pts',(4.59600288191152,-2.79330503361987,
-9.06553395124079)) ;
#141592=CARTESIAN_POINT('Ctrl Pts',(4.59613307952173,-2.79327450473786,
-9.06549928051942)) ;
#141593=CARTESIAN_POINT('Ctrl Pts',(4.59620389659311,-2.79325970788819,
-9.06548500605856)) ;
#141594=CARTESIAN_POINT('Ctrl Pts',(4.5965119298477,-2.79322709231927,-9.06545027786287)) ;
#141595=CARTESIAN_POINT('Ctrl Pts',(4.59679543741295,-2.79320989448354,
-9.06542934418242)) ;
#141596=CARTESIAN_POINT('Ctrl Pts',(4.59784475938522,-2.793166495242,-9.0653578835066)) ;
#141597=CARTESIAN_POINT('Ctrl Pts',(4.59874915064779,-2.79313948637392,
-9.06529926431075)) ;
#141598=CARTESIAN_POINT('Ctrl Pts',(4.59999999999999,-2.79310344827586,
-9.06520635404224)) ;
#141599=CARTESIAN_POINT('Origin',(4.4,-2.7,-7.62)) ;
#141600=CARTESIAN_POINT('Origin',(4.4,-2.7,-11.6831546211728)) ;
#141601=CARTESIAN_POINT('Ctrl Pts',(4.5011795914298,-2.68531903459926,-11.7420290201723)) ;
#141602=CARTESIAN_POINT('Ctrl Pts',(4.51828670358939,-2.8,-11.7412138251405)) ;
#141603=CARTESIAN_POINT('Ctrl Pts',(4.40240952225579,-2.8,-11.7505883721107)) ;
#141604=CARTESIAN_POINT('Ctrl Pts',(4.49717774927193,-2.71005310920069,
-11.6429655323627)) ;
#141605=CARTESIAN_POINT('Ctrl Pts',(4.48574628541092,-2.8,-11.6573148520406)) ;
#141606=CARTESIAN_POINT('Ctrl Pts',(4.39431668173581,-2.8,-11.6363402695085)) ;
#141607=CARTESIAN_POINT('Ctrl Pts',(4.50328690685192,-2.73351987602563,
-11.5429733978619)) ;
#141608=CARTESIAN_POINT('Ctrl Pts',(4.47485145549543,-2.8,-11.5466766957412)) ;
#141609=CARTESIAN_POINT('Ctrl Pts',(4.40646789472119,-2.8,-11.5251226186383)) ;
#141610=CARTESIAN_POINT('Ctrl Pts',(4.52749311797091,-2.76348183928881,
-11.4037129921595)) ;
#141611=CARTESIAN_POINT('Ctrl Pts',(4.49873206155795,-2.8,-11.3937330953071)) ;
#141612=CARTESIAN_POINT('Ctrl Pts',(4.45486817043772,-2.8,-11.3749566433661)) ;
#141613=CARTESIAN_POINT('Ctrl Pts',(4.53619745972499,-2.77169205010106,
-11.3640190471852)) ;
#141614=CARTESIAN_POINT('Ctrl Pts',(4.50883664816671,-2.8,-11.3517394381721)) ;
#141615=CARTESIAN_POINT('Ctrl Pts',(4.47227975612147,-2.8,-11.3327273846037)) ;
#141616=CARTESIAN_POINT('Ctrl Pts',(4.55447795090009,-2.78248459830339,
-11.3099078127334)) ;
#141617=CARTESIAN_POINT('Ctrl Pts',(4.53370055749885,-2.8,-11.2946579183699)) ;
#141618=CARTESIAN_POINT('Ctrl Pts',(4.50886586566854,-2.8,-11.2757478882722)) ;
#141619=CARTESIAN_POINT('Ctrl Pts',(4.56160154376425,-2.78591123334062,
-11.2923494428157)) ;
#141620=CARTESIAN_POINT('Ctrl Pts',(4.54365878772218,-2.8,-11.2762910664542)) ;
#141621=CARTESIAN_POINT('Ctrl Pts',(4.52312452397684,-2.8,-11.2573699954867)) ;
#141622=CARTESIAN_POINT('Ctrl Pts',(4.58735772267363,-2.79384903998488,
-11.2510842943985)) ;
#141623=CARTESIAN_POINT('Ctrl Pts',(4.58063087367387,-2.79999999999999,
-11.2336839633809)) ;
#141624=CARTESIAN_POINT('Ctrl Pts',(4.57468550767192,-2.8,-11.2143374866056)) ;
#141625=CARTESIAN_POINT('Ctrl Pts',(4.61212536563478,-2.79628002040289,
-11.2376015865952)) ;
#141626=CARTESIAN_POINT('Ctrl Pts',(4.61826745782989,-2.79999999999994,
-11.2190848793758)) ;
#141627=CARTESIAN_POINT('Ctrl Pts',(4.62435992349563,-2.8,-11.2005015173212)) ;
#141628=CARTESIAN_POINT('Ctrl Pts',(4.63586710715927,-2.78569036914628,
-11.2943752946759)) ;
#141629=CARTESIAN_POINT('Ctrl Pts',(4.65405106945726,-2.80000000000018,
-11.2795525238836)) ;
#141630=CARTESIAN_POINT('Ctrl Pts',(4.67158355065755,-2.8,-11.2592450797815)) ;
#141631=CARTESIAN_POINT('Ctrl Pts',(4.59999999999999,-2.79310344827586,
-11.2547936459578)) ;
#141632=CARTESIAN_POINT('Ctrl Pts',(4.59840954578226,-2.79314968944988,
-11.2546756726912)) ;
#141633=CARTESIAN_POINT('Ctrl Pts',(4.59737383489105,-2.7931815960622,-11.2546133239717)) ;
#141634=CARTESIAN_POINT('Ctrl Pts',(4.59650507521659,-2.79322931786012,
-11.25455037726)) ;
#141635=CARTESIAN_POINT('Ctrl Pts',(4.59632758424311,-2.79324472590582,
-11.2545345791767)) ;
#141636=CARTESIAN_POINT('Ctrl Pts',(4.5961184721085,-2.79327477162036,-11.2545047565773)) ;
#141637=CARTESIAN_POINT('Ctrl Pts',(4.59606489504931,-2.79328892979786,
-11.2544910265853)) ;
#141638=CARTESIAN_POINT('Ctrl Pts',(4.59594601677698,-2.79331605564258,
-11.254459114495)) ;
#141639=CARTESIAN_POINT('Ctrl Pts',(4.59588597444861,-2.7933285533825,-11.2544426561835)) ;
#141640=CARTESIAN_POINT('Ctrl Pts',(4.59549967474365,-2.79337285752324,
-11.2543702787606)) ;
#141641=CARTESIAN_POINT('Ctrl Pts',(4.59527331486238,-2.7934062238596,-11.2543100807084)) ;
#141642=CARTESIAN_POINT('Ctrl Pts',(4.5949320123953,-2.79346950514992,-11.2541870402937)) ;
#141643=CARTESIAN_POINT('Ctrl Pts',(4.59480393230128,-2.79349821606423,
-11.254128474279)) ;
#141644=CARTESIAN_POINT('Ctrl Pts',(4.59460326813595,-2.79353924388983,
-11.2540476351491)) ;
#141645=CARTESIAN_POINT('Ctrl Pts',(4.59455075953096,-2.79354963432651,
-11.2540274276715)) ;
#141646=CARTESIAN_POINT('Ctrl Pts',(4.59417008680875,-2.79361944405452,
-11.2538955937176)) ;
#141647=CARTESIAN_POINT('Ctrl Pts',(4.59377742096549,-2.79368602572532,
-11.2537773461555)) ;
#141648=CARTESIAN_POINT('Ctrl Pts',(4.59289939109632,-2.7938335466559,-11.2535254190241)) ;
#141649=CARTESIAN_POINT('Ctrl Pts',(4.59245006584783,-2.79390305456781,
-11.253416036199)) ;
#141650=CARTESIAN_POINT('Ctrl Pts',(4.59099552519185,-2.79413629528614,
-11.2530568524092)) ;
#141651=CARTESIAN_POINT('Ctrl Pts',(4.5900219788147,-2.79430302757336,-11.2528063701757)) ;
#141652=CARTESIAN_POINT('Ctrl Pts',(4.58861122644562,-2.79456793455724,
-11.2523921365665)) ;
#141653=CARTESIAN_POINT('Ctrl Pts',(4.5881790489434,-2.79465210327465,-11.2522585234303)) ;
#141654=CARTESIAN_POINT('Ctrl Pts',(4.58736872283365,-2.79481449815582,
-11.2519941835896)) ;
#141655=CARTESIAN_POINT('Ctrl Pts',(4.58699491219415,-2.79489135860975,
-11.2518665823581)) ;
#141656=CARTESIAN_POINT('Ctrl Pts',(4.58468897497187,-2.79537899446709,
-11.2510351906196)) ;
#141657=CARTESIAN_POINT('Ctrl Pts',(4.582907177187,-2.79577019617637,-11.2503420642284)) ;
#141658=CARTESIAN_POINT('Ctrl Pts',(4.57867627871776,-2.79666451416568,
-11.2486707882875)) ;
#141659=CARTESIAN_POINT('Ctrl Pts',(4.57626321554131,-2.79715040843618,
-11.2476877651429)) ;
#141660=CARTESIAN_POINT('Ctrl Pts',(4.57243386308706,-2.79784156172336,
-11.2461367865103)) ;
#141661=CARTESIAN_POINT('Ctrl Pts',(4.57107519984216,-2.79807176647234,
-11.245584021445)) ;
#141662=CARTESIAN_POINT('Ctrl Pts',(4.56513452430478,-2.7990007429439,-11.2431693903581)) ;
#141663=CARTESIAN_POINT('Ctrl Pts',(4.56062162665752,-2.79951267011378,
-11.2413309293495)) ;
#141664=CARTESIAN_POINT('Ctrl Pts',(4.55365420596644,-2.79992470862867,
-11.2384610302784)) ;
#141665=CARTESIAN_POINT('Ctrl Pts',(4.55124660967272,-2.79999983267432,
-11.2374632392507)) ;
#141666=CARTESIAN_POINT('Ctrl Pts',(4.54880051362942,-2.79999999972164,
-11.2364378607329)) ;
#141667=CARTESIAN_POINT('Ctrl Pts',(4.54879236166274,-2.8,-9.08356555651516)) ;
#141668=CARTESIAN_POINT('Ctrl Pts',(4.5622387183224,-2.79999999999679,-9.10123152627487)) ;
#141669=CARTESIAN_POINT('Ctrl Pts',(4.57442182196495,-2.80939476060287,
-9.11723782046681)) ;
#141670=CARTESIAN_POINT('Ctrl Pts',(4.55556842517599,-2.79999999999889,
-9.0807250640488)) ;
#141671=CARTESIAN_POINT('Ctrl Pts',(4.56783337210914,-2.80040661803736,
-9.09618630155187)) ;
#141672=CARTESIAN_POINT('Ctrl Pts',(4.57961823522365,-2.80818164104597,
-9.11001834132729)) ;
#141673=CARTESIAN_POINT('Ctrl Pts',(4.56238982831619,-2.79942602551759,
-9.07795285151706)) ;
#141674=CARTESIAN_POINT('Ctrl Pts',(4.57357810388182,-2.80014618986472,
-9.09093107214123)) ;
#141675=CARTESIAN_POINT('Ctrl Pts',(4.58462643299474,-2.80630261261112,
-9.10252327116488)) ;
#141676=CARTESIAN_POINT('Ctrl Pts',(4.57328757735258,-2.7977370397245,-9.07356999795014)) ;
#141677=CARTESIAN_POINT('Ctrl Pts',(4.58237922839514,-2.79856394574987,
-9.08226640893135)) ;
#141678=CARTESIAN_POINT('Ctrl Pts',(4.59151541127592,-2.80237286596198,
-9.09008300288059)) ;
#141679=CARTESIAN_POINT('Ctrl Pts',(4.57700059755676,-2.79703714667161,
-9.07207607634204)) ;
#141680=CARTESIAN_POINT('Ctrl Pts',(4.58532305318675,-2.79784352093717,
-9.07926254300446)) ;
#141681=CARTESIAN_POINT('Ctrl Pts',(4.59370961102546,-2.80088045369937,
-9.08574551418945)) ;
#141682=CARTESIAN_POINT('Ctrl Pts',(4.58319893207065,-2.79574016930783,
-9.06965467052113)) ;
#141683=CARTESIAN_POINT('Ctrl Pts',(4.5899041610924,-2.79637293360539,-9.07433035456224)) ;
#141684=CARTESIAN_POINT('Ctrl Pts',(4.59665800356694,-2.79825577077759,
-9.07858194486972)) ;
#141685=CARTESIAN_POINT('Ctrl Pts',(4.58534994317986,-2.79526732601294,
-9.06881886188718)) ;
#141686=CARTESIAN_POINT('Ctrl Pts',(4.59144552977844,-2.79581844972913,
-9.07262003661071)) ;
#141687=CARTESIAN_POINT('Ctrl Pts',(4.59758018705035,-2.79731769672697,
-9.07608858039388)) ;
#141688=CARTESIAN_POINT('Ctrl Pts',(4.58899927751306,-2.79450268149332,
-9.06751730126711)) ;
#141689=CARTESIAN_POINT('Ctrl Pts',(4.59386223202755,-2.79488630507105,
-9.06994951703029)) ;
#141690=CARTESIAN_POINT('Ctrl Pts',(4.59874684688641,-2.79582009356912,
-9.07218136524475)) ;
#141691=CARTESIAN_POINT('Ctrl Pts',(4.59026755692868,-2.79423885380164,
-9.06707439958003)) ;
#141692=CARTESIAN_POINT('Ctrl Pts',(4.59467706068311,-2.79455862385203,
-9.06904054333605)) ;
#141693=CARTESIAN_POINT('Ctrl Pts',(4.59910266898802,-2.79530499526365,
-9.07084863990216)) ;
#141694=CARTESIAN_POINT('Ctrl Pts',(4.59257623319517,-2.79382131826659,
-9.06638413145)) ;
#141695=CARTESIAN_POINT('Ctrl Pts',(4.59605751036346,-2.79403163929513,
-9.06762276103362)) ;
#141696=CARTESIAN_POINT('Ctrl Pts',(4.59954701072604,-2.79449510806573,
-9.06876576681698)) ;
#141697=CARTESIAN_POINT('Ctrl Pts',(4.59342976933296,-2.79367543507711,
-9.06614453745337)) ;
#141698=CARTESIAN_POINT('Ctrl Pts',(4.59655016100493,-2.79384713427256,
-9.06713488953029)) ;
#141699=CARTESIAN_POINT('Ctrl Pts',(4.59967640178298,-2.79421605292373,
-9.06805021393703)) ;
#141700=CARTESIAN_POINT('Ctrl Pts',(4.59428414179641,-2.79346156087783,
-9.06570693618526)) ;
#141701=CARTESIAN_POINT('Ctrl Pts',(4.59704519451433,-2.7935546974653,-9.06637363574795)) ;
#141702=CARTESIAN_POINT('Ctrl Pts',(4.5998104157401,-2.79379877456676,-9.06698237127069)) ;
#141703=CARTESIAN_POINT('Ctrl Pts',(4.59432658472653,-2.7933916625364,-9.06553381814949)) ;
#141704=CARTESIAN_POINT('Ctrl Pts',(4.59708408719786,-2.79345234504014,
-9.06610907664629)) ;
#141705=CARTESIAN_POINT('Ctrl Pts',(4.59984563524626,-2.79366003518351,
-9.06662765435266)) ;
#141706=CARTESIAN_POINT('Ctrl Pts',(4.59537197237733,-2.79324260992761,
-9.06528726159385)) ;
#141707=CARTESIAN_POINT('Ctrl Pts',(4.59764722167537,-2.79326383513928,
-9.065620961855)) ;
#141708=CARTESIAN_POINT('Ctrl Pts',(4.59992475053754,-2.79338190759658,
-9.06591703064758)) ;
#141709=CARTESIAN_POINT('Ctrl Pts',(4.59364183392371,-2.79313407032025,
-9.06528447884512)) ;
#141710=CARTESIAN_POINT('Ctrl Pts',(4.59684754854893,-2.79327107597598,
-9.06563893104521)) ;
#141711=CARTESIAN_POINT('Ctrl Pts',(4.59996664298755,-2.79324102308608,
-9.06556177368153)) ;
#141712=CARTESIAN_POINT('Ctrl Pts',(4.59999999999999,-2.79310344827586,
-9.06520635404224)) ;
#141713=CARTESIAN_POINT('Ctrl Pts',(4.59999999999999,-2.79310344827586,
-9.06520635404224)) ;
#141714=CARTESIAN_POINT('Ctrl Pts',(4.59999999999999,-2.79310344827586,
-9.06520635404224)) ;
#141715=CARTESIAN_POINT('Origin',(4.54879236168542,-2.9,-9.08356555651607)) ;
#141716=CARTESIAN_POINT('Ctrl Pts',(4.39959973407451,-2.8,-10.2705922428027)) ;
#141717=CARTESIAN_POINT('Ctrl Pts',(4.49922290141875,-2.8,-10.2701052483316)) ;
#141718=CARTESIAN_POINT('Ctrl Pts',(4.49980764094185,-2.8996950427637,-10.2706080458952)) ;
#141719=CARTESIAN_POINT('Ctrl Pts',(4.40142712570759,-2.8,-10.0495338960075)) ;
#141720=CARTESIAN_POINT('Ctrl Pts',(4.50593622119643,-2.8,-10.046048013468)) ;
#141721=CARTESIAN_POINT('Ctrl Pts',(4.50067611734352,-2.90411960318532,
-10.0496502871252)) ;
#141722=CARTESIAN_POINT('Ctrl Pts',(4.39573539165433,-2.8,-9.82762254178866)) ;
#141723=CARTESIAN_POINT('Ctrl Pts',(4.49039105203439,-2.8,-9.84644486600902)) ;
#141724=CARTESIAN_POINT('Ctrl Pts',(4.4979321089857,-2.89506044297338,-9.82659283506982)) ;
#141725=CARTESIAN_POINT('Ctrl Pts',(4.41164816536272,-2.8,-9.51449214865639)) ;
#141726=CARTESIAN_POINT('Ctrl Pts',(4.48203507549531,-2.8,-9.52300753838907)) ;
#141727=CARTESIAN_POINT('Ctrl Pts',(4.50604587949362,-2.86657833599726,
-9.52179163345499)) ;
#141728=CARTESIAN_POINT('Ctrl Pts',(4.41940490599909,-2.8,-9.42215713199873)) ;
#141729=CARTESIAN_POINT('Ctrl Pts',(4.48133975791564,-2.8,-9.43332746373862)) ;
#141730=CARTESIAN_POINT('Ctrl Pts',(4.50997623336224,-2.85625883833129,
-9.43306464323899)) ;
#141731=CARTESIAN_POINT('Ctrl Pts',(4.44577434373642,-2.8,-9.28702065882596)) ;
#141732=CARTESIAN_POINT('Ctrl Pts',(4.49360122670476,-2.8,-9.29933058766784)) ;
#141733=CARTESIAN_POINT('Ctrl Pts',(4.5231855860418,-2.83896465559561,-9.3054850424376)) ;
#141734=CARTESIAN_POINT('Ctrl Pts',(4.45692583760033,-2.8,-9.2424768930528)) ;
#141735=CARTESIAN_POINT('Ctrl Pts',(4.49949391572663,-2.8,-9.25605430264614)) ;
#141736=CARTESIAN_POINT('Ctrl Pts',(4.52876348458379,-2.83289258157626,
-9.26380298860431)) ;
#141737=CARTESIAN_POINT('Ctrl Pts',(4.50378503771657,-2.8,-9.12107591625827)) ;
#141738=CARTESIAN_POINT('Ctrl Pts',(4.5287351960681,-2.8,-9.13992534227475)) ;
#141739=CARTESIAN_POINT('Ctrl Pts',(4.55214466721902,-2.81552005845341,
-9.15122486980152)) ;
#141740=CARTESIAN_POINT('Ctrl Pts',(4.54714423790162,-2.8,-9.0422684950468)) ;
#141741=CARTESIAN_POINT('Ctrl Pts',(4.55761617337313,-2.8,-9.06320656418836)) ;
#141742=CARTESIAN_POINT('Ctrl Pts',(4.572595848134,-2.80338245043804,-9.08123859518892)) ;
#141743=CARTESIAN_POINT('Ctrl Pts',(4.67762904165649,-2.8,-9.05149504479602)) ;
#141744=CARTESIAN_POINT('Ctrl Pts',(4.66093484724955,-2.8,-9.06706706583778)) ;
#141745=CARTESIAN_POINT('Ctrl Pts',(4.64133868807413,-2.80368623369319,
-9.08468800638624)) ;
#141746=CARTESIAN_POINT('Origin',(4.4,-2.9,-10.1600000000039)) ;
#141747=CARTESIAN_POINT('Ctrl Pts',(4.7217278356698,-2.8000000024879,-11.2603629549123)) ;
#141748=CARTESIAN_POINT('Ctrl Pts',(4.69645430307825,-2.79999660525747,
-11.247070047311)) ;
#141749=CARTESIAN_POINT('Ctrl Pts',(4.66463283185016,-2.80454824226955,
-11.2294903682927)) ;
#141750=CARTESIAN_POINT('Ctrl Pts',(4.55709227475155,-2.80000000030524,
-11.2959964363105)) ;
#141751=CARTESIAN_POINT('Ctrl Pts',(4.56399237478739,-2.79999958643667,
-11.2739593792004)) ;
#141752=CARTESIAN_POINT('Ctrl Pts',(4.57729370999484,-2.80055804294512,
-11.2551759050809)) ;
#141753=CARTESIAN_POINT('Ctrl Pts',(4.50667826286321,-2.80000000784871,
-11.2066146479981)) ;
#141754=CARTESIAN_POINT('Ctrl Pts',(4.53037382014981,-2.79998899178922,
-11.1870846001166)) ;
#141755=CARTESIAN_POINT('Ctrl Pts',(4.55348183854634,-2.81434699509191,
-11.1759466041139)) ;
#141756=CARTESIAN_POINT('Ctrl Pts',(4.45692280158725,-2.80000001789831,
-11.0776422182876)) ;
#141757=CARTESIAN_POINT('Ctrl Pts',(4.4993802926736,-2.79997354447563,-11.0640998880094)) ;
#141758=CARTESIAN_POINT('Ctrl Pts',(4.52864149761196,-2.83271033979,-11.05632906208)) ;
#141759=CARTESIAN_POINT('Ctrl Pts',(4.44554661086166,-2.80000002126189,
-11.032377440014)) ;
#141760=CARTESIAN_POINT('Ctrl Pts',(4.49333665154849,-2.7999679796365,-11.0200969398739)) ;
#141761=CARTESIAN_POINT('Ctrl Pts',(4.52295544156351,-2.83885474437117,
-11.013967858228)) ;
#141762=CARTESIAN_POINT('Ctrl Pts',(4.41903322104334,-2.8000000307772,-10.8958947975772)) ;
#141763=CARTESIAN_POINT('Ctrl Pts',(4.4810061608023,-2.79995095769182,-10.8847300040205)) ;
#141764=CARTESIAN_POINT('Ctrl Pts',(4.50969337368895,-2.85623179093863,
-10.885069623609)) ;
#141765=CARTESIAN_POINT('Ctrl Pts',(4.41147189908675,-2.8000000363501,-10.8042415900435)) ;
#141766=CARTESIAN_POINT('Ctrl Pts',(4.48178828424046,-2.79993989905029,
-10.7957891492056)) ;
#141767=CARTESIAN_POINT('Ctrl Pts',(4.50589025525737,-2.86640526991131,
-10.7969681512011)) ;
#141768=CARTESIAN_POINT('Ctrl Pts',(4.39523119070911,-2.80000005228415,
-10.4831795198329)) ;
#141769=CARTESIAN_POINT('Ctrl Pts',(4.4903383634589,-2.79990261688304,-10.4630741316606)) ;
#141770=CARTESIAN_POINT('Ctrl Pts',(4.49769757367176,-2.89547737952985,
-10.4843332157617)) ;
#141771=CARTESIAN_POINT('Ctrl Pts',(4.40178225889357,-2.80000005718968,
-10.2526239782851)) ;
#141772=CARTESIAN_POINT('Ctrl Pts',(4.50681341018175,-2.79988784121843,
-10.2570581988245)) ;
#141773=CARTESIAN_POINT('Ctrl Pts',(4.50092255053476,-2.90441958896084,
-10.2524406960391)) ;
#141774=CARTESIAN_POINT('Ctrl Pts',(4.39924589760307,-2.80000005405717,
-10.0230311688801)) ;
#141775=CARTESIAN_POINT('Ctrl Pts',(4.49795607191393,-2.79989746608217,
-10.023922937496)) ;
#141776=CARTESIAN_POINT('Ctrl Pts',(4.49968270404898,-2.89870974459553,
-10.0230284945916)) ;
#141777=CARTESIAN_POINT('Origin',(4.54879236168626,-2.9,-11.2364344434846)) ;
#141778=CARTESIAN_POINT('Ctrl Pts',(4.57442492185553,-2.809397151199,-11.2027581068621)) ;
#141779=CARTESIAN_POINT('Ctrl Pts',(4.56210583156796,-2.7998961275033,-11.2189430617887)) ;
#141780=CARTESIAN_POINT('Ctrl Pts',(4.54850917782857,-2.80000109307748,
-11.2368064934881)) ;
#141781=CARTESIAN_POINT('Ctrl Pts',(4.57959763980856,-2.80818914940072,
-11.2099453004955)) ;
#141782=CARTESIAN_POINT('Ctrl Pts',(4.56768008075465,-2.80031924975225,
-11.2239410457291)) ;
#141783=CARTESIAN_POINT('Ctrl Pts',(4.55527876038347,-2.79999229227378,
-11.2395899763868)) ;
#141784=CARTESIAN_POINT('Ctrl Pts',(4.58464248447265,-2.80630474344638,
-11.2174843126383)) ;
#141785=CARTESIAN_POINT('Ctrl Pts',(4.57346944634371,-2.80008318972135,
-11.2292012910522)) ;
#141786=CARTESIAN_POINT('Ctrl Pts',(4.56216307187795,-2.79941338753917,
-11.2423280915335)) ;
#141787=CARTESIAN_POINT('Ctrl Pts',(4.59159231899494,-2.80232720646228,
-11.2300563692959)) ;
#141788=CARTESIAN_POINT('Ctrl Pts',(4.58237910662986,-2.79850221241048,
-11.2379149362578)) ;
#141789=CARTESIAN_POINT('Ctrl Pts',(4.57321634584968,-2.79769868647539,
-11.2466644864947)) ;
#141790=CARTESIAN_POINT('Ctrl Pts',(4.59378564167737,-2.8008235544484,-11.2344145837654)) ;
#141791=CARTESIAN_POINT('Ctrl Pts',(4.58533966160572,-2.79778056279966,
-11.2409180694478)) ;
#141792=CARTESIAN_POINT('Ctrl Pts',(4.5769613009382,-2.79699227428059,-11.2481320740362)) ;
#141793=CARTESIAN_POINT('Ctrl Pts',(4.59669734138576,-2.79821861236081,
-11.2415174469091)) ;
#141794=CARTESIAN_POINT('Ctrl Pts',(4.58989502505307,-2.79633072300511,
-11.245783702985)) ;
#141795=CARTESIAN_POINT('Ctrl Pts',(4.58314295739386,-2.79570785369251,
-11.2504789031814)) ;
#141796=CARTESIAN_POINT('Ctrl Pts',(4.59760632414569,-2.79728965034655,
-11.2439852466291)) ;
#141797=CARTESIAN_POINT('Ctrl Pts',(4.59142619397023,-2.79578507327358,
-11.2474678937229)) ;
#141798=CARTESIAN_POINT('Ctrl Pts',(4.58528630332434,-2.79524119148169,
-11.251287378375)) ;
#141799=CARTESIAN_POINT('Ctrl Pts',(4.59875741430933,-2.79580683383093,
-11.247853004496)) ;
#141800=CARTESIAN_POINT('Ctrl Pts',(4.59383193680337,-2.79486773439436,
-11.2500980055339)) ;
#141801=CARTESIAN_POINT('Ctrl Pts',(4.58892874314202,-2.79448758877844,
-11.2525464730129)) ;
#141802=CARTESIAN_POINT('Ctrl Pts',(4.59910834609947,-2.79529718130591,
-11.2491714993014)) ;
#141803=CARTESIAN_POINT('Ctrl Pts',(4.59464343907624,-2.79454543406795,
-11.2509926958501)) ;
#141804=CARTESIAN_POINT('Ctrl Pts',(4.59019511689903,-2.79422790851556,
-11.2529746712091)) ;
#141805=CARTESIAN_POINT('Ctrl Pts',(4.59954688679867,-2.79449699552072,
-11.2512293846587)) ;
#141806=CARTESIAN_POINT('Ctrl Pts',(4.59601732089133,-2.79402779797774,
-11.2523863363518)) ;
#141807=CARTESIAN_POINT('Ctrl Pts',(4.59249627585267,-2.79381771894921,
-11.2536411141675)) ;
#141808=CARTESIAN_POINT('Ctrl Pts',(4.59967529310588,-2.79422450025963,
-11.2519354645612)) ;
#141809=CARTESIAN_POINT('Ctrl Pts',(4.59651100242295,-2.79384821317135,
-11.2528644108735)) ;
#141810=CARTESIAN_POINT('Ctrl Pts',(4.593352874124,-2.79367727499394,-11.2538714476574)) ;
#141811=CARTESIAN_POINT('Ctrl Pts',(4.59980981518572,-2.79380630943631,
-11.2530056452101)) ;
#141812=CARTESIAN_POINT('Ctrl Pts',(4.59701056623719,-2.79355888022806,
-11.2536249350365)) ;
#141813=CARTESIAN_POINT('Ctrl Pts',(4.59421559911326,-2.79346462438277,
-11.2543030289899)) ;
#141814=CARTESIAN_POINT('Ctrl Pts',(4.59984534134842,-2.79366726490194,
-11.2533646067489)) ;
#141815=CARTESIAN_POINT('Ctrl Pts',(4.59705039509825,-2.79345667046145,
-11.2538917393962)) ;
#141816=CARTESIAN_POINT('Ctrl Pts',(4.59425962044003,-2.79339574833516,
-11.2544765637043)) ;
#141817=CARTESIAN_POINT('Ctrl Pts',(4.59992484646001,-2.7933873519883,-11.25407980384)) ;
#141818=CARTESIAN_POINT('Ctrl Pts',(4.59761652863209,-2.79326682373741,
-11.254380589531)) ;
#141819=CARTESIAN_POINT('Ctrl Pts',(4.59531061070857,-2.79324678512396,
-11.2547204137335)) ;
#141820=CARTESIAN_POINT('Ctrl Pts',(4.59996721368508,-2.79324340897637,
-11.254436569794)) ;
#141821=CARTESIAN_POINT('Ctrl Pts',(4.59680854952869,-2.79327323421043,
-11.2543604778616)) ;
#141822=CARTESIAN_POINT('Ctrl Pts',(4.59356174266138,-2.79313094944462,
-11.2547234833207)) ;
#141823=CARTESIAN_POINT('Ctrl Pts',(4.59999999999999,-2.79310344827586,
-11.2547936459578)) ;
#141824=CARTESIAN_POINT('Ctrl Pts',(4.59999999999999,-2.79310344827586,
-11.2547936459578)) ;
#141825=CARTESIAN_POINT('Ctrl Pts',(4.59999999999999,-2.79310344827586,
-11.2547936459578)) ;
#170119=UNCERTAINTY_MEASURE_WITH_UNIT(LENGTH_MEASURE(0.01),#170128,
'DISTANCE_ACCURACY_VALUE',
'Maximum model space distance between geometric entities at asserted c
onnectivities') ;
#170122=UNCERTAINTY_MEASURE_WITH_UNIT(LENGTH_MEASURE(0.01),#170128,
'DISTANCE_ACCURACY_VALUE',
'Maximum model space distance between geometric entities at asserted c
onnectivities') ;
#170124=(
GEOMETRIC_REPRESENTATION_CONTEXT(3)
GLOBAL_UNCERTAINTY_ASSIGNED_CONTEXT((#170119))
GLOBAL_UNIT_ASSIGNED_CONTEXT((#170128,#170130,#170131))
REPRESENTATION_CONTEXT('','3D')
) ;
#170127=(
GEOMETRIC_REPRESENTATION_CONTEXT(3)
GLOBAL_UNCERTAINTY_ASSIGNED_CONTEXT((#170122))
GLOBAL_UNIT_ASSIGNED_CONTEXT((#170128,#170130,#170131))
REPRESENTATION_CONTEXT('','3D')
) ;
#170128=(
LENGTH_UNIT()
NAMED_UNIT(*)
SI_UNIT(.MILLI.,.METRE.)
) ;
#170130=(
NAMED_UNIT(*)
PLANE_ANGLE_UNIT()
SI_UNIT($,.RADIAN.)
) ;
#170131=(
NAMED_UNIT(*)
SI_UNIT($,.STERADIAN.)
SOLID_ANGLE_UNIT()
) ;
#170133=SHAPE_DEFINITION_REPRESENTATION(#170137,#170144) ;
#170137=PRODUCT_DEFINITION_SHAPE('',$,#170149) ;
#170144=SHAPE_REPRESENTATION('',(#91123),#170124) ;
#170147=PRODUCT_DEFINITION_CONTEXT('part definition',#170161,'design') ;
#170149=PRODUCT_DEFINITION('Pin_Header_Plug','Pin_Header_Plug',#170153,
#170147) ;
#170153=PRODUCT_DEFINITION_FORMATION('',$,#170164) ;
#170161=APPLICATION_CONTEXT(
'Core Data for Automotive Mechanical Design Process') ;
#170162=PRODUCT_CONTEXT('part definition',#170161,'mechanical') ;
#170164=PRODUCT('Pin_Header_Plug','Pin_Header_Plug',$,(#170162)) ;
#170168=PRESENTATION_STYLE_ASSIGNMENT((#170174)) ;
#170169=PRESENTATION_STYLE_ASSIGNMENT((#170175)) ;
#170170=PRESENTATION_STYLE_ASSIGNMENT((#170176)) ;
#170171=PRESENTATION_STYLE_ASSIGNMENT((#170177)) ;
#170174=SURFACE_STYLE_USAGE(.BOTH.,#170180) ;
#170175=SURFACE_STYLE_USAGE(.BOTH.,#170181) ;
#170176=SURFACE_STYLE_USAGE(.BOTH.,#170182) ;
#170177=SURFACE_STYLE_USAGE(.BOTH.,#170183) ;
#170180=SURFACE_SIDE_STYLE('',(#170186)) ;
#170181=SURFACE_SIDE_STYLE('',(#170187)) ;
#170182=SURFACE_SIDE_STYLE('',(#170188)) ;
#170183=SURFACE_SIDE_STYLE('',(#170189)) ;
#170186=SURFACE_STYLE_FILL_AREA(#170192) ;
#170187=SURFACE_STYLE_FILL_AREA(#170193) ;
#170188=SURFACE_STYLE_FILL_AREA(#170194) ;
#170189=SURFACE_STYLE_FILL_AREA(#170195) ;
#170192=FILL_AREA_STYLE('Opaque(202,209,238)',(#170198)) ;
#170193=FILL_AREA_STYLE('Opaque(128,255,128)',(#170199)) ;
#170194=FILL_AREA_STYLE('Opaque(189,191,0)',(#170200)) ;
#170195=FILL_AREA_STYLE('Opaque(204,207,204)',(#170201)) ;
#170198=FILL_AREA_STYLE_COLOUR('Opaque(202,209,238)',#170204) ;
#170199=FILL_AREA_STYLE_COLOUR('Opaque(128,255,128)',#170205) ;
#170200=FILL_AREA_STYLE_COLOUR('Opaque(189,191,0)',#170206) ;
#170201=FILL_AREA_STYLE_COLOUR('Opaque(204,207,204)',#170207) ;
#170204=COLOUR_RGB('Opaque(202,209,238)', 0.09019608, 0.27058824, 0.51372549) ;
#170205=COLOUR_RGB('Opaque(128,255,128)', 0.09019608, 0.27058824, 0.51372549) ;
#170206=COLOUR_RGB('Opaque(189,191,0)', 0.72549020, 0.75294118, 0.79215686) ;
#170207=COLOUR_RGB('Opaque(204,207,204)', 0.09019608, 0.27058824, 0.51372549) ;
ENDSEC;
END-ISO-10303-21;
